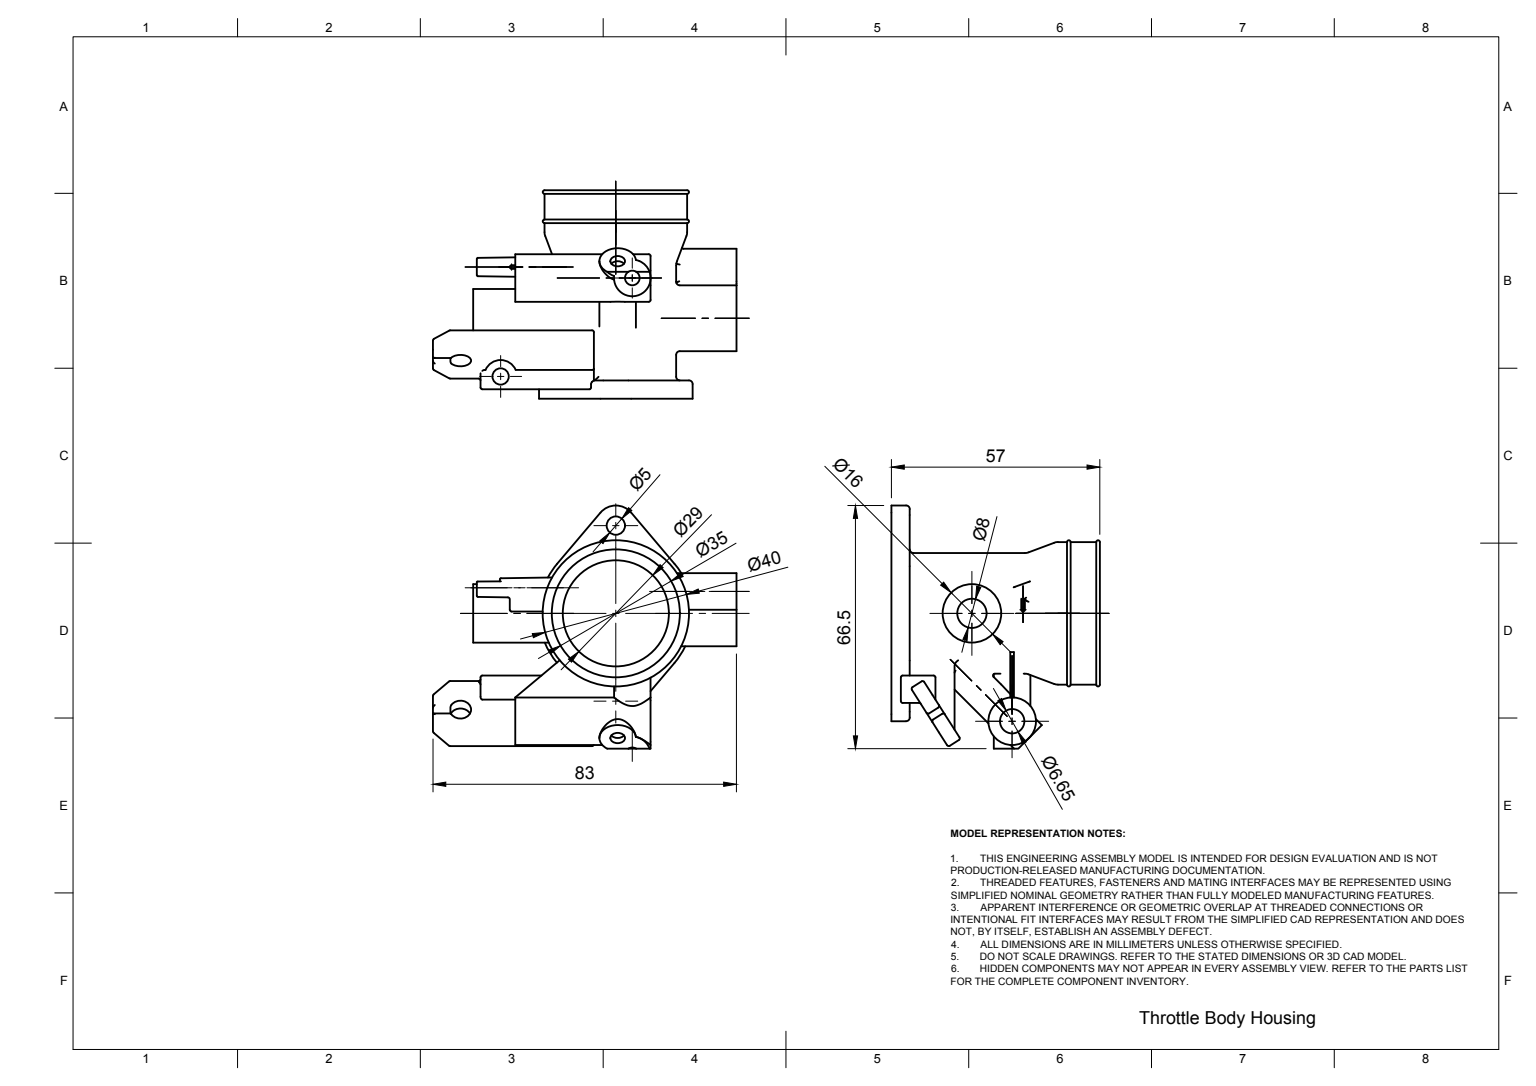
ISO-10303-21;
HEADER;
/* Generated by software containing ST-Developer
 * from STEP Tools, Inc. (www.steptools.com) 
 */

FILE_DESCRIPTION(
/* description */ ('STEP AP214'),
/* implementation_level */ '2;1');

FILE_NAME(
/* name */ 'Throttle Body Housing.step',
/* time_stamp */ '2026-10-07T12:18:07-07:00',
/* author */ (''),
/* organization */ (''),
/* preprocessor_version */ 'ST-DEVELOPER v20.2',
/* originating_system */ 'Autodesk Translation Framework v15.15.0.0',
/* authorisation */ '');

FILE_SCHEMA (('AUTOMOTIVE_DESIGN { 1 0 10303 214 3 1 1 }'));
ENDSEC;

DATA;
#10=MECHANICAL_DESIGN_GEOMETRIC_PRESENTATION_REPRESENTATION('',(#130),#62974);
#83=SPHERICAL_SURFACE('',#16593,0.5);
#84=SPHERICAL_SURFACE('',#16603,0.5);
#85=SPHERICAL_SURFACE('',#16608,0.5);
#86=SPHERICAL_SURFACE('',#16674,0.5);
#87=SPHERICAL_SURFACE('',#16680,0.5);
#88=SPHERICAL_SURFACE('',#16687,0.5);
#89=SPHERICAL_SURFACE('',#16695,0.5);
#90=SPHERICAL_SURFACE('',#16702,0.5);
#91=SPHERICAL_SURFACE('',#16709,0.5);
#92=SPHERICAL_SURFACE('',#16717,0.5);
#93=SPHERICAL_SURFACE('',#16725,0.5);
#94=SPHERICAL_SURFACE('',#16730,0.5);
#95=SPHERICAL_SURFACE('',#16733,0.5);
#96=SPHERICAL_SURFACE('',#16778,0.5);
#97=SPHERICAL_SURFACE('',#16816,1.);
#106=SHAPE_REPRESENTATION_RELATIONSHIP('SRR','None',#63029,#118);
#118=ADVANCED_BREP_SHAPE_REPRESENTATION('',(#142),#62970);
#130=STYLED_ITEM('',(#63090),#142);
#142=MANIFOLD_SOLID_BREP('Body1',#15200);
#168=(
BOUNDED_SURFACE()
B_SPLINE_SURFACE(3,2,((#50715,#50716,#50717),(#50718,#50719,#50720),(#50721,
#50722,#50723),(#50724,#50725,#50726),(#50727,#50728,#50729),(#50730,#50731,
#50732),(#50733,#50734,#50735),(#50736,#50737,#50738),(#50739,#50740,#50741),
(#50742,#50743,#50744),(#50745,#50746,#50747),(#50748,#50749,#50750),(#50751,
#50752,#50753),(#50754,#50755,#50756),(#50757,#50758,#50759),(#50760,#50761,
#50762),(#50763,#50764,#50765),(#50766,#50767,#50768),(#50769,#50770,#50771),
(#50772,#50773,#50774),(#50775,#50776,#50777),(#50778,#50779,#50780),(#50781,
#50782,#50783),(#50784,#50785,#50786),(#50787,#50788,#50789),(#50790,#50791,
#50792),(#50793,#50794,#50795),(#50796,#50797,#50798),(#50799,#50800,#50801),
(#50802,#50803,#50804),(#50805,#50806,#50807),(#50808,#50809,#50810),(#50811,
#50812,#50813),(#50814,#50815,#50816),(#50817,#50818,#50819),(#50820,#50821,
#50822),(#50823,#50824,#50825),(#50826,#50827,#50828),(#50829,#50830,#50831),
(#50832,#50833,#50834),(#50835,#50836,#50837),(#50838,#50839,#50840),(#50841,
#50842,#50843),(#50844,#50845,#50846),(#50847,#50848,#50849),(#50850,#50851,
#50852),(#50853,#50854,#50855),(#50856,#50857,#50858),(#50859,#50860,#50861),
(#50862,#50863,#50864),(#50865,#50866,#50867),(#50868,#50869,#50870),(#50871,
#50872,#50873),(#50874,#50875,#50876),(#50877,#50878,#50879),(#50880,#50881,
#50882),(#50883,#50884,#50885),(#50886,#50887,#50888),(#50889,#50890,#50891),
(#50892,#50893,#50894),(#50895,#50896,#50897),(#50898,#50899,#50900),(#50901,
#50902,#50903),(#50904,#50905,#50906),(#50907,#50908,#50909),(#50910,#50911,
#50912),(#50913,#50914,#50915),(#50916,#50917,#50918),(#50919,#50920,#50921),
(#50922,#50923,#50924),(#50925,#50926,#50927),(#50928,#50929,#50930),(#50931,
#50932,#50933),(#50934,#50935,#50936),(#50937,#50938,#50939),(#50940,#50941,
#50942),(#50943,#50944,#50945),(#50946,#50947,#50948),(#50949,#50950,#50951),
(#50952,#50953,#50954),(#50955,#50956,#50957),(#50958,#50959,#50960),(#50961,
#50962,#50963),(#50964,#50965,#50966),(#50967,#50968,#50969),(#50970,#50971,
#50972),(#50973,#50974,#50975),(#50976,#50977,#50978),(#50979,#50980,#50981),
(#50982,#50983,#50984),(#50985,#50986,#50987),(#50988,#50989,#50990),(#50991,
#50992,#50993),(#50994,#50995,#50996),(#50997,#50998,#50999),(#51000,#51001,
#51002),(#51003,#51004,#51005),(#51006,#51007,#51008),(#51009,#51010,#51011),
(#51012,#51013,#51014),(#51015,#51016,#51017),(#51018,#51019,#51020),(#51021,
#51022,#51023),(#51024,#51025,#51026),(#51027,#51028,#51029),(#51030,#51031,
#51032),(#51033,#51034,#51035),(#51036,#51037,#51038),(#51039,#51040,#51041),
(#51042,#51043,#51044),(#51045,#51046,#51047),(#51048,#51049,#51050),(#51051,
#51052,#51053),(#51054,#51055,#51056),(#51057,#51058,#51059),(#51060,#51061,
#51062),(#51063,#51064,#51065),(#51066,#51067,#51068),(#51069,#51070,#51071),
(#51072,#51073,#51074),(#51075,#51076,#51077),(#51078,#51079,#51080),(#51081,
#51082,#51083),(#51084,#51085,#51086),(#51087,#51088,#51089),(#51090,#51091,
#51092),(#51093,#51094,#51095),(#51096,#51097,#51098),(#51099,#51100,#51101),
(#51102,#51103,#51104),(#51105,#51106,#51107),(#51108,#51109,#51110),(#51111,
#51112,#51113),(#51114,#51115,#51116),(#51117,#51118,#51119),(#51120,#51121,
#51122),(#51123,#51124,#51125),(#51126,#51127,#51128),(#51129,#51130,#51131),
(#51132,#51133,#51134),(#51135,#51136,#51137),(#51138,#51139,#51140),(#51141,
#51142,#51143),(#51144,#51145,#51146),(#51147,#51148,#51149),(#51150,#51151,
#51152),(#51153,#51154,#51155),(#51156,#51157,#51158),(#51159,#51160,#51161),
(#51162,#51163,#51164),(#51165,#51166,#51167),(#51168,#51169,#51170),(#51171,
#51172,#51173),(#51174,#51175,#51176),(#51177,#51178,#51179),(#51180,#51181,
#51182),(#51183,#51184,#51185),(#51186,#51187,#51188),(#51189,#51190,#51191),
(#51192,#51193,#51194),(#51195,#51196,#51197),(#51198,#51199,#51200),(#51201,
#51202,#51203),(#51204,#51205,#51206),(#51207,#51208,#51209),(#51210,#51211,
#51212),(#51213,#51214,#51215),(#51216,#51217,#51218),(#51219,#51220,#51221),
(#51222,#51223,#51224),(#51225,#51226,#51227),(#51228,#51229,#51230),(#51231,
#51232,#51233),(#51234,#51235,#51236),(#51237,#51238,#51239),(#51240,#51241,
#51242),(#51243,#51244,#51245),(#51246,#51247,#51248),(#51249,#51250,#51251),
(#51252,#51253,#51254),(#51255,#51256,#51257),(#51258,#51259,#51260),(#51261,
#51262,#51263),(#51264,#51265,#51266),(#51267,#51268,#51269),(#51270,#51271,
#51272),(#51273,#51274,#51275),(#51276,#51277,#51278),(#51279,#51280,#51281),
(#51282,#51283,#51284),(#51285,#51286,#51287),(#51288,#51289,#51290),(#51291,
#51292,#51293),(#51294,#51295,#51296),(#51297,#51298,#51299),(#51300,#51301,
#51302),(#51303,#51304,#51305),(#51306,#51307,#51308),(#51309,#51310,#51311),
(#51312,#51313,#51314),(#51315,#51316,#51317),(#51318,#51319,#51320),(#51321,
#51322,#51323),(#51324,#51325,#51326),(#51327,#51328,#51329),(#51330,#51331,
#51332),(#51333,#51334,#51335),(#51336,#51337,#51338),(#51339,#51340,#51341),
(#51342,#51343,#51344),(#51345,#51346,#51347),(#51348,#51349,#51350),(#51351,
#51352,#51353),(#51354,#51355,#51356),(#51357,#51358,#51359),(#51360,#51361,
#51362),(#51363,#51364,#51365),(#51366,#51367,#51368),(#51369,#51370,#51371),
(#51372,#51373,#51374),(#51375,#51376,#51377),(#51378,#51379,#51380),(#51381,
#51382,#51383),(#51384,#51385,#51386),(#51387,#51388,#51389),(#51390,#51391,
#51392),(#51393,#51394,#51395),(#51396,#51397,#51398),(#51399,#51400,#51401),
(#51402,#51403,#51404),(#51405,#51406,#51407),(#51408,#51409,#51410),(#51411,
#51412,#51413),(#51414,#51415,#51416),(#51417,#51418,#51419),(#51420,#51421,
#51422),(#51423,#51424,#51425),(#51426,#51427,#51428),(#51429,#51430,#51431),
(#51432,#51433,#51434),(#51435,#51436,#51437),(#51438,#51439,#51440),(#51441,
#51442,#51443),(#51444,#51445,#51446),(#51447,#51448,#51449),(#51450,#51451,
#51452),(#51453,#51454,#51455),(#51456,#51457,#51458),(#51459,#51460,#51461),
(#51462,#51463,#51464),(#51465,#51466,#51467),(#51468,#51469,#51470),(#51471,
#51472,#51473),(#51474,#51475,#51476),(#51477,#51478,#51479),(#51480,#51481,
#51482),(#51483,#51484,#51485),(#51486,#51487,#51488),(#51489,#51490,#51491),
(#51492,#51493,#51494),(#51495,#51496,#51497),(#51498,#51499,#51500)),
 .UNSPECIFIED.,.T.,.F.,.F.)
B_SPLINE_SURFACE_WITH_KNOTS((4,2,2,2,2,2,2,2,2,2,2,2,2,2,2,2,2,2,2,2,2,
2,2,2,2,2,2,2,2,2,2,2,2,2,2,2,2,2,2,2,2,2,2,2,2,2,2,2,2,2,2,2,2,2,2,2,2,
2,2,2,2,2,2,2,2,2,2,2,2,2,2,2,2,2,2,2,2,2,2,2,2,2,2,2,2,2,2,2,2,2,2,2,2,
2,2,2,2,2,2,2,2,2,2,2,2,2,2,2,2,2,2,2,2,2,2,2,2,2,2,2,2,2,2,2,2,2,2,2,2,
2,4),(3,3),(0.,5.58974039156775E-5,0.000111794807831355,0.00022358961566271,
0.00044717923132542,0.000894358462650841,0.00178871692530168,0.00268307538795252,
0.00279487019578388,0.00290666500361523,0.00313025461927794,0.00357743385060336,
0.0044717923132542,0.00536615077590504,0.0054779455837364,0.00558974039156775,
0.00581333000723046,0.00626050923855589,0.00715486770120673,0.00804922616385757,
0.00827281577952028,0.00838461058735163,0.00849640539518299,0.00894358462650841,
0.00983794308915925,0.0107323015518101,0.0111794807831355,0.0114030703987982,
0.0115148652066296,0.0116266600144609,0.0125210184771118,0.0134153769397626,
0.013862556171088,0.0143097354024135,0.0145333250180762,0.0146451198259075,
0.0147569146337389,0.0152040938650643,0.0160984523277151,0.016992810790366,
0.0172164004060287,0.01732819521386,0.0174399900216914,0.0178871692530168,
0.0187815277156677,0.0196758861783185,0.0198994757939812,0.0201230654096439,
0.0205702446409693,0.0214646031036202,0.022358961566271,0.0228061407975964,
0.0230297304132591,0.0232533200289219,0.0241476784915727,0.0250420369542235,
0.0259363954168744,0.0261599850325371,0.0262717798403685,0.0263835746481998,
0.0268307538795252,0.0277251123421761,0.0286194708048269,0.0290666500361523,
0.029290239651815,0.0294020344596464,0.0295138292674777,0.0299610084988032,
0.0301845981144659,0.0302963929222972,0.0304081877301286,0.0313025461927794,
0.0321969046554303,0.0330912631180811,0.0332030579259125,0.0333148527337438,
0.0335384423494065,0.0339856215807319,0.0348799800433828,0.0357743385060336,
0.0359979281216963,0.0361097229295277,0.036221517737359,0.0366686969686845,
0.0375630554313353,0.0384574138939862,0.0389045931253116,0.0391281827409743,
0.0392399775488056,0.039351772356637,0.0402461308192878,0.0411404892819387,
0.0420348477445895,0.0424820269759149,0.0425938217837463,0.0427056165915777,
0.0429292062072404,0.0433763854385658,0.0438235646698912,0.044717923132542,
0.0451651023638675,0.0452768971716988,0.0453886919795302,0.0456122815951929,
0.0465066400578437,0.0474009985204946,0.04784817775182,0.0479599725596513,
0.0480717673674827,0.0482953569831454,0.0491897154457962,0.0500840739084471,
0.0505312531397725,0.0507548427554352,0.0508666375632666,0.0509784323710979,
0.0518727908337488,0.0527671492963996,0.0536615077590504,0.0538850973747132,
0.0539968921825445,0.0541086869903759,0.0545558662217013,0.0554502246843521,
0.056344583147003,0.0567917623783284,0.0570153519939911,0.0571271468018225,
0.0571830442057381,0.057210992907696,0.0572389416096538),(0.,1.),
 .UNSPECIFIED.)
GEOMETRIC_REPRESENTATION_ITEM()
RATIONAL_B_SPLINE_SURFACE(((1.,0.869037098890924,1.),(1.,0.869090662160833,
1.),(1.,0.869142132128297,1.),(1.,0.869241273997536,1.),(1.,0.869288882663707,
1.),(1.,0.869425835273797,1.),(1.,0.869509305917427,1.),(1.,0.869736328335375,
1.),(1.,0.869856492063896,1.),(1.,0.870124205131434,1.),(1.,0.870178998389397,
1.),(1.,0.869977707911342,1.),(1.,0.869356264735848,1.),(1.,0.867159523791841,
1.),(1.,0.865584183970151,1.),(1.,0.863281618119441,1.),(1.,0.86301835474559,
1.),(1.,0.862477312320675,1.),(1.,0.862200065545979,1.),(1.,0.861348450829986,
1.),(1.,0.860754210958995,1.),(1.,0.858894323573958,1.),(1.,0.857551540639133,
1.),(1.,0.853231873120265,1.),(1.,0.849963976579328,1.),(1.,0.8427337476379,
1.),(1.,0.838771159914112,1.),(1.,0.833964492549446,1.),(1.,0.83342564158097,
1.),(1.,0.832341102831786,1.),(1.,0.831795088875303,1.),(1.,0.83014615568217,
1.),(1.,0.829032346207458,1.),(1.,0.825650047625046,1.),(1.,0.823340697393356,
1.),(1.,0.816270214875414,1.),(1.,0.811366531889991,1.),(1.,0.801290493401484,
1.),(1.,0.796117786007922,1.),(1.,0.789558114002489,1.),(1.,0.788241524410975,
1.),(1.,0.786261176106014,1.),(1.,0.785600666410631,1.),(1.,0.784281253478811,
1.),(1.,0.783622032027989,1.),(1.,0.780329023537139,1.),(1.,0.777704514650253,
1.),(1.,0.76988692542286,1.),(1.,0.764749330047637,1.),(1.,0.75477051537079,
1.),(1.,0.749929030998746,1.),(1.,0.743012971461713,1.),(1.,0.740765474239869,
1.),(1.,0.73749827976927,1.),(1.,0.736426570328376,1.),(1.,0.734847329496033,
1.),(1.,0.734325595116705,1.),(1.,0.733292134556225,1.),(1.,0.732781563072735,
1.),(1.,0.728242967029025,1.),(1.,0.724610876621003,1.),(1.,0.718276943716503,
1.),(1.,0.715575135642169,1.),(1.,0.712312229125148,1.),(1.,0.711356200483893,
1.),(1.,0.709722323386846,1.),(1.,0.709044475655852,1.),(1.,0.708247344579823,
1.),(1.,0.708018238565296,1.),(1.,0.707730840005604,1.),(1.,0.707644376240716,
1.),(1.,0.707490608795043,1.),(1.,0.707423402545753,1.),(1.,0.707135559015692,
1.),(1.,0.707059523314824,1.),(1.,0.707285549205988,1.),(1.,0.708042221657254,
1.),(1.,0.710710092253751,1.),(1.,0.712621237041365,1.),(1.,0.715686665981657,
1.),(1.,0.716333543550958,1.),(1.,0.717353607349392,1.),(1.,0.717701919486094,
1.),(1.,0.718414964313171,1.),(1.,0.718779962361759,1.),(1.,0.720642167884513,
1.),(1.,0.722248110686464,1.),(1.,0.727379897082438,1.),(1.,0.731219242886661,
1.),(1.,0.739562059134817,1.),(1.,0.744065650037015,1.),(1.,0.750011006364496,
1.),(1.,0.751215898212902,1.),(1.,0.753654939425893,1.),(1.,0.754889413958793,
1.),(1.,0.758631191877784,1.),(1.,0.761160349547001,1.),(1.,0.768820010203822,
1.),(1.,0.774022074432147,1.),(1.,0.784467204631247,1.),(1.,0.789710609506525,
1.),(1.,0.797506397811445,1.),(1.,0.800093535602747,1.),(1.,0.803945021596591,
1.),(1.,0.805223982229172,1.),(1.,0.807770172561434,1.),(1.,0.80903292134295,
1.),(1.,0.815288089794111,1.),(1.,0.820107499923359,1.),(1.,0.829279685729609,
1.),(1.,0.833632779776828,1.),(1.,0.841777168809211,1.),(1.,0.845568802174027,
1.),(1.,0.849892563199079,1.),(1.,0.850736491533872,1.),(1.,0.851969804909359,
1.),(1.,0.852375793676684,1.),(1.,0.853174988795519,1.),(1.,0.853568068159912,
1.),(1.,0.855500704900974,1.),(1.,0.856941996550435,1.),(1.,0.860944601199298,
1.),(1.,0.863184927882986,1.),(1.,0.866767461005655,1.),(1.,0.868109793594765,
1.),(1.,0.869410481594525,1.),(1.,0.869725148569242,1.),(1.,0.870012890040282,
1.),(1.,0.870078086396283,1.),(1.,0.870128990964309,1.),(1.,0.870138141570321,
1.),(1.,0.870140676091054,1.),(1.,0.870134072965078,1.),(1.,0.870061808448095,
1.),(1.,0.869878426760649,1.),(1.,0.869416656440071,1.),(1.,0.869231611413219,
1.),(1.,0.868907522254946,1.),(1.,0.868791738615037,1.),(1.,0.868544686539316,
1.),(1.,0.868413337134317,1.),(1.,0.867163505604549,1.),(1.,0.865575442228637,
1.),(1.,0.861527724393334,1.),(1.,0.859067845844723,1.),(1.,0.853343564886148,
1.),(1.,0.850078971827717,1.),(1.,0.84598647975218,1.),(1.,0.845525923915504,
1.),(1.,0.844593252383724,1.),(1.,0.84412081177775,1.),(1.,0.842688930644052,
1.),(1.,0.841715504172781,1.),(1.,0.83874140215334,1.),(1.,0.836686926299113,
1.),(1.,0.830328826430023,1.),(1.,0.825830615536545,1.),(1.,0.816419106847222,
1.),(1.,0.81150547118942,1.),(1.,0.805169234170547,1.),(1.,0.803892294076685,
1.),(1.,0.801963643202623,1.),(1.,0.801318553163188,1.),(1.,0.800024181787751,
1.),(1.,0.799374551464301,1.),(1.,0.796123838581708,1.),(1.,0.793511112507122,
1.),(1.,0.785661232785625,1.),(1.,0.780412024366977,1.),(1.,0.770019050951368,
1.),(1.,0.76487497595969,1.),(1.,0.757351702086758,1.),(1.,0.754876228736365,
1.),(1.,0.751227350622943,1.),(1.,0.750021792912108,1.),(1.,0.748231675946372,
1.),(1.,0.747638007827609,1.),(1.,0.746457111568753,1.),(1.,0.745869506104255,
1.),(1.,0.740620037686994,1.),(1.,0.736256100649653,1.),(1.,0.728276221758877,
1.),(1.,0.724660242842317,1.),(1.,0.718324000111086,1.),(1.,0.715603718055959,
1.),(1.,0.712309706535428,1.),(1.,0.711342812014489,1.),(1.,0.710310353740139,
1.),(1.,0.710112755568336,1.),(1.,0.709736703375217,1.),(1.,0.709558069154282,
1.),(1.,0.709050371012769,1.),(1.,0.708749513760786,1.),(1.,0.70795992094024,
1.),(1.,0.707584199551303,1.),(1.,0.707134092959367,1.),(1.,0.70705970821773,
1.),(1.,0.707286843642986,1.),(1.,0.70803921126881,1.),(1.,0.710052147725902,
1.),(1.,0.710870383211632,1.),(1.,0.71207445357331,1.),(1.,0.712324328892365,
1.),(1.,0.712842122035176,1.),(1.,0.713110243316174,1.),(1.,0.713939993830723,
1.),(1.,0.714526359388936,1.),(1.,0.717617638747993,1.),(1.,0.720600584023788,
1.),(1.,0.727424242013839,1.),(1.,0.731264995819141,1.),(1.,0.737553652730096,
1.),(1.,0.739737848764794,1.),(1.,0.742566372039795,1.),(1.,0.74313699147918,
1.),(1.,0.744287770846871,1.),(1.,0.744868257643384,1.),(1.,0.746621209706891,
1.),(1.,0.747803690023989,1.),(1.,0.753778025133493,1.),(1.,0.758754654573864,
1.),(1.,0.768933369155768,1.),(1.,0.774135775395061,1.),(1.,0.781997810487323,
1.),(1.,0.784628358204622,1.),(1.,0.788575987637978,1.),(1.,0.789892170142193,
1.),(1.,0.791865311260895,1.),(1.,0.792522836387841,1.),(1.,0.793837245909085,
1.),(1.,0.794493861510745,1.),(1.,0.800385048001281,1.),(1.,0.80551453306944,
1.),(1.,0.815446188856963,1.),(1.,0.820248709446964,1.),(1.,0.829421742411055,
1.),(1.,0.833792601959078,1.),(1.,0.838919085477355,1.),(1.,0.839927506491091,
1.),(1.,0.841413476855047,1.),(1.,0.841904356336916,1.),(1.,0.842876996646255,
1.),(1.,0.843358860518912,1.),(1.,0.845737639832195,1.),(1.,0.847548776311049,
1.),(1.,0.852696372188048,1.),(1.,0.855747262756165,1.),(1.,0.861029201702321,
1.),(1.,0.863260436478246,1.),(1.,0.865941546711405,1.),(1.,0.86672419811369,
1.),(1.,0.867724144067475,1.),(1.,0.868028445735918,1.),(1.,0.868440362182281,
1.),(1.,0.868570244374482,1.),(1.,0.868753799883508,1.),(1.,0.868813107052922,
1.),(1.,0.868899233803952,1.),(1.,0.868927470387005,1.),(1.,0.868982996012711,
1.),(1.,0.86901031725597,1.),(1.,0.869037098890924,1.)))
REPRESENTATION_ITEM('')
SURFACE()
);
#169=(
BOUNDED_SURFACE()
B_SPLINE_SURFACE(3,2,((#52221,#52222,#52223),(#52224,#52225,#52226),(#52227,
#52228,#52229),(#52230,#52231,#52232),(#52233,#52234,#52235),(#52236,#52237,
#52238),(#52239,#52240,#52241),(#52242,#52243,#52244),(#52245,#52246,#52247),
(#52248,#52249,#52250),(#52251,#52252,#52253),(#52254,#52255,#52256),(#52257,
#52258,#52259),(#52260,#52261,#52262),(#52263,#52264,#52265),(#52266,#52267,
#52268),(#52269,#52270,#52271),(#52272,#52273,#52274),(#52275,#52276,#52277),
(#52278,#52279,#52280),(#52281,#52282,#52283),(#52284,#52285,#52286),(#52287,
#52288,#52289),(#52290,#52291,#52292),(#52293,#52294,#52295),(#52296,#52297,
#52298),(#52299,#52300,#52301),(#52302,#52303,#52304),(#52305,#52306,#52307),
(#52308,#52309,#52310),(#52311,#52312,#52313),(#52314,#52315,#52316),(#52317,
#52318,#52319),(#52320,#52321,#52322),(#52323,#52324,#52325),(#52326,#52327,
#52328),(#52329,#52330,#52331),(#52332,#52333,#52334),(#52335,#52336,#52337),
(#52338,#52339,#52340),(#52341,#52342,#52343),(#52344,#52345,#52346),(#52347,
#52348,#52349),(#52350,#52351,#52352),(#52353,#52354,#52355),(#52356,#52357,
#52358),(#52359,#52360,#52361),(#52362,#52363,#52364),(#52365,#52366,#52367),
(#52368,#52369,#52370),(#52371,#52372,#52373),(#52374,#52375,#52376),(#52377,
#52378,#52379),(#52380,#52381,#52382),(#52383,#52384,#52385),(#52386,#52387,
#52388),(#52389,#52390,#52391),(#52392,#52393,#52394),(#52395,#52396,#52397),
(#52398,#52399,#52400),(#52401,#52402,#52403),(#52404,#52405,#52406),(#52407,
#52408,#52409),(#52410,#52411,#52412),(#52413,#52414,#52415),(#52416,#52417,
#52418),(#52419,#52420,#52421),(#52422,#52423,#52424),(#52425,#52426,#52427),
(#52428,#52429,#52430),(#52431,#52432,#52433),(#52434,#52435,#52436),(#52437,
#52438,#52439),(#52440,#52441,#52442),(#52443,#52444,#52445),(#52446,#52447,
#52448),(#52449,#52450,#52451),(#52452,#52453,#52454),(#52455,#52456,#52457),
(#52458,#52459,#52460),(#52461,#52462,#52463),(#52464,#52465,#52466),(#52467,
#52468,#52469),(#52470,#52471,#52472),(#52473,#52474,#52475),(#52476,#52477,
#52478),(#52479,#52480,#52481),(#52482,#52483,#52484),(#52485,#52486,#52487),
(#52488,#52489,#52490),(#52491,#52492,#52493),(#52494,#52495,#52496),(#52497,
#52498,#52499),(#52500,#52501,#52502),(#52503,#52504,#52505),(#52506,#52507,
#52508),(#52509,#52510,#52511),(#52512,#52513,#52514),(#52515,#52516,#52517),
(#52518,#52519,#52520),(#52521,#52522,#52523),(#52524,#52525,#52526),(#52527,
#52528,#52529),(#52530,#52531,#52532),(#52533,#52534,#52535),(#52536,#52537,
#52538),(#52539,#52540,#52541),(#52542,#52543,#52544),(#52545,#52546,#52547),
(#52548,#52549,#52550),(#52551,#52552,#52553),(#52554,#52555,#52556),(#52557,
#52558,#52559),(#52560,#52561,#52562),(#52563,#52564,#52565),(#52566,#52567,
#52568),(#52569,#52570,#52571),(#52572,#52573,#52574),(#52575,#52576,#52577),
(#52578,#52579,#52580),(#52581,#52582,#52583),(#52584,#52585,#52586),(#52587,
#52588,#52589),(#52590,#52591,#52592),(#52593,#52594,#52595),(#52596,#52597,
#52598),(#52599,#52600,#52601),(#52602,#52603,#52604),(#52605,#52606,#52607),
(#52608,#52609,#52610),(#52611,#52612,#52613),(#52614,#52615,#52616),(#52617,
#52618,#52619),(#52620,#52621,#52622),(#52623,#52624,#52625),(#52626,#52627,
#52628),(#52629,#52630,#52631),(#52632,#52633,#52634),(#52635,#52636,#52637),
(#52638,#52639,#52640),(#52641,#52642,#52643),(#52644,#52645,#52646),(#52647,
#52648,#52649),(#52650,#52651,#52652),(#52653,#52654,#52655),(#52656,#52657,
#52658),(#52659,#52660,#52661),(#52662,#52663,#52664),(#52665,#52666,#52667),
(#52668,#52669,#52670),(#52671,#52672,#52673),(#52674,#52675,#52676),(#52677,
#52678,#52679),(#52680,#52681,#52682),(#52683,#52684,#52685),(#52686,#52687,
#52688),(#52689,#52690,#52691),(#52692,#52693,#52694),(#52695,#52696,#52697),
(#52698,#52699,#52700),(#52701,#52702,#52703),(#52704,#52705,#52706),(#52707,
#52708,#52709),(#52710,#52711,#52712),(#52713,#52714,#52715),(#52716,#52717,
#52718),(#52719,#52720,#52721),(#52722,#52723,#52724),(#52725,#52726,#52727),
(#52728,#52729,#52730),(#52731,#52732,#52733),(#52734,#52735,#52736),(#52737,
#52738,#52739),(#52740,#52741,#52742),(#52743,#52744,#52745),(#52746,#52747,
#52748),(#52749,#52750,#52751),(#52752,#52753,#52754),(#52755,#52756,#52757),
(#52758,#52759,#52760),(#52761,#52762,#52763),(#52764,#52765,#52766),(#52767,
#52768,#52769),(#52770,#52771,#52772),(#52773,#52774,#52775),(#52776,#52777,
#52778),(#52779,#52780,#52781),(#52782,#52783,#52784),(#52785,#52786,#52787),
(#52788,#52789,#52790),(#52791,#52792,#52793),(#52794,#52795,#52796),(#52797,
#52798,#52799),(#52800,#52801,#52802),(#52803,#52804,#52805),(#52806,#52807,
#52808),(#52809,#52810,#52811),(#52812,#52813,#52814),(#52815,#52816,#52817),
(#52818,#52819,#52820),(#52821,#52822,#52823),(#52824,#52825,#52826),(#52827,
#52828,#52829),(#52830,#52831,#52832),(#52833,#52834,#52835),(#52836,#52837,
#52838),(#52839,#52840,#52841),(#52842,#52843,#52844),(#52845,#52846,#52847),
(#52848,#52849,#52850),(#52851,#52852,#52853),(#52854,#52855,#52856),(#52857,
#52858,#52859),(#52860,#52861,#52862),(#52863,#52864,#52865),(#52866,#52867,
#52868),(#52869,#52870,#52871),(#52872,#52873,#52874),(#52875,#52876,#52877),
(#52878,#52879,#52880),(#52881,#52882,#52883),(#52884,#52885,#52886),(#52887,
#52888,#52889),(#52890,#52891,#52892),(#52893,#52894,#52895),(#52896,#52897,
#52898),(#52899,#52900,#52901),(#52902,#52903,#52904),(#52905,#52906,#52907),
(#52908,#52909,#52910),(#52911,#52912,#52913),(#52914,#52915,#52916),(#52917,
#52918,#52919),(#52920,#52921,#52922),(#52923,#52924,#52925),(#52926,#52927,
#52928),(#52929,#52930,#52931),(#52932,#52933,#52934),(#52935,#52936,#52937),
(#52938,#52939,#52940),(#52941,#52942,#52943),(#52944,#52945,#52946),(#52947,
#52948,#52949),(#52950,#52951,#52952),(#52953,#52954,#52955),(#52956,#52957,
#52958),(#52959,#52960,#52961),(#52962,#52963,#52964),(#52965,#52966,#52967),
(#52968,#52969,#52970),(#52971,#52972,#52973),(#52974,#52975,#52976),(#52977,
#52978,#52979),(#52980,#52981,#52982),(#52983,#52984,#52985),(#52986,#52987,
#52988),(#52989,#52990,#52991),(#52992,#52993,#52994),(#52995,#52996,#52997),
(#52998,#52999,#53000),(#53001,#53002,#53003),(#53004,#53005,#53006),(#53007,
#53008,#53009),(#53010,#53011,#53012),(#53013,#53014,#53015),(#53016,#53017,
#53018)),.UNSPECIFIED.,.T.,.F.,.F.)
B_SPLINE_SURFACE_WITH_KNOTS((4,2,2,2,2,2,2,2,2,2,2,2,2,2,2,2,2,2,2,2,2,
2,2,2,2,2,2,2,2,2,2,2,2,2,2,2,2,2,2,2,2,2,2,2,2,2,2,2,2,2,2,2,2,2,2,2,2,
2,2,2,2,2,2,2,2,2,2,2,2,2,2,2,2,2,2,2,2,2,2,2,2,2,2,2,2,2,2,2,2,2,2,2,2,
2,2,2,2,2,2,2,2,2,2,2,2,2,2,2,2,2,2,2,2,2,2,2,2,2,2,2,2,2,2,2,2,2,2,2,2,
2,2,2,4),(3,3),(0.,4.12881615541384E-5,8.25763231082768E-5,0.000165152646216554,
0.000330305292433107,0.000660610584866214,0.000990915877299321,0.00132122116973243,
0.00148637381594898,0.00156895013905726,0.00165152646216554,0.00198183175459864,
0.00264244233946486,0.00297274763189796,0.00313790027811452,0.00322047660122279,
0.00330305292433107,0.00396366350919728,0.0046242740940635,0.00495457938649661,
0.00503715570960488,0.00511973203271316,0.00528488467892971,0.00594549526379593,
0.00660610584866214,0.00693641114109525,0.00701898746420353,0.0071015637873118,
0.00726671643352836,0.00792732701839457,0.00858793760326078,0.009248548188127,
0.00990915877299321,0.0100743114192098,0.0102394640654263,0.0105697693578594,
0.0112303799427256,0.0118909905275919,0.0125516011124581,0.0132122116973243,
0.0138728222821905,0.0139553986052988,0.0140379749284071,0.0142031275746236,
0.0145334328670567,0.0151940434519229,0.0158546540367891,0.0165152646216554,
0.0166804172678719,0.0168455699140885,0.0171758752065216,0.0175061804989547,
0.0178364857913878,0.0181667910838209,0.0183319437300374,0.0184145200531457,
0.018497096376254,0.0188274016686871,0.0191577069611202,0.0194880122535533,
0.0196531648997699,0.0197357412228781,0.0198183175459864,0.0201486228384195,
0.0204789281308526,0.0208092334232857,0.020891809746394,0.0209743860695023,
0.0211395387157189,0.021469844008152,0.0215524203312602,0.0216349966543685,
0.0218001493005851,0.0221304545930182,0.0224607598854513,0.0227910651778844,
0.0231213704703175,0.0232039467934258,0.023286523116534,0.0234516757627506,
0.0237819810551837,0.0241122863476168,0.0244425916400499,0.0251032022249161,
0.0252683548711327,0.0254335075173492,0.0257638128097823,0.0264244233946486,
0.0270850339795148,0.027745644564381,0.0284062551492472,0.0285714077954638,
0.0287365604416803,0.0290668657341134,0.0297274763189796,0.0303880869038458,
0.0310486974887121,0.0317093080735783,0.0320396133660114,0.0322047660122279,
0.0323699186584445,0.0330305292433107,0.0336911398281769,0.0343517504130431,
0.0346820557054762,0.0348472083516928,0.0349297846748011,0.0350123609979093,
0.0356729715827756,0.0363335821676418,0.036994192752508,0.0370767690756163,
0.0371593453987245,0.0373244980449411,0.0376548033373742,0.0383154139222404,
0.0386457192146735,0.0388108718608901,0.0389760245071066,0.0396366350919728,
0.039966940384406,0.0402972456768391,0.0404623983230556,0.0405449746461639,
0.0406275509692722,0.0409578562617053,0.0412881615541384,0.0416184668465715,
0.0419487721390046,0.0421139247852211,0.0421965011083294,0.0422377892698836,
0.0422790774314377),(0.,1.),.UNSPECIFIED.)
GEOMETRIC_REPRESENTATION_ITEM()
RATIONAL_B_SPLINE_SURFACE(((1.,0.923590675042016,1.),(1.,0.923572320945391,
1.),(1.,0.923553587090577,1.),(1.,0.923515495478205,1.),(1.,0.923496115237016,
1.),(1.,0.923436971524286,1.),(1.,0.923396205307423,1.),(1.,0.923269889059141,
1.),(1.,0.923180325181551,1.),(1.,0.922895385428438,1.),(1.,0.922683818431749,
1.),(1.,0.922215055006499,1.),(1.,0.921957857869856,1.),(1.,0.921393597668949,
1.),(1.,0.921086537396165,1.),(1.,0.920583987620736,1.),(1.,0.920409463147971,
1.),(1.,0.920136456599823,1.),(1.,0.920043583473226,1.),(1.,0.919853965179493,
1.),(1.,0.919757130552995,1.),(1.,0.919264385051497,1.),(1.,0.918842556687909,
1.),(1.,0.917485342839882,1.),(1.,0.916458802712932,1.),(1.,0.914690614339645,
1.),(1.,0.914063012700798,1.),(1.,0.913057237216573,1.),(1.,0.912711240257362,
1.),(1.,0.912175163335873,1.),(1.,0.911993623483323,1.),(1.,0.911624678363091,
1.),(1.,0.911437120441042,1.),(1.,0.909726149783902,1.),(1.,0.908041888239718,
1.),(1.,0.904290424256204,1.),(1.,0.90222325436422,1.),(1.,0.898787650803265,
1.),(1.,0.897586580689637,1.),(1.,0.896009931734525,1.),(1.,0.895690686714278,
1.),(1.,0.895045201490737,1.),(1.,0.894719248531258,1.),(1.,0.893731649644609,
1.),(1.,0.893060263975502,1.),(1.,0.889636937842127,1.),(1.,0.886685904879282,
1.),(1.,0.880320125821774,1.),(1.,0.876905428959452,1.),(1.,0.871403913130991,
1.),(1.,0.869506798646649,1.),(1.,0.867052723787093,1.),(1.,0.866557553196408,
1.),(1.,0.865560870035344,1.),(1.,0.865059173595903,1.),(1.,0.863543964995002,
1.),(1.,0.862520333878055,1.),(1.,0.857333970909859,1.),(1.,0.852966736393177,
1.),(1.,0.843775067927313,1.),(1.,0.838950667880686,1.),(1.,0.828820205567495,
1.),(1.,0.823514183332928,1.),(1.,0.812391307349727,1.),(1.,0.806574504385483,
1.),(1.,0.798962220591142,1.),(1.,0.797421706068384,1.),(1.,0.794315888151595,
1.),(1.,0.792749600433445,1.),(1.,0.788010186024153,1.),(1.,0.784796515809518,
1.),(1.,0.77498973461648,1.),(1.,0.768230990620621,1.),(1.,0.754249477539376,
1.),(1.,0.7470267311596,1.),(1.,0.732090338555257,1.),(1.,0.724376719977163,
1.),(1.,0.708426290764442,1.),(1.,0.700189512530531,1.),(1.,0.683154153538125,
1.),(1.,0.674355607127678,1.),(1.,0.664115385685685,1.),(1.,0.66297302996927,
1.),(1.,0.660682162177284,1.),(1.,0.659533241882799,1.),(1.,0.65607598168352,
1.),(1.,0.653757142047767,1.),(1.,0.646758317475323,1.),(1.,0.642036016956393,
1.),(1.,0.627697700195677,1.),(1.,0.61790996153014,1.),(1.,0.597870566155991,
1.),(1.,0.58761854570598,1.),(1.,0.566657940545553,1.),(1.,0.555948596069607,
1.),(1.,0.542299741359184,1.),(1.,0.539556972501121,1.),(1.,0.53404656747395,
1.),(1.,0.531276245933983,1.),(1.,0.522962675372791,1.),(1.,0.517409973114278,
1.),(1.,0.506307878837006,1.),(1.,0.500758405674242,1.),(1.,0.489694670444622,
1.),(1.,0.484180295137749,1.),(1.,0.473229585826254,1.),(1.,0.467793092024575,
1.),(1.,0.459740217505025,1.),(1.,0.457073035061414,1.),(1.,0.453104759629238,
1.),(1.,0.451787428134069,1.),(1.,0.449164897866363,1.),(1.,0.447859036145478,
1.),(1.,0.441385443166445,1.),(1.,0.436368154024372,1.),(1.,0.426750681610345,
1.),(1.,0.422150388759125,1.),(1.,0.413481583263519,1.),(1.,0.409412966405537,
1.),(1.,0.403813005360145,1.),(1.,0.402030377100019,1.),(1.,0.399497383040528,
1.),(1.,0.398676556272897,1.),(1.,0.397084562446663,1.),(1.,0.396315545546773,
1.),(1.,0.392617462025358,1.),(1.,0.390121311666049,1.),(1.,0.386146893571918,
1.),(1.,0.384668848565874,1.),(1.,0.382812549250897,1.),(1.,0.382434470212711,
1.),(1.,0.38268919558194,1.),(1.,0.382776371338327,1.),(1.,0.383022089646797,
1.),(1.,0.383180660969252,1.),(1.,0.383762017423613,1.),(1.,0.384290482158863,
1.),(1.,0.386285206501931,1.),(1.,0.388161225874796,1.),(1.,0.391136736543832,
1.),(1.,0.391763914323658,1.),(1.,0.393077192923473,1.),(1.,0.393761818570545,
1.),(1.,0.395895524715283,1.),(1.,0.397424386821021,1.),(1.,0.402298884562898,
1.),(1.,0.405931683845182,1.),(1.,0.413815239487506,1.),(1.,0.418066059410145,
1.),(1.,0.42706069079461,1.),(1.,0.431804585246568,1.),(1.,0.441681473676376,
1.),(1.,0.446814558722576,1.),(1.,0.453420699181124,1.),(1.,0.454748719848507,
1.),(1.,0.457413317151073,1.),(1.,0.458750495400507,1.),(1.,0.462774945482169,
1.),(1.,0.465475093536882,1.),(1.,0.473614842385458,1.),(1.,0.479093267976819,
1.),(1.,0.490102288950609,1.),(1.,0.495633034030675,1.),(1.,0.506709011958283,
1.),(1.,0.512254349645873,1.),(1.,0.528870329213323,1.),(1.,0.539918495566728,
1.),(1.,0.553602176080216,1.),(1.,0.556334955909364,1.),(1.,0.561765821980307,
1.),(1.,0.564466028627623,1.),(1.,0.572520418051971,1.),(1.,0.577828317778608,
1.),(1.,0.593564847150334,1.),(1.,0.603805896926842,1.),(1.,0.623792543125198,
1.),(1.,0.633538444526384,1.),(1.,0.652550041804049,1.),(1.,0.661815883466955,
1.),(1.,0.679885915223711,1.),(1.,0.6886901762844,1.),(1.,0.699418770951675,
1.),(1.,0.701551513084995,1.),(1.,0.705785767125964,1.),(1.,0.707884945612412,
1.),(1.,0.714129661070711,1.),(1.,0.718222393457039,1.),(1.,0.730296979845767,
1.),(1.,0.738075438054285,1.),(1.,0.753124875298064,1.),(1.,0.760395819580576,
1.),(1.,0.774458730322372,1.),(1.,0.781250671280861,1.),(1.,0.794378512232147,
1.),(1.,0.800714394746321,1.),(1.,0.809889696081597,1.),(1.,0.81289333920085,
1.),(1.,0.817317988310256,1.),(1.,0.81877983910783,1.),(1.,0.821667696260936,
1.),(1.,0.823094832962587,1.),(1.,0.830147792104091,1.),(1.,0.835525690411864,
1.),(1.,0.845780003457637,1.),(1.,0.85065638391852,1.),(1.,0.859929290650844,
1.),(1.,0.864325793621342,1.),(1.,0.870573221979968,1.),(1.,0.872597774409058,
1.),(1.,0.875548982801159,1.),(1.,0.876518446809548,1.),(1.,0.877951374397237,
1.),(1.,0.878425435719338,1.),(1.,0.879364277600825,1.),(1.,0.87982934145049,
1.),(1.,0.883976089465827,1.),(1.,0.887386226523438,1.),(1.,0.893695391832222,
1.),(1.,0.896594377182112,1.),(1.,0.901916757914401,1.),(1.,0.904340130964184,
1.),(1.,0.906816643976781,1.),(1.,0.907088077234898,1.),(1.,0.907622483818774,
1.),(1.,0.907885627787149,1.),(1.,0.908663109051759,1.),(1.,0.909165497176662,
1.),(1.,0.910626625009093,1.),(1.,0.911539350769517,1.),(1.,0.91410668701056,
1.),(1.,0.915590785243887,1.),(1.,0.917522428376818,1.),(1.,0.918117142015421,
1.),(1.,0.918940550747601,1.),(1.,0.919203618073144,1.),(1.,0.919707451070459,
1.),(1.,0.919946845560599,1.),(1.,0.921084971631206,1.),(1.,0.921808216030194,
1.),(1.,0.922671204445732,1.),(1.,0.922921678056867,1.),(1.,0.923355716047376,
1.),(1.,0.923539280063381,1.),(1.,0.923768924823362,1.),(1.,0.923837844568734,
1.),(1.,0.923930235120147,1.),(1.,0.923959199701402,1.),(1.,0.924013530789645,
1.),(1.,0.924038911854136,1.),(1.,0.924156810216913,1.),(1.,0.924221785724258,
1.),(1.,0.924299796558392,1.),(1.,0.924312823752853,1.),(1.,0.924291460660933,
1.),(1.,0.924257066663858,1.),(1.,0.924143360666746,1.),(1.,0.924064049018983,
1.),(1.,0.923911786837651,1.),(1.,0.923855468182103,1.),(1.,0.923762549501941,
1.),(1.,0.923730168815134,1.),(1.,0.923679465051457,1.),(1.,0.923662208277328,
1.),(1.,0.923626979380171,1.),(1.,0.923609029138641,1.),(1.,0.923590675042016,
1.)))
REPRESENTATION_ITEM('')
SURFACE()
);
#170=(
BOUNDED_SURFACE()
B_SPLINE_SURFACE(3,2,((#55159,#55160,#55161),(#55162,#55163,#55164),(#55165,
#55166,#55167),(#55168,#55169,#55170),(#55171,#55172,#55173),(#55174,#55175,
#55176),(#55177,#55178,#55179),(#55180,#55181,#55182),(#55183,#55184,#55185),
(#55186,#55187,#55188),(#55189,#55190,#55191),(#55192,#55193,#55194),(#55195,
#55196,#55197),(#55198,#55199,#55200),(#55201,#55202,#55203),(#55204,#55205,
#55206),(#55207,#55208,#55209),(#55210,#55211,#55212),(#55213,#55214,#55215),
(#55216,#55217,#55218),(#55219,#55220,#55221),(#55222,#55223,#55224),(#55225,
#55226,#55227),(#55228,#55229,#55230),(#55231,#55232,#55233),(#55234,#55235,
#55236),(#55237,#55238,#55239),(#55240,#55241,#55242)),.UNSPECIFIED.,.F.,
 .F.,.F.)
B_SPLINE_SURFACE_WITH_KNOTS((4,2,2,2,2,2,2,2,2,2,2,2,2,4),(3,3),(0.00343304549842295,
0.00356923072896442,0.00370541595950589,0.00373946226714126,0.00377350857477663,
0.00384160119004736,0.00397778642058883,0.00404587903585957,0.00407992534349494,
0.00411397165113031,0.00425015688167178,0.00438634211221325,0.00445443472748398,
0.00452252734275472),(0.,1.),.UNSPECIFIED.)
GEOMETRIC_REPRESENTATION_ITEM()
RATIONAL_B_SPLINE_SURFACE(((1.,0.625459232033944,1.),(1.,0.624403554488493,
1.),(1.,0.624295083285682,1.),(1.,0.625831833978692,1.),(1.,0.627477973201858,
1.),(1.,0.630511098040852,1.),(1.,0.631166352850721,1.),(1.,0.632570492553873,
1.),(1.,0.633320984647136,1.),(1.,0.635690804695334,1.),(1.,0.637429575912633,
1.),(1.,0.643040864092948,1.),(1.,0.647308049492937,1.),(1.,0.654182879861181,
1.),(1.,0.656553630245541,1.),(1.,0.660189296321541,1.),(1.,0.661414443264157,
1.),(1.,0.663884637649682,1.),(1.,0.665127312746621,1.),(1.,0.671327551077645,
1.),(1.,0.676275464921448,1.),(1.,0.68573549857353,1.),(1.,0.69024936841657,
1.),(1.,0.696399354422299,1.),(1.,0.698350363530641,1.),(1.,0.70194011110859,
1.),(1.,0.703586217954793,1.),(1.,0.705067492006796,1.)))
REPRESENTATION_ITEM('')
SURFACE()
);
#171=(
BOUNDED_SURFACE()
B_SPLINE_SURFACE(3,2,((#55329,#55330,#55331),(#55332,#55333,#55334),(#55335,
#55336,#55337),(#55338,#55339,#55340)),.UNSPECIFIED.,.F.,.F.,.F.)
B_SPLINE_SURFACE_WITH_KNOTS((4,4),(3,3),(0.0261617207655415,0.0383020860576645),
(-4.27038486529046E-6,1.),.UNSPECIFIED.)
GEOMETRIC_REPRESENTATION_ITEM()
RATIONAL_B_SPLINE_SURFACE(((1.00000160860429,0.811655818092484,1.),(1.0000016253793,
0.809691707667514,1.),(1.00000164120802,0.80783839465713,1.),(1.00000165623531,
0.806078918112741,1.)))
REPRESENTATION_ITEM('')
SURFACE()
);
#172=(
BOUNDED_SURFACE()
B_SPLINE_SURFACE(3,2,((#55354,#55355,#55356),(#55357,#55358,#55359),(#55360,
#55361,#55362),(#55363,#55364,#55365),(#55366,#55367,#55368),(#55369,#55370,
#55371),(#55372,#55373,#55374),(#55375,#55376,#55377),(#55378,#55379,#55380),
(#55381,#55382,#55383),(#55384,#55385,#55386),(#55387,#55388,#55389),(#55390,
#55391,#55392),(#55393,#55394,#55395),(#55396,#55397,#55398),(#55399,#55400,
#55401),(#55402,#55403,#55404),(#55405,#55406,#55407),(#55408,#55409,#55410),
(#55411,#55412,#55413),(#55414,#55415,#55416),(#55417,#55418,#55419),(#55420,
#55421,#55422),(#55423,#55424,#55425),(#55426,#55427,#55428),(#55429,#55430,
#55431),(#55432,#55433,#55434),(#55435,#55436,#55437),(#55438,#55439,#55440),
(#55441,#55442,#55443),(#55444,#55445,#55446),(#55447,#55448,#55449),(#55450,
#55451,#55452),(#55453,#55454,#55455),(#55456,#55457,#55458),(#55459,#55460,
#55461),(#55462,#55463,#55464),(#55465,#55466,#55467),(#55468,#55469,#55470),
(#55471,#55472,#55473),(#55474,#55475,#55476),(#55477,#55478,#55479),(#55480,
#55481,#55482),(#55483,#55484,#55485),(#55486,#55487,#55488),(#55489,#55490,
#55491),(#55492,#55493,#55494),(#55495,#55496,#55497),(#55498,#55499,#55500),
(#55501,#55502,#55503),(#55504,#55505,#55506),(#55507,#55508,#55509),(#55510,
#55511,#55512),(#55513,#55514,#55515),(#55516,#55517,#55518),(#55519,#55520,
#55521),(#55522,#55523,#55524),(#55525,#55526,#55527),(#55528,#55529,#55530),
(#55531,#55532,#55533),(#55534,#55535,#55536),(#55537,#55538,#55539),(#55540,
#55541,#55542),(#55543,#55544,#55545),(#55546,#55547,#55548),(#55549,#55550,
#55551),(#55552,#55553,#55554),(#55555,#55556,#55557),(#55558,#55559,#55560),
(#55561,#55562,#55563),(#55564,#55565,#55566),(#55567,#55568,#55569),(#55570,
#55571,#55572),(#55573,#55574,#55575),(#55576,#55577,#55578),(#55579,#55580,
#55581),(#55582,#55583,#55584),(#55585,#55586,#55587),(#55588,#55589,#55590),
(#55591,#55592,#55593),(#55594,#55595,#55596),(#55597,#55598,#55599),(#55600,
#55601,#55602),(#55603,#55604,#55605),(#55606,#55607,#55608),(#55609,#55610,
#55611),(#55612,#55613,#55614),(#55615,#55616,#55617)),.UNSPECIFIED.,.F.,
 .F.,.F.)
B_SPLINE_SURFACE_WITH_KNOTS((4,2,2,2,2,2,2,2,2,2,2,2,2,2,2,2,2,2,2,2,2,
2,2,2,2,2,2,2,2,2,2,2,2,2,2,2,2,2,2,2,2,2,2,4),(3,3),(0.00330261648339416,
0.00340081661298013,0.0034990167425661,0.00359721687215207,0.00364631693694505,
0.00369541700173804,0.003793617131324,0.00389181726090997,0.00394091732570296,
0.00396546735809945,0.00399001739049594,0.00408821752008191,0.00418641764966788,
0.00428461777925385,0.00438281790883982,0.00448101803842579,0.00457921816801176,
0.00462831823280474,0.00467741829759773,0.0047756184271837,0.00487381855676967,
0.00492291862156265,0.00494746865395914,0.00497201868635564,0.00507021881594161,
0.00516841894552758,0.00526661907511355,0.00531571913990653,0.00536481920469952,
0.00546301933428548,0.00556121946387145,0.00561031952866444,0.00565941959345742,
0.00575761972304339,0.00585581985262936,0.00590491991742235,0.00595401998221533,
0.0060522201118013,0.00615042024138727,0.00624862037097324,0.00627317040336973,
0.00629772043576622,0.00634682050055921,0.00644502063014518),(0.,1.),
 .UNSPECIFIED.)
GEOMETRIC_REPRESENTATION_ITEM()
RATIONAL_B_SPLINE_SURFACE(((1.,0.811656622391199,1.),(1.,0.811832571892841,
1.),(1.,0.811683313300623,1.),(1.,0.810765075561372,1.),(1.,0.809996124532223,
1.),(1.,0.807864448627461,1.),(1.,0.806501656926263,1.),(1.,0.804028901809539,
1.),(1.,0.803130322510617,1.),(1.,0.801211698750432,1.),(1.,0.800191446782092,
1.),(1.,0.796961352096929,1.),(1.,0.794582241729763,1.),(1.,0.789440647694272,
1.),(1.,0.786677989170548,1.),(1.,0.782296748929349,1.),(1.,0.780796800906642,
1.),(1.,0.77849415738182,1.),(1.,0.777717216045269,1.),(1.,0.776155137355144,
1.),(1.,0.77536909367214,1.),(1.,0.771417467466651,1.),(1.,0.768187639991458,
1.),(1.,0.761682357768366,1.),(1.,0.758406710407249,1.),(1.,0.751903933721366,
1.),(1.,0.748676603631679,1.),(1.,0.742373233767419,1.),(1.,0.739347411643543,
1.),(1.,0.733646267736223,1.),(1.,0.730969295702006,1.),(1.,0.726052823770446,
1.),(1.,0.723813234691965,1.),(1.,0.720852062565936,1.),(1.,0.719931403475167,
1.),(1.,0.718235111366214,1.),(1.,0.717466660341387,1.),(1.,0.715409033219939,
1.),(1.,0.714366635072083,1.),(1.,0.712967965168178,1.),(1.,0.712611690057782,
1.),(1.,0.712607635738503,1.),(1.,0.712694626675192,1.),(1.,0.71295915503469,
1.),(1.,0.713069668154168,1.),(1.,0.713335587614801,1.),(1.,0.713491283850726,
1.),(1.,0.714377922232085,1.),(1.,0.715432840757552,1.),(1.,0.718169210541053,
1.),(1.,0.719850696145383,1.),(1.,0.723773857278612,1.),(1.,0.726015568252412,
1.),(1.,0.72974661827765,1.),(1.,0.731052887236837,1.),(1.,0.733748031839737,
1.),(1.,0.735140203148474,1.),(1.,0.739430403187765,1.),(1.,0.742441933617721,
1.),(1.,0.748666868677604,1.),(1.,0.751880423473639,1.),(1.,0.756780279406297,
1.),(1.,0.758426889889258,1.),(1.,0.761734578028716,1.),(1.,0.763382933672718,
1.),(1.,0.768291653115061,1.),(1.,0.7715165857284,1.),(1.,0.777785013497246,
1.),(1.,0.780828707268701,1.),(1.,0.785196484807998,1.),(1.,0.786619464822865,
1.),(1.,0.78938908710468,1.),(1.,0.790737454081499,1.),(1.,0.794640861183113,
1.),(1.,0.797024425496887,1.),(1.,0.801307056342078,1.),(1.,0.803206253057746,
1.),(1.,0.806472900192383,1.),(1.,0.807840481551189,1.),(1.,0.809185497223154,
1.),(1.,0.809436262730181,1.),(1.,0.809900438192552,1.),(1.,0.810114130417425,
1.),(1.,0.810695487125602,1.),(1.,0.811003336720787,1.),(1.,0.811689316099667,
1.),(1.,0.811829944488298,1.),(1.,0.811656622391197,1.)))
REPRESENTATION_ITEM('')
SURFACE()
);
#173=(
BOUNDED_SURFACE()
B_SPLINE_SURFACE(3,2,((#55619,#55620,#55621),(#55622,#55623,#55624),(#55625,
#55626,#55627),(#55628,#55629,#55630)),.UNSPECIFIED.,.F.,.F.,.F.)
B_SPLINE_SURFACE_WITH_KNOTS((4,4),(3,3),(-7.97972798949331E-17,0.0113332794371223),
(0.,1.),.UNSPECIFIED.)
GEOMETRIC_REPRESENTATION_ITEM()
RATIONAL_B_SPLINE_SURFACE(((1.,0.806431892643699,1.),(1.,0.808086137640199,
1.),(1.,0.809823081379547,1.),(1.,0.811656622391199,1.)))
REPRESENTATION_ITEM('')
SURFACE()
);
#174=(
BOUNDED_SURFACE()
B_SPLINE_SURFACE(3,2,((#55637,#55638,#55639),(#55640,#55641,#55642),(#55643,
#55644,#55645),(#55646,#55647,#55648),(#55649,#55650,#55651),(#55652,#55653,
#55654),(#55655,#55656,#55657),(#55658,#55659,#55660),(#55661,#55662,#55663),
(#55664,#55665,#55666),(#55667,#55668,#55669),(#55670,#55671,#55672),(#55673,
#55674,#55675),(#55676,#55677,#55678),(#55679,#55680,#55681),(#55682,#55683,
#55684),(#55685,#55686,#55687),(#55688,#55689,#55690),(#55691,#55692,#55693),
(#55694,#55695,#55696),(#55697,#55698,#55699),(#55700,#55701,#55702),(#55703,
#55704,#55705),(#55706,#55707,#55708),(#55709,#55710,#55711),(#55712,#55713,
#55714),(#55715,#55716,#55717),(#55718,#55719,#55720),(#55721,#55722,#55723),
(#55724,#55725,#55726),(#55727,#55728,#55729),(#55730,#55731,#55732),(#55733,
#55734,#55735),(#55736,#55737,#55738),(#55739,#55740,#55741),(#55742,#55743,
#55744),(#55745,#55746,#55747),(#55748,#55749,#55750),(#55751,#55752,#55753),
(#55754,#55755,#55756),(#55757,#55758,#55759),(#55760,#55761,#55762),(#55763,
#55764,#55765),(#55766,#55767,#55768),(#55769,#55770,#55771),(#55772,#55773,
#55774)),.UNSPECIFIED.,.F.,.F.,.F.)
B_SPLINE_SURFACE_WITH_KNOTS((4,2,2,2,2,2,2,2,2,2,2,2,2,2,2,2,2,2,2,2,2,
2,4),(3,3),(-4.82469966756049E-18,5.50518151362045E-5,0.000110103630272414,
0.000165155445408623,0.000192681352976728,0.000220207260544833,0.000275259075681042,
0.000330310890817251,0.000357836798385356,0.000371599752169408,0.000385362705953461,
0.00044041452108967,0.000495466336225879,0.000522992243793984,0.000550518151362089,
0.000605569966498298,0.000660621781634507,0.000688147689202612,0.000701910642986664,
0.000715673596770717,0.000770725411906926,0.000825777227043135,0.000880829042179345),
(0.,1.),.UNSPECIFIED.)
GEOMETRIC_REPRESENTATION_ITEM()
RATIONAL_B_SPLINE_SURFACE(((1.,0.707106781185485,1.),(1.,0.710477894989039,
1.),(1.,0.713841886492236,1.),(1.,0.720556846901308,1.),(1.,0.723907847252579,
1.),(1.,0.730596240721846,1.),(1.,0.733933644391114,1.),(1.,0.738927431407798,
1.),(1.,0.740594246210395,1.),(1.,0.743888192923081,1.),(1.,0.745518215666872,
1.),(1.,0.750357382687748,1.),(1.,0.753515818763767,1.),(1.,0.75969242534585,
1.),(1.,0.76271062408444,1.),(1.,0.76712420463012,1.),(1.,0.76857639446933,
1.),(1.,0.770724569363179,1.),(1.,0.771434643119713,1.),(1.,0.772836027726094,
1.),(1.,0.773528322117743,1.),(1.,0.776947799211149,1.),(1.,0.779549385320001,
1.),(1.,0.784478174057131,1.),(1.,0.78680540757744,1.),(1.,0.790078083140807,
1.),(1.,0.791132534016176,1.),(1.,0.793165396446497,1.),(1.,0.794146568495307,
1.),(1.,0.796938387532037,1.),(1.,0.79860524372839,1.),(1.,0.801549647651601,
1.),(1.,0.802827202148284,1.),(1.,0.804441694539674,1.),(1.,0.80492945694585,
1.),(1.,0.805583313651139,1.),(1.,0.805788296097707,1.),(1.,0.806171865231364,
1.),(1.,0.806350694157879,1.),(1.,0.807172777122824,1.),(1.,0.807603802187835,
1.),(1.,0.808025829002193,1.),(1.,0.808016790860372,1.),(1.,0.807558204302794,
1.),(1.,0.807108474283634,1.),(1.,0.806431892643561,1.)))
REPRESENTATION_ITEM('')
SURFACE()
);
#175=(
BOUNDED_SURFACE()
B_SPLINE_SURFACE(3,2,((#55886,#55887,#55888),(#55889,#55890,#55891),(#55892,
#55893,#55894),(#55895,#55896,#55897),(#55898,#55899,#55900),(#55901,#55902,
#55903),(#55904,#55905,#55906),(#55907,#55908,#55909),(#55910,#55911,#55912),
(#55913,#55914,#55915),(#55916,#55917,#55918),(#55919,#55920,#55921),(#55922,
#55923,#55924),(#55925,#55926,#55927),(#55928,#55929,#55930),(#55931,#55932,
#55933),(#55934,#55935,#55936),(#55937,#55938,#55939),(#55940,#55941,#55942),
(#55943,#55944,#55945),(#55946,#55947,#55948),(#55949,#55950,#55951),(#55952,
#55953,#55954),(#55955,#55956,#55957),(#55958,#55959,#55960),(#55961,#55962,
#55963),(#55964,#55965,#55966),(#55967,#55968,#55969),(#55970,#55971,#55972),
(#55973,#55974,#55975),(#55976,#55977,#55978),(#55979,#55980,#55981),(#55982,
#55983,#55984),(#55985,#55986,#55987),(#55988,#55989,#55990),(#55991,#55992,
#55993),(#55994,#55995,#55996),(#55997,#55998,#55999),(#56000,#56001,#56002),
(#56003,#56004,#56005),(#56006,#56007,#56008),(#56009,#56010,#56011),(#56012,
#56013,#56014),(#56015,#56016,#56017),(#56018,#56019,#56020),(#56021,#56022,
#56023),(#56024,#56025,#56026),(#56027,#56028,#56029),(#56030,#56031,#56032),
(#56033,#56034,#56035),(#56036,#56037,#56038),(#56039,#56040,#56041),(#56042,
#56043,#56044),(#56045,#56046,#56047),(#56048,#56049,#56050),(#56051,#56052,
#56053)),.UNSPECIFIED.,.F.,.F.,.F.)
B_SPLINE_SURFACE_WITH_KNOTS((4,2,2,2,2,2,2,2,2,2,2,2,2,2,2,2,2,2,2,2,2,
2,2,2,2,2,2,4),(3,3),(0.0032383527045278,0.00336554775906757,0.00349274281360733,
0.00355634034087722,0.00358813910451216,0.0036199378681471,0.00374713292268687,
0.00387432797722664,0.00390612674086158,0.00393792550449652,0.0040015230317664,
0.00412871808630617,0.00419231561357605,0.00422411437721099,0.00425591314084594,
0.0043831081953857,0.00451030324992547,0.00457390077719535,0.0046056995408303,
0.00463749830446524,0.004764693359005,0.00489188841354477,0.00492368717717971,
0.00495548594081465,0.00501908346808454,0.0051462785226243,0.00520987604989419,
0.00527347357716407),(0.,1.),.UNSPECIFIED.)
GEOMETRIC_REPRESENTATION_ITEM()
RATIONAL_B_SPLINE_SURFACE(((1.,0.70710678118655,1.),(1.,0.706213957993281,
1.),(1.,0.705443938786405,1.),(1.,0.704136988709561,1.),(1.,0.703600079667857,
1.),(1.,0.702960418588502,1.),(1.,0.70277481545753,1.),(1.,0.702536660935443,
1.),(1.,0.702463890650407,1.),(1.,0.702332362486225,1.),(1.,0.702273501931224,
1.),(1.,0.70201213439835,1.),(1.,0.701908295200086,1.),(1.,0.701873429093663,
1.),(1.,0.701942493739908,1.),(1.,0.702114701888608,1.),(1.,0.70215343927011,
1.),(1.,0.702238949474263,1.),(1.,0.702285595803191,1.),(1.,0.702435575186992,
1.),(1.,0.702549116540971,1.),(1.,0.702921418342714,1.),(1.,0.703211731033178,
1.),(1.,0.703677757909964,1.),(1.,0.703838232332125,1.),(1.,0.704082806712229,
1.),(1.,0.704164976900933,1.),(1.,0.704329977699004,1.),(1.,0.704412960144125,
1.),(1.,0.704825691362464,1.),(1.,0.705148590086159,1.),(1.,0.705745128898862,
1.),(1.,0.706018867880871,1.),(1.,0.706371078301196,1.),(1.,0.706478786100633,
1.),(1.,0.706623371663295,1.),(1.,0.706668657551497,1.),(1.,0.706752667613401,
1.),(1.,0.706791471875649,1.),(1.,0.706969088136416,1.),(1.,0.7070584672857,
1.),(1.,0.707125223844347,1.),(1.,0.707102609206611,1.),(1.,0.70700357459,
1.),(1.,0.706980197085667,1.),(1.,0.706926650254296,1.),(1.,0.706896532893769,
1.),(1.,0.706796567062846,1.),(1.,0.70671709597817,1.),(1.,0.706443815084179,
1.),(1.,0.706214968750598,1.),(1.,0.705818771778775,1.),(1.,0.705677922813091,
1.),(1.,0.70538206823473,1.),(1.,0.705226726837797,1.),(1.,0.705067492006796,
1.)))
REPRESENTATION_ITEM('')
SURFACE()
);
#176=(
BOUNDED_SURFACE()
B_SPLINE_SURFACE(3,2,((#56268,#56269,#56270),(#56271,#56272,#56273),(#56274,
#56275,#56276),(#56277,#56278,#56279),(#56280,#56281,#56282),(#56283,#56284,
#56285),(#56286,#56287,#56288),(#56289,#56290,#56291),(#56292,#56293,#56294),
(#56295,#56296,#56297),(#56298,#56299,#56300),(#56301,#56302,#56303),(#56304,
#56305,#56306),(#56307,#56308,#56309),(#56310,#56311,#56312),(#56313,#56314,
#56315),(#56316,#56317,#56318),(#56319,#56320,#56321),(#56322,#56323,#56324),
(#56325,#56326,#56327),(#56328,#56329,#56330),(#56331,#56332,#56333),(#56334,
#56335,#56336),(#56337,#56338,#56339),(#56340,#56341,#56342),(#56343,#56344,
#56345),(#56346,#56347,#56348),(#56349,#56350,#56351)),.UNSPECIFIED.,.F.,
 .F.,.F.)
B_SPLINE_SURFACE_WITH_KNOTS((4,2,2,2,2,2,2,2,2,2,2,2,2,4),(3,3),(0.0012120764411892,
0.0013497499377862,0.00148742343438319,0.00162509693098018,0.00176277042757717,
0.00203811742077116,0.00231346441396515,0.00258881140715913,0.00286415840035312,
0.0031395053935471,0.0032771788901441,0.00334601563844259,0.00338043401259184,
0.00341485238674109),(0.,1.),.UNSPECIFIED.)
GEOMETRIC_REPRESENTATION_ITEM()
RATIONAL_B_SPLINE_SURFACE(((1.,0.707106781186468,1.),(1.,0.72002470605839,
1.),(1.,0.732433086825891,1.),(1.,0.756294061054311,1.),(1.,0.767746781874307,
1.),(1.,0.789743409782971,1.),(1.,0.800289212024087,1.),(1.,0.820486268600631,
1.),(1.,0.830140018061829,1.),(1.,0.857814961348585,1.),(1.,0.874552353369404,
1.),(1.,0.904768093055729,1.),(1.,0.918244574153276,1.),(1.,0.942040431761282,
1.),(1.,0.952358767872154,1.),(1.,0.969924448818458,1.),(1.,0.977171377622921,
1.),(1.,0.988685707102147,1.),(1.,0.992953212410708,1.),(1.,0.997195607349612,
1.),(1.,0.998249987789548,1.),(1.,0.999301490798357,1.),(1.,0.999563645238205,
1.),(1.,0.999825517691477,1.),(1.,0.999890914840196,1.),(1.,0.999978110425983,
1.),(1.,0.999999927945283,1.),(1.,1.,1.)))
REPRESENTATION_ITEM('')
SURFACE()
);
#177=(
BOUNDED_SURFACE()
B_SPLINE_SURFACE(3,2,((#56602,#56603,#56604),(#56605,#56606,#56607),(#56608,
#56609,#56610),(#56611,#56612,#56613),(#56614,#56615,#56616),(#56617,#56618,
#56619),(#56620,#56621,#56622),(#56623,#56624,#56625),(#56626,#56627,#56628),
(#56629,#56630,#56631),(#56632,#56633,#56634),(#56635,#56636,#56637),(#56638,
#56639,#56640),(#56641,#56642,#56643),(#56644,#56645,#56646),(#56647,#56648,
#56649),(#56650,#56651,#56652),(#56653,#56654,#56655),(#56656,#56657,#56658),
(#56659,#56660,#56661),(#56662,#56663,#56664),(#56665,#56666,#56667),(#56668,
#56669,#56670),(#56671,#56672,#56673),(#56674,#56675,#56676),(#56677,#56678,
#56679),(#56680,#56681,#56682),(#56683,#56684,#56685)),.UNSPECIFIED.,.F.,
 .F.,.F.)
B_SPLINE_SURFACE_WITH_KNOTS((4,2,2,2,2,2,2,2,2,2,2,2,2,4),(3,3),(0.00121207644118946,
0.00134974993778644,0.00148742343438341,0.00162509693098039,0.00176277042757736,
0.00203811742077132,0.00231346441396527,0.00258881140715922,0.00286415840035317,
0.00313950539354712,0.0032771788901441,0.00334601563844259,0.00338043401259183,
0.00341485238674108),(0.,1.),.UNSPECIFIED.)
GEOMETRIC_REPRESENTATION_ITEM()
RATIONAL_B_SPLINE_SURFACE(((1.,0.707106781186544,1.),(1.,0.720024706058528,
1.),(1.,0.732433086825873,1.),(1.,0.756294061054466,1.),(1.,0.767746781874374,
1.),(1.,0.78974340978302,1.),(1.,0.800289212024211,1.),(1.,0.820486268600606,
1.),(1.,0.830140018061826,1.),(1.,0.857814961348716,1.),(1.,0.87455235336949,
1.),(1.,0.90476809305572,1.),(1.,0.918244574153158,1.),(1.,0.942040431761433,
1.),(1.,0.952358767872266,1.),(1.,0.969924448818365,1.),(1.,0.977171377622992,
1.),(1.,0.988685707102086,1.),(1.,0.99295321241071,1.),(1.,0.997195607349613,
1.),(1.,0.998249987789543,1.),(1.,0.99930149079836,1.),(1.,0.999563645238205,
1.),(1.,0.999825517691477,1.),(1.,0.999890914840191,1.),(1.,0.999978110425987,
1.),(1.,0.999999927945279,1.),(1.,1.,1.)))
REPRESENTATION_ITEM('')
SURFACE()
);
#178=(
BOUNDED_SURFACE()
B_SPLINE_SURFACE(3,2,((#56792,#56793,#56794),(#56795,#56796,#56797),(#56798,
#56799,#56800),(#56801,#56802,#56803),(#56804,#56805,#56806),(#56807,#56808,
#56809),(#56810,#56811,#56812),(#56813,#56814,#56815),(#56816,#56817,#56818),
(#56819,#56820,#56821),(#56822,#56823,#56824),(#56825,#56826,#56827),(#56828,
#56829,#56830),(#56831,#56832,#56833),(#56834,#56835,#56836),(#56837,#56838,
#56839),(#56840,#56841,#56842),(#56843,#56844,#56845),(#56846,#56847,#56848),
(#56849,#56850,#56851),(#56852,#56853,#56854),(#56855,#56856,#56857),(#56858,
#56859,#56860),(#56861,#56862,#56863),(#56864,#56865,#56866),(#56867,#56868,
#56869),(#56870,#56871,#56872),(#56873,#56874,#56875)),.UNSPECIFIED.,.F.,
 .F.,.F.)
B_SPLINE_SURFACE_WITH_KNOTS((4,2,2,2,2,2,2,2,2,2,2,2,2,4),(3,3),(-1.34164157599756E-5,
2.06868368462185E-5,5.47900894524126E-5,0.000122996594664801,0.000259409605089577,
0.00053223562593913,0.000805061646788683,0.00107788766763824,0.00135071368848779,
0.00162353970933734,0.00175995271976212,0.0018963657301869,0.00203277874061167,
0.00216919175103645),(0.,1.),.UNSPECIFIED.)
GEOMETRIC_REPRESENTATION_ITEM()
RATIONAL_B_SPLINE_SURFACE(((1.,1.,1.),(1.,1.00000001507238,1.),(1.,0.999978441292673,
1.),(1.,0.999891806781135,1.),(1.,0.9998267650581,1.),(1.,0.999566166629267,
1.),(1.,0.999305138400123,1.),(1.,0.99825771444247,1.),(1.,0.997206984918604,
1.),(1.,0.992977382403944,1.),(1.,0.988720812320532,1.),(1.,0.977229079290884,
1.),(1.,0.969993795445904,1.),(1.,0.952449695699923,1.),(1.,0.942140526220492,
1.),(1.,0.918365194495103,1.),(1.,0.90490049697849,1.),(1.,0.874707837529653,
1.),(1.,0.85798179866746,1.),(1.,0.830317205299946,1.),(1.,0.820664626400707,
1.),(1.,0.80047208844851,1.),(1.,0.789932732031198,1.),(1.,0.767926390428376,
1.),(1.,0.756459594779169,1.),(1.,0.732541332877355,1.),(1.,0.720089718170756,
1.),(1.,0.707106781186543,1.)))
REPRESENTATION_ITEM('')
SURFACE()
);
#179=(
BOUNDED_SURFACE()
B_SPLINE_SURFACE(3,2,((#56962,#56963,#56964),(#56965,#56966,#56967),(#56968,
#56969,#56970),(#56971,#56972,#56973),(#56974,#56975,#56976),(#56977,#56978,
#56979),(#56980,#56981,#56982),(#56983,#56984,#56985),(#56986,#56987,#56988),
(#56989,#56990,#56991),(#56992,#56993,#56994),(#56995,#56996,#56997),(#56998,
#56999,#57000),(#57001,#57002,#57003),(#57004,#57005,#57006),(#57007,#57008,
#57009),(#57010,#57011,#57012),(#57013,#57014,#57015),(#57016,#57017,#57018),
(#57019,#57020,#57021),(#57022,#57023,#57024),(#57025,#57026,#57027),(#57028,
#57029,#57030),(#57031,#57032,#57033),(#57034,#57035,#57036),(#57037,#57038,
#57039),(#57040,#57041,#57042),(#57043,#57044,#57045)),.UNSPECIFIED.,.F.,
 .F.,.F.)
B_SPLINE_SURFACE_WITH_KNOTS((4,2,2,2,2,2,2,2,2,2,2,2,2,4),(3,3),(-1.34164157599273E-5,
2.06868368462668E-5,5.47900894524609E-5,0.000122996594664849,0.000259409605089626,
0.000532235625939179,0.000805061646788732,0.00107788766763828,0.00135071368848784,
0.00162353970933739,0.00175995271976217,0.00189636573018694,0.00203277874061172,
0.0021691917510365),(0.,1.),.UNSPECIFIED.)
GEOMETRIC_REPRESENTATION_ITEM()
RATIONAL_B_SPLINE_SURFACE(((1.,1.,1.),(1.,1.00000001507238,1.),(1.,0.999978441292673,
1.),(1.,0.999891806781135,1.),(1.,0.9998267650581,1.),(1.,0.999566166629267,
1.),(1.,0.999305138400118,1.),(1.,0.998257714442481,1.),(1.,0.997206984918586,
1.),(1.,0.992977382403979,1.),(1.,0.988720812320531,1.),(1.,0.977229079290883,
1.),(1.,0.969993795445918,1.),(1.,0.952449695699907,1.),(1.,0.942140526220349,
1.),(1.,0.918365194495244,1.),(1.,0.904900496979517,1.),(1.,0.874707837530609,
1.),(1.,0.857981798667344,1.),(1.,0.830317205300004,1.),(1.,0.82066462640065,
1.),(1.,0.800472088448564,1.),(1.,0.789932732031166,1.),(1.,0.767926390428401,
1.),(1.,0.756459594779094,1.),(1.,0.732541332877426,1.),(1.,0.720089718170704,
1.),(1.,0.707106781186544,1.)))
REPRESENTATION_ITEM('')
SURFACE()
);
#180=(
BOUNDED_SURFACE()
B_SPLINE_SURFACE(3,2,((#57341,#57342,#57343),(#57344,#57345,#57346),(#57347,
#57348,#57349),(#57350,#57351,#57352),(#57353,#57354,#57355),(#57356,#57357,
#57358),(#57359,#57360,#57361),(#57362,#57363,#57364),(#57365,#57366,#57367),
(#57368,#57369,#57370),(#57371,#57372,#57373),(#57374,#57375,#57376),(#57377,
#57378,#57379),(#57380,#57381,#57382),(#57383,#57384,#57385),(#57386,#57387,
#57388),(#57389,#57390,#57391),(#57392,#57393,#57394),(#57395,#57396,#57397),
(#57398,#57399,#57400),(#57401,#57402,#57403),(#57404,#57405,#57406),(#57407,
#57408,#57409),(#57410,#57411,#57412),(#57413,#57414,#57415),(#57416,#57417,
#57418),(#57419,#57420,#57421),(#57422,#57423,#57424),(#57425,#57426,#57427),
(#57428,#57429,#57430),(#57431,#57432,#57433),(#57434,#57435,#57436),(#57437,
#57438,#57439),(#57440,#57441,#57442),(#57443,#57444,#57445),(#57446,#57447,
#57448),(#57449,#57450,#57451),(#57452,#57453,#57454),(#57455,#57456,#57457),
(#57458,#57459,#57460),(#57461,#57462,#57463),(#57464,#57465,#57466),(#57467,
#57468,#57469),(#57470,#57471,#57472),(#57473,#57474,#57475),(#57476,#57477,
#57478),(#57479,#57480,#57481),(#57482,#57483,#57484),(#57485,#57486,#57487),
(#57488,#57489,#57490),(#57491,#57492,#57493),(#57494,#57495,#57496),(#57497,
#57498,#57499),(#57500,#57501,#57502),(#57503,#57504,#57505),(#57506,#57507,
#57508),(#57509,#57510,#57511),(#57512,#57513,#57514),(#57515,#57516,#57517),
(#57518,#57519,#57520),(#57521,#57522,#57523),(#57524,#57525,#57526),(#57527,
#57528,#57529),(#57530,#57531,#57532),(#57533,#57534,#57535),(#57536,#57537,
#57538),(#57539,#57540,#57541),(#57542,#57543,#57544),(#57545,#57546,#57547),
(#57548,#57549,#57550),(#57551,#57552,#57553),(#57554,#57555,#57556),(#57557,
#57558,#57559),(#57560,#57561,#57562),(#57563,#57564,#57565),(#57566,#57567,
#57568),(#57569,#57570,#57571),(#57572,#57573,#57574),(#57575,#57576,#57577),
(#57578,#57579,#57580),(#57581,#57582,#57583),(#57584,#57585,#57586),(#57587,
#57588,#57589),(#57590,#57591,#57592),(#57593,#57594,#57595),(#57596,#57597,
#57598),(#57599,#57600,#57601),(#57602,#57603,#57604),(#57605,#57606,#57607),
(#57608,#57609,#57610),(#57611,#57612,#57613),(#57614,#57615,#57616),(#57617,
#57618,#57619),(#57620,#57621,#57622),(#57623,#57624,#57625),(#57626,#57627,
#57628),(#57629,#57630,#57631),(#57632,#57633,#57634),(#57635,#57636,#57637),
(#57638,#57639,#57640),(#57641,#57642,#57643),(#57644,#57645,#57646),(#57647,
#57648,#57649),(#57650,#57651,#57652),(#57653,#57654,#57655),(#57656,#57657,
#57658),(#57659,#57660,#57661),(#57662,#57663,#57664),(#57665,#57666,#57667),
(#57668,#57669,#57670),(#57671,#57672,#57673),(#57674,#57675,#57676),(#57677,
#57678,#57679),(#57680,#57681,#57682),(#57683,#57684,#57685),(#57686,#57687,
#57688),(#57689,#57690,#57691),(#57692,#57693,#57694),(#57695,#57696,#57697),
(#57698,#57699,#57700),(#57701,#57702,#57703),(#57704,#57705,#57706),(#57707,
#57708,#57709),(#57710,#57711,#57712),(#57713,#57714,#57715),(#57716,#57717,
#57718),(#57719,#57720,#57721),(#57722,#57723,#57724),(#57725,#57726,#57727),
(#57728,#57729,#57730),(#57731,#57732,#57733),(#57734,#57735,#57736),(#57737,
#57738,#57739),(#57740,#57741,#57742),(#57743,#57744,#57745),(#57746,#57747,
#57748),(#57749,#57750,#57751),(#57752,#57753,#57754),(#57755,#57756,#57757),
(#57758,#57759,#57760),(#57761,#57762,#57763),(#57764,#57765,#57766),(#57767,
#57768,#57769),(#57770,#57771,#57772),(#57773,#57774,#57775),(#57776,#57777,
#57778),(#57779,#57780,#57781),(#57782,#57783,#57784),(#57785,#57786,#57787),
(#57788,#57789,#57790),(#57791,#57792,#57793),(#57794,#57795,#57796),(#57797,
#57798,#57799),(#57800,#57801,#57802),(#57803,#57804,#57805),(#57806,#57807,
#57808),(#57809,#57810,#57811),(#57812,#57813,#57814),(#57815,#57816,#57817),
(#57818,#57819,#57820),(#57821,#57822,#57823),(#57824,#57825,#57826),(#57827,
#57828,#57829),(#57830,#57831,#57832),(#57833,#57834,#57835),(#57836,#57837,
#57838),(#57839,#57840,#57841),(#57842,#57843,#57844),(#57845,#57846,#57847),
(#57848,#57849,#57850),(#57851,#57852,#57853),(#57854,#57855,#57856),(#57857,
#57858,#57859),(#57860,#57861,#57862),(#57863,#57864,#57865),(#57866,#57867,
#57868),(#57869,#57870,#57871),(#57872,#57873,#57874),(#57875,#57876,#57877),
(#57878,#57879,#57880),(#57881,#57882,#57883),(#57884,#57885,#57886),(#57887,
#57888,#57889),(#57890,#57891,#57892),(#57893,#57894,#57895),(#57896,#57897,
#57898),(#57899,#57900,#57901),(#57902,#57903,#57904),(#57905,#57906,#57907),
(#57908,#57909,#57910),(#57911,#57912,#57913),(#57914,#57915,#57916),(#57917,
#57918,#57919),(#57920,#57921,#57922),(#57923,#57924,#57925),(#57926,#57927,
#57928),(#57929,#57930,#57931),(#57932,#57933,#57934),(#57935,#57936,#57937),
(#57938,#57939,#57940),(#57941,#57942,#57943),(#57944,#57945,#57946),(#57947,
#57948,#57949),(#57950,#57951,#57952),(#57953,#57954,#57955),(#57956,#57957,
#57958),(#57959,#57960,#57961),(#57962,#57963,#57964),(#57965,#57966,#57967),
(#57968,#57969,#57970),(#57971,#57972,#57973),(#57974,#57975,#57976),(#57977,
#57978,#57979),(#57980,#57981,#57982),(#57983,#57984,#57985),(#57986,#57987,
#57988),(#57989,#57990,#57991),(#57992,#57993,#57994),(#57995,#57996,#57997),
(#57998,#57999,#58000),(#58001,#58002,#58003),(#58004,#58005,#58006),(#58007,
#58008,#58009),(#58010,#58011,#58012),(#58013,#58014,#58015),(#58016,#58017,
#58018),(#58019,#58020,#58021),(#58022,#58023,#58024),(#58025,#58026,#58027),
(#58028,#58029,#58030),(#58031,#58032,#58033),(#58034,#58035,#58036),(#58037,
#58038,#58039),(#58040,#58041,#58042),(#58043,#58044,#58045),(#58046,#58047,
#58048),(#58049,#58050,#58051),(#58052,#58053,#58054),(#58055,#58056,#58057),
(#58058,#58059,#58060),(#58061,#58062,#58063),(#58064,#58065,#58066),(#58067,
#58068,#58069),(#58070,#58071,#58072),(#58073,#58074,#58075),(#58076,#58077,
#58078),(#58079,#58080,#58081),(#58082,#58083,#58084),(#58085,#58086,#58087),
(#58088,#58089,#58090),(#58091,#58092,#58093),(#58094,#58095,#58096),(#58097,
#58098,#58099),(#58100,#58101,#58102),(#58103,#58104,#58105),(#58106,#58107,
#58108),(#58109,#58110,#58111),(#58112,#58113,#58114),(#58115,#58116,#58117),
(#58118,#58119,#58120),(#58121,#58122,#58123),(#58124,#58125,#58126),(#58127,
#58128,#58129),(#58130,#58131,#58132),(#58133,#58134,#58135),(#58136,#58137,
#58138)),.UNSPECIFIED.,.T.,.F.,.F.)
B_SPLINE_SURFACE_WITH_KNOTS((4,2,2,2,2,2,2,2,2,2,2,2,2,2,2,2,2,2,2,2,2,
2,2,2,2,2,2,2,2,2,2,2,2,2,2,2,2,2,2,2,2,2,2,2,2,2,2,2,2,2,2,2,2,2,2,2,2,
2,2,2,2,2,2,2,2,2,2,2,2,2,2,2,2,2,2,2,2,2,2,2,2,2,2,2,2,2,2,2,2,2,2,2,2,
2,2,2,2,2,2,2,2,2,2,2,2,2,2,2,2,2,2,2,2,2,2,2,2,2,2,2,2,2,2,2,2,2,2,2,2,
2,2,2,4),(3,3),(0.,4.12881615541384E-5,8.25763231082768E-5,0.000165152646216554,
0.000330305292433107,0.000660610584866214,0.000990915877299321,0.00132122116973243,
0.00148637381594898,0.00156895013905726,0.00165152646216554,0.00198183175459864,
0.00264244233946486,0.00297274763189796,0.00313790027811452,0.00322047660122279,
0.00330305292433107,0.00396366350919728,0.0046242740940635,0.00495457938649661,
0.00503715570960488,0.00511973203271316,0.00528488467892971,0.00594549526379593,
0.00660610584866214,0.00693641114109525,0.00701898746420353,0.0071015637873118,
0.00726671643352836,0.00792732701839457,0.00858793760326078,0.009248548188127,
0.00990915877299321,0.0100743114192098,0.0102394640654263,0.0105697693578594,
0.0112303799427256,0.0118909905275919,0.0125516011124581,0.0132122116973243,
0.0138728222821905,0.0139553986052988,0.0140379749284071,0.0142031275746236,
0.0145334328670567,0.0151940434519229,0.0158546540367891,0.0165152646216554,
0.0166804172678719,0.0168455699140885,0.0171758752065216,0.0175061804989547,
0.0178364857913878,0.0181667910838209,0.0183319437300374,0.0184145200531457,
0.018497096376254,0.0188274016686871,0.0191577069611202,0.0194880122535533,
0.0196531648997699,0.0197357412228781,0.0198183175459864,0.0201486228384195,
0.0204789281308526,0.0208092334232857,0.020891809746394,0.0209743860695023,
0.0211395387157189,0.021469844008152,0.0215524203312602,0.0216349966543685,
0.0218001493005851,0.0221304545930182,0.0224607598854513,0.0227910651778844,
0.0231213704703175,0.0232039467934258,0.023286523116534,0.0234516757627506,
0.0237819810551837,0.0241122863476168,0.0244425916400499,0.0251032022249161,
0.0252683548711327,0.0254335075173492,0.0257638128097823,0.0264244233946486,
0.0270850339795148,0.027745644564381,0.0284062551492472,0.0285714077954638,
0.0287365604416803,0.0290668657341134,0.0297274763189796,0.0303880869038458,
0.0310486974887121,0.0317093080735783,0.0320396133660114,0.0322047660122279,
0.0323699186584445,0.0330305292433107,0.0336911398281769,0.0343517504130431,
0.0346820557054762,0.0348472083516928,0.0349297846748011,0.0350123609979093,
0.0356729715827756,0.0363335821676418,0.036994192752508,0.0370767690756163,
0.0371593453987245,0.0373244980449411,0.0376548033373742,0.0383154139222404,
0.0386457192146735,0.0388108718608901,0.0389760245071066,0.0396366350919728,
0.039966940384406,0.0402972456768391,0.0404623983230556,0.0405449746461639,
0.0406275509692722,0.0409578562617053,0.0412881615541384,0.0416184668465715,
0.0419487721390046,0.0421139247852211,0.0421965011083294,0.0422377892698836,
0.0422790774314377),(0.,1.),.UNSPECIFIED.)
GEOMETRIC_REPRESENTATION_ITEM()
RATIONAL_B_SPLINE_SURFACE(((1.,0.923590675042016,1.),(1.,0.923572320945391,
1.),(1.,0.923553587090577,1.),(1.,0.923515495478205,1.),(1.,0.923496115237016,
1.),(1.,0.923436971524286,1.),(1.,0.923396205307423,1.),(1.,0.923269889059141,
1.),(1.,0.923180325181551,1.),(1.,0.922895385428438,1.),(1.,0.922683818431749,
1.),(1.,0.922215055006499,1.),(1.,0.921957857869856,1.),(1.,0.921393597668949,
1.),(1.,0.921086537396165,1.),(1.,0.920583987620736,1.),(1.,0.920409463147971,
1.),(1.,0.920136456599823,1.),(1.,0.920043583473226,1.),(1.,0.919853965179493,
1.),(1.,0.919757130552995,1.),(1.,0.919264385051497,1.),(1.,0.918842556687909,
1.),(1.,0.917485342839882,1.),(1.,0.916458802712932,1.),(1.,0.914690614339645,
1.),(1.,0.914063012700798,1.),(1.,0.913057237216573,1.),(1.,0.912711240257362,
1.),(1.,0.912175163335873,1.),(1.,0.911993623483323,1.),(1.,0.911624678363091,
1.),(1.,0.911437120441042,1.),(1.,0.909726149783902,1.),(1.,0.908041888239718,
1.),(1.,0.904290424256204,1.),(1.,0.90222325436422,1.),(1.,0.898787650803265,
1.),(1.,0.897586580689637,1.),(1.,0.896009931734525,1.),(1.,0.895690686714278,
1.),(1.,0.895045201490737,1.),(1.,0.894719248531258,1.),(1.,0.893731649644609,
1.),(1.,0.893060263975502,1.),(1.,0.889636937842127,1.),(1.,0.886685904879282,
1.),(1.,0.880320125821774,1.),(1.,0.876905428959452,1.),(1.,0.871403913130991,
1.),(1.,0.869506798646649,1.),(1.,0.867052723787093,1.),(1.,0.866557553196408,
1.),(1.,0.865560870035344,1.),(1.,0.865059173595903,1.),(1.,0.863543964995002,
1.),(1.,0.862520333878055,1.),(1.,0.857333970909859,1.),(1.,0.852966736393177,
1.),(1.,0.843775067927313,1.),(1.,0.838950667880686,1.),(1.,0.828820205567495,
1.),(1.,0.823514183332928,1.),(1.,0.812391307349727,1.),(1.,0.806574504385483,
1.),(1.,0.798962220591142,1.),(1.,0.797421706068384,1.),(1.,0.794315888151595,
1.),(1.,0.792749600433445,1.),(1.,0.788010186024153,1.),(1.,0.784796515809518,
1.),(1.,0.77498973461648,1.),(1.,0.768230990620621,1.),(1.,0.754249477539376,
1.),(1.,0.7470267311596,1.),(1.,0.732090338555257,1.),(1.,0.724376719977163,
1.),(1.,0.708426290764442,1.),(1.,0.700189512530531,1.),(1.,0.683154153538125,
1.),(1.,0.674355607127678,1.),(1.,0.664115385685685,1.),(1.,0.66297302996927,
1.),(1.,0.660682162177284,1.),(1.,0.659533241882799,1.),(1.,0.65607598168352,
1.),(1.,0.653757142047767,1.),(1.,0.646758317475323,1.),(1.,0.642036016956393,
1.),(1.,0.627697700195677,1.),(1.,0.61790996153014,1.),(1.,0.597870566155991,
1.),(1.,0.58761854570598,1.),(1.,0.566657940545553,1.),(1.,0.555948596069607,
1.),(1.,0.542299741359184,1.),(1.,0.539556972501121,1.),(1.,0.53404656747395,
1.),(1.,0.531276245933983,1.),(1.,0.522962675372791,1.),(1.,0.517409973114278,
1.),(1.,0.506307878837006,1.),(1.,0.500758405674242,1.),(1.,0.489694670444622,
1.),(1.,0.484180295137749,1.),(1.,0.473229585826254,1.),(1.,0.467793092024575,
1.),(1.,0.459740217505025,1.),(1.,0.457073035061414,1.),(1.,0.453104759629238,
1.),(1.,0.451787428134069,1.),(1.,0.449164897866363,1.),(1.,0.447859036145478,
1.),(1.,0.441385443166445,1.),(1.,0.436368154024372,1.),(1.,0.426750681610345,
1.),(1.,0.422150388759125,1.),(1.,0.413481583263519,1.),(1.,0.409412966405537,
1.),(1.,0.403813005360145,1.),(1.,0.402030377100019,1.),(1.,0.399497383040528,
1.),(1.,0.398676556272897,1.),(1.,0.397084562446663,1.),(1.,0.396315545546773,
1.),(1.,0.392617462025358,1.),(1.,0.390121311666049,1.),(1.,0.386146893571918,
1.),(1.,0.384668848565874,1.),(1.,0.382812549250897,1.),(1.,0.382434470212711,
1.),(1.,0.38268919558194,1.),(1.,0.382776371338327,1.),(1.,0.383022089646797,
1.),(1.,0.383180660969252,1.),(1.,0.383762017423613,1.),(1.,0.384290482158863,
1.),(1.,0.386285206501931,1.),(1.,0.388161225874796,1.),(1.,0.391136736543832,
1.),(1.,0.391763914323658,1.),(1.,0.393077192923473,1.),(1.,0.393761818570545,
1.),(1.,0.395895524715283,1.),(1.,0.397424386821021,1.),(1.,0.402298884562898,
1.),(1.,0.405931683845182,1.),(1.,0.413815239487506,1.),(1.,0.418066059410145,
1.),(1.,0.42706069079461,1.),(1.,0.431804585246568,1.),(1.,0.441681473676376,
1.),(1.,0.446814558722576,1.),(1.,0.453420699181124,1.),(1.,0.454748719848507,
1.),(1.,0.457413317151073,1.),(1.,0.458750495400507,1.),(1.,0.462774945482169,
1.),(1.,0.465475093536882,1.),(1.,0.473614842385458,1.),(1.,0.479093267976819,
1.),(1.,0.490102288950609,1.),(1.,0.495633034030675,1.),(1.,0.506709011958283,
1.),(1.,0.512254349645873,1.),(1.,0.528870329213323,1.),(1.,0.539918495566728,
1.),(1.,0.553602176080216,1.),(1.,0.556334955909364,1.),(1.,0.561765821980307,
1.),(1.,0.564466028627623,1.),(1.,0.572520418051971,1.),(1.,0.577828317778608,
1.),(1.,0.593564847150334,1.),(1.,0.603805896926842,1.),(1.,0.623792543125198,
1.),(1.,0.633538444526384,1.),(1.,0.652550041804049,1.),(1.,0.661815883466955,
1.),(1.,0.679885915223711,1.),(1.,0.6886901762844,1.),(1.,0.699418770951675,
1.),(1.,0.701551513084995,1.),(1.,0.705785767125964,1.),(1.,0.707884945612412,
1.),(1.,0.714129661070711,1.),(1.,0.718222393457039,1.),(1.,0.730296979845767,
1.),(1.,0.738075438054285,1.),(1.,0.753124875298064,1.),(1.,0.760395819580576,
1.),(1.,0.774458730322372,1.),(1.,0.781250671280861,1.),(1.,0.794378512232147,
1.),(1.,0.800714394746321,1.),(1.,0.809889696081597,1.),(1.,0.81289333920085,
1.),(1.,0.817317988310256,1.),(1.,0.81877983910783,1.),(1.,0.821667696260936,
1.),(1.,0.823094832962587,1.),(1.,0.830147792104091,1.),(1.,0.835525690411864,
1.),(1.,0.845780003457637,1.),(1.,0.85065638391852,1.),(1.,0.859929290650844,
1.),(1.,0.864325793621342,1.),(1.,0.870573221979968,1.),(1.,0.872597774409058,
1.),(1.,0.875548982801159,1.),(1.,0.876518446809548,1.),(1.,0.877951374397237,
1.),(1.,0.878425435719338,1.),(1.,0.879364277600825,1.),(1.,0.87982934145049,
1.),(1.,0.883976089465827,1.),(1.,0.887386226523438,1.),(1.,0.893695391832222,
1.),(1.,0.896594377182112,1.),(1.,0.901916757914401,1.),(1.,0.904340130964184,
1.),(1.,0.906816643976781,1.),(1.,0.907088077234898,1.),(1.,0.907622483818774,
1.),(1.,0.907885627787149,1.),(1.,0.908663109051759,1.),(1.,0.909165497176662,
1.),(1.,0.910626625009093,1.),(1.,0.911539350769517,1.),(1.,0.91410668701056,
1.),(1.,0.915590785243887,1.),(1.,0.917522428376818,1.),(1.,0.918117142015421,
1.),(1.,0.918940550747601,1.),(1.,0.919203618073144,1.),(1.,0.919707451070459,
1.),(1.,0.919946845560599,1.),(1.,0.921084971631206,1.),(1.,0.921808216030194,
1.),(1.,0.922671204445732,1.),(1.,0.922921678056867,1.),(1.,0.923355716047376,
1.),(1.,0.923539280063381,1.),(1.,0.923768924823362,1.),(1.,0.923837844568734,
1.),(1.,0.923930235120147,1.),(1.,0.923959199701402,1.),(1.,0.924013530789645,
1.),(1.,0.924038911854136,1.),(1.,0.924156810216913,1.),(1.,0.924221785724258,
1.),(1.,0.924299796558392,1.),(1.,0.924312823752853,1.),(1.,0.924291460660933,
1.),(1.,0.924257066663858,1.),(1.,0.924143360666746,1.),(1.,0.924064049018983,
1.),(1.,0.923911786837651,1.),(1.,0.923855468182103,1.),(1.,0.923762549501941,
1.),(1.,0.923730168815134,1.),(1.,0.923679465051457,1.),(1.,0.923662208277328,
1.),(1.,0.923626979380171,1.),(1.,0.923609029138641,1.),(1.,0.923590675042016,
1.)))
REPRESENTATION_ITEM('')
SURFACE()
);
#181=(
BOUNDED_SURFACE()
B_SPLINE_SURFACE(3,2,((#58139,#58140,#58141),(#58142,#58143,#58144),(#58145,
#58146,#58147),(#58148,#58149,#58150),(#58151,#58152,#58153),(#58154,#58155,
#58156),(#58157,#58158,#58159),(#58160,#58161,#58162),(#58163,#58164,#58165),
(#58166,#58167,#58168),(#58169,#58170,#58171),(#58172,#58173,#58174),(#58175,
#58176,#58177),(#58178,#58179,#58180),(#58181,#58182,#58183),(#58184,#58185,
#58186),(#58187,#58188,#58189),(#58190,#58191,#58192),(#58193,#58194,#58195),
(#58196,#58197,#58198),(#58199,#58200,#58201),(#58202,#58203,#58204),(#58205,
#58206,#58207),(#58208,#58209,#58210),(#58211,#58212,#58213),(#58214,#58215,
#58216),(#58217,#58218,#58219),(#58220,#58221,#58222),(#58223,#58224,#58225),
(#58226,#58227,#58228),(#58229,#58230,#58231),(#58232,#58233,#58234),(#58235,
#58236,#58237),(#58238,#58239,#58240),(#58241,#58242,#58243),(#58244,#58245,
#58246),(#58247,#58248,#58249),(#58250,#58251,#58252),(#58253,#58254,#58255),
(#58256,#58257,#58258),(#58259,#58260,#58261),(#58262,#58263,#58264),(#58265,
#58266,#58267),(#58268,#58269,#58270),(#58271,#58272,#58273),(#58274,#58275,
#58276),(#58277,#58278,#58279),(#58280,#58281,#58282),(#58283,#58284,#58285),
(#58286,#58287,#58288),(#58289,#58290,#58291),(#58292,#58293,#58294),(#58295,
#58296,#58297),(#58298,#58299,#58300),(#58301,#58302,#58303),(#58304,#58305,
#58306),(#58307,#58308,#58309),(#58310,#58311,#58312),(#58313,#58314,#58315),
(#58316,#58317,#58318),(#58319,#58320,#58321),(#58322,#58323,#58324),(#58325,
#58326,#58327),(#58328,#58329,#58330),(#58331,#58332,#58333),(#58334,#58335,
#58336),(#58337,#58338,#58339),(#58340,#58341,#58342),(#58343,#58344,#58345),
(#58346,#58347,#58348),(#58349,#58350,#58351),(#58352,#58353,#58354),(#58355,
#58356,#58357),(#58358,#58359,#58360),(#58361,#58362,#58363),(#58364,#58365,
#58366),(#58367,#58368,#58369),(#58370,#58371,#58372),(#58373,#58374,#58375),
(#58376,#58377,#58378),(#58379,#58380,#58381),(#58382,#58383,#58384),(#58385,
#58386,#58387),(#58388,#58389,#58390),(#58391,#58392,#58393),(#58394,#58395,
#58396),(#58397,#58398,#58399),(#58400,#58401,#58402),(#58403,#58404,#58405),
(#58406,#58407,#58408),(#58409,#58410,#58411),(#58412,#58413,#58414),(#58415,
#58416,#58417),(#58418,#58419,#58420),(#58421,#58422,#58423),(#58424,#58425,
#58426),(#58427,#58428,#58429),(#58430,#58431,#58432),(#58433,#58434,#58435),
(#58436,#58437,#58438),(#58439,#58440,#58441),(#58442,#58443,#58444),(#58445,
#58446,#58447),(#58448,#58449,#58450),(#58451,#58452,#58453),(#58454,#58455,
#58456),(#58457,#58458,#58459),(#58460,#58461,#58462),(#58463,#58464,#58465),
(#58466,#58467,#58468),(#58469,#58470,#58471),(#58472,#58473,#58474),(#58475,
#58476,#58477),(#58478,#58479,#58480),(#58481,#58482,#58483),(#58484,#58485,
#58486),(#58487,#58488,#58489),(#58490,#58491,#58492),(#58493,#58494,#58495),
(#58496,#58497,#58498),(#58499,#58500,#58501),(#58502,#58503,#58504),(#58505,
#58506,#58507),(#58508,#58509,#58510),(#58511,#58512,#58513),(#58514,#58515,
#58516),(#58517,#58518,#58519),(#58520,#58521,#58522),(#58523,#58524,#58525),
(#58526,#58527,#58528),(#58529,#58530,#58531),(#58532,#58533,#58534),(#58535,
#58536,#58537),(#58538,#58539,#58540),(#58541,#58542,#58543),(#58544,#58545,
#58546),(#58547,#58548,#58549),(#58550,#58551,#58552),(#58553,#58554,#58555),
(#58556,#58557,#58558),(#58559,#58560,#58561),(#58562,#58563,#58564),(#58565,
#58566,#58567),(#58568,#58569,#58570),(#58571,#58572,#58573),(#58574,#58575,
#58576),(#58577,#58578,#58579),(#58580,#58581,#58582),(#58583,#58584,#58585),
(#58586,#58587,#58588),(#58589,#58590,#58591),(#58592,#58593,#58594),(#58595,
#58596,#58597),(#58598,#58599,#58600),(#58601,#58602,#58603),(#58604,#58605,
#58606),(#58607,#58608,#58609),(#58610,#58611,#58612),(#58613,#58614,#58615),
(#58616,#58617,#58618),(#58619,#58620,#58621),(#58622,#58623,#58624),(#58625,
#58626,#58627),(#58628,#58629,#58630),(#58631,#58632,#58633),(#58634,#58635,
#58636),(#58637,#58638,#58639),(#58640,#58641,#58642),(#58643,#58644,#58645),
(#58646,#58647,#58648),(#58649,#58650,#58651),(#58652,#58653,#58654),(#58655,
#58656,#58657),(#58658,#58659,#58660),(#58661,#58662,#58663),(#58664,#58665,
#58666),(#58667,#58668,#58669),(#58670,#58671,#58672),(#58673,#58674,#58675),
(#58676,#58677,#58678),(#58679,#58680,#58681),(#58682,#58683,#58684),(#58685,
#58686,#58687),(#58688,#58689,#58690),(#58691,#58692,#58693),(#58694,#58695,
#58696),(#58697,#58698,#58699),(#58700,#58701,#58702),(#58703,#58704,#58705),
(#58706,#58707,#58708),(#58709,#58710,#58711),(#58712,#58713,#58714),(#58715,
#58716,#58717),(#58718,#58719,#58720),(#58721,#58722,#58723),(#58724,#58725,
#58726),(#58727,#58728,#58729),(#58730,#58731,#58732),(#58733,#58734,#58735),
(#58736,#58737,#58738),(#58739,#58740,#58741),(#58742,#58743,#58744),(#58745,
#58746,#58747),(#58748,#58749,#58750),(#58751,#58752,#58753),(#58754,#58755,
#58756),(#58757,#58758,#58759),(#58760,#58761,#58762),(#58763,#58764,#58765),
(#58766,#58767,#58768),(#58769,#58770,#58771),(#58772,#58773,#58774),(#58775,
#58776,#58777),(#58778,#58779,#58780),(#58781,#58782,#58783),(#58784,#58785,
#58786),(#58787,#58788,#58789),(#58790,#58791,#58792),(#58793,#58794,#58795),
(#58796,#58797,#58798),(#58799,#58800,#58801),(#58802,#58803,#58804),(#58805,
#58806,#58807),(#58808,#58809,#58810),(#58811,#58812,#58813),(#58814,#58815,
#58816),(#58817,#58818,#58819),(#58820,#58821,#58822),(#58823,#58824,#58825),
(#58826,#58827,#58828),(#58829,#58830,#58831),(#58832,#58833,#58834),(#58835,
#58836,#58837),(#58838,#58839,#58840)),.UNSPECIFIED.,.F.,.F.,.F.)
B_SPLINE_SURFACE_WITH_KNOTS((4,2,2,2,2,2,2,2,2,2,2,2,2,2,2,2,2,2,2,2,2,
2,2,2,2,2,2,2,2,2,2,2,2,2,2,2,2,2,2,2,2,2,2,2,2,2,2,2,2,2,2,2,2,2,2,2,2,
2,2,2,2,2,2,2,2,2,2,2,2,2,2,2,2,2,2,2,2,2,2,2,2,2,2,2,2,2,2,2,2,2,2,2,2,
2,2,2,2,2,2,2,2,2,2,2,2,2,2,2,2,2,2,2,2,2,2,2,4),(3,3),(0.0290103847129019,
0.0295538338054091,0.0298255583516626,0.029893489488226,0.0299614206247894,
0.0300972828979162,0.0306407319904233,0.0311841810829305,0.031455905629184,
0.0315917679023108,0.0316596990388742,0.0317276301754376,0.0322710792679447,
0.0328145283604518,0.033357977452959,0.0334938397260857,0.0335617708626491,
0.0336297019992125,0.0339014265454661,0.0344448756379732,0.0349883247304803,
0.0352600492767339,0.0353279804132973,0.0353959115498607,0.0355317738229875,
0.0360752229154946,0.0366186720080017,0.0368903965542553,0.0370262588273821,
0.0371621211005088,0.037705570193016,0.0382490192855231,0.0387924683780302,
0.038928330651157,0.0389962617877204,0.0390641929242838,0.0393359174705374,
0.0398793665630445,0.0404228156555516,0.0406945402018052,0.0408304024749319,
0.0409662647480587,0.0415097138405659,0.042053162933073,0.0425966120255801,
0.0428683365718337,0.0430041988449605,0.0431400611180872,0.0436835102105944,
0.0442269593031015,0.0447704083956086,0.044838339532172,0.0449062706687354,
0.0450421329418622,0.0453138574881158,0.0458573065806229,0.04640075567313,
0.0465366179462568,0.0466045490828202,0.0466724802193836,0.0469442047656371,
0.0474876538581443,0.0480311029506514,0.0480990340872148,0.0481669652237782,
0.0483028274969049,0.0485745520431585,0.0491180011356656,0.0493897256819192,
0.049525587955046,0.0496614502281728,0.0502048993206799,0.050748348413187,
0.0512917975056942,0.0514276597788209,0.0515635220519477,0.0518352465982013,
0.0523786956907084,0.0529221447832155,0.0534655938757227,0.0536014561488494,
0.0537373184219762,0.0540090429682298,0.0541449052413566,0.0542807675144833,
0.0545524920607369,0.055095941153244,0.0556393902457512,0.0559111147920047,
0.0560469770651315,0.0561149082016949,0.0561828393382583,0.0567262884307654,
0.0572697375232725,0.0578131866157797,0.0579490488889065,0.0580849111620332,
0.0583566357082868,0.0589000848007939,0.0594435338933011,0.0597152584395546,
0.059783189576118,0.0598511207126814,0.0599869829858082,0.0605304320783153,
0.0610738811708224,0.061345605717076,0.0614814679902028,0.0615493991267662,
0.0616173302633296,0.0621607793558367,0.0627042284483438,0.0632476775408509,
0.0633156086774143,0.0633835398139777,0.0635194020871045,0.0637911266333581),
(-1.72788130968728E-6,1.),.UNSPECIFIED.)
GEOMETRIC_REPRESENTATION_ITEM()
RATIONAL_B_SPLINE_SURFACE(((1.00000094197663,0.727418595914212,1.),(1.00000094277455,
0.727187698108613,1.),(1.00000094430839,0.726743850528363,1.),(1.00000094768065,
0.725768013810579,1.),(1.00000094898323,0.725391083151896,1.),(1.0000009508298,
0.724856736725869,1.),(1.0000009512101,0.72474668983897,1.),(1.00000095199009,
0.724520983240094,1.),(1.00000095239004,0.724405249820312,1.),(1.00000095361912,
0.72404958662569,1.),(1.00000095447751,0.72380119340961,1.),(1.00000095895618,
0.72250519314825,1.),(1.00000096313739,0.721295268540489,1.),(1.00000097247495,
0.718593243085756,1.),(1.00000097763181,0.717100995140168,1.),(1.00000098591273,
0.714704729614825,1.),(1.00000098876372,0.713879733273474,1.),(1.00000099314999,
0.712610471336212,1.),(1.00000099463035,0.712182096269172,1.),(1.00000099687479,
0.711532620097953,1.),(1.00000099762691,0.711314976265769,1.),(1.00000099913852,
0.710877561277227,1.),(1.00000099989841,0.710657670723553,1.),(1.00000100674924,
0.708675232626428,1.),(1.00000101294924,0.706881126980666,1.),(1.00000102520803,
0.703333782029864,1.),(1.00000103126738,0.701580377140293,1.),(1.00000104286114,
0.698225469884114,1.),(1.00000104839618,0.696623786464909,1.),(1.00000105472174,
0.694793346516954,1.),(1.00000105595707,0.694435878132859,1.),(1.00000105775998,
0.693914167092214,1.),(1.00000105835303,0.693742555644265,1.),(1.00000105951902,
0.693405150014371,1.),(1.00000106009194,0.693239364605067,1.),(1.00000106290441,
0.692425515296011,1.),(1.00000106498762,0.69182269211634,1.),(1.0000010706726,
0.690177620996682,1.),(1.00000107370956,0.689298810815767,1.),(1.00000107793992,
0.688074663091584,1.),(1.00000107913354,0.687729261620368,1.),(1.00000107928995,
0.687684002572033,1.),(1.00000107906974,0.68774772463205,1.),(1.0000010784276,
0.687933540851868,1.),(1.00000107828083,0.687976012571821,1.),(1.00000107794993,
0.688071765808802,1.),(1.00000107776568,0.688125082395367,1.),(1.00000107715803,
0.688300919176998,1.),(1.0000010766791,0.688439508022508,1.),(1.00000107391216,
0.689240182223478,1.),(1.00000107050605,0.690225813636976,1.),(1.0000010612487,
0.692904628638751,1.),(1.00000105539763,0.694597763995586,1.),(1.00000104476396,
0.697674847330772,1.),(1.0000010409101,0.69879004455908,1.),(1.00000103466414,
0.700597449749866,1.),(1.00000103250463,0.70122234989242,1.),(1.0000010280305,
0.702517037582702,1.),(1.00000102571495,0.703187092703321,1.),(1.000001013759,
0.706646805799464,1.),(1.00000100311034,0.709728226570205,1.),(1.00000097986549,
0.716454630491264,1.),(1.00000096726932,0.720099604613224,1.),(1.0000009403451,
0.727890713049425,1.),(1.00000092601706,0.732036842434526,1.),(1.00000090715593,
0.73749472092308,1.),(1.00000090333614,0.738600061506044,1.),(1.00000089753751,
0.74027801909495,1.),(1.00000089559232,0.740840901529955,1.),(1.00000089168822,
0.741970640142475,1.),(1.00000088972839,0.742537758394899,1.),(1.00000087989184,
0.745384178455298,1.),(1.00000087190293,0.74769594190517,1.),(1.00000084763024,
0.754719772705337,1.),(1.00000083104128,0.75952014802879,1.),(1.00000079730879,
0.769281378915179,1.),(1.0000007801649,0.774242333982382,1.),(1.00000075421114,
0.781752620154195,1.),(1.00000074552009,0.784267564565214,1.),(1.00000073244522,
0.788051059686649,1.),(1.00000072808055,0.789314072476293,1.),(1.00000071934197,
0.791842771982262,1.),(1.00000071496481,0.793109396640888,1.),(1.00000069316053,
0.799418938941215,1.),(1.00000067591145,0.804410334492118,1.),(1.00000064200496,
0.81422191448303,1.),(1.00000062534704,0.819042245139272,1.),(1.00000059281998,
0.828454657464615,1.),(1.00000057695027,0.833046904849106,1.),(1.00000055389332,
0.839718934283668,1.),(1.00000054633241,0.841906847587564,1.),(1.00000053519969,
0.845128341016523,1.),(1.00000053152358,0.846192104502361,1.),(1.00000052424476,
0.848298387636058,1.),(1.00000052065556,0.849337000883416,1.),(1.00000050297139,
0.854454300511256,1.),(1.00000048965526,0.858307611902219,1.),(1.00000046484844,
0.865486003998872,1.),(1.00000045335714,0.868811260812436,1.),(1.00000043240277,
0.874874863226948,1.),(1.00000042293878,0.87761347324732,1.),(1.00000041358206,
0.880321043280489,1.),(1.00000041256186,0.880616260389349,1.),(1.000000410564,
0.881194384595568,1.),(1.00000040958579,0.88147745358052,1.),(1.00000040671335,
0.882308655927517,1.),(1.00000040488134,0.882838786291053,1.),(1.00000039963509,
0.884356904421394,1.),(1.0000003964705,0.885272645328228,1.),(1.00000038798589,
0.887727851822622,1.),(1.00000038367343,0.888975755802617,1.),(1.00000037782766,
0.890667356064376,1.),(1.00000037629401,0.891111152415122,1.),(1.00000037620463,
0.891137016136596,1.),(1.00000037627829,0.891115701568441,1.),(1.00000037652826,
0.891043367082923,1.),(1.00000037663496,0.891012491709624,1.),(1.00000037689415,
0.890937487212343,1.),(1.00000037704668,0.890893349204927,1.),(1.000000377923,
0.890639767831579,1.),(1.00000037898762,0.890331698329217,1.),(1.00000038323813,
0.889101720659685,1.),(1.00000038747899,0.887874535749084,1.),(1.00000039863949,
0.884645001760937,1.),(1.00000040555943,0.882642567397013,1.),(1.00000041480412,
0.879967413714825,1.),(1.00000041585162,0.879664298847342,1.),(1.0000004179871,
0.879046350923129,1.),(1.00000041907386,0.878731873543084,1.),(1.00000042238551,
0.877773573685649,1.),(1.00000042466376,0.877114313314577,1.),(1.00000043170345,
0.875077226776075,1.),(1.0000004366697,0.873640133605505,1.),(1.00000045234131,
0.869105213673524,1.),(1.00000046381801,0.865784181073996,1.),(1.00000048242379,
0.860400193058436,1.),(1.00000048885792,0.858538338109017,1.),(1.00000049884142,
0.855649395902143,1.),(1.00000050222466,0.854670383221197,1.),(1.00000050909947,
0.852681008046092,1.),(1.00000051259291,0.85167010350086,1.),(1.00000053030494,
0.846544742360046,1.),(1.00000054512528,0.842256156889833,1.),(1.00000057583858,
0.833368594516816,1.),(1.00000059173227,0.828769411125496,1.),(1.00000062439208,
0.81931858601259,1.),(1.00000064115875,0.814466783467411,1.),(1.00000066254231,
0.808278986583686,1.),(1.00000066684028,0.807035275537529,1.),(1.00000067547568,
0.804536435116907,1.),(1.00000067980235,0.803284419130001,1.),(1.00000069278865,
0.799526552678708,1.),(1.00000070146116,0.797016971575482,1.),(1.00000072748197,
0.789487284521765,1.),(1.00000074483388,0.784466133705224,1.),(1.00000077932073,
0.77448661498812,1.),(1.00000079645607,0.76952813210456,1.),(1.00000083026845,
0.759743783371996,1.),(1.00000084694591,0.754917798013528,1.),(1.00000086733813,
0.749016865533183,1.),(1.00000087139383,0.74784326137115,1.),(1.00000087942808,
0.745518375589863,1.),(1.00000088341008,0.744366098414126,1.),(1.00000089524472,
0.74094148805281,1.),(1.00000090298606,0.738701364424776,1.),(1.00000091435093,
0.735412692841522,1.),(1.00000091809802,0.734328390689723,1.),(1.0000009255056,
0.732184846770628,1.),(1.00000092916803,0.73112504109884,1.),(1.00000093998345,
0.727995364774212,1.),(1.00000094697548,0.725972070020501,1.),(1.00000096726284,
0.720101479727836,1.),(1.00000097986941,0.7164534949861,1.),(1.00000100306537,
0.709741240019853,1.),(1.00000101365467,0.706676997713043,1.),(1.00000102789253,
0.702556963714663,1.),(1.00000103236417,0.70126299759053,1.),(1.00000103864392,
0.69944581371337,1.),(1.00000104066589,0.698860712318966,1.),(1.00000104358993,
0.698014577829412,1.),(1.0000010445468,0.697737688580098,1.),(1.00000104641865,
0.697196027550747,1.),(1.0000010473343,0.696931065246606,1.),(1.00000105539338,
0.69459899336011,1.),(1.00000106126382,0.692900253988097,1.),(1.00000107051798,
0.690222363085288,1.),(1.00000107390152,0.689243262016709,1.),(1.00000107830538,
0.687968908792342,1.),(1.00000107932556,0.687673698960344,1.),(1.00000107921905,
0.687704517724663,1.),(1.00000107912874,0.687730650887494,1.),(1.00000107881281,
0.687822073848177,1.),(1.00000107858785,0.687887170866826,1.),(1.00000107772176,
0.688137791537803,1.),(1.00000107688939,0.688378656929289,1.),(1.00000107370219,
0.689300942103724,1.),(1.00000107065772,0.690181924746401,1.),(1.0000010631148,
0.692364632289744,1.),(1.00000105861603,0.693666449756497,1.),(1.00000105105817,
0.695853481128863,1.),(1.00000104840388,0.696621557639583,1.),(1.00000104494645,
0.697622039003881,1.),(1.00000104424769,0.69782424123167,1.),(1.00000104284087,
0.698231334628583,1.),(1.00000104213239,0.698436349669935,1.),(1.00000103999302,
0.699055423277568,1.),(1.00000103854822,0.699473508202277,1.),(1.00000103124828,
0.701585903182804,1.),(1.0000010251674,0.703345538833113,1.),(1.00000101291955,
0.706889718420206,1.),(1.00000100675193,0.708674454447466,1.),(1.00000099770163,
0.711293356482619,1.),(1.00000099471813,0.712156696596124,1.),(1.00000099032442,
0.713428111831309,1.),(1.00000098887343,0.713847987019327,1.),(1.00000098672121,
0.71447077836442,1.),(1.00000098600749,0.714677308358767,1.),(1.00000098459043,
0.715087365979716,1.),(1.00000098388775,0.715290702390871,1.),(1.00000097761853,
0.717104837900671,1.),(1.00000097243836,0.718603831103779,1.),(1.00000096309419,
0.721307768765821,1.),(1.00000095892963,0.722512874625052,1.),(1.00000095181024,
0.724573025448519,1.),(1.00000094885502,0.72542818325312,1.),(1.00000094630728,
0.72616542721051,1.),(1.00000094603498,0.726244223849717,1.),(1.00000094551225,
0.726395485734667,1.),(1.0000009452617,0.726467988945064,1.),(1.00000094454426,
0.726675594380443,1.),(1.00000094411234,0.726800580220694,1.),(1.00000094295592,
0.727135216917278,1.),(1.00000094237078,0.727304540475937,1.),(1.00000094197156,
0.72742006218996,1.)))
REPRESENTATION_ITEM('')
SURFACE()
);
#182=(
BOUNDED_SURFACE()
B_SPLINE_SURFACE(3,2,((#58863,#58864,#58865),(#58866,#58867,#58868),(#58869,
#58870,#58871),(#58872,#58873,#58874),(#58875,#58876,#58877),(#58878,#58879,
#58880),(#58881,#58882,#58883),(#58884,#58885,#58886),(#58887,#58888,#58889),
(#58890,#58891,#58892),(#58893,#58894,#58895),(#58896,#58897,#58898),(#58899,
#58900,#58901),(#58902,#58903,#58904),(#58905,#58906,#58907),(#58908,#58909,
#58910),(#58911,#58912,#58913),(#58914,#58915,#58916),(#58917,#58918,#58919),
(#58920,#58921,#58922),(#58923,#58924,#58925),(#58926,#58927,#58928),(#58929,
#58930,#58931),(#58932,#58933,#58934),(#58935,#58936,#58937),(#58938,#58939,
#58940),(#58941,#58942,#58943),(#58944,#58945,#58946),(#58947,#58948,#58949),
(#58950,#58951,#58952),(#58953,#58954,#58955),(#58956,#58957,#58958),(#58959,
#58960,#58961),(#58962,#58963,#58964)),.UNSPECIFIED.,.F.,.F.,.F.)
B_SPLINE_SURFACE_WITH_KNOTS((4,2,2,2,2,2,2,2,2,2,2,2,2,2,2,2,4),(3,3),(1.57074065524005,
1.71325309204606,1.85570985729722,1.99816662254838,2.14062338779954,2.28308015305071,
2.42553691830187,2.56799368355303,2.71045044880419,2.85290721405535,2.99536397930651,
3.13782074455768,3.28027750980884,3.42273427506,3.56519104031116,3.70764780556232,
3.85010457081348),(0.,1.00005567155485),.UNSPECIFIED.)
GEOMETRIC_REPRESENTATION_ITEM()
RATIONAL_B_SPLINE_SURFACE(((1.,0.707079920138348,1.00003261463259),(1.,
0.716086689006554,1.00003161179093),(1.,0.724920009118845,1.0000306282616),
(1.,0.742104597504674,1.00002871487609),(1.,0.75045582409158,1.00002778502455),
(1.,0.76656425844358,1.00002599146138),(1.,0.774321529260281,1.00002512774272),
(1.,0.789143223578738,1.00002347744919),(1.,0.796207699042566,1.00002269086852),
(1.,0.809559621853178,1.00002120422392),(1.,0.815847110870319,1.00002050415534),
(1.,0.827574222198235,1.00001919842229),(1.,0.833013877192258,1.00001859275419),
(1.,0.842986797390786,1.00001748233824),(1.,0.847520087651854,1.00001697758761),
(1.,0.855633281940707,1.00001607423933),(1.,0.859213204604135,1.0000156756396),
(1.,0.865383603626224,1.00001498860819),(1.,0.867974093167104,1.00001470017503),
(1.,0.872140077171102,1.00001423632141),(1.,0.873715580073823,1.00001406090002),
(1.,0.875836267380118,1.0000138247761),(1.,0.876381455942513,1.00001376407311),
(1.,0.876436251233421,1.00001375797203),(1.,0.875945858068014,1.00001381257393),
(1.,0.873934231083751,1.00001403655474),(1.,0.872412993324182,1.00001420593408),
(1.,0.868354473220934,1.00001465782233),(1.,0.865817182673778,1.00001494033215),
(1.,0.859751567664865,1.00001561569659),(1.,0.856223230287758,1.00001600855264),
(1.,0.848211026545572,1.00001690065632),(1.,0.843727317065168,1.00001739988648),
(1.,0.838788701080504,1.00001794976734)))
REPRESENTATION_ITEM('')
SURFACE()
);
#183=(
BOUNDED_SURFACE()
B_SPLINE_SURFACE(3,2,((#59053,#59054,#59055),(#59056,#59057,#59058),(#59059,
#59060,#59061),(#59062,#59063,#59064),(#59065,#59066,#59067),(#59068,#59069,
#59070),(#59071,#59072,#59073),(#59074,#59075,#59076),(#59077,#59078,#59079),
(#59080,#59081,#59082),(#59083,#59084,#59085),(#59086,#59087,#59088),(#59089,
#59090,#59091),(#59092,#59093,#59094),(#59095,#59096,#59097),(#59098,#59099,
#59100),(#59101,#59102,#59103),(#59104,#59105,#59106),(#59107,#59108,#59109),
(#59110,#59111,#59112),(#59113,#59114,#59115),(#59116,#59117,#59118),(#59119,
#59120,#59121),(#59122,#59123,#59124),(#59125,#59126,#59127),(#59128,#59129,
#59130),(#59131,#59132,#59133),(#59134,#59135,#59136),(#59137,#59138,#59139),
(#59140,#59141,#59142),(#59143,#59144,#59145),(#59146,#59147,#59148),(#59149,
#59150,#59151),(#59152,#59153,#59154),(#59155,#59156,#59157),(#59158,#59159,
#59160),(#59161,#59162,#59163),(#59164,#59165,#59166),(#59167,#59168,#59169),
(#59170,#59171,#59172),(#59173,#59174,#59175),(#59176,#59177,#59178),(#59179,
#59180,#59181),(#59182,#59183,#59184),(#59185,#59186,#59187),(#59188,#59189,
#59190),(#59191,#59192,#59193),(#59194,#59195,#59196),(#59197,#59198,#59199),
(#59200,#59201,#59202)),.UNSPECIFIED.,.F.,.F.,.F.)
B_SPLINE_SURFACE_WITH_KNOTS((4,2,2,2,2,2,2,2,2,2,2,2,2,2,2,2,2,2,2,2,2,
2,2,2,4),(3,3),(0.0168736397610245,0.0173205003855472,0.0177673610100698,
0.0178790761662005,0.0179907913223312,0.0182142216345925,0.0186610822591151,
0.0191079428836378,0.0195548035081605,0.0197782338204218,0.0198899489765524,
0.0200016641326831,0.0204485247572058,0.0205602399133364,0.0206719550694671,
0.0208953853817284,0.0213422460062511,0.0217891066307737,0.0222359672552964,
0.0224593975675577,0.0225711127236884,0.022682827879819,0.0231296885043417,
0.0235765491288643,0.024023409753387),(0.,1.),.UNSPECIFIED.)
GEOMETRIC_REPRESENTATION_ITEM()
RATIONAL_B_SPLINE_SURFACE(((1.,0.676185655324359,1.),(1.,0.67630322416838,
1.),(1.,0.676584997615303,1.),(1.,0.67743451044132,1.),(1.,0.678002280027087,
1.),(1.,0.678863512103858,1.),(1.,0.679043447440726,1.),(1.,0.679417253471516,
1.),(1.,0.679610743089326,1.),(1.,0.680209528048005,1.),(1.,0.680633128730709,
1.),(1.,0.681966035229257,1.),(1.,0.682937305222825,1.),(1.,0.684989680316945,
1.),(1.,0.686070826789687,1.),(1.,0.688291564262565,1.),(1.,0.689431193575673,
1.),(1.,0.691148055248714,1.),(1.,0.691721597513498,1.),(1.,0.692579366019322,
1.),(1.,0.692864861918766,1.),(1.,0.693432626773667,1.),(1.,0.693715104487649,
1.),(1.,0.695118751522096,1.),(1.,0.696213531941737,1.),(1.,0.697521120294898,
1.),(1.,0.697779622667988,1.),(1.,0.698289874383767,1.),(1.,0.698541099245874,
1.),(1.,0.699282339144899,1.),(1.,0.699759908934221,1.),(1.,0.701137406672921,
1.),(1.,0.701981987768826,1.),(1.,0.703498354563225,1.),(1.,0.704170174913113,
1.),(1.,0.705319738998922,1.),(1.,0.705797505956189,1.),(1.,0.706354933867263,
1.),(1.,0.706514227956655,1.),(1.,0.706711865981927,1.),(1.,0.706770862676804,
1.),(1.,0.70687484959442,1.),(1.,0.706919686161599,1.),(1.,0.707108074228766,
1.),(1.,0.707144248395913,1.),(1.,0.706992159157227,1.),(1.,0.706803894595462,
1.),(1.,0.706210527095295,1.),(1.,0.705805464605862,1.),(1.,0.705297251064667,
1.)))
REPRESENTATION_ITEM('')
SURFACE()
);
#184=(
BOUNDED_SURFACE()
B_SPLINE_SURFACE(3,2,((#59299,#59300,#59301),(#59302,#59303,#59304),(#59305,
#59306,#59307),(#59308,#59309,#59310),(#59311,#59312,#59313),(#59314,#59315,
#59316),(#59317,#59318,#59319),(#59320,#59321,#59322),(#59323,#59324,#59325),
(#59326,#59327,#59328),(#59329,#59330,#59331),(#59332,#59333,#59334),(#59335,
#59336,#59337),(#59338,#59339,#59340),(#59341,#59342,#59343),(#59344,#59345,
#59346),(#59347,#59348,#59349),(#59350,#59351,#59352),(#59353,#59354,#59355),
(#59356,#59357,#59358),(#59359,#59360,#59361),(#59362,#59363,#59364),(#59365,
#59366,#59367),(#59368,#59369,#59370),(#59371,#59372,#59373),(#59374,#59375,
#59376),(#59377,#59378,#59379),(#59380,#59381,#59382),(#59383,#59384,#59385),
(#59386,#59387,#59388),(#59389,#59390,#59391),(#59392,#59393,#59394),(#59395,
#59396,#59397),(#59398,#59399,#59400),(#59401,#59402,#59403),(#59404,#59405,
#59406),(#59407,#59408,#59409),(#59410,#59411,#59412),(#59413,#59414,#59415),
(#59416,#59417,#59418),(#59419,#59420,#59421),(#59422,#59423,#59424),(#59425,
#59426,#59427),(#59428,#59429,#59430),(#59431,#59432,#59433),(#59434,#59435,
#59436),(#59437,#59438,#59439),(#59440,#59441,#59442),(#59443,#59444,#59445),
(#59446,#59447,#59448),(#59449,#59450,#59451),(#59452,#59453,#59454),(#59455,
#59456,#59457),(#59458,#59459,#59460),(#59461,#59462,#59463),(#59464,#59465,
#59466),(#59467,#59468,#59469),(#59470,#59471,#59472),(#59473,#59474,#59475),
(#59476,#59477,#59478),(#59479,#59480,#59481),(#59482,#59483,#59484),(#59485,
#59486,#59487),(#59488,#59489,#59490),(#59491,#59492,#59493),(#59494,#59495,
#59496),(#59497,#59498,#59499),(#59500,#59501,#59502),(#59503,#59504,#59505),
(#59506,#59507,#59508),(#59509,#59510,#59511),(#59512,#59513,#59514),(#59515,
#59516,#59517),(#59518,#59519,#59520),(#59521,#59522,#59523),(#59524,#59525,
#59526),(#59527,#59528,#59529),(#59530,#59531,#59532),(#59533,#59534,#59535),
(#59536,#59537,#59538),(#59539,#59540,#59541),(#59542,#59543,#59544),(#59545,
#59546,#59547),(#59548,#59549,#59550),(#59551,#59552,#59553),(#59554,#59555,
#59556),(#59557,#59558,#59559),(#59560,#59561,#59562),(#59563,#59564,#59565),
(#59566,#59567,#59568),(#59569,#59570,#59571),(#59572,#59573,#59574),(#59575,
#59576,#59577),(#59578,#59579,#59580),(#59581,#59582,#59583),(#59584,#59585,
#59586)),.UNSPECIFIED.,.F.,.F.,.F.)
B_SPLINE_SURFACE_WITH_KNOTS((4,2,2,2,2,2,2,2,2,2,2,2,2,2,2,2,2,2,2,2,2,
2,2,2,2,2,2,2,2,2,2,2,2,2,2,2,2,2,2,2,2,2,2,2,2,2,2,4),(3,3),(0.0133656719252939,
0.0137531204885812,0.0139468447702248,0.0140437069110466,0.0140921379814575,
0.0141405690518684,0.0145280176151557,0.0149154661784429,0.0153029147417302,
0.0154966390233738,0.0155935011641956,0.0156419322346065,0.0156903633050174,
0.0160778118683047,0.0164652604315919,0.0168527089948792,0.0170464332765228,
0.0171432954173446,0.0172401575581664,0.0176276061214537,0.0180150546847409,
0.0184025032480282,0.0187899518113154,0.0191774003746027,0.0192742625154245,
0.0193711246562463,0.0195648489378899,0.0199522975011772,0.020049159641999,
0.0201460217828208,0.0203397460644644,0.0207271946277517,0.0211146431910389,
0.0215020917543262,0.0218895403176134,0.0222769888809007,0.0224707131625443,
0.0225675753033661,0.0226644374441879,0.0234393345707625,0.0238267831340497,
0.024214231697337,0.0246016802606242,0.0249891288239115,0.0250859909647333,
0.0251828531055551,0.0253765773871987,0.025764025950486),(0.,1.),
 .UNSPECIFIED.)
GEOMETRIC_REPRESENTATION_ITEM()
RATIONAL_B_SPLINE_SURFACE(((1.,0.9140223922261,1.),(1.,0.915030492709283,
1.),(1.,0.915858639583001,1.),(1.,0.916817715499207,1.),(1.,0.917090200413126,
1.),(1.,0.917426174788986,1.),(1.,0.917526038338742,1.),(1.,0.917657375959307,
1.),(1.,0.917698072660668,1.),(1.,0.917773091161791,1.),(1.,0.917807443115215,
1.),(1.,0.918088314388304,1.),(1.,0.918136915427419,1.),(1.,0.917843376479416,
1.),(1.,0.917501223822225,1.),(1.,0.916433977111706,1.),(1.,0.915708876551461,
1.),(1.,0.914337422509701,1.),(1.,0.913832945692125,1.),(1.,0.913005446344792,
1.),(1.,0.912717814337712,1.),(1.,0.912268679644456,1.),(1.,0.912115982606894,
1.),(1.,0.911805397365888,1.),(1.,0.911647430343649,1.),(1.,0.910201898284099,
1.),(1.,0.908747768522694,1.),(1.,0.905525061106013,1.),(1.,0.903756442170294,
1.),(1.,0.899923635221016,1.),(1.,0.897859417630057,1.),(1.,0.89455261711194,
1.),(1.,0.893415243056036,1.),(1.,0.891657695042151,1.),(1.,0.891062827486455,
1.),(1.,0.889859964219412,1.),(1.,0.889251636022491,1.),(1.,0.886176395534851,
1.),(1.,0.883608843556552,1.),(1.,0.878278885688577,1.),(1.,0.875516441111426,
1.),(1.,0.869813110038265,1.),(1.,0.86687219535343,1.),(1.,0.860825971449527,
1.),(1.,0.857720640581297,1.),(1.,0.851357997915466,1.),(1.,0.848100668446161,
1.),(1.,0.843941117270504,1.),(1.,0.843104810668739,1.),(1.,0.841423576195933,
1.),(1.,0.840578661667794,1.),(1.,0.838036046535061,1.),(1.,0.83632889783711,
1.),(1.,0.831173872679246,1.),(1.,0.827692420000005,1.),(1.,0.823293277529827,
1.),(1.,0.822411082406562,1.),(1.,0.820642174664206,1.),(1.,0.819755100414045,
1.),(1.,0.817090095259101,1.),(1.,0.815309850858671,1.),(1.,0.809961218322665,
1.),(1.,0.806384920527092,1.),(1.,0.799226404991901,1.),(1.,0.79564417490575,
1.),(1.,0.788489405141087,1.),(1.,0.784916853795515,1.),(1.,0.777797878098423,
1.),(1.,0.774251441980022,1.),(1.,0.767202304821984,1.),(1.,0.763699591208166,
1.),(1.,0.758492675884238,1.),(1.,0.756764909690213,1.),(1.,0.754186996432683,
1.),(1.,0.753329982306773,1.),(1.,0.75162086832093,1.),(1.,0.750768672063171,
1.),(1.,0.743147593559799,1.),(1.,0.736674219140203,1.),(1.,0.727518317868808,
1.),(1.,0.724558786513214,1.),(1.,0.718842636618393,1.),(1.,0.716086018731709,
1.),(1.,0.710794331727339,1.),(1.,0.708259263721099,1.),(1.,0.703429876147357,
1.),(1.,0.701135557954403,1.),(1.,0.698430453857348,1.),(1.,0.697897573909109,
1.),(1.,0.696848408664233,1.),(1.,0.696333170170124,1.),(1.,0.694818010360577,
1.),(1.,0.693847579638783,1.),(1.,0.691055128022452,1.),(1.,0.689351969841444,
1.),(1.,0.687806373745967,1.)))
REPRESENTATION_ITEM('')
SURFACE()
);
#185=(
BOUNDED_SURFACE()
B_SPLINE_SURFACE(3,2,((#59772,#59773,#59774),(#59775,#59776,#59777),(#59778,
#59779,#59780),(#59781,#59782,#59783),(#59784,#59785,#59786),(#59787,#59788,
#59789),(#59790,#59791,#59792),(#59793,#59794,#59795),(#59796,#59797,#59798),
(#59799,#59800,#59801),(#59802,#59803,#59804),(#59805,#59806,#59807),(#59808,
#59809,#59810),(#59811,#59812,#59813),(#59814,#59815,#59816),(#59817,#59818,
#59819),(#59820,#59821,#59822),(#59823,#59824,#59825),(#59826,#59827,#59828),
(#59829,#59830,#59831),(#59832,#59833,#59834),(#59835,#59836,#59837),(#59838,
#59839,#59840),(#59841,#59842,#59843),(#59844,#59845,#59846),(#59847,#59848,
#59849),(#59850,#59851,#59852),(#59853,#59854,#59855),(#59856,#59857,#59858),
(#59859,#59860,#59861),(#59862,#59863,#59864),(#59865,#59866,#59867),(#59868,
#59869,#59870),(#59871,#59872,#59873),(#59874,#59875,#59876),(#59877,#59878,
#59879),(#59880,#59881,#59882),(#59883,#59884,#59885),(#59886,#59887,#59888),
(#59889,#59890,#59891),(#59892,#59893,#59894),(#59895,#59896,#59897),(#59898,
#59899,#59900),(#59901,#59902,#59903),(#59904,#59905,#59906),(#59907,#59908,
#59909),(#59910,#59911,#59912),(#59913,#59914,#59915),(#59916,#59917,#59918),
(#59919,#59920,#59921),(#59922,#59923,#59924),(#59925,#59926,#59927),(#59928,
#59929,#59930),(#59931,#59932,#59933),(#59934,#59935,#59936),(#59937,#59938,
#59939),(#59940,#59941,#59942),(#59943,#59944,#59945),(#59946,#59947,#59948),
(#59949,#59950,#59951),(#59952,#59953,#59954),(#59955,#59956,#59957),(#59958,
#59959,#59960),(#59961,#59962,#59963),(#59964,#59965,#59966),(#59967,#59968,
#59969),(#59970,#59971,#59972),(#59973,#59974,#59975),(#59976,#59977,#59978),
(#59979,#59980,#59981),(#59982,#59983,#59984),(#59985,#59986,#59987),(#59988,
#59989,#59990),(#59991,#59992,#59993),(#59994,#59995,#59996),(#59997,#59998,
#59999),(#60000,#60001,#60002),(#60003,#60004,#60005),(#60006,#60007,#60008),
(#60009,#60010,#60011),(#60012,#60013,#60014),(#60015,#60016,#60017),(#60018,
#60019,#60020),(#60021,#60022,#60023),(#60024,#60025,#60026),(#60027,#60028,
#60029),(#60030,#60031,#60032),(#60033,#60034,#60035),(#60036,#60037,#60038),
(#60039,#60040,#60041),(#60042,#60043,#60044),(#60045,#60046,#60047),(#60048,
#60049,#60050),(#60051,#60052,#60053),(#60054,#60055,#60056),(#60057,#60058,
#60059),(#60060,#60061,#60062),(#60063,#60064,#60065),(#60066,#60067,#60068),
(#60069,#60070,#60071),(#60072,#60073,#60074),(#60075,#60076,#60077),(#60078,
#60079,#60080),(#60081,#60082,#60083),(#60084,#60085,#60086),(#60087,#60088,
#60089),(#60090,#60091,#60092),(#60093,#60094,#60095),(#60096,#60097,#60098),
(#60099,#60100,#60101),(#60102,#60103,#60104),(#60105,#60106,#60107),(#60108,
#60109,#60110),(#60111,#60112,#60113),(#60114,#60115,#60116),(#60117,#60118,
#60119),(#60120,#60121,#60122),(#60123,#60124,#60125),(#60126,#60127,#60128),
(#60129,#60130,#60131),(#60132,#60133,#60134),(#60135,#60136,#60137),(#60138,
#60139,#60140),(#60141,#60142,#60143),(#60144,#60145,#60146),(#60147,#60148,
#60149),(#60150,#60151,#60152),(#60153,#60154,#60155),(#60156,#60157,#60158),
(#60159,#60160,#60161),(#60162,#60163,#60164),(#60165,#60166,#60167),(#60168,
#60169,#60170),(#60171,#60172,#60173),(#60174,#60175,#60176),(#60177,#60178,
#60179),(#60180,#60181,#60182),(#60183,#60184,#60185),(#60186,#60187,#60188),
(#60189,#60190,#60191),(#60192,#60193,#60194),(#60195,#60196,#60197),(#60198,
#60199,#60200),(#60201,#60202,#60203),(#60204,#60205,#60206),(#60207,#60208,
#60209),(#60210,#60211,#60212),(#60213,#60214,#60215),(#60216,#60217,#60218),
(#60219,#60220,#60221),(#60222,#60223,#60224),(#60225,#60226,#60227),(#60228,
#60229,#60230),(#60231,#60232,#60233),(#60234,#60235,#60236),(#60237,#60238,
#60239),(#60240,#60241,#60242),(#60243,#60244,#60245),(#60246,#60247,#60248),
(#60249,#60250,#60251),(#60252,#60253,#60254),(#60255,#60256,#60257),(#60258,
#60259,#60260),(#60261,#60262,#60263),(#60264,#60265,#60266),(#60267,#60268,
#60269),(#60270,#60271,#60272),(#60273,#60274,#60275),(#60276,#60277,#60278),
(#60279,#60280,#60281),(#60282,#60283,#60284),(#60285,#60286,#60287),(#60288,
#60289,#60290),(#60291,#60292,#60293),(#60294,#60295,#60296),(#60297,#60298,
#60299),(#60300,#60301,#60302),(#60303,#60304,#60305),(#60306,#60307,#60308),
(#60309,#60310,#60311),(#60312,#60313,#60314),(#60315,#60316,#60317),(#60318,
#60319,#60320),(#60321,#60322,#60323),(#60324,#60325,#60326),(#60327,#60328,
#60329),(#60330,#60331,#60332),(#60333,#60334,#60335),(#60336,#60337,#60338),
(#60339,#60340,#60341),(#60342,#60343,#60344),(#60345,#60346,#60347),(#60348,
#60349,#60350),(#60351,#60352,#60353),(#60354,#60355,#60356),(#60357,#60358,
#60359),(#60360,#60361,#60362),(#60363,#60364,#60365),(#60366,#60367,#60368),
(#60369,#60370,#60371),(#60372,#60373,#60374),(#60375,#60376,#60377),(#60378,
#60379,#60380),(#60381,#60382,#60383),(#60384,#60385,#60386),(#60387,#60388,
#60389),(#60390,#60391,#60392),(#60393,#60394,#60395),(#60396,#60397,#60398),
(#60399,#60400,#60401),(#60402,#60403,#60404),(#60405,#60406,#60407),(#60408,
#60409,#60410),(#60411,#60412,#60413),(#60414,#60415,#60416),(#60417,#60418,
#60419),(#60420,#60421,#60422),(#60423,#60424,#60425),(#60426,#60427,#60428),
(#60429,#60430,#60431),(#60432,#60433,#60434),(#60435,#60436,#60437),(#60438,
#60439,#60440),(#60441,#60442,#60443),(#60444,#60445,#60446),(#60447,#60448,
#60449),(#60450,#60451,#60452),(#60453,#60454,#60455),(#60456,#60457,#60458),
(#60459,#60460,#60461),(#60462,#60463,#60464),(#60465,#60466,#60467),(#60468,
#60469,#60470),(#60471,#60472,#60473),(#60474,#60475,#60476),(#60477,#60478,
#60479),(#60480,#60481,#60482),(#60483,#60484,#60485),(#60486,#60487,#60488),
(#60489,#60490,#60491),(#60492,#60493,#60494),(#60495,#60496,#60497),(#60498,
#60499,#60500),(#60501,#60502,#60503),(#60504,#60505,#60506),(#60507,#60508,
#60509),(#60510,#60511,#60512),(#60513,#60514,#60515),(#60516,#60517,#60518),
(#60519,#60520,#60521),(#60522,#60523,#60524),(#60525,#60526,#60527),(#60528,
#60529,#60530),(#60531,#60532,#60533),(#60534,#60535,#60536),(#60537,#60538,
#60539),(#60540,#60541,#60542),(#60543,#60544,#60545),(#60546,#60547,#60548),
(#60549,#60550,#60551),(#60552,#60553,#60554),(#60555,#60556,#60557)),
 .UNSPECIFIED.,.T.,.F.,.F.)
B_SPLINE_SURFACE_WITH_KNOTS((4,2,2,2,2,2,2,2,2,2,2,2,2,2,2,2,2,2,2,2,2,
2,2,2,2,2,2,2,2,2,2,2,2,2,2,2,2,2,2,2,2,2,2,2,2,2,2,2,2,2,2,2,2,2,2,2,2,
2,2,2,2,2,2,2,2,2,2,2,2,2,2,2,2,2,2,2,2,2,2,2,2,2,2,2,2,2,2,2,2,2,2,2,2,
2,2,2,2,2,2,2,2,2,2,2,2,2,2,2,2,2,2,2,2,2,2,2,2,2,2,2,2,2,2,2,2,2,2,2,2,
2,4),(3,3),(0.,5.58974039156775E-5,0.000111794807831355,0.00022358961566271,
0.00044717923132542,0.000894358462650841,0.00178871692530168,0.00268307538795252,
0.00279487019578388,0.00290666500361523,0.00313025461927794,0.00357743385060336,
0.0044717923132542,0.00536615077590504,0.0054779455837364,0.00558974039156775,
0.00581333000723046,0.00626050923855589,0.00715486770120673,0.00804922616385757,
0.00827281577952028,0.00838461058735163,0.00849640539518299,0.00894358462650841,
0.00983794308915925,0.0107323015518101,0.0111794807831355,0.0114030703987982,
0.0115148652066296,0.0116266600144609,0.0125210184771118,0.0134153769397626,
0.013862556171088,0.0143097354024135,0.0145333250180762,0.0146451198259075,
0.0147569146337389,0.0152040938650643,0.0160984523277151,0.016992810790366,
0.0172164004060287,0.01732819521386,0.0174399900216914,0.0178871692530168,
0.0187815277156677,0.0196758861783185,0.0198994757939812,0.0201230654096439,
0.0205702446409693,0.0214646031036202,0.022358961566271,0.0228061407975964,
0.0230297304132591,0.0232533200289219,0.0241476784915727,0.0250420369542235,
0.0259363954168744,0.0261599850325371,0.0262717798403685,0.0263835746481998,
0.0268307538795252,0.0277251123421761,0.0286194708048269,0.0290666500361523,
0.029290239651815,0.0294020344596464,0.0295138292674777,0.0299610084988032,
0.0301845981144659,0.0302963929222972,0.0304081877301286,0.0313025461927794,
0.0321969046554303,0.0330912631180811,0.0332030579259125,0.0333148527337438,
0.0335384423494065,0.0339856215807319,0.0348799800433828,0.0357743385060336,
0.0359979281216963,0.0361097229295277,0.036221517737359,0.0366686969686845,
0.0375630554313353,0.0384574138939862,0.0389045931253116,0.0391281827409743,
0.0392399775488056,0.039351772356637,0.0402461308192878,0.0411404892819387,
0.0420348477445895,0.0424820269759149,0.0425938217837463,0.0427056165915777,
0.0429292062072404,0.0433763854385658,0.0438235646698912,0.044717923132542,
0.0451651023638675,0.0452768971716988,0.0453886919795302,0.0456122815951929,
0.0465066400578437,0.0474009985204946,0.04784817775182,0.0479599725596513,
0.0480717673674827,0.0482953569831454,0.0491897154457962,0.0500840739084471,
0.0505312531397725,0.0507548427554352,0.0508666375632666,0.0509784323710979,
0.0518727908337488,0.0527671492963996,0.0536615077590504,0.0538850973747132,
0.0539968921825445,0.0541086869903759,0.0545558662217013,0.0554502246843521,
0.056344583147003,0.0567917623783284,0.0570153519939911,0.0571271468018225,
0.0571830442057381,0.057210992907696,0.0572389416096538),(0.,1.),
 .UNSPECIFIED.)
GEOMETRIC_REPRESENTATION_ITEM()
RATIONAL_B_SPLINE_SURFACE(((1.,0.869037098890924,1.),(1.,0.869090662160833,
1.),(1.,0.869142132128297,1.),(1.,0.869241273997536,1.),(1.,0.869288882663707,
1.),(1.,0.869425835273797,1.),(1.,0.869509305917427,1.),(1.,0.869736328335375,
1.),(1.,0.869856492063896,1.),(1.,0.870124205131434,1.),(1.,0.870178998389397,
1.),(1.,0.869977707911342,1.),(1.,0.869356264735848,1.),(1.,0.867159523791841,
1.),(1.,0.865584183970151,1.),(1.,0.863281618119441,1.),(1.,0.86301835474559,
1.),(1.,0.862477312320675,1.),(1.,0.862200065545979,1.),(1.,0.861348450829986,
1.),(1.,0.860754210958995,1.),(1.,0.858894323573958,1.),(1.,0.857551540639133,
1.),(1.,0.853231873120265,1.),(1.,0.849963976579328,1.),(1.,0.8427337476379,
1.),(1.,0.838771159914112,1.),(1.,0.833964492549446,1.),(1.,0.83342564158097,
1.),(1.,0.832341102831786,1.),(1.,0.831795088875303,1.),(1.,0.83014615568217,
1.),(1.,0.829032346207458,1.),(1.,0.825650047625046,1.),(1.,0.823340697393356,
1.),(1.,0.816270214875414,1.),(1.,0.811366531889991,1.),(1.,0.801290493401484,
1.),(1.,0.796117786007922,1.),(1.,0.789558114002489,1.),(1.,0.788241524410975,
1.),(1.,0.786261176106014,1.),(1.,0.785600666410631,1.),(1.,0.784281253478811,
1.),(1.,0.783622032027989,1.),(1.,0.780329023537139,1.),(1.,0.777704514650253,
1.),(1.,0.76988692542286,1.),(1.,0.764749330047637,1.),(1.,0.75477051537079,
1.),(1.,0.749929030998746,1.),(1.,0.743012971461713,1.),(1.,0.740765474239869,
1.),(1.,0.73749827976927,1.),(1.,0.736426570328376,1.),(1.,0.734847329496033,
1.),(1.,0.734325595116705,1.),(1.,0.733292134556225,1.),(1.,0.732781563072735,
1.),(1.,0.728242967029025,1.),(1.,0.724610876621003,1.),(1.,0.718276943716503,
1.),(1.,0.715575135642169,1.),(1.,0.712312229125148,1.),(1.,0.711356200483893,
1.),(1.,0.709722323386846,1.),(1.,0.709044475655852,1.),(1.,0.708247344579823,
1.),(1.,0.708018238565296,1.),(1.,0.707730840005604,1.),(1.,0.707644376240716,
1.),(1.,0.707490608795043,1.),(1.,0.707423402545753,1.),(1.,0.707135559015692,
1.),(1.,0.707059523314824,1.),(1.,0.707285549205988,1.),(1.,0.708042221657254,
1.),(1.,0.710710092253751,1.),(1.,0.712621237041365,1.),(1.,0.715686665981657,
1.),(1.,0.716333543550958,1.),(1.,0.717353607349392,1.),(1.,0.717701919486094,
1.),(1.,0.718414964313171,1.),(1.,0.718779962361759,1.),(1.,0.720642167884513,
1.),(1.,0.722248110686464,1.),(1.,0.727379897082438,1.),(1.,0.731219242886661,
1.),(1.,0.739562059134817,1.),(1.,0.744065650037015,1.),(1.,0.750011006364496,
1.),(1.,0.751215898212902,1.),(1.,0.753654939425893,1.),(1.,0.754889413958793,
1.),(1.,0.758631191877784,1.),(1.,0.761160349547001,1.),(1.,0.768820010203822,
1.),(1.,0.774022074432147,1.),(1.,0.784467204631247,1.),(1.,0.789710609506525,
1.),(1.,0.797506397811445,1.),(1.,0.800093535602747,1.),(1.,0.803945021596591,
1.),(1.,0.805223982229172,1.),(1.,0.807770172561434,1.),(1.,0.80903292134295,
1.),(1.,0.815288089794111,1.),(1.,0.820107499923359,1.),(1.,0.829279685729609,
1.),(1.,0.833632779776828,1.),(1.,0.841777168809211,1.),(1.,0.845568802174027,
1.),(1.,0.849892563199079,1.),(1.,0.850736491533872,1.),(1.,0.851969804909359,
1.),(1.,0.852375793676684,1.),(1.,0.853174988795519,1.),(1.,0.853568068159912,
1.),(1.,0.855500704900974,1.),(1.,0.856941996550435,1.),(1.,0.860944601199298,
1.),(1.,0.863184927882986,1.),(1.,0.866767461005655,1.),(1.,0.868109793594765,
1.),(1.,0.869410481594525,1.),(1.,0.869725148569242,1.),(1.,0.870012890040282,
1.),(1.,0.870078086396283,1.),(1.,0.870128990964309,1.),(1.,0.870138141570321,
1.),(1.,0.870140676091054,1.),(1.,0.870134072965078,1.),(1.,0.870061808448095,
1.),(1.,0.869878426760649,1.),(1.,0.869416656440071,1.),(1.,0.869231611413219,
1.),(1.,0.868907522254946,1.),(1.,0.868791738615037,1.),(1.,0.868544686539316,
1.),(1.,0.868413337134317,1.),(1.,0.867163505604549,1.),(1.,0.865575442228637,
1.),(1.,0.861527724393334,1.),(1.,0.859067845844723,1.),(1.,0.853343564886148,
1.),(1.,0.850078971827717,1.),(1.,0.84598647975218,1.),(1.,0.845525923915504,
1.),(1.,0.844593252383724,1.),(1.,0.84412081177775,1.),(1.,0.842688930644052,
1.),(1.,0.841715504172781,1.),(1.,0.83874140215334,1.),(1.,0.836686926299113,
1.),(1.,0.830328826430023,1.),(1.,0.825830615536545,1.),(1.,0.816419106847222,
1.),(1.,0.81150547118942,1.),(1.,0.805169234170547,1.),(1.,0.803892294076685,
1.),(1.,0.801963643202623,1.),(1.,0.801318553163188,1.),(1.,0.800024181787751,
1.),(1.,0.799374551464301,1.),(1.,0.796123838581708,1.),(1.,0.793511112507122,
1.),(1.,0.785661232785625,1.),(1.,0.780412024366977,1.),(1.,0.770019050951368,
1.),(1.,0.76487497595969,1.),(1.,0.757351702086758,1.),(1.,0.754876228736365,
1.),(1.,0.751227350622943,1.),(1.,0.750021792912108,1.),(1.,0.748231675946372,
1.),(1.,0.747638007827609,1.),(1.,0.746457111568753,1.),(1.,0.745869506104255,
1.),(1.,0.740620037686994,1.),(1.,0.736256100649653,1.),(1.,0.728276221758877,
1.),(1.,0.724660242842317,1.),(1.,0.718324000111086,1.),(1.,0.715603718055959,
1.),(1.,0.712309706535428,1.),(1.,0.711342812014489,1.),(1.,0.710310353740139,
1.),(1.,0.710112755568336,1.),(1.,0.709736703375217,1.),(1.,0.709558069154282,
1.),(1.,0.709050371012769,1.),(1.,0.708749513760786,1.),(1.,0.70795992094024,
1.),(1.,0.707584199551303,1.),(1.,0.707134092959367,1.),(1.,0.70705970821773,
1.),(1.,0.707286843642986,1.),(1.,0.70803921126881,1.),(1.,0.710052147725902,
1.),(1.,0.710870383211632,1.),(1.,0.71207445357331,1.),(1.,0.712324328892365,
1.),(1.,0.712842122035176,1.),(1.,0.713110243316174,1.),(1.,0.713939993830723,
1.),(1.,0.714526359388936,1.),(1.,0.717617638747993,1.),(1.,0.720600584023788,
1.),(1.,0.727424242013839,1.),(1.,0.731264995819141,1.),(1.,0.737553652730096,
1.),(1.,0.739737848764794,1.),(1.,0.742566372039795,1.),(1.,0.74313699147918,
1.),(1.,0.744287770846871,1.),(1.,0.744868257643384,1.),(1.,0.746621209706891,
1.),(1.,0.747803690023989,1.),(1.,0.753778025133493,1.),(1.,0.758754654573864,
1.),(1.,0.768933369155768,1.),(1.,0.774135775395061,1.),(1.,0.781997810487323,
1.),(1.,0.784628358204622,1.),(1.,0.788575987637978,1.),(1.,0.789892170142193,
1.),(1.,0.791865311260895,1.),(1.,0.792522836387841,1.),(1.,0.793837245909085,
1.),(1.,0.794493861510745,1.),(1.,0.800385048001281,1.),(1.,0.80551453306944,
1.),(1.,0.815446188856963,1.),(1.,0.820248709446964,1.),(1.,0.829421742411055,
1.),(1.,0.833792601959078,1.),(1.,0.838919085477355,1.),(1.,0.839927506491091,
1.),(1.,0.841413476855047,1.),(1.,0.841904356336916,1.),(1.,0.842876996646255,
1.),(1.,0.843358860518912,1.),(1.,0.845737639832195,1.),(1.,0.847548776311049,
1.),(1.,0.852696372188048,1.),(1.,0.855747262756165,1.),(1.,0.861029201702321,
1.),(1.,0.863260436478246,1.),(1.,0.865941546711405,1.),(1.,0.86672419811369,
1.),(1.,0.867724144067475,1.),(1.,0.868028445735918,1.),(1.,0.868440362182281,
1.),(1.,0.868570244374482,1.),(1.,0.868753799883508,1.),(1.,0.868813107052922,
1.),(1.,0.868899233803952,1.),(1.,0.868927470387005,1.),(1.,0.868982996012711,
1.),(1.,0.86901031725597,1.),(1.,0.869037098890924,1.)))
REPRESENTATION_ITEM('')
SURFACE()
);
#186=(
BOUNDED_SURFACE()
B_SPLINE_SURFACE(3,2,((#60558,#60559,#60560),(#60561,#60562,#60563),(#60564,
#60565,#60566),(#60567,#60568,#60569),(#60570,#60571,#60572),(#60573,#60574,
#60575),(#60576,#60577,#60578),(#60579,#60580,#60581),(#60582,#60583,#60584),
(#60585,#60586,#60587),(#60588,#60589,#60590),(#60591,#60592,#60593),(#60594,
#60595,#60596),(#60597,#60598,#60599),(#60600,#60601,#60602),(#60603,#60604,
#60605),(#60606,#60607,#60608),(#60609,#60610,#60611),(#60612,#60613,#60614),
(#60615,#60616,#60617),(#60618,#60619,#60620),(#60621,#60622,#60623),(#60624,
#60625,#60626),(#60627,#60628,#60629),(#60630,#60631,#60632),(#60633,#60634,
#60635),(#60636,#60637,#60638),(#60639,#60640,#60641),(#60642,#60643,#60644),
(#60645,#60646,#60647),(#60648,#60649,#60650),(#60651,#60652,#60653),(#60654,
#60655,#60656),(#60657,#60658,#60659),(#60660,#60661,#60662),(#60663,#60664,
#60665),(#60666,#60667,#60668),(#60669,#60670,#60671),(#60672,#60673,#60674),
(#60675,#60676,#60677),(#60678,#60679,#60680),(#60681,#60682,#60683),(#60684,
#60685,#60686),(#60687,#60688,#60689),(#60690,#60691,#60692),(#60693,#60694,
#60695),(#60696,#60697,#60698),(#60699,#60700,#60701),(#60702,#60703,#60704),
(#60705,#60706,#60707)),.UNSPECIFIED.,.F.,.F.,.F.)
B_SPLINE_SURFACE_WITH_KNOTS((4,2,2,2,2,2,2,2,2,2,2,2,2,2,2,2,2,2,2,2,2,
2,2,2,4),(3,3),(-1.43114686768087E-17,0.000151016387548822,0.000302032775097659,
0.000453049162646496,0.000490803259533705,0.000528557356420914,0.000604065550195332,
0.000755081937744169,0.000906098325293005,0.000943852422180215,0.000981606519067424,
0.00105711471284184,0.00120813110039068,0.00135914748793952,0.00143465568171393,
0.00147240977860114,0.00151016387548835,0.00166118026303719,0.00181219665058603,
0.00196321303813486,0.00200096713502207,0.00203872123190928,0.0021142294256837,
0.00226524581323253,0.00241626220078137),(0.,1.),.UNSPECIFIED.)
GEOMETRIC_REPRESENTATION_ITEM()
RATIONAL_B_SPLINE_SURFACE(((1.,0.597614304667196,1.),(1.,0.597614548659316,
1.),(1.,0.597759141644792,1.),(1.,0.598330594325125,1.),(1.,0.598757253597273,
1.),(1.,0.599899281590871,1.),(1.,0.600614622994012,1.),(1.,0.601702544890616,
1.),(1.,0.601930044560374,1.),(1.,0.602404142171764,1.),(1.,0.602650079607565,
1.),(1.,0.603414616291635,1.),(1.,0.603959917797353,1.),(1.,0.605703947627896,
1.),(1.,0.607010476636725,1.),(1.,0.609926264739714,1.),(1.,0.611535514537476,
1.),(1.,0.613752265337911,1.),(1.,0.614205901208812,1.),(1.,0.615134253798264,
1.),(1.,0.61560958725321,1.),(1.,0.617063403759804,1.),(1.,0.618067502552084,
1.),(1.,0.621185868361561,1.),(1.,0.623406027602217,1.),(1.,0.628140854568891,
1.),(1.,0.63065552053793,1.),(1.,0.634661693683576,1.),(1.,0.636036157866121,
1.),(1.,0.638158552325295,1.),(1.,0.638876846031255,1.),(1.,0.640330763885221,
1.),(1.,0.641065138363023,1.),(1.,0.644774107930351,1.),(1.,0.647859895490701,
1.),(1.,0.654270816871591,1.),(1.,0.65759594902533,1.),(1.,0.664490189617747,
1.),(1.,0.668059281341528,1.),(1.,0.672677743668185,1.),(1.,0.673609777828573,
1.),(1.,0.675481455951091,1.),(1.,0.676422055868733,1.),(1.,0.679258012829202,
1.),(1.,0.681167525351118,1.),(1.,0.686951752951439,1.),(1.,0.690882126194853,
1.),(1.,0.698887084712717,1.),(1.,0.702961683112489,1.),(1.,0.707106781186548,
1.)))
REPRESENTATION_ITEM('')
SURFACE()
);
#187=(
BOUNDED_SURFACE()
B_SPLINE_SURFACE(3,2,((#60738,#60739,#60740),(#60741,#60742,#60743),(#60744,
#60745,#60746),(#60747,#60748,#60749),(#60750,#60751,#60752),(#60753,#60754,
#60755),(#60756,#60757,#60758),(#60759,#60760,#60761),(#60762,#60763,#60764),
(#60765,#60766,#60767),(#60768,#60769,#60770),(#60771,#60772,#60773),(#60774,
#60775,#60776),(#60777,#60778,#60779),(#60780,#60781,#60782),(#60783,#60784,
#60785),(#60786,#60787,#60788),(#60789,#60790,#60791),(#60792,#60793,#60794),
(#60795,#60796,#60797),(#60798,#60799,#60800),(#60801,#60802,#60803),(#60804,
#60805,#60806),(#60807,#60808,#60809),(#60810,#60811,#60812),(#60813,#60814,
#60815),(#60816,#60817,#60818),(#60819,#60820,#60821),(#60822,#60823,#60824),
(#60825,#60826,#60827),(#60828,#60829,#60830),(#60831,#60832,#60833),(#60834,
#60835,#60836),(#60837,#60838,#60839),(#60840,#60841,#60842),(#60843,#60844,
#60845),(#60846,#60847,#60848),(#60849,#60850,#60851),(#60852,#60853,#60854),
(#60855,#60856,#60857),(#60858,#60859,#60860),(#60861,#60862,#60863),(#60864,
#60865,#60866),(#60867,#60868,#60869),(#60870,#60871,#60872),(#60873,#60874,
#60875),(#60876,#60877,#60878),(#60879,#60880,#60881),(#60882,#60883,#60884),
(#60885,#60886,#60887),(#60888,#60889,#60890),(#60891,#60892,#60893),(#60894,
#60895,#60896),(#60897,#60898,#60899),(#60900,#60901,#60902),(#60903,#60904,
#60905),(#60906,#60907,#60908),(#60909,#60910,#60911),(#60912,#60913,#60914),
(#60915,#60916,#60917),(#60918,#60919,#60920),(#60921,#60922,#60923),(#60924,
#60925,#60926),(#60927,#60928,#60929),(#60930,#60931,#60932),(#60933,#60934,
#60935),(#60936,#60937,#60938),(#60939,#60940,#60941),(#60942,#60943,#60944),
(#60945,#60946,#60947),(#60948,#60949,#60950),(#60951,#60952,#60953),(#60954,
#60955,#60956),(#60957,#60958,#60959),(#60960,#60961,#60962),(#60963,#60964,
#60965),(#60966,#60967,#60968),(#60969,#60970,#60971),(#60972,#60973,#60974),
(#60975,#60976,#60977),(#60978,#60979,#60980),(#60981,#60982,#60983),(#60984,
#60985,#60986),(#60987,#60988,#60989),(#60990,#60991,#60992),(#60993,#60994,
#60995),(#60996,#60997,#60998),(#60999,#61000,#61001),(#61002,#61003,#61004),
(#61005,#61006,#61007),(#61008,#61009,#61010),(#61011,#61012,#61013),(#61014,
#61015,#61016),(#61017,#61018,#61019),(#61020,#61021,#61022),(#61023,#61024,
#61025),(#61026,#61027,#61028),(#61029,#61030,#61031),(#61032,#61033,#61034),
(#61035,#61036,#61037),(#61038,#61039,#61040),(#61041,#61042,#61043),(#61044,
#61045,#61046),(#61047,#61048,#61049),(#61050,#61051,#61052),(#61053,#61054,
#61055),(#61056,#61057,#61058),(#61059,#61060,#61061),(#61062,#61063,#61064),
(#61065,#61066,#61067),(#61068,#61069,#61070),(#61071,#61072,#61073),(#61074,
#61075,#61076),(#61077,#61078,#61079),(#61080,#61081,#61082),(#61083,#61084,
#61085),(#61086,#61087,#61088),(#61089,#61090,#61091),(#61092,#61093,#61094),
(#61095,#61096,#61097),(#61098,#61099,#61100),(#61101,#61102,#61103),(#61104,
#61105,#61106),(#61107,#61108,#61109),(#61110,#61111,#61112),(#61113,#61114,
#61115),(#61116,#61117,#61118),(#61119,#61120,#61121),(#61122,#61123,#61124),
(#61125,#61126,#61127),(#61128,#61129,#61130),(#61131,#61132,#61133),(#61134,
#61135,#61136),(#61137,#61138,#61139),(#61140,#61141,#61142),(#61143,#61144,
#61145),(#61146,#61147,#61148),(#61149,#61150,#61151),(#61152,#61153,#61154),
(#61155,#61156,#61157),(#61158,#61159,#61160),(#61161,#61162,#61163),(#61164,
#61165,#61166),(#61167,#61168,#61169),(#61170,#61171,#61172),(#61173,#61174,
#61175),(#61176,#61177,#61178),(#61179,#61180,#61181),(#61182,#61183,#61184),
(#61185,#61186,#61187),(#61188,#61189,#61190),(#61191,#61192,#61193),(#61194,
#61195,#61196),(#61197,#61198,#61199),(#61200,#61201,#61202),(#61203,#61204,
#61205),(#61206,#61207,#61208),(#61209,#61210,#61211),(#61212,#61213,#61214),
(#61215,#61216,#61217),(#61218,#61219,#61220),(#61221,#61222,#61223),(#61224,
#61225,#61226),(#61227,#61228,#61229),(#61230,#61231,#61232),(#61233,#61234,
#61235),(#61236,#61237,#61238),(#61239,#61240,#61241),(#61242,#61243,#61244),
(#61245,#61246,#61247),(#61248,#61249,#61250),(#61251,#61252,#61253),(#61254,
#61255,#61256),(#61257,#61258,#61259),(#61260,#61261,#61262),(#61263,#61264,
#61265),(#61266,#61267,#61268),(#61269,#61270,#61271),(#61272,#61273,#61274),
(#61275,#61276,#61277),(#61278,#61279,#61280),(#61281,#61282,#61283),(#61284,
#61285,#61286),(#61287,#61288,#61289),(#61290,#61291,#61292),(#61293,#61294,
#61295),(#61296,#61297,#61298),(#61299,#61300,#61301),(#61302,#61303,#61304),
(#61305,#61306,#61307),(#61308,#61309,#61310),(#61311,#61312,#61313),(#61314,
#61315,#61316),(#61317,#61318,#61319),(#61320,#61321,#61322),(#61323,#61324,
#61325),(#61326,#61327,#61328),(#61329,#61330,#61331),(#61332,#61333,#61334),
(#61335,#61336,#61337),(#61338,#61339,#61340),(#61341,#61342,#61343),(#61344,
#61345,#61346),(#61347,#61348,#61349),(#61350,#61351,#61352),(#61353,#61354,
#61355),(#61356,#61357,#61358),(#61359,#61360,#61361),(#61362,#61363,#61364),
(#61365,#61366,#61367),(#61368,#61369,#61370),(#61371,#61372,#61373),(#61374,
#61375,#61376),(#61377,#61378,#61379),(#61380,#61381,#61382),(#61383,#61384,
#61385),(#61386,#61387,#61388),(#61389,#61390,#61391),(#61392,#61393,#61394),
(#61395,#61396,#61397),(#61398,#61399,#61400),(#61401,#61402,#61403),(#61404,
#61405,#61406),(#61407,#61408,#61409),(#61410,#61411,#61412),(#61413,#61414,
#61415),(#61416,#61417,#61418),(#61419,#61420,#61421),(#61422,#61423,#61424),
(#61425,#61426,#61427),(#61428,#61429,#61430),(#61431,#61432,#61433),(#61434,
#61435,#61436),(#61437,#61438,#61439),(#61440,#61441,#61442),(#61443,#61444,
#61445),(#61446,#61447,#61448),(#61449,#61450,#61451),(#61452,#61453,#61454),
(#61455,#61456,#61457),(#61458,#61459,#61460),(#61461,#61462,#61463),(#61464,
#61465,#61466),(#61467,#61468,#61469),(#61470,#61471,#61472),(#61473,#61474,
#61475),(#61476,#61477,#61478),(#61479,#61480,#61481),(#61482,#61483,#61484),
(#61485,#61486,#61487),(#61488,#61489,#61490),(#61491,#61492,#61493),(#61494,
#61495,#61496),(#61497,#61498,#61499),(#61500,#61501,#61502),(#61503,#61504,
#61505),(#61506,#61507,#61508),(#61509,#61510,#61511),(#61512,#61513,#61514),
(#61515,#61516,#61517),(#61518,#61519,#61520),(#61521,#61522,#61523),(#61524,
#61525,#61526),(#61527,#61528,#61529)),.UNSPECIFIED.,.F.,.F.,.F.)
B_SPLINE_SURFACE_WITH_KNOTS((4,2,2,2,2,2,2,2,2,2,2,2,2,2,2,2,2,2,2,2,2,
2,2,2,2,2,2,2,2,2,2,2,2,2,2,2,2,2,2,2,2,2,2,2,2,2,2,2,2,2,2,2,2,2,2,2,2,
2,2,2,2,2,2,2,2,2,2,2,2,2,2,2,2,2,2,2,2,2,2,2,2,2,2,2,2,2,2,2,2,2,2,2,2,
2,2,2,2,2,2,2,2,2,2,2,2,2,2,2,2,2,2,2,2,2,2,2,2,2,2,2,2,2,2,2,2,2,2,2,2,
2,2,4),(3,3),(0.00550389531139888,0.00574810157344769,0.0058702047044721,
0.0059923078354965,0.00648072035959412,0.00745754540778936,0.0084343704559846,
0.00892278298008221,0.00916698924213102,0.00928909237315543,0.00941119550417983,
0.0103880205523751,0.0113648456005703,0.0118532581246679,0.0123416706487656,
0.0125858769108144,0.0127079800418388,0.0128300831728632,0.0133184956969608,
0.014295320745156,0.0152721457933513,0.0155163520554001,0.0156384551864245,
0.0157605583174489,0.0162489708415465,0.0172257958897417,0.018202620937937,
0.0184468271999858,0.0185689303310102,0.0186910334620346,0.0191794459861322,
0.0201562710343275,0.0211330960825227,0.0213773023445715,0.0214994054755959,
0.0216215086066203,0.0221099211307179,0.0230867461789132,0.0240635712271084,
0.024551983751206,0.0246740868822304,0.0247961900132548,0.0250403962753037,
0.0260172213234989,0.0269940463716941,0.0279708714198894,0.0282150776819382,
0.0283371808129626,0.028459283943987,0.0289476964680846,0.0299245215162798,
0.0309013465644751,0.0313897590885727,0.0316339653506215,0.0317560684816459,
0.0318781716126703,0.0323665841367679,0.0328549966608656,0.0333434091849632,
0.0338318217090608,0.0343202342331584,0.0345644404952072,0.0346865436262316,
0.034808646757256,0.0352970592813537,0.0357854718054513,0.0367622968536465,
0.0377391219018418,0.0379833281638906,0.038105431294915,0.0382275344259394,
0.038715946950037,0.0396927719982322,0.0406695970464275,0.0411580095705251,
0.0414022158325739,0.0415243189635983,0.0416464220946227,0.0426232471428179,
0.0436000721910132,0.0440884847151108,0.0445768972392084,0.045065309763306,
0.0453095160253549,0.0455537222874037,0.0465305473355989,0.0475073723837941,
0.047751578645843,0.0478736817768674,0.0479957849078918,0.0484841974319894,
0.0494610224801846,0.0504378475283799,0.0506820537904287,0.0508041569214531,
0.0509262600524775,0.0514146725765751,0.0523914976247703,0.0533683226729656,
0.0536125289350144,0.0537346320660388,0.0538567351970632,0.0543451477211608,
0.055321972769356,0.0562987978175513,0.0567872103416489,0.0569093134726733,
0.0570314166036977,0.0572756228657465,0.0582524479139418,0.059229272962137,
0.0602060980103322,0.0604503042723811,0.0605724074034055,0.0606945105344299,
0.0611829230585275,0.0621597481067227,0.063136573154918,0.0636249856790156,
0.0638691919410644,0.0639302435065766,0.0639912950720888,0.0641133982031132,
0.0646018107272108,0.0650902232513084,0.0655786357754061,0.0660670482995037,
0.0665554608236013,0.0667996670856501,0.0669217702166745,0.0670438733476989,
0.0680206983958942),(-4.72906511448186E-7,1.),.UNSPECIFIED.)
GEOMETRIC_REPRESENTATION_ITEM()
RATIONAL_B_SPLINE_SURFACE(((1.00000023498091,0.751556694153118,1.),(1.00000023378176,
0.752824548397775,1.),(1.00000023256666,0.754109265472953,1.),(1.00000023072186,
0.756059754072068,1.),(1.00000023010324,0.756713819297174,1.),(1.0000002288589,
0.758029444458224,1.),(1.000000228233,0.75869120103434,1.),(1.00000022508853,
0.76201582674644,1.),(1.00000022253726,0.76471326317563,1.),(1.00000021480751,
0.77288585853503,1.),(1.00000020955378,0.778440589326931,1.),(1.00000019899112,
0.789608400404832,1.),(1.00000019368186,0.795221829049161,1.),(1.00000018577219,
0.803584653975839,1.),(1.00000018314456,0.806362824271203,1.),(1.00000017922784,
0.810503941986009,1.),(1.00000017792638,0.811879961599245,1.),(1.00000017598177,
0.813935983448259,1.),(1.0000001753352,0.814619594228044,1.),(1.00000017404777,
0.815980786342396,1.),(1.00000017340658,0.816658712809378,1.),(1.00000016765943,
0.822735126197709,1.),(1.0000001627188,0.827958812159829,1.),(1.00000015326503,
0.837954194734113,1.),(1.00000014875159,0.842726222382481,1.),(1.00000014236885,
0.849474639737199,1.),(1.00000014030585,0.851655826992419,1.),(1.00000013632082,
0.855869168446521,1.),(1.00000013439877,0.857901334912284,1.),(1.00000013163084,
0.860827846311646,1.),(1.00000013072739,0.861783052685079,1.),(1.00000012940227,
0.863184085582916,1.),(1.00000012896558,0.863645799803543,1.),(1.00000012810242,
0.864558404613122,1.),(1.00000012767567,0.865009605497141,1.),(1.00000012557194,
0.867233865854088,1.),(1.00000012398733,0.868909259809825,1.),(1.00000011953754,
0.873613984612272,1.),(1.00000011697604,0.876322231319804,1.),(1.00000011271749,
0.880824759327638,1.),(1.00000011102027,0.882619221541114,1.),(1.00000010948111,
0.884246560006968,1.),(1.00000010920244,0.884541198563755,1.),(1.00000010882909,
0.884935937378963,1.),(1.00000010871208,0.885059646520894,1.),(1.00000010849312,
0.885291153381852,1.),(1.00000010839109,0.88539903398853,1.),(1.00000010792017,
0.885896934847654,1.),(1.00000010766867,0.886162837228243,1.),(1.00000010728335,
0.886570231636448,1.),(1.00000010751835,0.886321775490983,1.),(1.00000010894598,
0.884812349368159,1.),(1.00000011013867,0.883551331717548,1.),(1.00000011221839,
0.881352460936778,1.),(1.0000001126638,0.88088153148373,1.),(1.000000113376,
0.880128522727162,1.),(1.00000011362075,0.879869750411651,1.),(1.00000011412494,
0.879336683160622,1.),(1.00000011438458,0.879062164951402,1.),(1.00000011571638,
0.877654060682486,1.),(1.0000001168888,0.876414476784003,1.),(1.00000012070877,
0.872375657113504,1.),(1.00000012365859,0.869256837455263,1.),(1.0000001302817,
0.86225427633696,1.),(1.00000013395525,0.858370260865121,1.),(1.0000001389552,
0.853083860085661,1.),(1.00000013997561,0.852004991745369,1.),(1.00000014153605,
0.850355143413675,1.),(1.00000014206137,0.849799736088604,1.),(1.00000014311937,
0.848681114911057,1.),(1.00000014365233,0.848117621698517,1.),(1.00000014633638,
0.845279799797655,1.),(1.0000001485452,0.842944430835434,1.),(1.00000015533688,
0.835763650211785,1.),(1.00000016008491,0.830743595177666,1.),(1.0000001699216,
0.820343351831782,1.),(1.00000017501058,0.814962810757057,1.),(1.0000001828229,
0.806702912434936,1.),(1.00000018545676,0.803918154992135,1.),(1.00000018877756,
0.800407100997016,1.),(1.00000018944312,0.799703414672647,1.),(1.00000019077364,
0.798296664875502,1.),(1.00000019143901,0.797593180627382,1.),(1.00000019343504,
0.795482793926751,1.),(1.00000019476564,0.794075956555709,1.),(1.00000020141324,
0.78704750614951,1.),(1.00000020671441,0.781442625039865,1.),(1.00000021714846,
0.770410799011106,1.),(1.00000022228161,0.764983560872734,1.),(1.00000023222946,
0.754465779333137,1.),(1.00000023704448,0.749374905591535,1.),(1.00000024275479,
0.743337436815082,1.),(1.00000024388136,0.742146327927527,1.),(1.00000024554567,
0.740386673133335,1.),(1.00000024609518,0.739805676275109,1.),(1.00000024718247,
0.738656092994039,1.),(1.0000002477204,0.738087342446234,1.),(1.00000025038083,
0.735274497907314,1.),(1.00000025241562,0.73312312519276,1.),(1.00000025821379,
0.726992773429071,1.),(1.00000026167096,0.723337538949804,1.),(1.00000026763152,
0.717035483201795,1.),(1.00000027013488,0.714388705392069,1.),(1.00000027307154,
0.711283802444097,1.),(1.00000027391403,0.710393041672387,1.),(1.00000027496038,
0.70928675234185,1.),(1.00000027527292,0.708956297159223,1.),(1.0000002756858,
0.708519762422626,1.),(1.00000027581414,0.708384075000737,1.),(1.00000027605176,
0.708132837756234,1.),(1.0000002761608,0.708017549283914,1.),(1.00000027665727,
0.707492635552901,1.),(1.00000027689845,0.707237643899567,1.),(1.00000027707247,
0.707053652944908,1.),(1.00000027700532,0.707124653493474,1.),(1.00000027656751,
0.707587539289571,1.),(1.00000027619686,0.707979423441002,1.),(1.00000027515804,
0.709077765452766,1.),(1.00000027448986,0.709784221424154,1.),(1.00000027286305,
0.711504238909358,1.),(1.00000027190441,0.71251779792269,1.),(1.00000027025468,
0.714262047196191,1.),(1.00000026966948,0.714880773824933,1.),(1.00000026873957,
0.715863955555072,1.),(1.00000026842092,0.716200864287518,1.),(1.00000026776639,
0.716892893458133,1.),(1.00000026743032,0.717248218521567,1.),(1.00000026570947,
0.719067653552063,1.),(1.00000026420991,0.720653126054481,1.),(1.00000026098872,
0.724058862455822,1.),(1.00000025926709,0.725879130357689,1.),(1.00000025380292,
0.731656351861655,1.),(1.00000024976157,0.73592923685194,1.),(1.00000024105014,
0.745139754107446,1.),(1.00000023637996,0.750077498999356,1.),(1.00000023024597,
0.756562909310098,1.),(1.00000022900433,0.757875682834899,1.),(1.00000022712135,
0.759866544520447,1.),(1.00000022649027,0.760533782306009,1.),(1.00000022522155,
0.761875189848965,1.),(1.00000022458429,0.762548959437356,1.),(1.00000022139052,
0.765925697624077,1.),(1.00000021880595,0.768658341855167,1.),(1.00000021099365,
0.776918218582894,1.),(1.00000020570797,0.782506721948014,1.),(1.00000019512297,
0.793698161123683,1.),(1.0000001898233,0.799301448123694,1.),(1.00000018195664,
0.807618799497514,1.),(1.00000017934813,0.810376757675791,1.),(1.00000017546704,
0.81448020734433,1.),(1.00000017417861,0.815842445219629,1.),(1.00000017225527,
0.817875977839375,1.),(1.00000017161558,0.818552316235376,1.),(1.00000017034262,
0.819898209492926,1.),(1.00000016970896,0.82056816809445,1.),(1.00000016403231,
0.826570043806966,1.),(1.0000001591733,0.831707434235114,1.),(1.00000014991731,
0.841493708708982,1.),(1.00000014552003,0.846142917478774,1.),(1.00000013933591,
0.852681332968294,1.),(1.0000001373432,0.854788213702908,1.),(1.00000013350673,
0.858844481985634,1.),(1.00000013166296,0.860793881731502,1.),(1.00000012813688,
0.864521979247798,1.),(1.00000012645455,0.866300691342452,1.),(1.00000012406244,
0.868829842162124,1.),(1.00000012329029,0.869646238009235,1.),(1.00000012179807,
0.87122394532148,1.),(1.00000012107784,0.871985436590129,1.),(1.00000011760779,
0.875654291255009,1.),(1.00000011525083,0.87814628298712,1.),(1.00000011142444,
0.882191896881282,1.),(1.00000010995485,0.883745677395368,1.),(1.00000010871133,
0.885060444051895,1.),(1.00000010849234,0.885291984185686,1.),(1.00000010820926,
0.885591273045841,1.),(1.00000010812248,0.885683031852686,1.),(1.00000010796419,
0.885850383459224,1.),(1.00000010789265,0.885926031072474,1.),(1.00000010757428,
0.886262631448316,1.),(1.00000010744539,0.886398908559158,1.),(1.00000010742813,
0.886417163206912,1.),(1.0000001079088,0.885908946265843,1.),(1.00000010982151,
0.88388666077102,1.),(1.0000001112536,0.882372526971855,1.),(1.00000011362453,
0.879865758662412,1.),(1.00000011412778,0.879333674429881,1.),(1.00000011492607,
0.878489652629009,1.),(1.0000001151994,0.87820066249251,1.),(1.0000001157605,
0.877607413101931,1.),(1.00000011604836,0.877303065972634,1.),(1.00000011751912,
0.875748046563914,1.),(1.00000011879965,0.87439415067658,1.),(1.00000012293461,
0.870022288419149,1.),(1.00000012608197,0.866694610164977,1.),(1.00000013307372,
0.859302298416578,1.),(1.00000013691837,0.855237378460135,1.),(1.00000014211423,
0.849743845714332,1.),(1.00000014317292,0.848624503463328,1.),(1.0000001447894,
0.846915410070114,1.),(1.00000014533277,0.846340908054068,1.),(1.00000014642633,
0.845184698703843,1.),(1.0000001469768,0.844602685849943,1.),(1.00000014974713,
0.841673639940311,1.),(1.00000015202083,0.839269684772021,1.),(1.00000015899447,
0.831896507955678,1.),(1.00000016384702,0.826765951203782,1.),(1.00000017385695,
0.816182532882831,1.),(1.00000017901468,0.810729315211788,1.),(1.00000018690038,
0.80239183329862,1.),(1.00000018955373,0.799586467378934,1.),(1.00000019289228,
0.796056651380399,1.),(1.00000019356127,0.795349331223752,1.),(1.00000019489798,
0.793936034393844,1.),(1.00000019556608,0.793229659050175,1.),(1.00000019756922,
0.791111755587851,1.),(1.00000019890311,0.789701448963109,1.),(1.0000002055597,
0.782663492366119,1.),(1.00000021084436,0.777076066790433,1.),(1.00000022119435,
0.766133106017418,1.),(1.00000022625995,0.7607772915656,1.),(1.00000023601756,
0.750460654634383,1.),(1.00000024070987,0.745499520465223,1.),(1.00000024622976,
0.739663381402246,1.),(1.0000002473164,0.738514495390714,1.),(1.00000024891798,
0.736821157275602,1.),(1.00000024944697,0.736261859406495,1.),(1.00000025049176,
0.73515720721303,1.),(1.00000025100799,0.73461140273185,1.),(1.00000025355765,
0.731915666474236,1.),(1.00000025549664,0.729865595746991,1.),(1.00000026098678,
0.724060911408639,1.),(1.00000026421107,0.720651898486557,1.),(1.00000026965822,
0.714892677044352,1.),(1.00000027188102,0.712542530134079,1.),(1.00000027436892,
0.709912091354844,1.),(1.0000002750572,0.709184377859772,1.),(1.00000027586651,
0.708328704157888,1.),(1.0000002760991,0.708082793128139,1.),(1.00000027634216,
0.707825802489092,1.),(1.00000027638839,0.707776924211404,1.),(1.00000027647605,
0.707684238567988,1.),(1.00000027651752,0.707640402018307,1.),(1.00000027663423,
0.707517005252166,1.),(1.00000027670223,0.707445102385259,1.),(1.00000027699347,
0.707137182867287,1.),(1.00000027707025,0.707055995209309,1.),(1.00000027691727,
0.707217741884412,1.),(1.0000002766875,0.707460675529496,1.),(1.00000027592831,
0.708263359580143,1.),(1.0000002753989,0.708823108402302,1.),(1.00000027404836,
0.710251021221229,1.),(1.00000027322724,0.711119182945965,1.),(1.00000027130223,
0.713154483324201,1.),(1.00000027019833,0.71432161923774,1.),(1.00000026833779,
0.716288757540562,1.),(1.0000002676835,0.716980535502155,1.),(1.00000026665187,
0.718071263738537,1.),(1.00000026629963,0.71844368295856,1.),(1.00000026557859,
0.719206030037194,1.),(1.00000026520954,0.719596229989639,1.),(1.0000002618201,
0.723179856882723,1.),(1.000000258339,0.726860386021971,1.),(1.00000025448214,
0.730938217147024,1.)))
REPRESENTATION_ITEM('')
SURFACE()
);
#188=(
BOUNDED_SURFACE()
B_SPLINE_SURFACE(3,2,((#61530,#61531,#61532),(#61533,#61534,#61535),(#61536,
#61537,#61538),(#61539,#61540,#61541),(#61542,#61543,#61544),(#61545,#61546,
#61547),(#61548,#61549,#61550),(#61551,#61552,#61553),(#61554,#61555,#61556),
(#61557,#61558,#61559),(#61560,#61561,#61562),(#61563,#61564,#61565),(#61566,
#61567,#61568),(#61569,#61570,#61571),(#61572,#61573,#61574),(#61575,#61576,
#61577),(#61578,#61579,#61580),(#61581,#61582,#61583),(#61584,#61585,#61586),
(#61587,#61588,#61589),(#61590,#61591,#61592),(#61593,#61594,#61595),(#61596,
#61597,#61598),(#61599,#61600,#61601),(#61602,#61603,#61604),(#61605,#61606,
#61607),(#61608,#61609,#61610),(#61611,#61612,#61613),(#61614,#61615,#61616),
(#61617,#61618,#61619),(#61620,#61621,#61622),(#61623,#61624,#61625),(#61626,
#61627,#61628),(#61629,#61630,#61631),(#61632,#61633,#61634),(#61635,#61636,
#61637),(#61638,#61639,#61640),(#61641,#61642,#61643),(#61644,#61645,#61646),
(#61647,#61648,#61649),(#61650,#61651,#61652),(#61653,#61654,#61655),(#61656,
#61657,#61658),(#61659,#61660,#61661),(#61662,#61663,#61664),(#61665,#61666,
#61667),(#61668,#61669,#61670),(#61671,#61672,#61673),(#61674,#61675,#61676),
(#61677,#61678,#61679),(#61680,#61681,#61682),(#61683,#61684,#61685),(#61686,
#61687,#61688),(#61689,#61690,#61691),(#61692,#61693,#61694),(#61695,#61696,
#61697),(#61698,#61699,#61700),(#61701,#61702,#61703),(#61704,#61705,#61706),
(#61707,#61708,#61709),(#61710,#61711,#61712),(#61713,#61714,#61715),(#61716,
#61717,#61718),(#61719,#61720,#61721),(#61722,#61723,#61724),(#61725,#61726,
#61727),(#61728,#61729,#61730),(#61731,#61732,#61733),(#61734,#61735,#61736),
(#61737,#61738,#61739),(#61740,#61741,#61742),(#61743,#61744,#61745),(#61746,
#61747,#61748),(#61749,#61750,#61751),(#61752,#61753,#61754),(#61755,#61756,
#61757),(#61758,#61759,#61760),(#61761,#61762,#61763),(#61764,#61765,#61766),
(#61767,#61768,#61769),(#61770,#61771,#61772),(#61773,#61774,#61775),(#61776,
#61777,#61778),(#61779,#61780,#61781),(#61782,#61783,#61784),(#61785,#61786,
#61787),(#61788,#61789,#61790),(#61791,#61792,#61793),(#61794,#61795,#61796),
(#61797,#61798,#61799),(#61800,#61801,#61802),(#61803,#61804,#61805),(#61806,
#61807,#61808),(#61809,#61810,#61811),(#61812,#61813,#61814),(#61815,#61816,
#61817),(#61818,#61819,#61820),(#61821,#61822,#61823),(#61824,#61825,#61826),
(#61827,#61828,#61829),(#61830,#61831,#61832),(#61833,#61834,#61835),(#61836,
#61837,#61838),(#61839,#61840,#61841),(#61842,#61843,#61844),(#61845,#61846,
#61847),(#61848,#61849,#61850),(#61851,#61852,#61853),(#61854,#61855,#61856),
(#61857,#61858,#61859),(#61860,#61861,#61862),(#61863,#61864,#61865),(#61866,
#61867,#61868),(#61869,#61870,#61871),(#61872,#61873,#61874),(#61875,#61876,
#61877),(#61878,#61879,#61880),(#61881,#61882,#61883)),.UNSPECIFIED.,.F.,
 .F.,.F.)
B_SPLINE_SURFACE_WITH_KNOTS((4,2,2,2,2,2,2,2,2,2,2,2,2,2,2,2,2,2,2,2,2,
2,2,2,2,2,2,2,2,2,2,2,2,2,2,2,2,2,2,2,2,2,2,2,2,2,2,2,2,2,2,2,2,2,2,2,2,
2,4),(3,3),(0.00917852058677495,0.00979162970055923,0.0104047388143435,
0.0110178479281278,0.0113244024850199,0.011477679763466,0.0116309570419121,
0.0122440661556963,0.0128571752694806,0.0134702843832649,0.0136235616617109,
0.013700200300934,0.013776838940157,0.0140833934970491,0.0146965026108334,
0.0150030571677256,0.0153096117246177,0.0156161662815098,0.0157694435599559,
0.015922720838402,0.0162292753952941,0.0165358299521862,0.0168423845090784,
0.0171489390659705,0.0174554936228627,0.0175321322620857,0.0176087709013087,
0.0177620481797548,0.0180686027366469,0.0183751572935391,0.0189882664073233,
0.0191415436857694,0.0192181823249925,0.0192948209642155,0.0196013755211076,
0.0202144846348919,0.0208275937486762,0.0209808710271222,0.0211341483055683,
0.0214407028624604,0.0217472574193526,0.0218238960585756,0.0219005346977986,
0.0220538119762447,0.022666921090029,0.0232800302038133,0.0238931393175975,
0.0245062484313818,0.024812802988274,0.02496608026672,0.0251193575451661,
0.0257324666589504,0.0263455757727346,0.0269586848865189,0.0275717940003032,
0.0278783485571953,0.0280316258356414,0.0281849031140875,0.0287980122278717),
(0.,1.),.UNSPECIFIED.)
GEOMETRIC_REPRESENTATION_ITEM()
RATIONAL_B_SPLINE_SURFACE(((1.,0.695382524078308,1.),(1.,0.690973084826369,
1.),(1.,0.686397501074747,1.),(1.,0.676941961810577,1.),(1.,0.672061709768397,
1.),(1.,0.66203086632443,1.),(1.,0.656880116106326,1.),(1.,0.64898582257856,
1.),(1.,0.646326468817071,1.),(1.,0.642301097907339,1.),(1.,0.640953260446955,
1.),(1.,0.638246544124457,1.),(1.,0.636892439350123,1.),(1.,0.630130032747308,
1.),(1.,0.624736470834729,1.),(1.,0.614080890649201,1.),(1.,0.608818559901416,
1.),(1.,0.598549562946725,1.),(1.,0.593542431435649,1.),(1.,0.587544087100298,
1.),(1.,0.586357558941886,1.),(1.,0.58459974489545,1.),(1.,0.584017471589961,
1.),(1.,0.58286065407134,1.),(1.,0.582285714201984,1.),(1.,0.579441033435682,
1.),(1.,0.577255035039604,1.),(1.,0.57099407208922,1.),(1.,0.567215424254483,
1.),(1.,0.562263998546966,1.),(1.,0.56073312267832,1.),(1.,0.557933367235571,
1.),(1.,0.556664483779403,1.),(1.,0.554413089085532,1.),(1.,0.55343057236855,
1.),(1.,0.552191143920635,1.),(1.,0.551817026223423,1.),(1.,0.551150559711954,
1.),(1.,0.550860123121361,1.),(1.,0.550117918145604,1.),(1.,0.54979527502456,
1.),(1.,0.549497678024855,1.),(1.,0.54952272712658,1.),(1.,0.549923199329552,
1.),(1.,0.550298623229659,1.),(1.,0.551401777926261,1.),(1.,0.552129507376673,
1.),(1.,0.553938461937551,1.),(1.,0.555019683583193,1.),(1.,0.55659246824619,
1.),(1.,0.556918368573493,1.),(1.,0.557590793133884,1.),(1.,0.557937171309798,
1.),(1.,0.559006327612528,1.),(1.,0.559759125759416,1.),(1.,0.56213386569043,
1.),(1.,0.563872123771208,1.),(1.,0.567639632538003,1.),(1.,0.56966888369193,
1.),(1.,0.576165737003702,1.),(1.,0.581041953914996,1.),(1.,0.587734307209788,
1.),(1.,0.589102670011644,1.),(1.,0.591198589894367,1.),(1.,0.591904329882334,
1.),(1.,0.593326306107057,1.),(1.,0.59404298699,1.),(1.,0.597653969719517,
1.),(1.,0.600630906054337,1.),(1.,0.609794672912413,1.),(1.,0.616213457755282,
1.),(1.,0.629529817492585,1.),(1.,0.636427647260283,1.),(1.,0.64528002230528,
1.),(1.,0.647062576663052,1.),(1.,0.650647123113913,1.),(1.,0.652446504467237,
1.),(1.,0.657863706040612,1.),(1.,0.661500537891968,1.),(1.,0.668814039957785,
1.),(1.,0.672490718153945,1.),(1.,0.677105532455178,1.),(1.,0.678029446716273,
1.),(1.,0.679879041255836,1.),(1.,0.6808048791055,1.),(1.,0.683580788138606,
1.),(1.,0.685430538496766,1.),(1.,0.694672821737992,1.),(1.,0.702045375777937,
1.),(1.,0.716701955734308,1.),(1.,0.723986149925766,1.),(1.,0.738431955919895,
1.),(1.,0.745593682702893,1.),(1.,0.759767797075294,1.),(1.,0.766780270092341,
1.),(1.,0.777170190252166,1.),(1.,0.780612058728018,1.),(1.,0.785740760463396,
1.),(1.,0.787445924233964,1.),(1.,0.790834278540273,1.),(1.,0.792518300408504,
1.),(1.,0.800887468641132,1.),(1.,0.807419900116371,1.),(1.,0.820153190581628,
1.),(1.,0.826354102318175,1.),(1.,0.838415054767577,1.),(1.,0.844275167314104,
1.),(1.,0.855639785590181,1.),(1.,0.86114440303444,1.),(1.,0.869117500840641,
1.),(1.,0.871727822221485,1.),(1.,0.875569253717761,1.),(1.,0.876838215848048,
1.),(1.,0.879341120217273,1.),(1.,0.880576146721508,1.),(1.,0.886668389923952,
1.),(1.,0.891277339697025,1.),(1.,0.895607410402154,1.)))
REPRESENTATION_ITEM('')
SURFACE()
);
#189=(
BOUNDED_SURFACE()
B_SPLINE_SURFACE(3,2,((#61911,#61912,#61913),(#61914,#61915,#61916),(#61917,
#61918,#61919),(#61920,#61921,#61922),(#61923,#61924,#61925),(#61926,#61927,
#61928),(#61929,#61930,#61931),(#61932,#61933,#61934),(#61935,#61936,#61937),
(#61938,#61939,#61940),(#61941,#61942,#61943),(#61944,#61945,#61946),(#61947,
#61948,#61949),(#61950,#61951,#61952),(#61953,#61954,#61955),(#61956,#61957,
#61958),(#61959,#61960,#61961),(#61962,#61963,#61964),(#61965,#61966,#61967),
(#61968,#61969,#61970),(#61971,#61972,#61973),(#61974,#61975,#61976),(#61977,
#61978,#61979),(#61980,#61981,#61982),(#61983,#61984,#61985),(#61986,#61987,
#61988),(#61989,#61990,#61991),(#61992,#61993,#61994),(#61995,#61996,#61997),
(#61998,#61999,#62000),(#62001,#62002,#62003),(#62004,#62005,#62006),(#62007,
#62008,#62009),(#62010,#62011,#62012),(#62013,#62014,#62015),(#62016,#62017,
#62018),(#62019,#62020,#62021),(#62022,#62023,#62024),(#62025,#62026,#62027),
(#62028,#62029,#62030),(#62031,#62032,#62033),(#62034,#62035,#62036),(#62037,
#62038,#62039),(#62040,#62041,#62042),(#62043,#62044,#62045),(#62046,#62047,
#62048),(#62049,#62050,#62051),(#62052,#62053,#62054),(#62055,#62056,#62057),
(#62058,#62059,#62060),(#62061,#62062,#62063),(#62064,#62065,#62066),(#62067,
#62068,#62069),(#62070,#62071,#62072),(#62073,#62074,#62075),(#62076,#62077,
#62078),(#62079,#62080,#62081),(#62082,#62083,#62084),(#62085,#62086,#62087),
(#62088,#62089,#62090),(#62091,#62092,#62093),(#62094,#62095,#62096),(#62097,
#62098,#62099),(#62100,#62101,#62102),(#62103,#62104,#62105),(#62106,#62107,
#62108),(#62109,#62110,#62111),(#62112,#62113,#62114),(#62115,#62116,#62117),
(#62118,#62119,#62120),(#62121,#62122,#62123),(#62124,#62125,#62126),(#62127,
#62128,#62129),(#62130,#62131,#62132),(#62133,#62134,#62135),(#62136,#62137,
#62138),(#62139,#62140,#62141),(#62142,#62143,#62144),(#62145,#62146,#62147),
(#62148,#62149,#62150),(#62151,#62152,#62153),(#62154,#62155,#62156),(#62157,
#62158,#62159),(#62160,#62161,#62162),(#62163,#62164,#62165),(#62166,#62167,
#62168),(#62169,#62170,#62171),(#62172,#62173,#62174),(#62175,#62176,#62177),
(#62178,#62179,#62180),(#62181,#62182,#62183),(#62184,#62185,#62186),(#62187,
#62188,#62189),(#62190,#62191,#62192),(#62193,#62194,#62195),(#62196,#62197,
#62198),(#62199,#62200,#62201),(#62202,#62203,#62204),(#62205,#62206,#62207),
(#62208,#62209,#62210),(#62211,#62212,#62213),(#62214,#62215,#62216),(#62217,
#62218,#62219),(#62220,#62221,#62222),(#62223,#62224,#62225),(#62226,#62227,
#62228),(#62229,#62230,#62231),(#62232,#62233,#62234),(#62235,#62236,#62237),
(#62238,#62239,#62240),(#62241,#62242,#62243),(#62244,#62245,#62246),(#62247,
#62248,#62249),(#62250,#62251,#62252),(#62253,#62254,#62255),(#62256,#62257,
#62258)),.UNSPECIFIED.,.F.,.F.,.F.)
B_SPLINE_SURFACE_WITH_KNOTS((4,2,2,2,2,2,2,2,2,2,2,2,2,2,2,2,2,2,2,2,2,
2,2,2,2,2,2,2,2,2,2,2,2,2,2,2,2,2,2,2,2,2,2,2,2,2,2,2,2,2,2,2,2,2,2,2,2,
4),(3,3),(0.0134638639862926,0.0138444481692976,0.0142250323523026,0.0144153244438052,
0.0145104704895564,0.0145580435124321,0.0146056165353077,0.0149862007183127,
0.0153667849013178,0.0155570769928203,0.0156046500156959,0.0156522230385716,
0.0157473690843228,0.0161279532673279,0.0165085374503329,0.0166036834960842,
0.0166988295418354,0.0168891216333379,0.017269705816343,0.017650289999348,
0.0178405820908505,0.0179357281366018,0.0180308741823531,0.0184114583653581,
0.0187920425483631,0.0191726267313682,0.0195532109143732,0.0196007839372489,
0.0196483569601245,0.0197435030058757,0.0199337950973783,0.0203143792803833,
0.0206949634633883,0.0210755476463934,0.0211706936921447,0.0212182667150203,
0.0212658397378959,0.0214561318293984,0.0218367160124035,0.0222173001954085,
0.0225978843784136,0.0226930304241648,0.0227406034470404,0.0227881764699161,
0.0229784685614186,0.0233590527444236,0.0237396369274287,0.0239299290189312,
0.0240250750646825,0.0240726480875581,0.0241202211104337,0.0245008052934388,
0.0248813894764438,0.0252619736594488,0.0253095466823245,0.0253571197052001,
0.0254522657509514,0.0256425578424539),(0.,1.),.UNSPECIFIED.)
GEOMETRIC_REPRESENTATION_ITEM()
RATIONAL_B_SPLINE_SURFACE(((1.,0.902225890492542,1.),(1.,0.903132443490707,
1.),(1.,0.903653998020159,1.),(1.,0.903944517231158,1.),(1.,0.903713722905418,
1.),(1.,0.902804847362988,1.),(1.,0.902407978119384,1.),(1.,0.901670791643955,
1.),(1.,0.901401407340477,1.),(1.,0.900961642998138,1.),(1.,0.900809228648317,
1.),(1.,0.900493618235616,1.),(1.,0.900330315112404,1.),(1.,0.898811704236251,
1.),(1.,0.897115152223068,1.),(1.,0.8930832276658,1.),(1.,0.890747678105234,
1.),(1.,0.886791425592428,1.),(1.,0.885397053276724,1.),(1.,0.88356139649318,
1.),(1.,0.883189677780271,1.),(1.,0.882439027225991,1.),(1.,0.882059854491219,
1.),(1.,0.880910975326534,1.),(1.,0.880129910230349,1.),(1.,0.876151119296445,
1.),(1.,0.872733625123037,1.),(1.,0.865476631221263,1.),(1.,0.861636969494005,
1.),(1.,0.856594588614554,1.),(1.,0.855573946399914,1.),(1.,0.85350876220382,
1.),(1.,0.85246323174813,1.),(1.,0.849298841078223,1.),(1.,0.847155538255743,
1.),(1.,0.840632122902037,1.),(1.,0.836158689703462,1.),(1.,0.82699763309876,
1.),(1.,0.822309914051737,1.),(1.,0.815139949640102,1.),(1.,0.812726867725303,
1.),(1.,0.809075207829036,1.),(1.,0.807852647321983,1.),(1.,0.805397269639103,
1.),(1.,0.804163344999755,1.),(1.,0.797982958897003,1.),(1.,0.793019937597689,
1.),(1.,0.783088423023321,1.),(1.,0.778119879402164,1.),(1.,0.76820928668916,
1.),(1.,0.763267195819894,1.),(1.,0.75344296730385,1.),(1.,0.748560790284006,
1.),(1.,0.743122393008669,1.),(1.,0.742518700341634,1.),(1.,0.741315692842442,
1.),(1.,0.740716049307044,1.),(1.,0.738922777819631,1.),(1.,0.737734808757582,
1.),(1.,0.734194170605456,1.),(1.,0.731864767933108,1.),(1.,0.724974784496934,
1.),(1.,0.720512392415405,1.),(1.,0.711877877500243,1.),(1.,0.70770576200713,
1.),(1.,0.699681270084328,1.),(1.,0.69582890373149,1.),(1.,0.691232191837726,
1.),(1.,0.690323788182993,1.),(1.,0.688977948962119,1.),(1.,0.688531815215766,
1.),(1.,0.687646982863273,1.),(1.,0.687208339799286,1.),(1.,0.685033941452217,
1.),(1.,0.68335464007595,1.),(1.,0.678495463402553,1.),(1.,0.675494391175647,
1.),(1.,0.669957389536595,1.),(1.,0.667421498945256,1.),(1.,0.662800458311643,
1.),(1.,0.660715343376615,1.),(1.,0.658379180374724,1.),(1.,0.657925448212519,
1.),(1.,0.6572648494954,1.),(1.,0.657048060234475,1.),(1.,0.656622369647382,
1.),(1.,0.65641330403604,1.),(1.,0.655386526701698,1.),(1.,0.654624456485959,
1.),(1.,0.65250324404021,1.),(1.,0.65130900668008,1.),(1.,0.649293555942829,
1.),(1.,0.648472385523653,1.),(1.,0.647472276924539,1.),(1.,0.64717753120397,
1.),(1.,0.64678743528618,1.),(1.,0.646666074433016,1.),(1.,0.646496305039786,
1.),(1.,0.646441723439099,1.),(1.,0.646336727153311,1.),(1.,0.646286326879338,
1.),(1.,0.6458508188832,1.),(1.,0.645591760552018,1.),(1.,0.645249142331117,
1.),(1.,0.645165683168743,1.),(1.,0.645106841085182,1.),(1.,0.645131514983531,
1.),(1.,0.645188093182711,1.),(1.,0.645194786243544,1.),(1.,0.645208884878214,
1.),(1.,0.645216298795827,1.),(1.,0.64523934086315,1.),(1.,0.645255850813146,
1.),(1.,0.645307638180231,1.),(1.,0.645345156614371,1.),(1.,0.64538287972702,
1.)))
REPRESENTATION_ITEM('')
SURFACE()
);
#190=(
BOUNDED_SURFACE()
B_SPLINE_SURFACE(3,2,((#62260,#62261,#62262),(#62263,#62264,#62265),(#62266,
#62267,#62268),(#62269,#62270,#62271),(#62272,#62273,#62274),(#62275,#62276,
#62277),(#62278,#62279,#62280),(#62281,#62282,#62283),(#62284,#62285,#62286),
(#62287,#62288,#62289),(#62290,#62291,#62292),(#62293,#62294,#62295)),
 .UNSPECIFIED.,.F.,.F.,.F.)
B_SPLINE_SURFACE_WITH_KNOTS((4,2,2,2,2,4),(3,3),(-4.34222970080445E-17,
0.000193738907016803,0.000387477814033649,0.000484347267542072,0.000581216721050495,
0.000774955628067341),(0.,1.),.UNSPECIFIED.)
GEOMETRIC_REPRESENTATION_ITEM()
RATIONAL_B_SPLINE_SURFACE(((1.,0.902225890492542,1.),(1.,0.900702231639175,
1.),(1.,0.898361639865931,1.),(1.,0.892256701302875,1.),(1.,0.88849270261023,
1.),(1.,0.881893015251816,1.),(1.,0.87953374069531,1.),(1.,0.87451093966713,
1.),(1.,0.871866113555864,1.),(1.,0.863573635793879,1.),(1.,0.857564565511076,
1.),(1.,0.851143038957624,1.)))
REPRESENTATION_ITEM('')
SURFACE()
);
#191=(
BOUNDED_SURFACE()
B_SPLINE_SURFACE(3,2,((#62297,#62298,#62299),(#62300,#62301,#62302),(#62303,
#62304,#62305),(#62306,#62307,#62308),(#62309,#62310,#62311),(#62312,#62313,
#62314),(#62315,#62316,#62317),(#62318,#62319,#62320),(#62321,#62322,#62323),
(#62324,#62325,#62326),(#62327,#62328,#62329),(#62330,#62331,#62332),(#62333,
#62334,#62335),(#62336,#62337,#62338),(#62339,#62340,#62341),(#62342,#62343,
#62344),(#62345,#62346,#62347),(#62348,#62349,#62350),(#62351,#62352,#62353),
(#62354,#62355,#62356),(#62357,#62358,#62359),(#62360,#62361,#62362),(#62363,
#62364,#62365),(#62366,#62367,#62368),(#62369,#62370,#62371),(#62372,#62373,
#62374),(#62375,#62376,#62377),(#62378,#62379,#62380),(#62381,#62382,#62383),
(#62384,#62385,#62386),(#62387,#62388,#62389),(#62390,#62391,#62392),(#62393,
#62394,#62395),(#62396,#62397,#62398),(#62399,#62400,#62401),(#62402,#62403,
#62404),(#62405,#62406,#62407),(#62408,#62409,#62410),(#62411,#62412,#62413),
(#62414,#62415,#62416),(#62417,#62418,#62419),(#62420,#62421,#62422),(#62423,
#62424,#62425),(#62426,#62427,#62428),(#62429,#62430,#62431),(#62432,#62433,
#62434),(#62435,#62436,#62437),(#62438,#62439,#62440),(#62441,#62442,#62443),
(#62444,#62445,#62446),(#62447,#62448,#62449),(#62450,#62451,#62452),(#62453,
#62454,#62455),(#62456,#62457,#62458),(#62459,#62460,#62461),(#62462,#62463,
#62464),(#62465,#62466,#62467),(#62468,#62469,#62470),(#62471,#62472,#62473),
(#62474,#62475,#62476),(#62477,#62478,#62479),(#62480,#62481,#62482),(#62483,
#62484,#62485),(#62486,#62487,#62488),(#62489,#62490,#62491),(#62492,#62493,
#62494),(#62495,#62496,#62497),(#62498,#62499,#62500),(#62501,#62502,#62503),
(#62504,#62505,#62506),(#62507,#62508,#62509),(#62510,#62511,#62512),(#62513,
#62514,#62515),(#62516,#62517,#62518),(#62519,#62520,#62521),(#62522,#62523,
#62524),(#62525,#62526,#62527),(#62528,#62529,#62530),(#62531,#62532,#62533),
(#62534,#62535,#62536),(#62537,#62538,#62539),(#62540,#62541,#62542),(#62543,
#62544,#62545),(#62546,#62547,#62548),(#62549,#62550,#62551),(#62552,#62553,
#62554),(#62555,#62556,#62557),(#62558,#62559,#62560),(#62561,#62562,#62563),
(#62564,#62565,#62566),(#62567,#62568,#62569),(#62570,#62571,#62572),(#62573,
#62574,#62575),(#62576,#62577,#62578),(#62579,#62580,#62581),(#62582,#62583,
#62584),(#62585,#62586,#62587),(#62588,#62589,#62590),(#62591,#62592,#62593),
(#62594,#62595,#62596),(#62597,#62598,#62599),(#62600,#62601,#62602)),
 .UNSPECIFIED.,.F.,.F.,.F.)
B_SPLINE_SURFACE_WITH_KNOTS((4,2,2,2,2,2,2,2,2,2,2,2,2,2,2,2,2,2,2,2,2,
2,2,2,2,2,2,2,2,2,2,2,2,2,2,2,2,2,2,2,2,2,2,2,2,2,2,2,2,2,4),(3,3),(0.0137607578966189,
0.0141248143649128,0.0144888708332067,0.0148529273015007,0.0152169837697946,
0.0155810402380886,0.015672054355162,0.0157630684722355,0.0159450967063825,
0.0163091531746764,0.0166732096429704,0.0170372661112643,0.0174013225795583,
0.0175833508137052,0.0176743649307787,0.0177653790478522,0.0181294355161461,
0.0184934919844401,0.018857548452734,0.019039576686881,0.0191305908039545,
0.019221604921028,0.0195856613893219,0.0199497178576158,0.0203137743259098,
0.0203592813844465,0.0204047884429833,0.0204958025600567,0.0206778307942037,
0.0210418872624977,0.0214059437307916,0.0215879719649386,0.0216789860820121,
0.0217700001990855,0.0221340566673795,0.0224981131356734,0.0226801413698204,
0.0227256484283571,0.0227711554868939,0.0228621696039674,0.0232262260722613,
0.0235902825405552,0.0237723107747022,0.0238633248917757,0.0239543390088492,
0.0243183954771431,0.0246824519454371,0.025046508413731,0.0251375225308045,
0.025228536647878,0.0254105648820249),(0.,1.),.UNSPECIFIED.)
GEOMETRIC_REPRESENTATION_ITEM()
RATIONAL_B_SPLINE_SURFACE(((1.,0.851143038957625,1.),(1.,0.846479387833395,
1.),(1.,0.841684047649747,1.),(1.,0.831843628329292,1.),(1.,0.826798581401555,
1.),(1.,0.816468255419326,1.),(1.,0.811182939537333,1.),(1.,0.800378089079313,
1.),(1.,0.79485852833921,1.),(1.,0.783588798399719,1.),(1.,0.77783860835381,
1.),(1.,0.770507923158056,1.),(1.,0.769034635357085,1.),(1.,0.766073776121258,
1.),(1.,0.764586399638179,1.),(1.,0.760117744617778,1.),(1.,0.757125076740806,
1.),(1.,0.748108634667927,1.),(1.,0.742046356031758,1.),(1.,0.729832440045022,
1.),(1.,0.723680764192416,1.),(1.,0.711303823843107,1.),(1.,0.705078509161493,
1.),(1.,0.6925739237358,1.),(1.,0.686294583365353,1.),(1.,0.676854046105913,
1.),(1.,0.673703662794336,1.),(1.,0.668975704676001,1.),(1.,0.667399235894792,
1.),(1.,0.664246417134242,1.),(1.,0.662674576423675,1.),(1.,0.654839788640746,
1.),(1.,0.648649695295625,1.),(1.,0.636471040983231,1.),(1.,0.630482388018559,
1.),(1.,0.618763892218915,1.),(1.,0.613033921427266,1.),(1.,0.604686972618327,
1.),(1.,0.601946116421347,1.),(1.,0.597905078993139,1.),(1.,0.596569784084661,
1.),(1.,0.593924099614706,1.),(1.,0.592613436616545,1.),(1.,0.586158271598212,
1.),(1.,0.581281465080226,1.),(1.,0.572174439101757,1.),(1.,0.567944193517853,
1.),(1.,0.560213073119294,1.),(1.,0.55671214421852,1.),(1.,0.553237178148869,
1.),(1.,0.55285751778881,1.),(1.,0.55211129142054,1.),(1.,0.551744475791875,
1.),(1.,0.550665824157476,1.),(1.,0.549976737095303,1.),(1.,0.54799961392759,
1.),(1.,0.546801718122489,1.),(1.,0.543569310149808,1.),(1.,0.54189614782828,
1.),(1.,0.539515970413853,1.),(1.,0.53880894909132,1.),(1.,0.538473378107389,
1.),(1.,0.538482331182785,1.),(1.,0.538676931129144,1.),(1.,0.538772236119652,
1.),(1.,0.539021359113027,1.),(1.,0.539175170865797,1.),(1.,0.540085972132753,
1.),(1.,0.541267672929542,1.),(1.,0.544430358927514,1.),(1.,0.546411368970525,
1.),(1.,0.549911779882456,1.),(1.,0.551166829738738,1.),(1.,0.552839328341023,
1.),(1.,0.553179014364036,1.),(1.,0.553868601162557,1.),(1.,0.554218660677656,
1.),(1.,0.555280888150674,1.),(1.,0.55600596370185,1.),(1.,0.559710766897414,
1.),(1.,0.562927650586242,1.),(1.,0.569753621382414,1.),(1.,0.573362909796628,
1.),(1.,0.579004661887682,1.),(1.,0.580923392305157,1.),(1.,0.58385183530157,
1.),(1.,0.584836827643457,1.),(1.,0.586820704360992,1.),(1.,0.587816792889683,
1.),(1.,0.592815092417132,1.),(1.,0.596870022611588,1.),(1.,0.605033066578426,
1.),(1.,0.609141359017907,1.),(1.,0.617370572384848,1.),(1.,0.621491593376493,
1.),(1.,0.626634299394224,1.),(1.,0.627661241677736,1.),(1.,0.629705159449786,
1.),(1.,0.630723104403595,1.),(1.,0.633764717654218,1.),(1.,0.635776155601376,
1.),(1.,0.637771010909975,1.)))
REPRESENTATION_ITEM('')
SURFACE()
);
#258=FACE_BOUND('',#5265,.T.);
#259=FACE_BOUND('',#5266,.T.);
#260=FACE_BOUND('',#5277,.T.);
#261=FACE_BOUND('',#5278,.T.);
#262=FACE_BOUND('',#5319,.T.);
#263=FACE_BOUND('',#5320,.T.);
#264=FACE_BOUND('',#5321,.T.);
#265=FACE_BOUND('',#5370,.T.);
#266=FACE_BOUND('',#5374,.T.);
#267=FACE_BOUND('',#5378,.T.);
#268=FACE_BOUND('',#5384,.T.);
#269=FACE_BOUND('',#5386,.T.);
#270=FACE_BOUND('',#5387,.T.);
#271=FACE_BOUND('',#5412,.T.);
#272=FACE_BOUND('',#5413,.T.);
#273=FACE_BOUND('',#5448,.T.);
#274=FACE_BOUND('',#5461,.T.);
#669=PLANE('',#16645);
#670=PLANE('',#16646);
#671=PLANE('',#16647);
#672=PLANE('',#16652);
#673=PLANE('',#16656);
#674=PLANE('',#16659);
#675=PLANE('',#16662);
#676=PLANE('',#16665);
#677=PLANE('',#16675);
#678=PLANE('',#16742);
#679=PLANE('',#16743);
#680=PLANE('',#16745);
#681=PLANE('',#16746);
#682=PLANE('',#16749);
#683=PLANE('',#16754);
#684=PLANE('',#16755);
#685=PLANE('',#16759);
#686=PLANE('',#16765);
#687=PLANE('',#16768);
#688=PLANE('',#16769);
#689=PLANE('',#16779);
#690=PLANE('',#16780);
#691=PLANE('',#16784);
#692=PLANE('',#16790);
#693=PLANE('',#16791);
#694=PLANE('',#16797);
#695=PLANE('',#16798);
#696=PLANE('',#16802);
#697=PLANE('',#16803);
#698=PLANE('',#16804);
#699=PLANE('',#16806);
#700=PLANE('',#16807);
#701=PLANE('',#16808);
#702=PLANE('',#16809);
#703=PLANE('',#16810);
#704=PLANE('',#16812);
#705=PLANE('',#16813);
#706=PLANE('',#16814);
#707=PLANE('',#16841);
#708=PLANE('',#16847);
#709=PLANE('',#16848);
#710=PLANE('',#16849);
#711=PLANE('',#16850);
#712=PLANE('',#16851);
#713=PLANE('',#16855);
#770=ELLIPSE('',#16490,0.787132929614446,0.490404666125977);
#771=ELLIPSE('',#16525,11.474561377534,5.80198696989729);
#772=ELLIPSE('',#16570,0.707106781186205,0.500000000000487);
#773=ELLIPSE('',#16578,7.07106781186394,4.99999999999909);
#774=ELLIPSE('',#16581,7.07106781196844,5.00000000004573);
#775=ELLIPSE('',#16584,2.82842712474406,1.99999999999928);
#776=ELLIPSE('',#16607,0.707106781180475,0.49999999999776);
#777=ELLIPSE('',#16694,0.65489735345099,0.499999999998802);
#778=ELLIPSE('',#16701,0.654897353451537,0.499999999999167);
#779=ELLIPSE('',#16706,0.93246545981575,0.499999999999451);
#780=ELLIPSE('',#16708,0.570504795854994,0.499999999999747);
#781=ELLIPSE('',#16729,0.520708654805954,0.500000000000599);
#782=ELLIPSE('',#16741,0.707106781185331,0.499999999999033);
#783=ELLIPSE('',#16748,1.30979470690588,1.00000000000042);
#784=ELLIPSE('',#16751,1.06587697723058,0.998342579493648);
#785=ELLIPSE('',#16756,7.07106781178892,4.99999999996606);
#786=ELLIPSE('',#16758,7.07106781478535,5.00000000116881);
#787=ELLIPSE('',#16766,1.02590924137892,0.995770746428315);
#788=ELLIPSE('',#16782,0.707106781186607,0.499999999999867);
#789=ELLIPSE('',#16788,0.501870829776834,0.499498521952907);
#790=ELLIPSE('',#16789,0.501871930366977,0.4994982286229);
#791=ELLIPSE('',#16793,0.80842845737287,0.499999999999691);
#792=ELLIPSE('',#16796,1.18473126058658,1.00000495319552);
#793=ELLIPSE('',#16831,1.30979470690618,1.00000000000064);
#794=ELLIPSE('',#16852,8.39218913835177,4.49999999999994);
#917=B_SPLINE_CURVE_WITH_KNOTS('',3,(#45572,#45573,#45574,#45575,#45576,
#45577,#45578,#45579,#45580,#45581,#45582,#45583),.UNSPECIFIED.,.F.,.F.,
(4,2,2,2,2,4),(9.92264902769865E-7,0.0122814154766666,0.0227351808389828,
0.0425013028347888,0.0639899300112591,0.0846625935368686),.UNSPECIFIED.);
#918=B_SPLINE_CURVE_WITH_KNOTS('',3,(#45602,#45603,#45604,#45605,#45606,
#45607,#45608,#45609,#45610,#45611,#45612,#45613,#45614,#45615,#45616,#45617,
#45618,#45619,#45620,#45621,#45622,#45623,#45624,#45625,#45626,#45627,#45628,
#45629,#45630,#45631,#45632,#45633,#45634,#45635,#45636,#45637,#45638,#45639,
#45640,#45641,#45642,#45643,#45644,#45645,#45646,#45647,#45648,#45649,#45650,
#45651,#45652,#45653,#45654,#45655,#45656,#45657,#45658,#45659,#45660,#45661,
#45662,#45663,#45664,#45665,#45666,#45667,#45668,#45669,#45670,#45671,#45672,
#45673,#45674,#45675,#45676,#45677,#45678,#45679,#45680,#45681,#45682,#45683,
#45684,#45685,#45686,#45687,#45688,#45689,#45690,#45691,#45692,#45693,#45694,
#45695,#45696,#45697,#45698,#45699,#45700,#45701,#45702,#45703,#45704,#45705,
#45706,#45707,#45708,#45709,#45710,#45711,#45712,#45713,#45714,#45715,#45716,
#45717,#45718,#45719,#45720,#45721,#45722,#45723,#45724,#45725,#45726,#45727,
#45728,#45729,#45730,#45731,#45732,#45733,#45734,#45735,#45736,#45737,#45738,
#45739,#45740,#45741,#45742,#45743,#45744,#45745,#45746),.UNSPECIFIED.,
 .F.,.F.,(4,3,3,3,3,3,3,3,3,3,3,3,3,3,3,3,3,3,3,3,3,3,3,3,3,3,3,3,3,3,3,
3,3,3,3,3,3,3,3,3,3,3,3,3,3,3,3,3,4),(0.0054539128671712,0.00548380874985591,
0.00565888988694723,0.00577243026300616,0.00591674101958129,0.00595688595087576,
0.00598889639786886,0.00603110776681321,0.00606105177615643,0.00606817280695972,
0.00610520328963597,0.00625299641255915,0.00634967328930671,0.00654698557014318,
0.00663829480245699,0.00683895447912464,0.00692691631560727,0.00707122707218241,
0.00712902509780294,0.00714338245046997,0.00717946013961376,0.0072012572687105,
0.00721553782875754,0.00723732988878856,0.00727337941031582,0.0074173491882449,
0.00750415934190779,0.00770421253731256,0.00779278085505804,0.0079897749319241,
0.00808140236820829,0.00813211305141546,0.00820317794008171,0.00822571312478341,
0.00823868030383458,0.00827417239358472,0.00829786850307098,0.00837002388135854,
0.00855773776014578,0.00865864539450881,0.00884069465909997,0.00894726690765908,
0.00909157766423421,0.00912311752903997,0.00915838665328199,0.00916373304252177,
0.00919361503382806,0.00919981073166556,0.00923588842080934),
 .UNSPECIFIED.);
#919=B_SPLINE_CURVE_WITH_KNOTS('',3,(#45748,#45749,#45750,#45751),
 .UNSPECIFIED.,.F.,.F.,(4,4),(1.4574000303393E-16,0.0113332377793703),
 .UNSPECIFIED.);
#920=B_SPLINE_CURVE_WITH_KNOTS('',3,(#45753,#45754,#45755,#45756,#45757,
#45758,#45759,#45760,#45761,#45762,#45763,#45764,#45765,#45766,#45767,#45768,
#45769,#45770,#45771,#45772,#45773,#45774,#45775,#45776,#45777,#45778,#45779,
#45780,#45781,#45782,#45783,#45784,#45785,#45786,#45787,#45788,#45789,#45790,
#45791,#45792,#45793,#45794,#45795,#45796,#45797,#45798,#45799,#45800,#45801,
#45802,#45803,#45804,#45805,#45806,#45807,#45808,#45809,#45810,#45811,#45812,
#45813,#45814,#45815,#45816,#45817,#45818,#45819,#45820,#45821,#45822,#45823,
#45824,#45825,#45826,#45827,#45828,#45829,#45830,#45831,#45832,#45833,#45834,
#45835,#45836,#45837,#45838,#45839,#45840,#45841,#45842,#45843,#45844,#45845,
#45846,#45847,#45848,#45849,#45850,#45851,#45852,#45853,#45854,#45855,#45856,
#45857,#45858,#45859,#45860,#45861,#45862,#45863,#45864,#45865,#45866,#45867,
#45868,#45869,#45870,#45871,#45872,#45873,#45874,#45875,#45876,#45877,#45878,
#45879,#45880,#45881,#45882,#45883,#45884,#45885,#45886,#45887,#45888,#45889,
#45890,#45891,#45892,#45893,#45894,#45895,#45896,#45897,#45898,#45899,#45900,
#45901,#45902,#45903,#45904,#45905,#45906,#45907,#45908,#45909,#45910,#45911,
#45912,#45913,#45914,#45915,#45916,#45917,#45918,#45919,#45920,#45921,#45922,
#45923,#45924,#45925,#45926,#45927,#45928,#45929,#45930,#45931,#45932,#45933,
#45934,#45935,#45936,#45937,#45938,#45939,#45940,#45941,#45942,#45943,#45944,
#45945,#45946,#45947,#45948,#45949,#45950,#45951,#45952,#45953,#45954,#45955,
#45956,#45957,#45958,#45959,#45960,#45961,#45962,#45963,#45964,#45965,#45966,
#45967,#45968,#45969,#45970,#45971,#45972,#45973,#45974,#45975,#45976,#45977,
#45978,#45979,#45980,#45981,#45982,#45983,#45984,#45985,#45986,#45987,#45988,
#45989,#45990,#45991,#45992,#45993,#45994,#45995,#45996,#45997,#45998,#45999,
#46000,#46001,#46002,#46003,#46004,#46005,#46006,#46007,#46008,#46009,#46010,
#46011,#46012,#46013,#46014,#46015,#46016,#46017,#46018,#46019,#46020,#46021,
#46022,#46023,#46024,#46025,#46026,#46027,#46028,#46029,#46030,#46031,#46032),
 .UNSPECIFIED.,.F.,.F.,(4,3,3,3,3,3,3,3,3,3,3,3,3,3,3,3,3,3,3,3,3,3,3,3,
3,3,3,3,3,3,3,3,3,3,3,3,3,3,3,3,3,3,3,3,3,3,3,3,3,3,3,3,3,3,3,3,3,3,3,3,
3,3,3,3,3,3,3,3,3,3,3,3,3,3,3,3,3,3,3,3,3,3,3,3,3,3,3,3,3,3,3,3,3,4),(0.,
9.06394666082451E-5,9.84186019154758E-5,0.00018127893321649,0.000196344891157804,
0.000271918399824735,0.000293789584677031,0.000317238133128857,0.000339897999780917,
0.000342304633973775,0.000362557866432978,0.000390537263439263,0.000453197333041227,
0.000486049915227595,0.000543836799649477,0.000580320870217935,0.000626990715264167,
0.000634476266257726,0.00065020402445471,0.000657136132909784,0.000673323081798869,
0.000679795999561842,0.000725115732865958,0.000764841371010614,0.000815755199474182,
0.0008548576554711,0.000906394666082406,0.000929054532734454,0.000943371418524607,
0.000951714399386503,0.000997034132690586,0.00103051440248908,0.00108767359929875,
0.0011164662936885,0.00117831306590692,0.00120123217101674,0.001223632799211,
0.00124316188010154,0.00124629266586303,0.00126895253251506,0.00128486511176821,
0.00135959199912321,0.00136785720613342,0.00145023146573136,0.00145030648535944,
0.0014728913323834,0.00149133041292132,0.00149555119903544,0.00151188331859317,
0.00151821106568749,0.001532528558112,0.00154087093233953,0.00161565551529423,
0.00163151039894771,0.00169958627364771,0.00172214986555588,0.00176746959885996,
0.00178431737336985,0.00179012946551201,0.00181278933216405,0.00182701790521884,
0.00187007299327093,0.00190342879877218,0.00195723834581456,0.00199406826538032,
0.00204581493813314,0.00208470773198846,0.00209063844107407,0.00210736759864049,
0.00213002746529252,0.00213582758039994,0.00217534719859659,0.00222729219943231,
0.00226598666520473,0.00232019847227704,0.00235662613181287,0.0023672014340626,
0.00240194586511693,0.00241457759770203,0.00242460573176897,0.00244726559842101,
0.00251014587586458,0.00253790506502916,0.00260663317312218,0.00262854453163731,
0.00270404516267542,0.00271918399824546,0.00272854743294039,0.00274184386489749,
0.00275310480366504,0.00276450373154952,0.00280223551954616,0.00280982346485358,
0.00290046293146171),.UNSPECIFIED.);
#921=B_SPLINE_CURVE_WITH_KNOTS('',3,(#46034,#46035,#46036,#46037),
 .UNSPECIFIED.,.F.,.F.,(4,4),(0.,0.011206889852584),.UNSPECIFIED.);
#922=B_SPLINE_CURVE_WITH_KNOTS('',3,(#46039,#46040,#46041,#46042,#46043,
#46044,#46045,#46046,#46047,#46048,#46049,#46050,#46051,#46052,#46053,#46054,
#46055,#46056,#46057,#46058,#46059,#46060,#46061,#46062,#46063,#46064,#46065,
#46066,#46067,#46068,#46069,#46070,#46071,#46072,#46073,#46074,#46075,#46076,
#46077,#46078,#46079,#46080,#46081,#46082,#46083,#46084),.UNSPECIFIED.,
 .F.,.F.,(4,2,1,2,2,2,2,2,2,1,2,2,2,2,1,1,2,2,2,2,2,2,1,1,2,4),(0.000392395285594788,
0.000660337424393816,0.000794308909059438,0.00086129465139225,0.000928280393725061,
0.00119622336305629,0.00146416633238753,0.00173210930171876,0.00179909504405157,
0.00186608078638437,0.00200005227104998,0.0022679952403812,0.00253593820971242,
0.00256943108087883,0.00260292395204523,0.00266990969437803,0.00280388117904364,
0.00307182414837484,0.00333976711770605,0.00340675286003885,0.00347373860237165,
0.00350723147353805,0.00354072434470446,0.00360771008703726,0.00387565305636847,
0.0040894670158376),.UNSPECIFIED.);
#923=B_SPLINE_CURVE_WITH_KNOTS('',3,(#46090,#46091,#46092,#46093,#46094,
#46095,#46096,#46097),.UNSPECIFIED.,.F.,.F.,(4,3,1,4),(0.000295555998119065,
0.00492308001881893,0.00630130897220404,0.00659646431556111),
 .UNSPECIFIED.);
#924=B_SPLINE_CURVE_WITH_KNOTS('',3,(#46101,#46102,#46103,#46104,#46105,
#46106,#46107,#46108,#46109,#46110),.UNSPECIFIED.,.F.,.F.,(4,3,3,4),(-0.000295155343349986,
1.44198888940572E-17,0.0051169388442874,0.00600575297407752),
 .UNSPECIFIED.);
#925=B_SPLINE_CURVE_WITH_KNOTS('',3,(#46113,#46114,#46115,#46116,#46117,
#46118,#46119,#46120,#46121,#46122,#46123,#46124,#46125,#46126,#46127,#46128,
#46129,#46130,#46131,#46132,#46133,#46134,#46135,#46136,#46137,#46138,#46139,
#46140,#46141,#46142,#46143,#46144,#46145,#46146,#46147,#46148,#46149,#46150,
#46151,#46152,#46153),.UNSPECIFIED.,.F.,.F.,(4,2,2,2,1,2,2,2,2,2,2,1,1,
1,1,1,2,1,2,2,1,1,1,1,2,4),(0.0040894670158376,0.00414359602569968,0.00441153899503089,
0.0044785247373637,0.0045455104796965,0.00467948196436211,0.00494742493369333,
0.00521536790302455,0.00548331087235577,0.00561728235702139,0.00568426809935419,
0.005751253841687,0.00601919681101826,0.00628713978034951,0.00655508274968077,
0.00682302571901203,0.00709096868834328,0.00722494017300891,0.00729192591534172,
0.00735891165767452,0.00762685462700575,0.00789479759633698,0.0081627405656682,
0.00843068353499943,0.00869862650433066,0.00896656947366188),
 .UNSPECIFIED.);
#926=B_SPLINE_CURVE_WITH_KNOTS('',3,(#46155,#46156,#46157,#46158,#46159,
#46160,#46161,#46162,#46163,#46164,#46165,#46166,#46167,#46168,#46169,#46170,
#46171,#46172,#46173,#46174,#46175,#46176,#46177,#46178,#46179,#46180,#46181,
#46182,#46183,#46184,#46185,#46186,#46187,#46188,#46189,#46190,#46191,#46192,
#46193,#46194,#46195,#46196,#46197),.UNSPECIFIED.,.F.,.F.,(4,3,3,3,3,3,
3,3,3,3,3,3,3,3,4),(0.,0.000117052501055883,0.000153349582659865,0.000161023794644849,
0.0002300243739898,0.000239696739155573,0.000268361769654766,0.000317031808608993,
0.000383373956649677,0.000460048747979621,0.000467463358429797,0.000498386143644593,
0.000523040524368854,0.000536723539309575,0.000613398330639558),
 .UNSPECIFIED.);
#927=B_SPLINE_CURVE_WITH_KNOTS('',3,(#46198,#46199,#46200,#46201,#46202,
#46203,#46204,#46205,#46206,#46207,#46208,#46209,#46210,#46211,#46212,#46213,
#46214,#46215,#46216,#46217,#46218,#46219,#46220,#46221,#46222,#46223,#46224,
#46225,#46226,#46227,#46228,#46229,#46230,#46231,#46232,#46233,#46234,#46235,
#46236,#46237,#46238,#46239,#46240,#46241,#46242,#46243,#46244,#46245,#46246,
#46247,#46248,#46249,#46250,#46251,#46252,#46253,#46254,#46255,#46256,#46257,
#46258,#46259,#46260,#46261,#46262,#46263,#46264,#46265,#46266,#46267,#46268,
#46269,#46270,#46271,#46272,#46273,#46274,#46275,#46276,#46277,#46278,#46279,
#46280,#46281,#46282,#46283,#46284,#46285,#46286,#46287,#46288,#46289,#46290,
#46291,#46292,#46293,#46294,#46295,#46296,#46297,#46298,#46299,#46300,#46301,
#46302,#46303,#46304,#46305,#46306,#46307,#46308,#46309,#46310,#46311,#46312,
#46313,#46314,#46315,#46316,#46317,#46318,#46319,#46320,#46321,#46322,#46323,
#46324,#46325,#46326,#46327,#46328,#46329,#46330,#46331,#46332,#46333,#46334,
#46335,#46336,#46337,#46338,#46339),.UNSPECIFIED.,.F.,.F.,(4,3,3,3,3,3,
3,3,3,3,3,3,3,3,3,3,3,3,3,3,3,3,3,3,3,3,3,3,3,3,3,3,3,3,3,3,3,3,3,3,3,3,
3,3,3,3,3,4),(0.,0.000218348361755657,0.000288621513150416,0.000509762429138871,
0.000577243026300831,0.000649398404588435,0.000685476093732232,0.000721553782876029,
0.000757631472019826,0.000793709161163623,0.000865864539451206,0.00106157890238537,
0.00115448605260153,0.00136621152949033,0.00144310756575185,0.00151526294403943,
0.00158741832232702,0.00173172907890218,0.00193773404538904,0.00202035059205251,
0.00224290230807321,0.00230897210520284,0.00238112748349041,0.00245328286177799,
0.00259759361835315,0.00282626847197688,0.00288621513150347,0.00312835477281512,
0.00317483664465379,0.00342364710957266,0.00346345815780411,0.0034995358469479,
0.00353561353609168,0.00360776891437925,0.00375207967095438,0.00400768565379299,
0.00404070118410464,0.0042978895511761,0.00432932269725489,0.00458016139294931,
0.00461794421040514,0.00476225496698027,0.00479833265612405,0.00483441034526783,
0.00490656572355539,0.00516688963479163,0.00519518723670565,0.00545391286716091),
 .UNSPECIFIED.);
#928=B_SPLINE_CURVE_WITH_KNOTS('',3,(#46344,#46345,#46346,#46347,#46348,
#46349,#46350,#46351,#46352,#46353),.UNSPECIFIED.,.F.,.F.,(4,2,2,2,4),(-0.188504168620313,
-0.178198215106625,-0.166932202633752,-0.154946150113528,-0.14212773138048),
 .UNSPECIFIED.);
#929=B_SPLINE_CURVE_WITH_KNOTS('',3,(#46354,#46355,#46356,#46357,#46358,
#46359,#46360,#46361,#46362,#46363),.UNSPECIFIED.,.F.,.F.,(4,2,2,2,4),(-0.0468417359580142,
-0.0340233172249645,-0.0220372647047389,-0.0107712522318653,-0.000465298718183977),
 .UNSPECIFIED.);
#930=B_SPLINE_CURVE_WITH_KNOTS('',3,(#46372,#46373,#46374,#46375,#46376,
#46377,#46378,#46379,#46380,#46381,#46382,#46383,#46384,#46385,#46386,#46387,
#46388,#46389,#46390,#46391,#46392,#46393,#46394,#46395,#46396,#46397,#46398,
#46399,#46400,#46401,#46402,#46403,#46404,#46405,#46406,#46407,#46408,#46409,
#46410,#46411,#46412,#46413,#46414,#46415,#46416,#46417,#46418,#46419,#46420,
#46421,#46422,#46423,#46424,#46425,#46426,#46427,#46428,#46429,#46430,#46431,
#46432,#46433,#46434,#46435,#46436,#46437,#46438,#46439,#46440,#46441,#46442,
#46443,#46444,#46445,#46446,#46447,#46448,#46449,#46450,#46451,#46452,#46453,
#46454,#46455,#46456,#46457,#46458,#46459,#46460,#46461,#46462,#46463,#46464,
#46465,#46466,#46467,#46468,#46469,#46470,#46471,#46472,#46473,#46474,#46475,
#46476,#46477,#46478,#46479,#46480,#46481,#46482,#46483,#46484,#46485,#46486,
#46487,#46488,#46489,#46490,#46491,#46492,#46493,#46494,#46495,#46496,#46497,
#46498,#46499,#46500,#46501,#46502,#46503,#46504,#46505,#46506,#46507,#46508,
#46509,#46510,#46511,#46512,#46513,#46514,#46515,#46516,#46517,#46518,#46519,
#46520,#46521,#46522,#46523,#46524,#46525,#46526,#46527,#46528,#46529,#46530,
#46531,#46532,#46533,#46534,#46535,#46536,#46537,#46538,#46539,#46540,#46541,
#46542,#46543,#46544,#46545,#46546,#46547,#46548,#46549,#46550,#46551,#46552,
#46553,#46554,#46555,#46556,#46557,#46558,#46559,#46560,#46561,#46562,#46563,
#46564,#46565,#46566,#46567,#46568,#46569,#46570,#46571,#46572,#46573,#46574,
#46575,#46576,#46577,#46578,#46579,#46580,#46581,#46582,#46583,#46584,#46585,
#46586,#46587,#46588,#46589,#46590,#46591,#46592,#46593,#46594,#46595,#46596,
#46597,#46598,#46599,#46600,#46601,#46602,#46603,#46604,#46605,#46606,#46607,
#46608,#46609,#46610,#46611,#46612,#46613,#46614,#46615,#46616,#46617,#46618,
#46619,#46620,#46621,#46622,#46623,#46624,#46625,#46626,#46627,#46628,#46629,
#46630,#46631,#46632,#46633,#46634,#46635,#46636,#46637,#46638,#46639,#46640,
#46641,#46642,#46643,#46644,#46645,#46646,#46647,#46648,#46649,#46650,#46651,
#46652,#46653,#46654),.UNSPECIFIED.,.F.,.F.,(4,3,3,3,3,3,3,3,3,3,3,3,3,
3,3,3,3,3,3,3,3,3,3,3,3,3,3,3,3,3,3,3,3,3,3,3,3,3,3,3,3,3,3,3,3,3,3,3,3,
3,3,3,3,3,3,3,3,3,3,3,3,3,3,3,3,3,3,3,3,3,3,3,3,3,3,3,3,3,3,3,3,3,3,3,3,
3,3,3,3,3,3,3,3,3,4),(0.,0.0003242112872066,0.000357261792737838,0.000648422574413201,
0.000713397984116496,0.000972633861619801,0.00106849099687377,0.0012968451488264,
0.00142259046797538,0.001621056436033,0.00177571862495347,0.0017831620796363,
0.00186384905495805,0.00186421490143795,0.00190474131233878,0.0019452677232396,
0.00195192061876334,0.00212790648128734,0.00226947901044622,0.00247923627193231,
0.00259369029765284,0.00282972486348799,0.00291790158485946,0.00317934752697371,
0.00324211287206608,0.00352806077583578,0.0035663241592727,0.00370205576559277,
0.00372842980287601,0.00376895621377683,0.00378895854388717,0.00380948262467766,
0.00387581262257363,0.00389053544647929,0.00421474673368583,0.00422290205403573,
0.00453895802089236,0.00456943462611516,0.0048631693080989,0.00491535430262632,
0.00508806280169499,0.00517434618899021,0.00518738059530543,0.00522790700620624,
0.00526059483948565,0.00526843341710705,0.00534948623890867,0.00551159188251191,
0.00560569480955727,0.00583580316971839,0.00595096223417242,0.00616001445692487,
0.00629637362108293,0.00632212010052811,0.00633956008149765,0.00636264651142892,
0.00638274886077817,0.00640317292232973,0.00646917189092978,0.00648422574413136,
0.00664226599303563,0.00680843703133785,0.00698941739492064,0.00713264831854435,
0.0073378495654889,0.00745685960575085,0.00751255500574631,0.00753791242755247,
0.00757843883845328,0.00760003330101165,0.00761896524935409,0.00768763257202629,
0.00778107089295735,0.00803922882622409,0.00810528218016386,0.00839270938616917,
0.00842949346737037,0.00857015221794751,0.00859159911097363,0.00861458669111193,
0.00865905017453961,0.00867265193277526,0.00874805663922665,0.00875370475457689,
0.00907791604178338,0.00910510377824634,0.00940212732898988,0.00946374650435997,
0.00964367022755659,0.00972633861619637,0.00973375433433046,0.00982383413264779,
0.0100505499034029,0.0101833725565308,0.0103747611906094),.UNSPECIFIED.);
#931=B_SPLINE_CURVE_WITH_KNOTS('',3,(#46658,#46659,#46660,#46661,#46662,
#46663,#46664,#46665,#46666,#46667,#46668,#46669,#46670,#46671,#46672,#46673,
#46674,#46675,#46676,#46677,#46678,#46679),.UNSPECIFIED.,.F.,.F.,(4,2,2,
2,2,2,2,2,2,2,4),(-0.516489735213594,-0.403297365402408,-0.304637803925453,
-0.258291991281017,-0.235867650221037,-0.22650069343662,-0.22227817689503,
-0.203792144791807,-0.176538654710716,-0.119127477076588,-5.65372251348784E-7),
 .UNSPECIFIED.);
#932=B_SPLINE_CURVE_WITH_KNOTS('',3,(#46683,#46684,#46685,#46686,#46687,
#46688,#46689,#46690,#46691,#46692,#46693,#46694,#46695,#46696,#46697,#46698,
#46699,#46700,#46701,#46702,#46703,#46704,#46705,#46706,#46707,#46708,#46709,
#46710,#46711,#46712,#46713,#46714,#46715,#46716,#46717,#46718,#46719,#46720,
#46721,#46722,#46723,#46724,#46725,#46726,#46727,#46728,#46729,#46730,#46731,
#46732,#46733,#46734,#46735,#46736,#46737,#46738,#46739,#46740,#46741,#46742,
#46743,#46744,#46745,#46746,#46747,#46748,#46749,#46750,#46751,#46752,#46753,
#46754,#46755,#46756,#46757,#46758,#46759,#46760,#46761,#46762,#46763,#46764,
#46765,#46766,#46767,#46768,#46769,#46770,#46771,#46772,#46773,#46774,#46775,
#46776,#46777,#46778,#46779,#46780,#46781,#46782,#46783,#46784,#46785,#46786,
#46787,#46788,#46789,#46790,#46791,#46792,#46793,#46794,#46795,#46796,#46797,
#46798,#46799,#46800,#46801,#46802,#46803,#46804,#46805,#46806,#46807,#46808,
#46809,#46810,#46811,#46812,#46813,#46814,#46815,#46816,#46817,#46818,#46819,
#46820,#46821,#46822,#46823,#46824,#46825,#46826,#46827,#46828,#46829,#46830,
#46831,#46832,#46833,#46834,#46835,#46836,#46837,#46838,#46839,#46840,#46841,
#46842,#46843,#46844,#46845,#46846,#46847,#46848,#46849,#46850,#46851,#46852,
#46853,#46854,#46855,#46856,#46857,#46858,#46859,#46860,#46861,#46862,#46863,
#46864,#46865,#46866,#46867,#46868,#46869,#46870,#46871,#46872,#46873,#46874,
#46875,#46876,#46877,#46878,#46879,#46880,#46881,#46882,#46883,#46884,#46885,
#46886,#46887,#46888,#46889,#46890,#46891,#46892,#46893,#46894,#46895,#46896,
#46897,#46898,#46899,#46900,#46901,#46902,#46903,#46904,#46905,#46906,#46907,
#46908,#46909,#46910,#46911,#46912,#46913,#46914,#46915,#46916,#46917,#46918,
#46919,#46920,#46921,#46922,#46923,#46924,#46925,#46926,#46927,#46928,#46929,
#46930,#46931,#46932,#46933,#46934,#46935,#46936,#46937,#46938,#46939,#46940,
#46941,#46942,#46943,#46944,#46945,#46946,#46947,#46948,#46949,#46950,#46951,
#46952,#46953,#46954,#46955,#46956,#46957,#46958,#46959,#46960,#46961,#46962,
#46963,#46964,#46965,#46966,#46967,#46968,#46969,#46970,#46971,#46972,#46973,
#46974,#46975,#46976,#46977,#46978,#46979,#46980,#46981,#46982,#46983,#46984,
#46985,#46986,#46987,#46988,#46989,#46990,#46991,#46992,#46993,#46994,#46995,
#46996,#46997,#46998,#46999,#47000,#47001,#47002,#47003,#47004,#47005,#47006,
#47007,#47008,#47009,#47010,#47011,#47012,#47013,#47014,#47015,#47016,#47017,
#47018,#47019,#47020,#47021,#47022,#47023,#47024,#47025),.UNSPECIFIED.,
 .F.,.F.,(4,3,3,3,3,3,3,3,3,3,3,3,3,3,3,3,3,3,3,3,3,3,3,3,3,3,3,3,3,3,3,
3,3,3,3,3,3,3,3,3,3,3,3,3,3,3,3,3,3,3,3,3,3,3,3,3,3,3,3,3,3,3,3,3,3,3,3,
3,3,3,3,3,3,3,3,3,3,3,3,3,3,3,3,3,3,3,3,3,3,3,3,3,3,3,3,3,3,3,3,3,3,3,3,
3,3,3,3,3,3,3,3,3,3,3,4),(0.,0.000559340172070426,0.00056312127745191,0.00111868034414085,
0.00117480882670147,0.00139835043017606,0.00148111639279807,0.00153818547319366,
0.00160810299470246,0.0016343904416067,0.00167802051621126,0.00178762749494104,
0.00223736068828162,0.00239897267727689,0.00279670086035198,0.00300768662511807,
0.00335604103242234,0.00361373793821833,0.00363571111845751,0.00376481945685295,
0.0037755461614751,0.00384029321466327,0.00384546368298389,0.00391538120449268,
0.00391572188407732,0.00421697465550928,0.00447472137656305,0.00481726522761212,
0.00503406154863342,0.00511629473858952,0.00531373163466861,0.00541456290638466,
0.00559340172070379,0.00571204633238695,0.00573323676372139,0.00580315428523019,
0.00583811304598459,0.00586048502912534,0.00587307180673899,0.00600876663145698,
0.00615274189277417,0.00630500853253195,0.00660082053734943,0.00671208206484454,
0.00689619939885552,0.00719113780032637,0.00727142223691492,0.00741125727993251,
0.00748117480144131,0.00748562537787358,0.0075161335621957,0.0075510923229501,
0.0075591756922752,0.00763271703837717,0.0077798197594622,0.00783076240898527,
0.00807404583962471,0.00811043249502045,0.0083682956412184,0.00839010258105563,
0.00894944275312598,0.0089568174998829,0.00908927779614357,0.00910394297613539,
0.00915919531765236,0.00917751112674336,0.00922911283916116,0.00925109949730556,
0.00950878292519633,0.00954566299720578,0.0100681230972667,0.0101357118688264,
0.010627463269337,0.0107268460053846,0.0107672983123546,0.0108372158338634,
0.0108747847708707,0.0109071333553722,0.0110227987810239,0.0111868034414074,
0.0113191040911945,0.0114664735274426,0.0116063085704602,0.0116157576196813,
0.011676226091969,0.011689973073376,0.0117461436134777,0.0117642110435597,
0.0119127713350278,0.0123054837855481,0.0125080251066784,0.0128648239576184,
0.013104832388234,0.0134241641296888,0.0137030875195115,0.0139835043017591,
0.014302741201141,0.0145428444738295,0.0146030956561195,0.0146826795168471,
0.0147533972581463,0.0148225145598647,0.0149038256869558,0.0151021846458999,
0.0155067400228327,0.0156615248179702,0.0161116197724483,0.0162208649900406,
0.0167185606475561,0.016780205162111,0.0173277427187631,0.0173395453341813,
0.0176334296012555,0.0177861596802748,0.0178988855062517),.UNSPECIFIED.);
#933=B_SPLINE_CURVE_WITH_KNOTS('',3,(#47040,#47041,#47042,#47043,#47044,
#47045,#47046,#47047,#47048,#47049,#47050,#47051,#47052,#47053,#47054,#47055,
#47056,#47057,#47058,#47059,#47060,#47061,#47062,#47063,#47064,#47065,#47066,
#47067,#47068,#47069,#47070,#47071,#47072,#47073,#47074,#47075,#47076,#47077,
#47078,#47079,#47080,#47081,#47082,#47083,#47084,#47085,#47086,#47087,#47088,
#47089,#47090,#47091,#47092,#47093,#47094,#47095,#47096,#47097,#47098,#47099,
#47100,#47101,#47102,#47103,#47104,#47105,#47106,#47107,#47108,#47109,#47110,
#47111,#47112,#47113,#47114,#47115,#47116,#47117,#47118,#47119,#47120,#47121,
#47122,#47123,#47124,#47125,#47126,#47127,#47128,#47129,#47130,#47131,#47132,
#47133,#47134,#47135,#47136,#47137,#47138,#47139,#47140,#47141,#47142,#47143,
#47144,#47145,#47146,#47147,#47148,#47149,#47150,#47151,#47152,#47153,#47154,
#47155,#47156,#47157,#47158,#47159,#47160,#47161,#47162,#47163,#47164,#47165,
#47166,#47167,#47168,#47169,#47170,#47171,#47172,#47173,#47174,#47175,#47176,
#47177,#47178,#47179,#47180,#47181,#47182,#47183,#47184,#47185,#47186,#47187,
#47188,#47189,#47190,#47191,#47192,#47193,#47194,#47195,#47196,#47197,#47198,
#47199,#47200,#47201,#47202,#47203,#47204,#47205,#47206,#47207,#47208,#47209,
#47210,#47211,#47212,#47213,#47214,#47215,#47216,#47217,#47218,#47219,#47220,
#47221,#47222,#47223,#47224,#47225,#47226,#47227,#47228,#47229,#47230,#47231,
#47232,#47233,#47234,#47235,#47236,#47237,#47238,#47239,#47240,#47241,#47242,
#47243,#47244,#47245,#47246,#47247,#47248,#47249,#47250,#47251,#47252,#47253,
#47254,#47255,#47256,#47257,#47258,#47259,#47260,#47261,#47262,#47263,#47264,
#47265,#47266,#47267,#47268,#47269,#47270,#47271,#47272,#47273,#47274,#47275,
#47276,#47277,#47278,#47279,#47280,#47281,#47282,#47283,#47284,#47285,#47286,
#47287,#47288,#47289,#47290,#47291,#47292,#47293,#47294,#47295),
 .UNSPECIFIED.,.F.,.F.,(4,3,3,3,3,3,3,3,3,3,3,3,3,3,3,3,3,3,3,3,3,3,3,3,
3,3,3,3,3,3,3,3,3,3,3,3,3,3,3,3,3,3,3,3,3,3,3,3,3,3,3,3,3,3,3,3,3,3,3,3,
3,3,3,3,3,3,3,3,3,3,3,3,3,3,3,3,3,3,3,3,3,3,3,3,3,4),(0.,1.47382713762708E-5,
8.1640167161615E-5,0.000113040897811508,0.000162304556226174,0.00016328033432323,
0.000211569726454149,0.00032656066864646,0.000605462375354082,0.000653121337292909,
0.000979682005939359,0.000998956362101892,0.00130624267458581,0.00139206000816881,
0.00158846721825144,0.00163280334323226,0.00168663405119503,0.00171444351039387,
0.00173570554393496,0.00178475826250593,0.00179608367755548,0.0019593640118787,
0.0021764066902377,0.00228592468052514,0.00256676504196455,0.00261248534917158,
0.00293904601781802,0.00295591148826027,0.00310232635214124,0.00315005096599843,
0.00318396651930285,0.00322478660288365,0.00324700883855564,0.00326560668646445,
0.00334387779966514,0.00359216735511088,0.00373044383356633,0.00391872802375731,
0.00411563875046019,0.00424528869240374,0.00449954862961719,0.00457184936105017,
0.00488223509352117,0.0048984100296966,0.00522497069834303,0.00526373999263159,
0.0053589350810355,0.00538825103266625,0.00545405001538152,0.00555153136698946,
0.00564409445256484,0.00587809203563587,0.00602336155693145,0.00604137236995909,
0.0061180115657291,0.00612301253712069,0.0062046527042823,0.00621259546927448,
0.00640159142864471,0.00653121337292871,0.0067789487108179,0.00685777404157513,
0.00715546455766113,0.00718433471022155,0.00751089537886797,0.00753114977976008,
0.00783745604751438,0.00790600171572738,0.0081640167161608,0.00828000681041783,
0.00846668442947774,0.00849057738480722,0.00855994046092843,0.00857221755196882,
0.00861303763554962,0.00865314855613666,0.00865385771913043,0.00881713805345364,
0.00914369872210006,0.0093982633178075,0.00947025939074649,0.00977046583129307,
0.00979682005939291,0.0101233807280393,0.0101424271025616,0.0104499413966858),
 .UNSPECIFIED.);
#934=B_SPLINE_CURVE_WITH_KNOTS('',3,(#47297,#47298,#47299,#47300,#47301,
#47302,#47303,#47304,#47305,#47306,#47307,#47308,#47309,#47310,#47311,#47312,
#47313,#47314,#47315,#47316,#47317,#47318,#47319,#47320,#47321,#47322,#47323,
#47324,#47325,#47326,#47327,#47328,#47329,#47330,#47331,#47332,#47333,#47334,
#47335,#47336,#47337,#47338,#47339,#47340,#47341,#47342,#47343,#47344,#47345,
#47346,#47347,#47348,#47349,#47350,#47351,#47352,#47353,#47354,#47355,#47356,
#47357,#47358,#47359,#47360,#47361,#47362,#47363,#47364,#47365,#47366,#47367,
#47368,#47369,#47370,#47371,#47372,#47373,#47374,#47375,#47376,#47377,#47378,
#47379,#47380,#47381,#47382,#47383,#47384,#47385,#47386,#47387,#47388,#47389,
#47390,#47391,#47392,#47393,#47394,#47395,#47396,#47397,#47398,#47399,#47400,
#47401,#47402,#47403,#47404,#47405,#47406,#47407,#47408,#47409,#47410,#47411,
#47412,#47413,#47414,#47415,#47416,#47417,#47418,#47419,#47420,#47421,#47422,
#47423,#47424,#47425,#47426,#47427,#47428,#47429,#47430,#47431,#47432,#47433,
#47434,#47435,#47436,#47437,#47438,#47439,#47440,#47441,#47442,#47443,#47444,
#47445,#47446,#47447,#47448,#47449,#47450,#47451,#47452,#47453,#47454,#47455,
#47456,#47457,#47458,#47459,#47460,#47461,#47462,#47463,#47464,#47465,#47466,
#47467,#47468,#47469,#47470,#47471,#47472,#47473,#47474,#47475,#47476,#47477,
#47478,#47479,#47480,#47481,#47482,#47483,#47484,#47485,#47486,#47487,#47488,
#47489,#47490,#47491,#47492,#47493,#47494,#47495,#47496,#47497,#47498,#47499,
#47500,#47501,#47502,#47503,#47504,#47505,#47506,#47507,#47508,#47509,#47510,
#47511,#47512,#47513,#47514,#47515,#47516,#47517,#47518,#47519,#47520,#47521,
#47522,#47523,#47524,#47525,#47526,#47527,#47528,#47529,#47530,#47531,#47532,
#47533,#47534,#47535,#47536,#47537,#47538,#47539,#47540,#47541,#47542,#47543,
#47544,#47545,#47546,#47547,#47548,#47549,#47550,#47551,#47552,#47553,#47554,
#47555,#47556,#47557,#47558,#47559,#47560,#47561,#47562,#47563,#47564,#47565,
#47566,#47567,#47568,#47569,#47570,#47571,#47572,#47573,#47574,#47575,#47576,
#47577,#47578,#47579,#47580,#47581,#47582,#47583,#47584,#47585,#47586,#47587,
#47588,#47589,#47590,#47591,#47592,#47593,#47594,#47595,#47596,#47597,#47598,
#47599,#47600,#47601,#47602,#47603,#47604,#47605,#47606,#47607,#47608,#47609,
#47610,#47611,#47612,#47613,#47614,#47615,#47616,#47617,#47618,#47619,#47620,
#47621,#47622,#47623,#47624,#47625,#47626,#47627,#47628,#47629,#47630,#47631,
#47632,#47633,#47634,#47635,#47636,#47637,#47638,#47639,#47640,#47641,#47642,
#47643,#47644,#47645,#47646,#47647,#47648,#47649,#47650,#47651,#47652,#47653,
#47654,#47655,#47656,#47657,#47658,#47659,#47660,#47661,#47662,#47663,#47664,
#47665,#47666,#47667,#47668,#47669,#47670,#47671,#47672,#47673,#47674,#47675,
#47676,#47677,#47678,#47679,#47680,#47681,#47682,#47683,#47684,#47685,#47686,
#47687,#47688,#47689,#47690,#47691,#47692,#47693,#47694,#47695,#47696,#47697,
#47698,#47699,#47700,#47701,#47702,#47703,#47704,#47705,#47706,#47707,#47708,
#47709,#47710,#47711,#47712,#47713,#47714,#47715,#47716,#47717,#47718,#47719,
#47720,#47721,#47722,#47723,#47724,#47725,#47726,#47727,#47728,#47729,#47730,
#47731,#47732,#47733,#47734,#47735,#47736,#47737,#47738,#47739,#47740,#47741,
#47742,#47743,#47744,#47745,#47746,#47747,#47748,#47749,#47750,#47751,#47752,
#47753,#47754,#47755,#47756,#47757,#47758,#47759,#47760,#47761,#47762,#47763,
#47764,#47765,#47766,#47767,#47768,#47769,#47770,#47771,#47772,#47773,#47774,
#47775,#47776,#47777,#47778,#47779,#47780,#47781,#47782,#47783,#47784,#47785,
#47786,#47787,#47788,#47789,#47790,#47791,#47792,#47793,#47794,#47795,#47796,
#47797,#47798,#47799,#47800,#47801,#47802,#47803,#47804,#47805,#47806,#47807,
#47808,#47809,#47810,#47811,#47812,#47813,#47814,#47815,#47816,#47817,#47818,
#47819,#47820,#47821,#47822,#47823,#47824,#47825,#47826,#47827,#47828,#47829,
#47830,#47831,#47832,#47833,#47834,#47835,#47836,#47837,#47838,#47839,#47840,
#47841,#47842,#47843,#47844,#47845,#47846,#47847,#47848,#47849,#47850,#47851,
#47852,#47853,#47854,#47855,#47856,#47857,#47858,#47859,#47860,#47861,#47862,
#47863,#47864,#47865,#47866,#47867,#47868,#47869,#47870,#47871,#47872,#47873,
#47874,#47875,#47876,#47877,#47878,#47879,#47880,#47881,#47882,#47883,#47884,
#47885,#47886,#47887,#47888,#47889,#47890,#47891,#47892,#47893,#47894,#47895,
#47896,#47897,#47898,#47899,#47900,#47901,#47902,#47903,#47904,#47905,#47906,
#47907,#47908,#47909,#47910,#47911,#47912,#47913,#47914,#47915,#47916,#47917,
#47918,#47919,#47920,#47921,#47922,#47923,#47924,#47925,#47926,#47927,#47928,
#47929,#47930,#47931,#47932,#47933,#47934,#47935,#47936,#47937,#47938,#47939,
#47940,#47941,#47942,#47943,#47944,#47945,#47946,#47947,#47948,#47949,#47950,
#47951,#47952,#47953,#47954,#47955,#47956,#47957,#47958,#47959,#47960,#47961,
#47962,#47963,#47964,#47965,#47966,#47967,#47968,#47969,#47970,#47971,#47972,
#47973,#47974,#47975,#47976,#47977,#47978,#47979,#47980,#47981,#47982,#47983,
#47984,#47985,#47986,#47987,#47988,#47989,#47990,#47991,#47992,#47993,#47994,
#47995,#47996,#47997,#47998,#47999,#48000,#48001,#48002,#48003,#48004,#48005,
#48006,#48007,#48008,#48009,#48010,#48011,#48012,#48013,#48014,#48015,#48016,
#48017,#48018,#48019,#48020,#48021,#48022,#48023,#48024,#48025,#48026,#48027,
#48028,#48029,#48030,#48031,#48032,#48033,#48034,#48035,#48036,#48037,#48038,
#48039,#48040,#48041,#48042,#48043,#48044,#48045,#48046,#48047,#48048,#48049,
#48050,#48051,#48052,#48053,#48054,#48055,#48056,#48057,#48058,#48059,#48060,
#48061,#48062,#48063,#48064,#48065,#48066,#48067,#48068,#48069,#48070,#48071,
#48072,#48073,#48074,#48075,#48076,#48077,#48078,#48079,#48080,#48081,#48082,
#48083,#48084,#48085,#48086,#48087,#48088,#48089,#48090,#48091,#48092,#48093,
#48094,#48095,#48096,#48097,#48098,#48099,#48100,#48101,#48102,#48103,#48104,
#48105,#48106,#48107,#48108,#48109,#48110,#48111,#48112,#48113,#48114,#48115,
#48116,#48117,#48118,#48119,#48120,#48121,#48122,#48123,#48124,#48125,#48126,
#48127,#48128,#48129,#48130,#48131,#48132,#48133,#48134,#48135,#48136,#48137,
#48138,#48139,#48140,#48141,#48142,#48143,#48144,#48145,#48146,#48147,#48148,
#48149,#48150,#48151,#48152,#48153,#48154,#48155,#48156,#48157,#48158,#48159,
#48160,#48161,#48162,#48163,#48164,#48165,#48166,#48167,#48168,#48169,#48170,
#48171,#48172,#48173,#48174,#48175,#48176,#48177,#48178,#48179,#48180,#48181,
#48182,#48183,#48184,#48185,#48186,#48187,#48188,#48189,#48190,#48191,#48192,
#48193,#48194),.UNSPECIFIED.,.F.,.F.,(4,3,3,3,3,3,3,3,3,3,3,3,3,3,3,3,3,
3,3,3,3,3,3,3,3,3,3,3,3,3,3,3,3,3,3,3,3,3,3,3,3,3,3,3,3,3,3,3,3,3,3,3,3,
3,3,3,3,3,3,3,3,3,3,3,3,3,3,3,3,3,3,3,3,3,3,3,3,3,3,3,3,3,3,3,3,3,3,3,3,
3,3,3,3,3,3,3,3,3,3,3,3,3,3,3,3,3,3,3,3,3,3,3,3,3,3,3,3,3,3,3,3,3,3,3,3,
3,3,3,3,3,3,3,3,3,3,3,3,3,3,3,3,3,3,3,3,3,3,3,3,3,3,3,3,3,3,3,3,3,3,3,3,
3,3,3,3,3,3,3,3,3,3,3,3,3,3,3,3,3,3,3,3,3,3,3,3,3,3,3,3,3,3,3,3,3,3,3,3,
3,3,3,3,3,3,3,3,3,3,3,3,3,3,3,3,3,3,3,3,3,3,3,3,3,3,3,3,3,3,3,3,3,3,3,3,
3,3,3,3,3,3,3,3,3,3,3,3,3,3,3,3,3,3,3,3,3,3,3,3,3,3,3,3,3,3,3,3,3,3,3,3,
3,3,3,3,3,3,3,3,3,3,3,3,3,3,3,3,3,3,3,3,3,3,3,3,3,3,3,3,3,3,4),(1.35130087435845E-15,
0.000427333961361783,0.000452399919294745,0.000904799838588138,0.00135719975788153,
0.00137425621759972,0.00180959967717493,0.00185103340846359,0.00203579963682163,
0.00209026025768216,0.00214889961664498,0.00221006611721062,0.00226199959646833,
0.00232994525493375,0.00271439951576174,0.00316679943505514,0.00329151263938818,
0.00361919935434855,0.00407159927364195,0.00425769262375026,0.00452399919293536,
0.004742581270083,0.00497639911222876,0.00522872838875649,0.00542879903152217,
0.00547229268389153,0.00559420535263831,0.00565499899116887,0.00571154898108054,
0.00571619320255349,0.00576809897099221,0.00588119895081556,0.00620467062394714,
0.006333598870109,0.00678599878940244,0.00718388137198869,0.00723839870869588,
0.00769079862798932,0.00814319854728276,0.00816621717001466,0.00841231680488797,
0.0085354464035452,0.0085955984665762,0.00865214845648787,0.00865861451015506,
0.00870869844639954,0.00882179842622286,0.00904799838586948,0.00915120921437489,
0.00950039830516272,0.00995279822445595,0.0101355902621457,0.0104051981437492,
0.0108575980630424,0.0111189149255724,0.0113099979823357,0.0113645824124405,
0.0114873943974255,0.0115361979419823,0.0115927479318939,0.011610181923162,
0.0116492979218056,0.0117623979016288,0.0121006755023117,0.012214797820922,
0.0126671977402151,0.0130783720079958,0.0131195976595082,0.0135719975788014,
0.0140243974980945,0.0140519386107737,0.0142505974577411,0.0142947100135889,
0.0143636974375644,0.0144159988972164,0.0144767974173877,0.014537210921105,
0.0149291973366808,0.015021231024896,0.015381597255974,0.0158339971752671,
0.0159855037164582,0.0162863970945603,0.0167387970138534,0.0169449728021871,
0.0171911969331465,0.0174173968927931,0.0174229451715688,0.0175304968726164,
0.017542255502331,0.0176435968524397,0.017661493031398,0.0178997543853799,
0.0180959967717328,0.0185483966910259,0.0188499922611146,0.019000796610319,
0.0194531965296122,0.0197958007633236,0.0199055964489053,0.0203579963681984,
0.0207371351958851,0.0208103962874915,0.0209234962673148,0.0209717468832201,
0.0210365962471381,0.0210889332304238,0.0212060192761904,0.0212627962067846,
0.0216733657645927,0.0217151961260777,0.0221675960453708,0.0226033011190297,
0.0226199959646638,0.0230723958839569,0.02352479580325,0.0235268185559895,
0.0236378957830733,0.0236944457729849,0.0237509957628965,0.0239771957225431,
0.0239870003329634,0.0242033956821896,0.0242182941868268,0.0243164956620129,
0.0243343114281531,0.0244295956418361,0.0244504496828121,0.0248819955611292,
0.0249151395533867,0.0253343954804223,0.0253800487757404,0.0257867953997154,
0.0258451744241752,0.0262391953190085,0.0263105151891527,0.0266915952383015,
0.0267760697666888,0.0270089229795263,0.0271253799242098,0.0271439951575946,
0.0272005451475063,0.0272418465555986,0.0272570951374179,0.0273701951172412,
0.0275963950768877,0.0277082392254462,0.0280487949961807,0.0281755795546116,
0.0285011949154738,0.0289535948347668,0.0291130107793379,0.0294059947540599,
0.029858394673353,0.0300540403436757,0.0302898597551073,0.030310794592646,
0.0304078553652295,0.0304238945724693,0.0305259116030602,0.0305369945522925,
0.030763194511939,0.0309988867607011,0.031215594431232,0.031667994350525,
0.0319483580710528,0.032120394269818,0.0325727941891111,0.032902491485125,
0.0330251941084041,0.0333813343952388,0.0334775940276971,0.0335906940075203,
0.0336212117526858,0.033647243997432,0.0337037939873436,0.0337412639505102,
0.0338613888123318,0.0339299939469901,0.0343823938662831,0.0348248994526247,
0.0348347937855762,0.0352871937048692,0.0357395936241622,0.035792980893805,
0.0361919935434553,0.0362788063756478,0.0366443934627483,0.0367658817816997,
0.0370967933820413,0.0372098933618646,0.0372542658321182,0.0373229933416879,
0.03749888830684,0.0375491933013344,0.0377436804253305,0.0380015932206275,
0.0384539931399206,0.0387245633800817,0.0389063930592137,0.0393587929785068,
0.0397082869870636,0.0398111928977999,0.0399546805469956,0.0400373928574464,
0.0400779528497158,0.0401504928372697,0.040201261975522,0.0402070428271813,
0.040263592817093,0.0406943510040045,0.0407159927363861,0.0411683926556793,
0.0416207925749724,0.0416794507159706,0.0420731924942656,0.0425255924135587,
0.0426631474812632,0.0429088555037357,0.0429779923328519,0.0430316764271511,
0.0430910923126752,0.0431544637395062,0.0432041922924984,0.0434303922521449,
0.043644905175834,0.043882792171438,0.0443351920907311,0.0446223981991244,
0.0447875920100241,0.0452399919293172,0.0455956456638855,0.0456923918486102,
0.0458054918284335,0.0458383181596209,0.0459185918082567,0.0459595566553906,
0.0460807118303458,0.0461447917679033,0.046564511684252,0.0465971916871963,
0.0470495916064894,0.0475019915257824,0.0475283529694127,0.0479543914450755,
0.0484067913643685,0.0484873842239486,0.0488591912836615,0.0489651292319899,
0.0489722912634848,0.0490843814225022,0.0490853912433081,0.0492035625454086,
0.0493115912029546,0.0494417143659409,0.0497639911222476,0.0502163910415407,
0.0503915617699481,0.0506687909608337,0.0511211908801268,0.0513370475099055,
0.0515735907994198,0.0520259907187128,0.0522781180849262,0.0524783906380059,
0.052512674995964,0.0525349406279175,0.0525914906178291,0.0526298364378429,
0.0527045905976524,0.0527469056214694,0.0529307905572989,0.0532142274876769,
0.0533831904765919,0.053835590395885,0.0541443207096413,0.054287990315178,
0.054740390234471,0.0550682858845152,0.0551927901537641,0.0552493401436757,
0.0553058901335873,0.0554189901134106,0.055528729013877,0.0556451900730571,
0.0557582900528804,0.0557601597824457,0.0558181936376942,0.0558713900327036,
0.0558762162462772,0.055992094547227,0.0560975899923501,0.0564548298442276,
0.0565499899116432,0.0569164222442635,0.0570023898309362,0.0573768793379545,
0.0574547897502292,0.057836211703915,0.0579071896695223),.UNSPECIFIED.);
#935=B_SPLINE_CURVE_WITH_KNOTS('',3,(#48196,#48197,#48198,#48199,#48200,
#48201,#48202,#48203,#48204,#48205,#48206,#48207,#48208,#48209,#48210,#48211,
#48212,#48213,#48214,#48215,#48216,#48217,#48218,#48219,#48220,#48221,#48222,
#48223,#48224,#48225,#48226,#48227),.UNSPECIFIED.,.F.,.F.,(4,1,1,1,2,2,
2,1,2,2,2,1,1,1,1,1,2,2,1,1,1,4),(0.00150858273324743,0.00182098751393329,
0.00213339229461915,0.00244579707530502,0.00275820185599088,0.00283630305116235,
0.00291440424633382,0.00307060663667675,0.00338301141736263,0.00353921380770556,
0.0036954161980485,0.00400782097873437,0.00432022575942025,0.00463263054010612,
0.00494503532079199,0.00525744010147787,0.00556984488216374,0.00564794607733521,
0.00572604727250669,0.00588224966284963,0.00619465444353553,0.00650705856419875),
 .UNSPECIFIED.);
#936=B_SPLINE_CURVE_WITH_KNOTS('',3,(#48231,#48232,#48233,#48234,#48235,
#48236,#48237,#48238,#48239,#48240,#48241,#48242,#48243,#48244,#48245,#48246,
#48247,#48248,#48249,#48250,#48251,#48252,#48253,#48254,#48255,#48256,#48257,
#48258,#48259,#48260,#48261,#48262,#48263,#48264,#48265,#48266,#48267,#48268,
#48269,#48270,#48271,#48272,#48273,#48274,#48275,#48276,#48277,#48278,#48279,
#48280,#48281,#48282,#48283,#48284,#48285,#48286,#48287,#48288,#48289,#48290,
#48291,#48292,#48293,#48294,#48295,#48296,#48297,#48298,#48299,#48300,#48301,
#48302,#48303,#48304,#48305,#48306,#48307,#48308,#48309,#48310,#48311,#48312,
#48313,#48314,#48315,#48316,#48317,#48318,#48319,#48320,#48321,#48322,#48323,
#48324,#48325,#48326,#48327,#48328,#48329,#48330,#48331,#48332,#48333,#48334,
#48335,#48336,#48337,#48338,#48339,#48340,#48341),.UNSPECIFIED.,.F.,.F.,
(4,2,2,2,1,1,1,1,2,1,2,2,1,1,1,1,1,2,2,1,1,1,1,2,2,2,1,1,1,2,2,2,1,1,1,
1,1,2,2,1,1,1,1,1,1,2,2,2,1,2,2,2,1,1,1,1,1,2,2,1,1,1,1,1,2,1,2,2,1,1,1,
1,2,2,1,1,1,1,1,4),(0.,0.000327684171192303,0.000409605213990379,0.000491526256788455,
0.000655368342384606,0.000983052513576909,0.00131073668476921,0.00163842085596152,
0.00196610502715382,0.00212994711274997,0.002170907634149,0.00221186815554804,
0.0022937891983461,0.0026214733695384,0.00294915754073069,0.00327684171192298,
0.00360452588311527,0.00393221005430756,0.00401413109710564,0.00409605213990371,
0.00425989422549987,0.00458757839669218,0.0049152625678845,0.00524294673907681,
0.00540678882467297,0.00557063091026913,0.00589831508146146,0.00622599925265378,
0.00655368342384611,0.00688136759503843,0.0070452096806346,0.00712713072343267,
0.00720905176623075,0.00753673593742304,0.00786442010861533,0.00819210427980761,
0.0085197884509999,0.00884747262219219,0.00892939366499025,0.00901131470778832,
0.00917515679338446,0.00950284096457672,0.00983052513576899,0.0101582093069613,
0.0104858934781535,0.0108135776493458,0.0108954986921438,0.0109774197349419,
0.011141261820538,0.0114689459917303,0.0116327880773264,0.0117147091201244,
0.0117966301629225,0.0121243143341147,0.012451998505307,0.0127796826764992,
0.0131073668476915,0.0134350510188837,0.0135169720616818,0.0135988931044798,
0.0137627351900759,0.0140904193612682,0.0144181035324604,0.0147457877036527,
0.0150734718748449,0.015237313960441,0.0153192350032391,0.0154011560460371,
0.0157288402172293,0.0160565243884215,0.0163842085596138,0.016711892730806,
0.0170395769019982,0.0170805374233972,0.0171214979447962,0.0172034189875943,
0.0173672610731904,0.0176949452443827,0.018022629415575,0.0180959256708578),
 .UNSPECIFIED.);
#937=B_SPLINE_CURVE_WITH_KNOTS('',3,(#48343,#48344,#48345,#48346,#48347,
#48348,#48349,#48350,#48351,#48352,#48353,#48354,#48355,#48356,#48357,#48358,
#48359,#48360,#48361,#48362,#48363,#48364,#48365),.UNSPECIFIED.,.F.,.F.,
(4,1,2,1,2,2,1,1,1,1,1,2,2,2,4),(0.0180959256708578,0.0183503135867672,
0.0186779977579595,0.0188418398435556,0.0188828003649547,0.0189237608863537,
0.0190056819291518,0.019333366100344,0.0196610502715362,0.0199887344427285,
0.0203164186139207,0.020644102785113,0.020726023827911,0.0208079448707091,
0.0209717869563052),.UNSPECIFIED.);
#938=B_SPLINE_CURVE_WITH_KNOTS('',3,(#48373,#48374,#48375,#48376,#48377,
#48378,#48379,#48380,#48381,#48382,#48383,#48384,#48385,#48386,#48387,#48388,
#48389,#48390,#48391,#48392,#48393,#48394,#48395,#48396),.UNSPECIFIED.,
 .F.,.F.,(4,2,2,2,1,1,1,1,1,2,2,2,1,2,4),(0.,0.000404302057260319,0.000606453085890479,
0.000656990843048018,0.000707528600205558,0.000808604114520648,0.00121290617178103,
0.00161720822904141,0.00202151028630179,0.00242581234356217,0.00247635010071971,
0.00252688785787726,0.00262796337219236,0.00283011440082255,0.00287050024670353),
 .UNSPECIFIED.);
#939=B_SPLINE_CURVE_WITH_KNOTS('',3,(#48402,#48403,#48404,#48405,#48406,
#48407,#48408,#48409,#48410,#48411,#48412,#48413,#48414,#48415,#48416,#48417,
#48418,#48419,#48420,#48421,#48422,#48423,#48424,#48425,#48426,#48427,#48428,
#48429,#48430,#48431,#48432,#48433,#48434,#48435,#48436,#48437,#48438,#48439,
#48440,#48441,#48442,#48443,#48444,#48445,#48446,#48447,#48448,#48449,#48450,
#48451,#48452,#48453,#48454,#48455,#48456,#48457,#48458,#48459,#48460,#48461,
#48462,#48463,#48464,#48465,#48466,#48467,#48468,#48469,#48470,#48471,#48472,
#48473,#48474,#48475,#48476,#48477,#48478,#48479,#48480,#48481,#48482,#48483,
#48484,#48485,#48486,#48487,#48488,#48489,#48490,#48491,#48492,#48493,#48494,
#48495,#48496,#48497,#48498,#48499,#48500,#48501,#48502,#48503,#48504,#48505,
#48506,#48507,#48508,#48509,#48510,#48511,#48512,#48513,#48514,#48515,#48516,
#48517,#48518,#48519,#48520,#48521,#48522,#48523,#48524,#48525,#48526,#48527,
#48528,#48529,#48530,#48531,#48532,#48533,#48534,#48535,#48536,#48537,#48538,
#48539,#48540,#48541,#48542,#48543,#48544,#48545,#48546,#48547,#48548,#48549,
#48550,#48551,#48552,#48553,#48554,#48555,#48556,#48557,#48558,#48559,#48560,
#48561,#48562,#48563,#48564),.UNSPECIFIED.,.F.,.F.,(4,3,3,3,3,3,3,3,3,3,
3,3,3,3,3,3,3,3,3,3,3,3,3,3,3,3,3,3,3,3,3,3,3,3,3,3,3,3,3,3,3,3,3,3,3,3,
3,3,3,3,3,3,3,3,4),(0.,3.18639464890314E-5,6.37278929780629E-5,6.41210145326926E-5,
0.000127455785956126,0.000128345084208553,0.000254911571912252,0.000256986082187868,
0.00031863946489032,0.000321403032292237,0.000350503411379359,0.000353635933676641,
0.000382367357868398,0.000385879972497687,0.000509823143824565,0.00051482305046768,
0.000637278929780732,0.00064371589233994,0.000675940606633055,0.000701006822758811,
0.000708139232281018,0.000764734715736889,0.000772510059645793,0.000892190501693046,
0.000900992059381932,0.0010196462876492,0.00102913438127321,0.00105151023413824,
0.00106111543219135,0.00108337418062729,0.00109306546511644,0.00114710207360537,
0.00115687341539025,0.00127455785956153,0.00128412906516313,0.0013382857525396,
0.0013475774277107,0.00137014969902864,0.00137925494612773,0.00138608167227316,
0.00140201364551768,0.00141090288465876,0.00152946943147388,0.00153723730022466,
0.00165692521743007,0.00166315794950942,0.00168878916391913,0.00169457239304465,
0.00172065311040818,0.001725963985598,0.00178438100338628,0.00178871072439317,
0.0019118367893425,0.00191408283353941,0.00203929257529871),
 .UNSPECIFIED.);
#940=B_SPLINE_CURVE_WITH_KNOTS('',3,(#48568,#48569,#48570,#48571,#48572,
#48573,#48574,#48575,#48576,#48577,#48578,#48579,#48580,#48581,#48582,#48583,
#48584,#48585,#48586,#48587,#48588,#48589,#48590,#48591,#48592,#48593,#48594,
#48595,#48596,#48597,#48598,#48599,#48600,#48601,#48602,#48603,#48604,#48605,
#48606,#48607,#48608,#48609,#48610,#48611,#48612,#48613,#48614,#48615,#48616,
#48617,#48618,#48619,#48620,#48621,#48622,#48623,#48624,#48625,#48626,#48627,
#48628,#48629,#48630,#48631,#48632,#48633,#48634,#48635,#48636,#48637,#48638,
#48639,#48640,#48641,#48642,#48643,#48644,#48645,#48646,#48647,#48648,#48649,
#48650,#48651,#48652,#48653,#48654,#48655,#48656,#48657,#48658,#48659,#48660,
#48661,#48662,#48663,#48664,#48665,#48666,#48667,#48668,#48669,#48670,#48671,
#48672,#48673,#48674,#48675,#48676,#48677,#48678,#48679,#48680,#48681,#48682,
#48683,#48684,#48685,#48686,#48687,#48688,#48689,#48690,#48691,#48692,#48693,
#48694,#48695,#48696,#48697,#48698,#48699,#48700,#48701,#48702,#48703,#48704,
#48705,#48706,#48707,#48708,#48709,#48710,#48711,#48712,#48713,#48714,#48715,
#48716,#48717,#48718,#48719,#48720,#48721,#48722,#48723,#48724,#48725,#48726,
#48727,#48728,#48729,#48730,#48731,#48732,#48733,#48734,#48735,#48736,#48737,
#48738,#48739,#48740,#48741,#48742,#48743,#48744,#48745,#48746,#48747,#48748,
#48749,#48750,#48751,#48752,#48753,#48754,#48755,#48756,#48757,#48758,#48759,
#48760,#48761,#48762,#48763,#48764,#48765,#48766,#48767,#48768,#48769,#48770,
#48771,#48772,#48773,#48774,#48775,#48776,#48777,#48778,#48779,#48780,#48781,
#48782,#48783,#48784,#48785,#48786,#48787,#48788,#48789,#48790,#48791,#48792,
#48793,#48794,#48795,#48796,#48797,#48798,#48799,#48800,#48801,#48802,#48803,
#48804,#48805,#48806,#48807,#48808,#48809,#48810,#48811,#48812,#48813,#48814,
#48815,#48816,#48817,#48818,#48819,#48820,#48821,#48822,#48823,#48824,#48825,
#48826,#48827,#48828,#48829,#48830,#48831,#48832,#48833,#48834,#48835,#48836,
#48837,#48838,#48839,#48840,#48841,#48842,#48843,#48844,#48845,#48846,#48847,
#48848,#48849,#48850,#48851,#48852,#48853,#48854,#48855,#48856,#48857,#48858,
#48859,#48860,#48861,#48862,#48863,#48864,#48865,#48866,#48867,#48868,#48869,
#48870,#48871,#48872,#48873,#48874,#48875,#48876,#48877,#48878,#48879,#48880,
#48881,#48882,#48883,#48884,#48885,#48886,#48887,#48888,#48889,#48890,#48891,
#48892,#48893,#48894,#48895,#48896,#48897,#48898,#48899,#48900,#48901,#48902,
#48903,#48904),.UNSPECIFIED.,.F.,.F.,(4,3,3,3,3,3,3,3,3,3,3,3,3,3,3,3,3,
3,3,3,3,3,3,3,3,3,3,3,3,3,3,3,3,3,3,3,3,3,3,3,3,3,3,3,3,3,3,3,3,3,3,3,3,
3,3,3,3,3,3,3,3,3,3,3,3,3,3,3,3,3,3,3,3,3,3,3,3,3,3,3,3,3,3,3,3,3,3,3,3,
3,3,3,3,3,3,3,3,3,3,3,3,3,3,3,3,3,3,3,3,3,3,3,4),(0.000508896922368124,
0.00062679268456143,0.000694215802633637,0.000722273925456762,0.000770115844337078,
0.000786875242766394,0.000817979061112908,0.00087953468289915,0.00119981935441286,
0.00125017244343018,0.00157976306645661,0.0016208102039612,0.00195781302661255,
0.00199144796449223,0.00200493413523007,0.00203777768455861,0.00205203895394171,
0.00208410740462498,0.00214614867439737,0.00217676684475773,0.00233394447481585,
0.00236208572502323,0.00270788036409555,0.00273272348555424,0.00307964429810653,
0.00310336124608524,0.00326471182245848,0.00328868012635075,0.00331089450480051,
0.00333500984641712,0.00335704244288744,0.00338133956648349,0.00344925827006305,
0.00347399900661624,0.00381721458198522,0.00384463676714722,0.00418375979341684,
0.0042152745276782,0.00454893518005286,0.00458591228820918,0.00473101305800698,
0.00477123116847467,0.00477647916606545,0.00481756088854104,0.00482192941622211,
0.00486389060860741,0.0049128277143484,0.00495655004874015,0.00527642614332629,
0.00532718780927112,0.00564003173827683,0.00569782556980208,0.00600364422750113,
0.00606846333033304,0.00618545305026818,0.00625378221059853,0.0062763590005516,
0.00632181397973453,0.00634644165073127,0.00636726387109635,0.00643910109086401,
0.00673150520028908,0.00680973885139497,0.00709682934653332,0.00718037661192593,
0.00746321783764368,0.0075510143724569,0.00773633325272238,0.00782899269285512,
0.00783068046334138,0.00787532241292148,0.00792165213298785,0.00792272840334262,
0.00801488016841674,0.00819949185806941,0.00829228989351877,0.00856996656715454,
0.00866292765404969,0.00894215245343001,0.00903356541458061,0.00912622485471334,
0.00912891711519763,0.0091725545747797,0.00921888429484607,0.00922247490999389,
0.00931615226136386,0.00940420317511152,0.00969206179812406,0.00977484093564244,
0.0100699886879928,0.0101454786961734,0.0101648047219716,0.0102122670821918,
0.0102381381363061,0.0102597607703787,0.0102844678563724,0.0103307975764388,
0.0104499952267052,0.0105161164567042,0.0108316606729338,0.0108867542172351,
0.0112149921303994,0.011257391977766,0.0112630319454068,0.0113110990680315,
0.0113500514178987,0.0114072584462233,0.0114427108580314,0.0115996012232503,
0.0116280297382968,0.0119843864839696,0.0119986674988277,0.0123693052593585),
 .UNSPECIFIED.);
#941=B_SPLINE_CURVE_WITH_KNOTS('',3,(#48913,#48914,#48915,#48916,#48917,
#48918,#48919,#48920,#48921,#48922,#48923,#48924,#48925,#48926,#48927,#48928,
#48929,#48930,#48931,#48932,#48933,#48934,#48935,#48936,#48937,#48938,#48939,
#48940,#48941,#48942,#48943,#48944,#48945,#48946,#48947,#48948,#48949,#48950,
#48951,#48952,#48953,#48954,#48955,#48956,#48957,#48958,#48959,#48960,#48961,
#48962,#48963,#48964,#48965,#48966,#48967,#48968,#48969,#48970,#48971,#48972,
#48973,#48974,#48975,#48976,#48977,#48978,#48979,#48980,#48981,#48982,#48983,
#48984,#48985,#48986,#48987,#48988,#48989,#48990,#48991,#48992,#48993,#48994,
#48995,#48996,#48997,#48998,#48999,#49000,#49001,#49002,#49003,#49004,#49005,
#49006,#49007,#49008,#49009,#49010,#49011,#49012,#49013,#49014,#49015,#49016,
#49017,#49018,#49019,#49020,#49021,#49022,#49023,#49024,#49025,#49026,#49027,
#49028,#49029,#49030,#49031,#49032,#49033,#49034,#49035,#49036,#49037,#49038,
#49039,#49040,#49041,#49042),.UNSPECIFIED.,.F.,.F.,(4,3,3,3,3,3,3,3,3,3,
3,3,3,3,3,3,3,3,3,3,3,3,3,3,3,3,3,3,3,3,3,3,3,3,3,3,3,3,3,3,3,3,3,4),(0.,
0.000143006486471262,0.000286213476805868,0.000357892947021547,0.00036795089748439,
0.00039375248651578,0.00040474598723283,0.000429627568206775,0.00044154107698127,
0.000573487553939991,0.00058872143597501,0.000717955417591896,0.00073590179496875,
0.000863039500904423,0.000883082153962491,0.000899407029589682,0.000919877243710927,
0.000935823910690361,0.000956672333459362,0.00100881580072779,0.00103026251295622,
0.00115543610824654,0.00117744287194994,0.0013029129807526,0.00132462323094365,
0.00136141832069209,0.00137697769414036,0.00139821341044052,0.00141409436919456,
0.00145125851741666,0.00147180358993741,0.00160037565935921,0.00161898394893119,
0.00175023704203193,0.00176616430792498,0.00182545039553862,0.00183975448742187,
0.00186312708189405,0.0018765495771703,0.00190084390658505,0.00191334466691873,
0.00205189593230952,0.00220324218187337,0.00235488574389977),
 .UNSPECIFIED.);
#942=B_SPLINE_CURVE_WITH_KNOTS('',3,(#49048,#49049,#49050,#49051,#49052,
#49053,#49054,#49055,#49056,#49057,#49058,#49059,#49060,#49061,#49062,#49063,
#49064,#49065,#49066,#49067,#49068,#49069,#49070,#49071,#49072,#49073,#49074,
#49075,#49076,#49077,#49078,#49079,#49080,#49081,#49082,#49083,#49084,#49085,
#49086,#49087,#49088,#49089,#49090,#49091,#49092,#49093,#49094,#49095,#49096,
#49097,#49098,#49099,#49100,#49101,#49102,#49103,#49104,#49105,#49106,#49107,
#49108,#49109,#49110,#49111,#49112,#49113,#49114,#49115,#49116,#49117,#49118,
#49119,#49120,#49121,#49122,#49123,#49124,#49125,#49126,#49127,#49128,#49129,
#49130,#49131,#49132,#49133,#49134,#49135,#49136,#49137,#49138,#49139,#49140,
#49141,#49142,#49143,#49144,#49145,#49146,#49147,#49148,#49149,#49150,#49151,
#49152,#49153,#49154,#49155,#49156,#49157,#49158,#49159,#49160,#49161,#49162,
#49163,#49164,#49165,#49166,#49167,#49168,#49169,#49170,#49171,#49172,#49173,
#49174,#49175,#49176,#49177,#49178,#49179,#49180,#49181,#49182,#49183,#49184,
#49185,#49186,#49187,#49188,#49189,#49190,#49191,#49192,#49193,#49194,#49195,
#49196,#49197,#49198,#49199,#49200,#49201,#49202,#49203,#49204,#49205,#49206,
#49207,#49208,#49209,#49210,#49211,#49212,#49213,#49214,#49215,#49216,#49217,
#49218,#49219,#49220,#49221,#49222,#49223,#49224,#49225,#49226,#49227,#49228,
#49229,#49230,#49231,#49232,#49233,#49234,#49235,#49236,#49237,#49238,#49239,
#49240,#49241,#49242,#49243,#49244,#49245,#49246,#49247,#49248,#49249,#49250,
#49251,#49252,#49253,#49254,#49255,#49256,#49257,#49258,#49259,#49260,#49261,
#49262,#49263,#49264,#49265,#49266,#49267,#49268,#49269,#49270,#49271,#49272,
#49273,#49274,#49275,#49276,#49277,#49278,#49279,#49280,#49281,#49282,#49283,
#49284,#49285,#49286,#49287,#49288,#49289,#49290,#49291,#49292,#49293,#49294,
#49295,#49296,#49297,#49298,#49299,#49300,#49301,#49302,#49303,#49304,#49305,
#49306,#49307,#49308,#49309,#49310,#49311,#49312,#49313,#49314,#49315,#49316,
#49317,#49318,#49319,#49320,#49321,#49322,#49323,#49324,#49325,#49326,#49327,
#49328,#49329,#49330,#49331,#49332,#49333,#49334,#49335,#49336,#49337,#49338,
#49339,#49340,#49341,#49342,#49343,#49344,#49345,#49346,#49347,#49348,#49349,
#49350,#49351,#49352,#49353,#49354,#49355,#49356,#49357,#49358,#49359,#49360,
#49361,#49362,#49363,#49364,#49365,#49366,#49367,#49368,#49369,#49370,#49371,
#49372,#49373,#49374,#49375,#49376,#49377,#49378,#49379,#49380,#49381,#49382,
#49383,#49384,#49385,#49386,#49387,#49388,#49389,#49390,#49391,#49392,#49393,
#49394,#49395,#49396,#49397,#49398,#49399,#49400,#49401,#49402,#49403,#49404,
#49405,#49406,#49407,#49408,#49409,#49410,#49411,#49412,#49413,#49414,#49415,
#49416,#49417,#49418,#49419,#49420,#49421,#49422,#49423,#49424,#49425,#49426,
#49427,#49428,#49429,#49430,#49431,#49432,#49433,#49434,#49435,#49436,#49437,
#49438,#49439,#49440,#49441,#49442,#49443,#49444,#49445,#49446,#49447,#49448,
#49449,#49450,#49451,#49452,#49453,#49454,#49455,#49456,#49457,#49458,#49459,
#49460,#49461,#49462,#49463,#49464,#49465,#49466,#49467,#49468),
 .UNSPECIFIED.,.F.,.F.,(4,3,3,3,3,3,3,3,3,3,3,3,3,3,3,3,3,3,3,3,3,3,3,3,
3,3,3,3,3,3,3,3,3,3,3,3,3,3,3,3,3,3,3,3,3,3,3,3,3,3,3,3,3,3,3,3,3,3,3,3,
3,3,3,3,3,3,3,3,3,3,3,3,3,3,3,3,3,3,3,3,3,3,3,3,3,3,3,3,3,3,3,3,3,3,3,3,
3,3,3,3,3,3,3,3,3,3,3,3,3,3,3,3,3,3,3,3,3,3,3,3,3,3,3,3,3,3,3,3,3,3,3,3,
3,3,3,3,3,3,3,3,4),(0.0206553117127684,0.0206652454314341,0.020977754093757,
0.0209932652001871,0.0210342676712812,0.0210584056073977,0.0210752701423753,
0.0211390602079718,0.0211572750845636,0.0213003887218439,0.0213212849689401,
0.0216231006468298,0.021649304737693,0.0219458804428054,0.021977324506446,
0.0222687230927608,0.022305344275199,0.0223873492173872,0.0224693541595754,
0.0225513591017637,0.0225921303763807,0.0226333640439519,0.0226734259721932,
0.0227547651406014,0.0229175515000403,0.0229613838127049,0.0232435588607619,
0.0232894035814578,0.0235700957719074,0.0236174233502108,0.0238971166937416,
0.0239454431189638,0.0242734628877167,0.024552476688935,0.0246014826564697,
0.0246834875986579,0.0247165657485061,0.0247654925408462,0.0248807370535453,
0.0249295024252226,0.0252092956009399,0.0252575221939756,0.0255855419627286,
0.0258672170688867,0.0262415815002346,0.0265261212738976,0.0268976210377406,
0.0271859382610359,0.0275536605752466,0.0278466298598623,0.0278816803439996,
0.0279800382563648,0.0280119405217654,0.028045690228376,0.0281772804766694,
0.0282097001127526,0.0285080316106845,0.0288657396502586,0.0291697976252322,
0.0295217791877647,0.0298319150904524,0.0301778187252707,0.0304943913353953,
0.0308338582627768,0.0311572425264474,0.0314888172862714,0.0314898978002828,
0.0315719027424711,0.0316539076846594,0.031654635200809,0.0318179175690359,
0.031820437092583,0.032145937337789,0.0324834414874758,0.0328019768752952,
0.0331461052792798,0.0334580164128014,0.0337860361815545,0.0338084021110293,
0.0341140559503076,0.0341394015335586,0.0342780658346841,0.03430486008473,
0.0343600707768724,0.0343875772698666,0.0344420757190606,0.0344702734924882,
0.0347700954878137,0.0351310507499728,0.0354261350253198,0.0357541547940729,
0.0357903626390529,0.036082174562826,0.036410194331579,0.0364480861093856,
0.0364921992737673,0.0365301816915314,0.0365742042159556,0.0366122412866671,
0.0367382141003321,0.0367762502272079,0.0370662338690852,0.0371038366868402,
0.0373942536378383,0.0377222734065914,0.0377572542435978,0.0380502931753445,
0.0380830589309606,0.0382143030597211,0.0382457257725544,0.0382553055308152,
0.0382963080019093,0.0383783129440976,0.0384082492712995,0.0387063327128507,
0.0390343524816037,0.0390570819824594,0.0393623722503567,0.0393807475270067,
0.0396903920191098,0.0397039097155817,0.0398544019034863,0.0398652996031417,
0.0399459546746198,0.0400184117878628,0.0400265578380655,0.0403464315566159,
0.0403488907999544,0.0406710878644882,0.0406744513253689,0.0409931525516835,
0.041002471094122,0.0413150852190492,0.041330490862875,0.0414760016616697,
0.0414945007472516,0.0415564472644614,0.0415765056894398,0.0415966652495433,
0.041617508160534,0.0416368845266418),.UNSPECIFIED.);
#943=B_SPLINE_CURVE_WITH_KNOTS('',3,(#49471,#49472,#49473,#49474,#49475,
#49476,#49477,#49478,#49479,#49480,#49481,#49482,#49483,#49484,#49485,#49486,
#49487,#49488,#49489,#49490,#49491,#49492,#49493,#49494,#49495,#49496,#49497,
#49498,#49499,#49500,#49501,#49502,#49503,#49504,#49505,#49506,#49507,#49508,
#49509,#49510,#49511,#49512,#49513,#49514,#49515,#49516,#49517,#49518,#49519,
#49520,#49521,#49522,#49523,#49524,#49525,#49526,#49527,#49528,#49529,#49530,
#49531,#49532,#49533,#49534,#49535,#49536,#49537,#49538,#49539,#49540,#49541,
#49542,#49543,#49544,#49545,#49546,#49547,#49548,#49549,#49550,#49551,#49552,
#49553,#49554,#49555,#49556,#49557,#49558,#49559,#49560,#49561,#49562,#49563,
#49564,#49565,#49566,#49567,#49568,#49569,#49570,#49571,#49572,#49573,#49574,
#49575,#49576,#49577,#49578,#49579,#49580,#49581,#49582,#49583,#49584,#49585,
#49586,#49587,#49588,#49589,#49590,#49591,#49592,#49593,#49594,#49595,#49596,
#49597,#49598,#49599,#49600,#49601,#49602,#49603,#49604,#49605,#49606,#49607,
#49608,#49609,#49610,#49611,#49612,#49613,#49614,#49615,#49616,#49617,#49618,
#49619,#49620,#49621,#49622,#49623,#49624,#49625,#49626,#49627,#49628,#49629,
#49630,#49631,#49632,#49633,#49634,#49635,#49636,#49637,#49638,#49639,#49640,
#49641,#49642,#49643,#49644,#49645,#49646,#49647,#49648,#49649,#49650,#49651,
#49652,#49653,#49654,#49655,#49656,#49657,#49658,#49659,#49660,#49661,#49662,
#49663,#49664,#49665,#49666,#49667,#49668,#49669,#49670,#49671,#49672,#49673,
#49674,#49675,#49676,#49677,#49678,#49679,#49680,#49681,#49682,#49683,#49684,
#49685,#49686,#49687,#49688,#49689,#49690,#49691,#49692,#49693,#49694,#49695,
#49696,#49697,#49698,#49699,#49700,#49701,#49702,#49703,#49704,#49705,#49706,
#49707,#49708,#49709,#49710,#49711,#49712,#49713,#49714,#49715,#49716,#49717,
#49718,#49719,#49720,#49721,#49722,#49723,#49724,#49725,#49726,#49727,#49728,
#49729,#49730,#49731,#49732,#49733,#49734,#49735,#49736,#49737,#49738,#49739,
#49740,#49741,#49742,#49743,#49744,#49745,#49746,#49747,#49748,#49749,#49750,
#49751,#49752,#49753,#49754,#49755,#49756,#49757,#49758,#49759,#49760,#49761,
#49762,#49763,#49764,#49765,#49766,#49767,#49768,#49769,#49770,#49771,#49772,
#49773,#49774,#49775,#49776,#49777,#49778,#49779,#49780,#49781,#49782,#49783,
#49784,#49785,#49786,#49787,#49788,#49789,#49790,#49791,#49792,#49793,#49794,
#49795,#49796,#49797,#49798,#49799,#49800,#49801,#49802,#49803,#49804,#49805,
#49806,#49807,#49808,#49809,#49810,#49811,#49812,#49813,#49814,#49815,#49816,
#49817,#49818,#49819,#49820,#49821,#49822,#49823,#49824,#49825,#49826,#49827,
#49828,#49829,#49830,#49831,#49832,#49833,#49834,#49835,#49836,#49837,#49838,
#49839,#49840,#49841,#49842,#49843,#49844,#49845,#49846,#49847,#49848,#49849,
#49850,#49851,#49852,#49853,#49854,#49855,#49856,#49857,#49858,#49859,#49860,
#49861),.UNSPECIFIED.,.F.,.F.,(4,3,3,3,3,3,3,3,3,3,3,3,3,3,3,3,3,3,3,3,
3,3,3,3,3,3,3,3,3,3,3,3,3,3,3,3,3,3,3,3,3,3,3,3,3,3,3,3,3,3,3,3,3,3,3,3,
3,3,3,3,3,3,3,3,3,3,3,3,3,3,3,3,3,3,3,3,3,3,3,3,3,3,3,3,3,3,3,3,3,3,3,3,
3,3,3,3,3,3,3,3,3,3,3,3,3,3,3,3,3,3,3,3,3,3,3,3,3,3,3,3,3,3,3,3,3,3,3,3,
3,3,4),(0.041957164410437,0.0419580282593461,0.0419865304003811,0.0422778480319385,
0.0423145501691341,0.042598747472383,0.042642569937887,0.0429207530509651,
0.04297058970664,0.0430821721477515,0.0431345995910165,0.0431629890966594,
0.0432166045332047,0.0432438666760118,0.0432986094753929,0.0435677751170178,
0.0436266292441459,0.0439546490128989,0.0442172193461882,0.0442826687816519,
0.0445427409092368,0.0446106885504049,0.0447057005683472,0.0447746984347814,
0.0447872307357854,0.0448400446384891,0.0448567033769696,0.0448687931306013,
0.0449387083191578,0.0452667280879107,0.0455225904419517,0.0455947478566636,
0.0459227676254165,0.046178592821652,0.0462507873941694,0.0465074031590051,
0.0465788071629223,0.0465896703494642,0.0466719689207823,0.0468366677402474,
0.0469068269316752,0.0472348467004281,0.0474963684871569,0.0478908862379339,
0.0481574787691429,0.0482189060066868,0.0483829158910632,0.0484649208332514,
0.048488535463458,0.0485469257754396,0.0485713483333225,0.0486541709718429,
0.0488198358119608,0.0488749455441925,0.0492029653129454,0.0494827516683778,
0.0498590048504511,0.0501460513738034,0.0505150443879569,0.0508097071743785,
0.0511710839254627,0.0514736994554526,0.0514991036942155,0.0515811086364038,
0.0516397419533068,0.051663113578592,0.0518057633287904,0.0518271234629685,
0.0521377210298803,0.0524831630004743,0.0528013150691172,0.0531392025379801,
0.0534644977760899,0.053795242075486,0.0541272802645444,0.0544512816129918,
0.0547896633480624,0.0551073211504977,0.0554353409192506,0.0554516373676069,
0.0555173458614388,0.0555343525719785,0.0555993508036271,0.0556170522770077,
0.0557633606880035,0.0557824062888781,0.0561129301282526,0.0564194002255094,
0.0567732198580588,0.0570754397630152,0.0574034595317682,0.0574324401050507,
0.0577314793005211,0.058059499069274,0.0580904787336963,0.0582235089536505,
0.0582547858893481,0.0583055138958387,0.058375815716685,0.0584189997464737,
0.0587155386067799,0.0587471023565642,0.0590435583755328,0.0590747344055545,
0.0593715781442858,0.0594018599075076,0.0596995979130387,0.0597284330635356,
0.0598636077974152,0.0598914947728063,0.0599456127396034,0.059972965839742,
0.0599866152106975,0.0600276176817916,0.0600543950381653,0.0603556374505446,
0.0603797504464674,0.0606836572192975,0.0607044891413336,0.0610116769880505,
0.061028559959805,0.0611756868724269,0.0611903246948573,0.0612576918146152,
0.0612711334768389,0.0612986942857093,0.0613396967568034,0.0613519093639181,
0.0616677165255564,0.0616748080368333,0.0619121248264431),.UNSPECIFIED.);
#944=B_SPLINE_CURVE_WITH_KNOTS('',3,(#49864,#49865,#49866,#49867,#49868,
#49869,#49870,#49871,#49872,#49873,#49874,#49875,#49876,#49877,#49878,#49879,
#49880,#49881,#49882,#49883,#49884,#49885,#49886,#49887,#49888,#49889,#49890,
#49891,#49892,#49893,#49894,#49895,#49896,#49897,#49898,#49899,#49900,#49901,
#49902,#49903,#49904,#49905,#49906,#49907,#49908,#49909,#49910,#49911,#49912,
#49913,#49914,#49915,#49916,#49917,#49918,#49919,#49920,#49921,#49922,#49923,
#49924,#49925,#49926,#49927,#49928,#49929,#49930,#49931,#49932,#49933,#49934,
#49935,#49936,#49937,#49938,#49939,#49940,#49941,#49942,#49943,#49944,#49945,
#49946,#49947,#49948,#49949,#49950,#49951,#49952,#49953,#49954,#49955,#49956,
#49957,#49958,#49959,#49960,#49961,#49962,#49963,#49964,#49965,#49966,#49967,
#49968,#49969,#49970,#49971,#49972,#49973,#49974,#49975,#49976,#49977,#49978,
#49979,#49980,#49981),.UNSPECIFIED.,.F.,.F.,(4,2,1,1,1,1,1,2,2,1,1,1,2,
2,2,1,1,1,1,1,2,2,2,1,1,1,1,1,1,1,2,1,1,1,1,1,1,1,1,1,2,2,1,1,1,1,1,1,1,
1,2,2,1,1,1,1,1,1,2,2,1,1,1,1,1,1,2,2,2,1,1,1,1,1,2,2,1,1,1,1,1,1,2,1,2,
2,1,1,1,1,1,4),(0.0551992890963671,0.0552052082809216,0.0553145255250422,
0.0555331600132834,0.0557517945015246,0.0558611117456452,0.0559157703677055,
0.0559635966620083,0.0559704289897659,0.0564076979662487,0.0568449669427315,
0.0572822359192143,0.0577195048956971,0.0579381393839385,0.0580474566280592,
0.0581567738721799,0.0585940428486627,0.0590313118251455,0.0594685808016283,
0.0599058497781111,0.0603431187545939,0.0605617532428353,0.0606164118648956,
0.0606710704869559,0.0607803877310766,0.0612176567075593,0.061654925684042,
0.0620921946605247,0.0625294636370074,0.0629667326134901,0.0634040015899728,
0.0634586602120332,0.0635133188340935,0.0636226360782142,0.0638412705664556,
0.0642785395429383,0.0647158085194211,0.0651530774959038,0.0655903464723866,
0.0660276154488694,0.0664648844253521,0.0665195430474125,0.0665742016694728,
0.0666835189135935,0.0669021534018348,0.0673394223783175,0.0677766913548003,
0.068213960331283,0.0686512293077657,0.0690884982842484,0.0695257672607311,
0.0696350845048518,0.0697444017489724,0.0699630362372138,0.0704003052136965,
0.0708375741901792,0.0712748431666619,0.0717121121431446,0.0721493811196273,
0.0722040397416877,0.072258698363748,0.0723680156078687,0.07258665009611,
0.0730239190725927,0.0734611880490754,0.0738984570255581,0.0743357260020407,
0.0745543604902821,0.0747729949785234,0.0752102639550061,0.0756475329314888,
0.0760848019079715,0.0765220708844541,0.0769593398609368,0.0773966088374195,
0.0776152433256608,0.0778338778139022,0.0782711467903849,0.0787084157668675,
0.0791456847433502,0.0795829537198329,0.0800202226963156,0.0804574916727983,
0.0806761261610396,0.0807854434051603,0.0808947606492809,0.0813320296257635,
0.0817692986022461,0.0822065675787287,0.0826438365552113,0.0830811055316939,
0.0831743481010765),.UNSPECIFIED.);
#945=B_SPLINE_CURVE_WITH_KNOTS('',3,(#49982,#49983,#49984,#49985,#49986,
#49987,#49988,#49989,#49990,#49991,#49992,#49993,#49994,#49995,#49996,#49997,
#49998,#49999,#50000,#50001,#50002,#50003,#50004,#50005,#50006,#50007,#50008,
#50009,#50010,#50011,#50012,#50013,#50014,#50015,#50016,#50017,#50018,#50019,
#50020,#50021,#50022,#50023,#50024,#50025,#50026,#50027,#50028,#50029,#50030,
#50031,#50032,#50033,#50034,#50035,#50036,#50037,#50038,#50039,#50040,#50041,
#50042,#50043,#50044,#50045,#50046,#50047,#50048,#50049,#50050,#50051,#50052,
#50053,#50054,#50055,#50056,#50057,#50058,#50059,#50060,#50061,#50062,#50063,
#50064,#50065,#50066,#50067,#50068,#50069,#50070,#50071,#50072,#50073,#50074,
#50075,#50076,#50077,#50078,#50079,#50080,#50081,#50082,#50083,#50084,#50085,
#50086,#50087,#50088,#50089,#50090,#50091,#50092,#50093,#50094,#50095,#50096,
#50097,#50098,#50099,#50100,#50101,#50102,#50103,#50104,#50105,#50106),
 .UNSPECIFIED.,.F.,.F.,(4,2,1,1,2,2,1,2,2,2,1,1,1,1,1,2,1,1,2,2,1,1,1,1,
1,2,1,2,2,1,1,1,1,1,1,2,1,2,2,1,1,1,1,1,1,2,1,2,2,1,1,1,1,1,2,2,2,1,1,1,
1,1,2,2,2,1,1,1,1,2,1,2,2,1,1,1,1,1,1,2,1,1,2,2,1,1,1,1,1,1,2,4),(0.0272039191113106,
0.0275479455184106,0.0277665800066519,0.0278758972507726,0.0279305558728329,
0.0279852144948932,0.0284224834713757,0.0288597524478581,0.0289690696919787,
0.0290783869360993,0.0292970214243406,0.029734290400823,0.0301715593773054,
0.0306088283537878,0.0310460973302702,0.0314833663067526,0.0317020007949938,
0.0318113180391144,0.0318659766611747,0.031920635283235,0.0323579042597174,
0.0327951732361998,0.0332324422126821,0.0336697111891645,0.0341069801656468,
0.0345442491421292,0.0346535663862498,0.0347082250083101,0.0347628836303704,
0.0349815181186115,0.0354187870950939,0.0358560560715762,0.0362933250480586,
0.0367305940245409,0.0371678630010232,0.0376051319775056,0.0377144492216262,
0.0377691078436864,0.0378237664657467,0.0380424009539879,0.0384796699304703,
0.0389169389069527,0.039354207883435,0.0397914768599174,0.0402287458363998,
0.0406660148128821,0.0407753320570027,0.040829990679063,0.0408846493011233,
0.0411032837893645,0.0415405527658469,0.0419778217423292,0.0424150907188116,
0.042852359695294,0.0432896286717764,0.0435082631600175,0.0436175804041381,
0.0437268976482587,0.0441641666247411,0.0446014356012235,0.0450387045777058,
0.0454759735541882,0.0459132425306706,0.0461318770189118,0.0463505115071529,
0.0467877804836353,0.0472250494601177,0.0476623184366001,0.0480995874130824,
0.0485368563895648,0.048755490877806,0.0488648081219266,0.0489194667439869,
0.0489741253660472,0.0494113943425296,0.049848663319012,0.0502859322954944,
0.0507232012719768,0.0511604702484592,0.0515977392249416,0.0518163737131828,
0.0519256909573034,0.0519803495793637,0.0520350082014241,0.0524722771779065,
0.0529095461543889,0.0533468151308713,0.0537840841073537,0.0542213530838361,
0.0546586220603186,0.055095891036801,0.0551992890963671),.UNSPECIFIED.);
#946=B_SPLINE_CURVE_WITH_KNOTS('',3,(#50114,#50115,#50116,#50117,#50118,
#50119),.UNSPECIFIED.,.F.,.F.,(4,1,1,4),(0.00380072940365624,0.00412124310825456,
0.00444175681285289,0.00448635962221661),.UNSPECIFIED.);
#947=B_SPLINE_CURVE_WITH_KNOTS('',3,(#50121,#50122,#50123,#50124,#50125,
#50126,#50127,#50128,#50129,#50130,#50131,#50132,#50133,#50134,#50135,#50136,
#50137,#50138,#50139,#50140,#50141,#50142,#50143,#50144,#50145,#50146,#50147,
#50148,#50149,#50150,#50151,#50152,#50153,#50154,#50155,#50156,#50157,#50158,
#50159,#50160,#50161,#50162,#50163,#50164,#50165,#50166,#50167,#50168,#50169,
#50170,#50171,#50172,#50173,#50174,#50175,#50176,#50177,#50178,#50179,#50180,
#50181,#50182,#50183,#50184,#50185,#50186,#50187,#50188,#50189,#50190,#50191,
#50192,#50193,#50194,#50195,#50196,#50197,#50198,#50199,#50200,#50201,#50202,
#50203,#50204,#50205,#50206,#50207,#50208,#50209,#50210,#50211,#50212,#50213,
#50214,#50215,#50216,#50217,#50218,#50219,#50220,#50221,#50222,#50223,#50224,
#50225,#50226,#50227,#50228,#50229,#50230,#50231,#50232,#50233,#50234,#50235,
#50236,#50237,#50238),.UNSPECIFIED.,.F.,.F.,(4,3,3,3,3,3,3,3,3,3,3,3,3,
3,3,3,3,3,3,3,3,3,3,3,3,3,3,3,3,3,3,3,3,3,3,3,3,3,3,4),(0.00448635962221661,
0.00473358542950409,0.00476227051745122,0.00480233473052602,0.00482691085287281,
0.00484239894360081,0.00492023496407616,0.00508278422204955,0.00510688429789094,
0.00540329792664787,0.005480183189725,0.00572381163124619,0.00585348292348728,
0.00604432533584451,0.00622678424286061,0.00636483904044283,0.00641343584205939,
0.0064449674665924,0.00650676142924672,0.00652509589274198,0.00660008754740501,
0.00668535274504114,0.0069734073638536,0.00700586644963945,0.00706674043229878,
0.00708599487578904,0.00716007751974228,0.00732638015423778,0.00734684552356649,
0.00764689385883611,0.00772082703711819,0.00796740756343444,0.00809541822331551,
0.00828792126803276,0.0084706476028549,0.00860843497263109,0.00865852771923415,
0.00875251842491186,0.00884627452670677,0.00892894867722942),
 .UNSPECIFIED.);
#948=B_SPLINE_CURVE_WITH_KNOTS('',3,(#50246,#50247,#50248,#50249,#50250,
#50251,#50252,#50253,#50254,#50255,#50256,#50257,#50258,#50259,#50260,#50261,
#50262,#50263,#50264,#50265,#50266,#50267,#50268,#50269,#50270,#50271,#50272,
#50273,#50274,#50275,#50276,#50277,#50278,#50279,#50280,#50281,#50282,#50283,
#50284,#50285,#50286,#50287,#50288,#50289,#50290,#50291,#50292,#50293,#50294,
#50295,#50296,#50297,#50298,#50299,#50300,#50301,#50302,#50303,#50304,#50305,
#50306,#50307,#50308),.UNSPECIFIED.,.F.,.F.,(4,2,2,1,1,1,1,1,1,2,1,2,2,
1,1,1,1,1,1,2,2,2,1,2,2,2,1,1,1,1,1,2,2,2,1,1,1,2,2,1,1,1,1,1,4),(8.54252242016652E-18,
0.000160194806869816,0.000240292210304721,0.000320389613739627,0.000640779227479243,
0.000961168841218859,0.00128155845495848,0.00160194806869809,0.00192233768243771,
0.00224272729617732,0.00232282469961223,0.00236287340132968,0.00240292210304713,
0.00256311690991691,0.00288350652365649,0.00320389613739606,0.00352428575113563,
0.0038446753648752,0.00416506497861477,0.00448545459235434,0.00456555199578923,
0.00464564939922412,0.00480584420609392,0.00512623381983351,0.00528642862670331,
0.00536652603013821,0.00544662343357311,0.00576701304731269,0.00608740266105227,
0.00640779227479185,0.00672818188853143,0.00704857150227101,0.0072087663091408,
0.00728886371257569,0.00736896111601059,0.00768935072975016,0.00800974034348972,
0.00833012995722929,0.00849032476409908,0.00853037346581653,0.00857042216753398,
0.00865051957096888,0.00897090918470849,0.0092912987984481,0.00956209106146699),
 .UNSPECIFIED.);
#949=B_SPLINE_CURVE_WITH_KNOTS('',3,(#50310,#50311,#50312,#50313,#50314,
#50315,#50316,#50317,#50318,#50319,#50320,#50321,#50322,#50323,#50324,#50325,
#50326,#50327,#50328,#50329,#50330,#50331),.UNSPECIFIED.,.F.,.F.,(4,3,3,
3,3,3,3,4),(0.00956209106146699,0.00961168841218771,0.00976759725391833,
0.00980857291316444,0.00984954064048262,0.00993152890309068,0.0100957710509459,
0.0102524676396669),.UNSPECIFIED.);
#950=B_SPLINE_CURVE_WITH_KNOTS('',3,(#50332,#50333,#50334,#50335,#50336,
#50337,#50338,#50339,#50340,#50341,#50342,#50343,#50344,#50345,#50346,#50347,
#50348,#50349,#50350,#50351,#50352,#50353,#50354,#50355,#50356,#50357,#50358,
#50359,#50360,#50361,#50362,#50363,#50364,#50365,#50366,#50367,#50368,#50369,
#50370,#50371,#50372,#50373,#50374,#50375,#50376,#50377,#50378,#50379,#50380,
#50381,#50382,#50383,#50384,#50385,#50386,#50387,#50388,#50389,#50390,#50391,
#50392,#50393,#50394,#50395,#50396,#50397,#50398,#50399,#50400,#50401,#50402,
#50403,#50404,#50405,#50406,#50407,#50408,#50409,#50410,#50411,#50412,#50413,
#50414,#50415,#50416,#50417,#50418,#50419,#50420,#50421,#50422,#50423,#50424,
#50425,#50426,#50427,#50428,#50429,#50430,#50431,#50432,#50433,#50434,#50435,
#50436,#50437,#50438,#50439,#50440,#50441,#50442,#50443,#50444,#50445,#50446,
#50447,#50448,#50449,#50450,#50451,#50452,#50453,#50454,#50455,#50456,#50457,
#50458,#50459,#50460,#50461,#50462,#50463,#50464,#50465,#50466,#50467,#50468,
#50469,#50470,#50471,#50472,#50473,#50474,#50475,#50476,#50477,#50478,#50479,
#50480,#50481,#50482,#50483,#50484,#50485,#50486,#50487,#50488,#50489,#50490,
#50491,#50492,#50493,#50494,#50495,#50496,#50497,#50498,#50499,#50500,#50501,
#50502,#50503,#50504,#50505,#50506,#50507,#50508,#50509,#50510,#50511,#50512,
#50513,#50514,#50515,#50516,#50517,#50518,#50519,#50520,#50521,#50522,#50523,
#50524,#50525,#50526,#50527,#50528,#50529,#50530,#50531,#50532,#50533,#50534,
#50535,#50536,#50537,#50538,#50539,#50540,#50541,#50542,#50543,#50544,#50545,
#50546,#50547,#50548,#50549,#50550,#50551,#50552,#50553,#50554,#50555,#50556,
#50557,#50558,#50559,#50560,#50561,#50562,#50563,#50564,#50565,#50566,#50567,
#50568,#50569,#50570,#50571,#50572,#50573,#50574,#50575,#50576,#50577,#50578,
#50579,#50580,#50581,#50582,#50583,#50584,#50585,#50586,#50587,#50588,#50589,
#50590,#50591,#50592,#50593,#50594,#50595,#50596,#50597,#50598,#50599,#50600,
#50601,#50602,#50603,#50604,#50605,#50606,#50607,#50608,#50609,#50610,#50611,
#50612,#50613,#50614,#50615,#50616,#50617,#50618,#50619,#50620,#50621,#50622,
#50623,#50624,#50625,#50626,#50627,#50628,#50629,#50630,#50631,#50632,#50633,
#50634,#50635,#50636,#50637,#50638,#50639,#50640,#50641,#50642,#50643,#50644,
#50645,#50646,#50647,#50648,#50649,#50650,#50651,#50652,#50653,#50654,#50655,
#50656,#50657,#50658,#50659,#50660,#50661,#50662,#50663,#50664,#50665,#50666,
#50667,#50668,#50669,#50670,#50671,#50672,#50673,#50674,#50675,#50676,#50677,
#50678,#50679,#50680,#50681,#50682,#50683,#50684,#50685,#50686,#50687,#50688,
#50689,#50690,#50691,#50692,#50693,#50694,#50695,#50696,#50697,#50698,#50699,
#50700,#50701),.UNSPECIFIED.,.F.,.F.,(4,3,3,3,3,3,3,3,3,3,3,3,3,3,3,3,3,
3,3,3,3,3,3,3,3,3,3,3,3,3,3,3,3,3,3,3,3,3,3,3,3,3,3,3,3,3,3,3,3,3,3,3,3,
3,3,3,3,3,3,3,3,3,3,3,3,3,3,3,3,3,3,3,3,3,3,3,3,3,3,3,3,3,3,3,3,3,3,3,3,
3,3,3,3,3,3,3,3,3,3,3,3,3,3,3,3,3,3,3,3,3,3,3,3,3,3,3,3,3,3,3,3,3,3,4),
(2.59922340967641E-10,0.000262388289418012,0.000329189181563099,0.000467357547817636,
0.000524776578836023,0.000590373651190526,0.000605976118520986,0.00065597072354503,
0.000883792457061135,0.00104955315767209,0.00144104403044228,0.00157432973650817,
0.00200001764535897,0.00209910631534426,0.00256029609833201,0.00262388289418034,
0.00312154984340054,0.00314865947301643,0.00326198305548787,0.00327985361772545,
0.00334545069007997,0.00340244081200927,0.00341104776243449,0.00367343605185254,
0.00368317018991879,0.00419821263068866,0.00424371040228981,0.00472298920952478,
0.00480285009820333,0.0052477657883609,0.00536037435326884,0.00577254236719702,
0.00591605037941538,0.00603493065661509,0.00605465039573207,0.00612389765881176,
0.00616612480132412,0.00619309863725878,0.00629731894603315,0.00646939602860005,
0.0067448599582135,0.00682209552486926,0.0068822653254087,0.00695328966957829,
0.00701944169990729,0.00708448381428732,0.00734687210370539,0.00756558389005768,
0.00787164868254153,0.0081074466846592,0.0081340369719596,0.00837667669017726,
0.00839642526137767,0.00844379880569796,0.00846202233373219,0.00851084615263126,
0.0085276194060867,0.00864473211587614,0.00865881355079574,0.00892120184021382,
0.00917757482779576,0.0091835901296319,0.00944234903430452,0.00944597841904998,
0.00970599790514705,0.00970836670846806,0.00983739163427776,0.00983956085317709,
0.00990297905228762,0.00990515792553161,0.00993795646170887,0.00996850338831347,
0.00997075499788612,0.0102302598050392,0.0104914878165698,0.0104955315767223,
0.0107521972284278,0.0107579198661403,0.0110123944037893,0.0110203081555584,
0.0112720829688689,0.0112826964449765,0.011348293517331,0.0113810920535082,
0.0114017360867843,0.0114138905896855,0.0115313481146533,0.0115450847343945,
0.0117907037577083,0.0118074730238126,0.0120502249089893,0.0120698613132307,
0.0123098994004552,0.0123322496026488,0.0125946378920669,0.012829666102776,
0.012857026181485,0.0129882203261941,0.0130538173985486,0.013089795720895,
0.0131194144709031,0.0131550420289316,0.0132203550964659,0.0133511192354543,
0.0133818027603212,0.0136441910497393,0.0138755852809746,0.0139065793391574,
0.0141689676285755,0.0144021169982843,0.0146937442074117,0.0149304527077196,
0.0149561324968298,0.0150217295691844,0.0150627981915921,0.0150873266415389,
0.015195189240927,0.0152185207862479,0.0154599955937371,0.0157432973650841,
0.0159896040980766,0.0162680739439203,0.016519074845501,0.0167928505227559),
 .UNSPECIFIED.);
#951=B_SPLINE_CURVE_WITH_KNOTS('',3,(#51506,#51507,#51508,#51509,#51510,
#51511,#51512,#51513,#51514,#51515,#51516,#51517,#51518,#51519,#51520,#51521,
#51522,#51523,#51524,#51525,#51526,#51527,#51528,#51529,#51530,#51531,#51532,
#51533,#51534,#51535,#51536,#51537,#51538,#51539,#51540,#51541,#51542,#51543,
#51544,#51545,#51546,#51547,#51548,#51549,#51550,#51551,#51552,#51553,#51554,
#51555,#51556,#51557,#51558,#51559,#51560,#51561,#51562,#51563,#51564,#51565,
#51566,#51567,#51568,#51569,#51570,#51571,#51572,#51573,#51574,#51575,#51576,
#51577,#51578,#51579,#51580,#51581,#51582,#51583,#51584,#51585,#51586,#51587,
#51588,#51589,#51590,#51591,#51592,#51593,#51594,#51595,#51596,#51597,#51598,
#51599,#51600,#51601,#51602,#51603,#51604,#51605,#51606,#51607,#51608,#51609,
#51610,#51611,#51612,#51613,#51614,#51615,#51616,#51617,#51618,#51619,#51620,
#51621,#51622,#51623,#51624),.UNSPECIFIED.,.F.,.F.,(4,2,1,1,1,1,1,1,2,2,
2,1,2,1,1,1,1,1,2,1,2,2,1,1,1,1,1,2,2,2,1,1,1,1,1,1,2,2,2,1,1,1,1,1,1,2,
2,2,1,1,1,1,1,1,2,2,2,1,1,1,1,1,1,2,1,2,2,1,1,1,1,1,2,2,2,1,1,1,1,1,1,2,
1,2,2,1,1,4),(0.000691744478869641,0.000711184477407308,0.00081278225989404,
0.00121917338984095,0.00162556451978785,0.00203195564973476,0.00243834677968166,
0.00284473790962857,0.00325112903957547,0.00335272682206222,0.00345432460454896,
0.0035559223870357,0.00365752016952244,0.00406391129946942,0.00447030242941641,
0.00487669355936339,0.00528308468931038,0.00568947581925736,0.00609586694920435,
0.00629906251417784,0.00640066029666459,0.00650225807915134,0.00690864920909835,
0.00731504033904536,0.00772143146899237,0.00812782259893938,0.00853421372888639,
0.0089406048588334,0.00904220264132015,0.00909300153256353,0.00914380042380691,
0.00934699598878044,0.00975338711872751,0.0101597782486746,0.0105661693786217,
0.0109725605085687,0.0113789516385158,0.0114805494210026,0.0115313483122459,
0.0115821472034893,0.0117853427684629,0.0121917338984099,0.012598125028357,
0.0130045161583041,0.0134109072882511,0.0138172984181982,0.0140204939831718,
0.0141220917656585,0.0142236895481453,0.0146300806780924,0.0150364718080394,
0.0154428629379865,0.0158492540679336,0.0162556451978807,0.0166620363278277,
0.0168652318928013,0.016966829675288,0.0170684274577748,0.0174748185877219,
0.017881209717669,0.0182876008476161,0.0186939919775632,0.0191003831075103,
0.0195067742374574,0.0197099698024309,0.0198115675849177,0.0199131653674045,
0.0203195564973515,0.0207259476272986,0.0211323387572457,0.0215387298871928,
0.0219451210171399,0.022351512147087,0.0224531099295737,0.0225039088208171,
0.0225547077120605,0.0227579032770339,0.0231642944069809,0.0235706855369278,
0.0239770766668748,0.0243834677968217,0.0247898589267687,0.0249930544917421,
0.0250946522742289,0.0251454511654722,0.0251962500567156,0.0256026411866625,
0.0259925502271156),.UNSPECIFIED.);
#952=B_SPLINE_CURVE_WITH_KNOTS('',3,(#51628,#51629,#51630,#51631,#51632,
#51633,#51634,#51635,#51636,#51637,#51638,#51639),.UNSPECIFIED.,.F.,.F.,
(4,2,2,2,2,4),(0.193494937972427,0.221478557046408,0.257021340074901,0.304852388878296,
0.36775906785294,0.368268523654839),.UNSPECIFIED.);
#953=B_SPLINE_CURVE_WITH_KNOTS('',3,(#51648,#51649,#51650,#51651,#51652,
#51653,#51654,#51655,#51656,#51657,#51658,#51659,#51660,#51661,#51662,#51663,
#51664,#51665,#51666,#51667,#51668,#51669,#51670,#51671,#51672,#51673,#51674,
#51675,#51676,#51677,#51678,#51679,#51680,#51681,#51682,#51683,#51684,#51685,
#51686,#51687,#51688,#51689,#51690,#51691,#51692,#51693,#51694,#51695,#51696,
#51697,#51698,#51699,#51700,#51701,#51702,#51703,#51704,#51705,#51706,#51707,
#51708,#51709,#51710,#51711,#51712,#51713,#51714,#51715,#51716,#51717,#51718,
#51719,#51720,#51721,#51722,#51723,#51724,#51725,#51726,#51727,#51728,#51729,
#51730,#51731,#51732,#51733,#51734,#51735,#51736,#51737,#51738,#51739,#51740,
#51741,#51742,#51743,#51744,#51745,#51746,#51747,#51748,#51749,#51750,#51751,
#51752,#51753,#51754,#51755,#51756,#51757,#51758,#51759,#51760,#51761,#51762,
#51763,#51764,#51765,#51766,#51767,#51768,#51769,#51770,#51771,#51772,#51773),
 .UNSPECIFIED.,.F.,.F.,(4,1,1,1,1,2,2,2,2,2,1,1,1,1,1,1,1,2,2,2,1,1,1,1,
1,1,2,1,2,2,1,1,1,1,2,1,2,2,1,1,1,1,1,1,2,2,1,1,1,1,1,1,2,1,1,2,2,1,1,1,
1,1,1,2,2,2,1,1,1,1,1,1,2,1,2,2,1,1,1,1,1,2,2,2,1,1,1,1,2,1,1,1,2,4),(0.0267086453492391,
0.0268218145765036,0.0272282057064507,0.0276345968363977,0.0280409879663448,
0.0284473790962919,0.0286505746612654,0.0287521724437522,0.0288537702262389,
0.0289553680087257,0.0290569657912125,0.029260161356186,0.029666552486133,
0.0300729436160801,0.0304793347460271,0.0308857258759742,0.0312921170059213,
0.0316985081358683,0.0317493070271117,0.0318001059183551,0.0319017037008419,
0.0321048992658154,0.0325112903957626,0.0329176815257097,0.0333240726556568,
0.0337304637856039,0.0341368549155511,0.0343400504805246,0.0344416482630114,
0.0345432460454982,0.0349496371754453,0.0353560283053924,0.0357624194353395,
0.0361688105652867,0.0365752016952338,0.0367783972602073,0.0368799950426941,
0.0369307939339375,0.0369815928251809,0.0373879839551279,0.037794375085075,
0.0382007662150221,0.0386071573449691,0.0390135484749162,0.0394199396048632,
0.03952153738735,0.0396231351698367,0.0398263307348103,0.0402327218647573,
0.0406391129947044,0.0410455041246514,0.0414518952545985,0.0418582863845456,
0.0420614819495191,0.0421630797320059,0.0422138786232492,0.0422646775144926,
0.0426710686444397,0.0430774597743867,0.0434838509043337,0.0438902420342808,
0.0442966331642278,0.0447030242941749,0.0451094154241219,0.0451602143153653,
0.0452110132066086,0.0453126109890954,0.0455158065540689,0.0459221976840159,
0.0463285888139629,0.04673497994391,0.047141371073857,0.047547762203804,
0.0477509577687775,0.0478017566600209,0.0478525555512643,0.047954153333751,
0.0483605444636982,0.0487669355936454,0.0491733267235925,0.0495797178535397,
0.0499861089834869,0.0501893045484605,0.0502401034397039,0.0502909023309472,
0.050392500113434,0.0507988912433812,0.0512052823733283,0.0516116735032755,
0.051814869068249,0.0519164668507358,0.0519672657419792,0.0520053649104118,
0.0520180646332226),.UNSPECIFIED.);
#954=B_SPLINE_CURVE_WITH_KNOTS('',3,(#51778,#51779,#51780,#51781,#51782,
#51783,#51784,#51785,#51786,#51787,#51788,#51789,#51790,#51791,#51792,#51793,
#51794,#51795,#51796,#51797,#51798,#51799,#51800,#51801,#51802,#51803,#51804,
#51805,#51806,#51807,#51808,#51809,#51810,#51811,#51812,#51813,#51814,#51815,
#51816,#51817,#51818,#51819,#51820,#51821,#51822,#51823,#51824,#51825,#51826,
#51827,#51828,#51829,#51830,#51831,#51832,#51833,#51834,#51835,#51836,#51837,
#51838,#51839,#51840,#51841,#51842,#51843,#51844,#51845,#51846,#51847,#51848),
 .UNSPECIFIED.,.F.,.F.,(4,1,1,1,1,1,2,2,1,1,1,1,1,1,1,2,2,2,1,2,2,1,1,1,
1,1,1,2,2,2,1,1,1,1,1,1,2,1,2,2,1,1,1,1,2,1,2,2,1,1,1,1,4),(2.81851621706032E-10,
0.000430383770082051,0.000860767540164102,0.00129115131024615,0.0017215350803282,
0.00215191885041026,0.00258230262049231,0.00263610059175256,0.00268989856301282,
0.00279749450553333,0.00301268639057435,0.0034430701606564,0.00387345393073844,
0.00430383770082048,0.00473422147090253,0.00516460524098457,0.00537979712602559,
0.0054873930685461,0.00559498901106661,0.00581018089610763,0.00602537278114865,
0.00645575655123069,0.00688614032131272,0.00731652409139476,0.0077469078614768,
0.00817729163155883,0.00860767540164087,0.00903805917172291,0.00909185714298317,
0.00914565511424342,0.00925325105676395,0.00946844294180499,0.00989882671188708,
0.0103292104819692,0.0107595942520513,0.0111899780221333,0.0116203617922154,
0.0118355536772565,0.011943149619777,0.0120507455622975,0.0124811293323796,
0.0129115131024617,0.0133418968725438,0.013772280642626,0.0142026644127081,
0.0144178562977491,0.0145254522402697,0.0146330481827902,0.0150634319528723,
0.0154938157229543,0.0159241994930364,0.0163545832631185,0.0167022853636743),
 .UNSPECIFIED.);
#955=B_SPLINE_CURVE_WITH_KNOTS('',3,(#51850,#51851,#51852,#51853,#51854,
#51855,#51856,#51857,#51858,#51859,#51860,#51861,#51862,#51863,#51864,#51865,
#51866,#51867,#51868,#51869,#51870,#51871,#51872,#51873,#51874,#51875,#51876,
#51877,#51878,#51879,#51880,#51881,#51882,#51883,#51884,#51885,#51886,#51887,
#51888,#51889,#51890,#51891,#51892,#51893,#51894,#51895,#51896,#51897,#51898,
#51899,#51900,#51901,#51902,#51903,#51904,#51905,#51906,#51907,#51908,#51909,
#51910,#51911,#51912,#51913,#51914,#51915,#51916,#51917,#51918,#51919,#51920,
#51921,#51922,#51923,#51924,#51925,#51926,#51927,#51928,#51929,#51930,#51931,
#51932,#51933,#51934,#51935,#51936,#51937,#51938,#51939,#51940,#51941,#51942,
#51943,#51944,#51945,#51946,#51947,#51948,#51949,#51950,#51951,#51952,#51953,
#51954,#51955,#51956,#51957,#51958,#51959,#51960,#51961,#51962,#51963,#51964,
#51965,#51966,#51967,#51968,#51969,#51970,#51971),.UNSPECIFIED.,.F.,.F.,
(4,2,1,1,2,2,1,1,1,1,1,2,1,1,1,1,1,1,2,2,2,1,1,1,1,1,1,2,1,2,2,1,1,1,1,
1,1,2,1,2,2,1,1,1,1,1,1,2,2,1,1,1,1,1,1,1,1,2,2,2,1,1,1,1,1,1,2,2,2,1,1,
1,1,1,1,2,1,2,2,1,1,1,1,2,1,2,2,1,1,1,1,1,4),(0.0167022853636743,0.0167849670332005,
0.0170001589182416,0.0171077548607621,0.0171615528320224,0.0172153508032826,
0.0176457345733647,0.0180761183434467,0.0185065021135288,0.0189368858836108,
0.0193672696536929,0.0197976534237749,0.020228037193857,0.020658420963939,
0.0210888047340211,0.0215191885041031,0.0219495722741852,0.0223799560442672,
0.0228103398143493,0.0230255316993903,0.0231331276419108,0.0232407235844313,
0.0236711073545133,0.0241014911245954,0.0245318748946774,0.0249622586647594,
0.0253926424348414,0.0258230262049235,0.0260382180899645,0.0260920160612247,
0.026145814032485,0.0262534099750055,0.0266837937450876,0.0271141775151697,
0.0275445612852518,0.0279749450553339,0.028405328825416,0.0288357125954981,
0.0290509044805392,0.0291047024517994,0.0291585004230597,0.0292660963655802,
0.0296964801356624,0.0301268639057445,0.0305572476758266,0.0309876314459087,
0.0314180152159908,0.0318483989860729,0.0319021969573332,0.0319559949285935,
0.032063590871114,0.0322787827561551,0.0327091665262372,0.0331395502963193,
0.0335699340664014,0.0340003178364836,0.0344307016065657,0.0348610853766478,
0.0350762772616889,0.0352914691467299,0.0357218529168121,0.0361522366868942,
0.0365826204569763,0.0370130042270585,0.0374433879971406,0.0378737717672227,
0.0383041555373048,0.0383579535085651,0.0384117514798254,0.0385193474223459,
0.038734539307387,0.0391649230774692,0.0395953068475513,0.0400256906176335,
0.0404560743877157,0.0408864581577978,0.0411016500428389,0.0412092459853594,
0.0413168419278799,0.0417472256979621,0.0421776094680442,0.0426079932381263,
0.0430383770082085,0.0434687607782906,0.0436839526633316,0.0437377506345919,
0.0437915486058522,0.0438991445483727,0.0443295283184549,0.044759912088537,
0.0451902958586192,0.0456206796287013,0.0457216170362868),.UNSPECIFIED.);
#956=B_SPLINE_CURVE_WITH_KNOTS('',3,(#51973,#51974,#51975,#51976,#51977,
#51978,#51979,#51980,#51981,#51982,#51983,#51984,#51985,#51986,#51987,#51988,
#51989,#51990,#51991,#51992,#51993,#51994,#51995,#51996,#51997,#51998,#51999,
#52000,#52001,#52002,#52003,#52004,#52005,#52006,#52007,#52008,#52009,#52010,
#52011,#52012,#52013,#52014,#52015,#52016,#52017,#52018,#52019,#52020,#52021,
#52022,#52023,#52024,#52025,#52026,#52027,#52028,#52029,#52030,#52031,#52032,
#52033,#52034,#52035,#52036,#52037,#52038,#52039,#52040,#52041,#52042,#52043,
#52044,#52045,#52046,#52047,#52048,#52049,#52050,#52051,#52052,#52053,#52054,
#52055,#52056,#52057,#52058,#52059,#52060,#52061,#52062,#52063,#52064,#52065,
#52066,#52067,#52068,#52069,#52070,#52071,#52072,#52073,#52074,#52075,#52076,
#52077,#52078,#52079,#52080,#52081,#52082,#52083,#52084,#52085,#52086,#52087,
#52088,#52089,#52090,#52091,#52092,#52093,#52094,#52095,#52096,#52097,#52098,
#52099,#52100,#52101,#52102,#52103,#52104,#52105,#52106,#52107,#52108,#52109,
#52110,#52111,#52112,#52113,#52114,#52115,#52116,#52117),.UNSPECIFIED.,
 .F.,.F.,(4,3,3,3,3,3,3,3,3,3,3,3,3,3,3,3,3,3,3,3,3,3,3,3,3,3,3,3,3,3,3,
3,3,3,3,3,3,3,3,3,3,3,3,3,3,3,3,3,4),(0.0457216170362868,0.0459525676539145,
0.0460510633987835,0.0462662552838245,0.046373851226345,0.0463932769063991,
0.0464814471688656,0.0465034399505402,0.0466136393573502,0.046834101971899,
0.0469118309389477,0.0473422147090298,0.0477171542116892,0.047772598479112,
0.0482029822491941,0.0486019149928958,0.0486333660192762,0.0490448701065293,
0.0490637497893583,0.0491175477606186,0.0491556645204495,0.0491713457318789,
0.0492664939120745,0.0492789416743994,0.0494882446468033,0.0499245173295227,
0.0503549010996049,0.0503763267500335,0.0507852848696871,0.0512156686397693,
0.0512657528394623,0.0516460524098514,0.0520764361799336,0.0521560599808391,
0.0522673906331406,0.0522916280649747,0.0523787273298763,0.0523992240074953,
0.0525068199500158,0.0526013663393763,0.052937203720098,0.05304644767749,
0.0533675874901802,0.0537979712602624,0.0539356438209761,0.0542283550303446,
0.0546587388004268,0.0548232174784346,0.055089122570509),.UNSPECIFIED.);
#957=B_SPLINE_CURVE_WITH_KNOTS('',3,(#52126,#52127,#52128,#52129,#52130,
#52131),.UNSPECIFIED.,.F.,.F.,(4,2,4),(-0.349779142867042,-0.290997733300589,
-0.252766120019253),.UNSPECIFIED.);
#958=B_SPLINE_CURVE_WITH_KNOTS('',3,(#52145,#52146,#52147,#52148,#52149,
#52150,#52151,#52152,#52153,#52154,#52155,#52156,#52157,#52158,#52159,#52160,
#52161,#52162),.UNSPECIFIED.,.F.,.F.,(4,2,2,2,2,2,2,2,4),(-1.81830740171076,
-1.66679770229951,-1.51528800288825,-1.36374646868162,-1.21220493447498,
-1.06066340026809,-0.909121866061206,-0.757612166650203,-0.606102467239199),
 .UNSPECIFIED.);
#959=B_SPLINE_CURVE_WITH_KNOTS('',3,(#52163,#52164,#52165,#52166,#52167,
#52168,#52169,#52170,#52171,#52172,#52173,#52174,#52175,#52176,#52177,#52178,
#52179,#52180,#52181),.UNSPECIFIED.,.F.,.F.,(4,2,2,2,3,2,2,2,4),(-0.606102467239199,
-0.454592767826692,-0.303083068414184,-0.151541534207092,0.,0.151541534207344,
0.303083068414688,0.454592767826944,0.6061024672392),.UNSPECIFIED.);
#960=B_SPLINE_CURVE_WITH_KNOTS('',3,(#52184,#52185,#52186,#52187,#52188,
#52189,#52190,#52191,#52192,#52193,#52194,#52195,#52196,#52197,#52198,#52199,
#52200,#52201,#52202),.UNSPECIFIED.,.F.,.F.,(4,2,2,2,3,2,2,2,4),(1.81830740171076,
1.96981710112327,2.12132680053578,2.27286833474287,2.42440986894996,2.57595140315705,
2.72749293736415,2.87900263677665,3.03051233618916),.UNSPECIFIED.);
#961=B_SPLINE_CURVE_WITH_KNOTS('',3,(#52203,#52204,#52205,#52206,#52207,
#52208,#52209,#52210,#52211,#52212,#52213,#52214,#52215,#52216,#52217,#52218,
#52219,#52220),.UNSPECIFIED.,.F.,.F.,(4,2,2,2,2,2,2,2,4),(3.03051233618916,
3.18202203560017,3.33353173501117,3.48507326921806,3.63661480342494,3.78815633763183,
3.93969787183872,4.09120757124972,4.24271727066072),.UNSPECIFIED.);
#962=B_SPLINE_CURVE_WITH_KNOTS('',3,(#53022,#53023,#53024,#53025,#53026,
#53027,#53028,#53029,#53030,#53031,#53032,#53033,#53034,#53035,#53036,#53037,
#53038,#53039,#53040,#53041,#53042,#53043,#53044,#53045,#53046,#53047,#53048,
#53049,#53050,#53051,#53052,#53053,#53054,#53055,#53056,#53057,#53058,#53059,
#53060,#53061,#53062,#53063,#53064,#53065,#53066,#53067,#53068,#53069,#53070,
#53071,#53072,#53073,#53074,#53075,#53076,#53077,#53078,#53079,#53080,#53081,
#53082,#53083,#53084,#53085,#53086,#53087,#53088,#53089,#53090,#53091,#53092,
#53093,#53094,#53095,#53096,#53097,#53098,#53099,#53100,#53101,#53102,#53103,
#53104,#53105,#53106,#53107,#53108,#53109,#53110,#53111,#53112,#53113,#53114,
#53115,#53116,#53117,#53118,#53119,#53120,#53121,#53122,#53123,#53124,#53125,
#53126,#53127,#53128,#53129,#53130,#53131,#53132,#53133,#53134,#53135,#53136,
#53137,#53138,#53139,#53140,#53141,#53142,#53143,#53144,#53145,#53146,#53147,
#53148,#53149,#53150,#53151,#53152,#53153,#53154,#53155,#53156,#53157,#53158,
#53159,#53160,#53161,#53162,#53163,#53164,#53165,#53166,#53167,#53168,#53169,
#53170,#53171,#53172,#53173,#53174,#53175,#53176,#53177,#53178,#53179,#53180,
#53181,#53182,#53183,#53184,#53185,#53186,#53187,#53188,#53189,#53190,#53191,
#53192,#53193,#53194,#53195,#53196,#53197,#53198,#53199,#53200,#53201,#53202,
#53203,#53204,#53205,#53206,#53207,#53208,#53209,#53210,#53211,#53212,#53213,
#53214,#53215,#53216,#53217,#53218,#53219,#53220,#53221,#53222,#53223,#53224,
#53225,#53226,#53227,#53228,#53229,#53230,#53231,#53232,#53233,#53234,#53235,
#53236,#53237,#53238,#53239,#53240,#53241,#53242,#53243,#53244,#53245,#53246,
#53247,#53248,#53249,#53250,#53251,#53252,#53253,#53254,#53255,#53256,#53257,
#53258,#53259,#53260,#53261,#53262,#53263,#53264,#53265,#53266,#53267,#53268,
#53269,#53270,#53271,#53272,#53273,#53274,#53275,#53276,#53277,#53278,#53279,
#53280,#53281,#53282,#53283,#53284,#53285,#53286,#53287,#53288,#53289,#53290,
#53291,#53292,#53293,#53294,#53295,#53296,#53297,#53298,#53299,#53300,#53301,
#53302,#53303,#53304,#53305,#53306,#53307,#53308,#53309,#53310,#53311,#53312,
#53313,#53314,#53315,#53316,#53317,#53318,#53319,#53320,#53321,#53322,#53323,
#53324,#53325,#53326,#53327,#53328,#53329,#53330,#53331,#53332,#53333,#53334,
#53335,#53336,#53337,#53338,#53339,#53340,#53341,#53342,#53343,#53344,#53345,
#53346,#53347,#53348,#53349,#53350,#53351,#53352,#53353,#53354,#53355,#53356,
#53357,#53358,#53359,#53360,#53361,#53362,#53363,#53364,#53365,#53366,#53367,
#53368,#53369,#53370,#53371,#53372,#53373,#53374,#53375,#53376,#53377,#53378,
#53379,#53380,#53381,#53382,#53383,#53384,#53385,#53386,#53387,#53388,#53389,
#53390,#53391,#53392,#53393,#53394,#53395,#53396,#53397,#53398,#53399,#53400,
#53401,#53402,#53403,#53404,#53405,#53406,#53407,#53408,#53409,#53410,#53411,
#53412,#53413,#53414,#53415,#53416,#53417,#53418),.UNSPECIFIED.,.F.,.F.,
(4,3,3,3,3,3,3,3,3,3,3,3,3,3,3,3,3,3,3,3,3,3,3,3,3,3,3,3,3,3,3,3,3,3,3,
3,3,3,3,3,3,3,3,3,3,3,3,3,3,3,3,3,3,3,3,3,3,3,3,3,3,3,3,3,3,3,3,3,3,3,3,
3,3,3,3,3,3,3,3,3,3,3,3,3,3,3,3,3,3,3,3,3,3,3,3,3,3,3,3,3,3,3,3,3,3,3,3,
3,3,3,3,3,3,3,3,3,3,3,3,3,3,3,3,3,3,3,3,3,3,3,3,3,4),(0.000484419199971794,
0.000627975952031815,0.000633556641722834,0.000937055221123302,0.000941963928047723,
0.00124047713506422,0.00125595190406363,0.0015438228113822,0.00156993988007954,
0.00172693386808749,0.00180543086209147,0.00184712765684463,0.00188392785609545,
0.0019231050380993,0.00199911452758639,0.00215120575891999,0.00219791583211137,
0.00245570735767525,0.00251190380812729,0.00276063659439479,0.00282589178414321,
0.00313987976015913,0.00337182000724591,0.00345386773617505,0.00352490446840894,
0.00353236473017903,0.00361086172418301,0.00367813944513374,0.00376785571219098,
0.00398516274434557,0.0040818436882069,0.00439583166422282,0.00460142477316655,
0.00470981964023874,0.00491068197299154,0.00502380761625467,0.00506559805970609,
0.005143130947568,0.00518080160426262,0.00522005010126462,0.00522070868137605,
0.00525929859826661,0.00565178356828666,0.00584312899461437,0.00596577154430269,
0.00627975952031873,0.00646865865529118,0.00690773547235079,0.00709724487102262,
0.00717602996170373,0.00722172344836684,0.00725485607089141,0.00730022044237085,
0.00737871743637487,0.00741262727130941,0.00753571142438291,0.00772857997468013,
0.00816368737641506,0.00836205996678017,0.00879166332844721,0.00899754377132439,
0.00941963928047937,0.0096349306909179,0.00973362725649546,0.00979456994957919,
0.0098906212445035,0.00995430020341104,0.0100476152325115,0.010273940467961,
0.0106755911845437,0.0109137046578717,0.0113035671365759,0.0115540605555347,
0.0119315430886081,0.0121949278647927,0.0125595190406403,0.0128362231911716,
0.0131570039176619,0.0131874949926725,0.0133174226179354,0.0133444889806806,
0.0134778312741732,0.0135014829686886,0.0138154709447047,0.0141189436345339,
0.0144434468967369,0.0147591048294073,0.0150714228487691,0.0153981466426708,
0.0156993988008013,0.0160133867768174,0.0160358430959,0.0163273747528335,
0.0163540945915774,0.0164843687408416,0.0165130520803898,0.0165628657348456,
0.0166413627288497,0.0166718779414906,0.0169553507048658,0.0172693386808819,
0.0173052583666035,0.0175833266568981,0.0176206583646067,0.0178973146329142,
0.0179350856965279,0.0182113026089303,0.0182484317842081,0.0184046583785325,
0.0184826536878379,0.0185252905849465,0.0185605610228719,0.0185645390819485,
0.0186037875789505,0.0186822845729545,0.0188392785609626,0.0188708516293508,
0.0191532665369787,0.0191787177616934,0.0194672545129949,0.0194839639398301,
0.0196242485010029,0.019663496998005,0.019702745495007,0.019781242489011,
0.019786707220997,0.0199382364770191,0.0199386450109174,0.0200149458360611,
0.0200167334710231,0.0200913742141244,0.0200952304650272,0.0203967023487183),
 .UNSPECIFIED.);
#963=B_SPLINE_CURVE_WITH_KNOTS('',3,(#53436,#53437,#53438,#53439,#53440,
#53441,#53442,#53443,#53444,#53445),.UNSPECIFIED.,.F.,.F.,(4,2,2,2,4),(-0.0798726046250498,
-0.058584918995045,-0.0372972333650401,-0.0186486166825216,-3.09474668114262E-15),
 .UNSPECIFIED.);
#964=B_SPLINE_CURVE_WITH_KNOTS('',3,(#53449,#53450,#53451,#53452,#53453,
#53454,#53455,#53456,#53457,#53458),.UNSPECIFIED.,.F.,.F.,(4,2,2,2,4),(0.,
0.0191590048998788,0.0383180097997576,0.0590954157667988,0.07987282173384),
 .UNSPECIFIED.);
#965=B_SPLINE_CURVE_WITH_KNOTS('',3,(#53462,#53463,#53464,#53465,#53466,
#53467,#53468,#53469,#53470,#53471),.UNSPECIFIED.,.F.,.F.,(4,2,2,2,4),(-0.0798726046250503,
-0.0585849189950454,-0.0372972333650404,-0.0186486166825219,-3.33066907387547E-15),
 .UNSPECIFIED.);
#966=B_SPLINE_CURVE_WITH_KNOTS('',3,(#53474,#53475,#53476,#53477,#53478,
#53479,#53480,#53481,#53482,#53483),.UNSPECIFIED.,.F.,.F.,(4,2,2,2,4),(-0.329829240504479,
-0.311180623821963,-0.292532007139446,-0.271244321509442,-0.249956635879439),
 .UNSPECIFIED.);
#967=B_SPLINE_CURVE_WITH_KNOTS('',3,(#53493,#53494,#53495,#53496,#53497,
#53498,#53499,#53500,#53501,#53502,#53503,#53504,#53505,#53506),
 .UNSPECIFIED.,.F.,.F.,(4,2,2,2,2,1,1,4),(0.,0.000277353300508432,0.000554706601016864,
0.000693383251271085,0.000728052413834634,0.000762721576398184,0.000832059901525293,
0.00110941320203372),.UNSPECIFIED.);
#968=B_SPLINE_CURVE_WITH_KNOTS('',3,(#53508,#53509,#53510,#53511,#53512,
#53513,#53514,#53515,#53516,#53517,#53518,#53519,#53520,#53521,#53522,#53523,
#53524,#53525,#53526,#53527,#53528,#53529,#53530,#53531,#53532,#53533,#53534,
#53535),.UNSPECIFIED.,.F.,.F.,(4,3,3,3,3,3,3,3,3,4),(-0.000640854183641207,
-0.000630840837021816,-0.000620827490402424,-0.000600800797163639,-0.00059215928153463,
-0.000560747410686068,-0.000480640637730918,-0.000320427091820608,-0.000103815349030914,
0.),.UNSPECIFIED.);
#969=B_SPLINE_CURVE_WITH_KNOTS('',3,(#53536,#53537,#53538,#53539,#53540,
#53541,#53542,#53543,#53544,#53545,#53546,#53547,#53548,#53549,#53550,#53551,
#53552,#53553,#53554,#53555,#53556,#53557,#53558,#53559,#53560,#53561,#53562,
#53563,#53564,#53565,#53566),.UNSPECIFIED.,.F.,.F.,(4,3,3,3,3,3,3,3,3,3,
4),(0.000821733649844019,0.00095608668379176,0.00102326333982933,0.00109043999586689,
0.00115888309266042,0.00122479330794202,0.00129196996397958,0.00132555829199836,
0.00134235245600775,0.00135074953801244,0.00135914662001713),
 .UNSPECIFIED.);
#970=B_SPLINE_CURVE_WITH_KNOTS('',3,(#53570,#53571,#53572,#53573,#53574,
#53575,#53576,#53577,#53578,#53579,#53580,#53581),.UNSPECIFIED.,.F.,.F.,
(4,2,2,2,2,4),(-3.10489780410495,-3.10241912589423,-3.00106326608238,-2.79835154645867,
-2.60059139286912,-2.40283123927957),.UNSPECIFIED.);
#971=B_SPLINE_CURVE_WITH_KNOTS('',3,(#53583,#53584,#53585,#53586,#53587,
#53588,#53589,#53590,#53591,#53592,#53593,#53594,#53595,#53596,#53597,#53598,
#53599,#53600,#53601,#53602,#53603,#53604),.UNSPECIFIED.,.F.,.F.,(4,2,2,
2,2,2,2,2,2,2,4),(0.800943746426511,0.998703900016066,1.19646405360562,
1.39917577322933,1.50053163304119,1.60188749285304,1.70324335266489,1.80459921247675,
2.00731093210046,2.20507108569001,2.35815643982996),.UNSPECIFIED.);
#972=B_SPLINE_CURVE_WITH_KNOTS('',3,(#53606,#53607,#53608,#53609,#53610,
#53611,#53612,#53613,#53614,#53615,#53616,#53617,#53618,#53619,#53620,#53621,
#53622,#53623,#53624),.UNSPECIFIED.,.F.,.F.,(4,3,3,3,3,3,4),(0.00615127099246931,
0.00628627180839864,0.00635377221636331,0.00642127262432798,0.00669127425618666,
0.00696127588804534,0.00723127751990402),.UNSPECIFIED.);
#973=B_SPLINE_CURVE_WITH_KNOTS('',3,(#53626,#53627,#53628,#53629,#53630,
#53631,#53632,#53633,#53634,#53635,#53636,#53637,#53638,#53639,#53640,#53641,
#53642,#53643,#53644,#53645,#53646,#53647,#53648,#53649,#53650,#53651,#53652,
#53653,#53654,#53655,#53656,#53657,#53658,#53659,#53660,#53661,#53662,#53663,
#53664,#53665,#53666,#53667,#53668,#53669,#53670,#53671,#53672,#53673,#53674,
#53675,#53676,#53677,#53678,#53679,#53680,#53681,#53682,#53683),
 .UNSPECIFIED.,.F.,.F.,(4,3,3,3,3,3,3,3,3,3,3,3,3,3,3,3,3,3,3,4),(0.00228250782718276,
0.00261772248031453,0.00276610322284359,0.00288700207175879,0.003007900920674,
0.00324969861850441,0.00357540633747326,0.00373329401416523,0.00406460842083867,
0.00421688940982604,0.00445868710765645,0.00451913653211405,0.00457958595657165,
0.00470048480548686,0.00502296949144011,0.00518408020114767,0.00542587789897808,
0.00566767559680849,0.0059094732946389,0.00615127099246931),
 .UNSPECIFIED.);
#974=B_SPLINE_CURVE_WITH_KNOTS('',3,(#53687,#53688,#53689,#53690,#53691,
#53692,#53693,#53694,#53695,#53696,#53697,#53698,#53699,#53700,#53701,#53702,
#53703,#53704,#53705,#53706),.UNSPECIFIED.,.F.,.F.,(4,2,2,2,2,2,2,2,2,4),
(0.850611926930939,0.998703900016074,1.19646405360563,1.39917577322933,
1.50053163304119,1.60188749285304,1.7032433526649,1.80459921247675,2.00731093210046,
2.1806981097713),.UNSPECIFIED.);
#975=B_SPLINE_CURVE_WITH_KNOTS('',3,(#53714,#53715,#53716,#53717,#53718,
#53719,#53720,#53721,#53722,#53723,#53724,#53725,#53726,#53727,#53728,#53729,
#53730,#53731,#53732,#53733,#53734,#53735,#53736,#53737,#53738,#53739,#53740,
#53741,#53742),.UNSPECIFIED.,.F.,.F.,(4,2,2,2,2,2,2,2,3,2,2,2,2,4),(-1.31557498404543,
-1.19646405360563,-0.998703900016074,-0.80094374642652,-0.603183592836967,
-0.405423439247414,-0.202711719623707,-0.101355859811853,0.,0.101355859811854,
0.202711719623707,0.405423439247413,0.603183592836967,0.756268946977335),
 .UNSPECIFIED.);
#976=B_SPLINE_CURVE_WITH_KNOTS('',3,(#53743,#53744,#53745,#53746,#53747,
#53748,#53749,#53750,#53751,#53752,#53753,#53754,#53755,#53756,#53757,#53758,
#53759,#53760,#53761,#53762,#53763,#53764,#53765,#53766,#53767,#53768,#53769,
#53770,#53771,#53772,#53773,#53774,#53775,#53776,#53777,#53778,#53779,#53780,
#53781,#53782,#53783,#53784,#53785,#53786,#53787,#53788,#53789,#53790,#53791,
#53792,#53793,#53794,#53795,#53796,#53797,#53798,#53799,#53800,#53801,#53802,
#53803,#53804,#53805,#53806,#53807,#53808,#53809,#53810,#53811,#53812),
 .UNSPECIFIED.,.F.,.F.,(4,3,3,3,3,3,3,3,3,3,3,3,3,3,3,3,3,3,3,3,3,3,3,4),
(0.00228250782718277,0.00259180593297786,0.00274645498587541,0.00282377951232418,
0.00290110403877294,0.00321040214456803,0.00351970025036311,0.0038289983561582,
0.00413829646195329,0.00444759456774837,0.00452491909419713,0.0046022436206459,
0.00475689267354343,0.0050661907793385,0.00537548888513356,0.00568478699092863,
0.0059940850967237,0.0062772128484052,0.00630338320251876,0.00638070772896753,
0.00645803225541631,0.00661268130831385,0.00692197941410894,0.00723127751990404),
 .UNSPECIFIED.);
#977=B_SPLINE_CURVE_WITH_KNOTS('',3,(#53813,#53814,#53815,#53816,#53817,
#53818,#53819,#53820,#53821,#53822,#53823,#53824,#53825,#53826,#53827,#53828,
#53829,#53830,#53831,#53832,#53833),.UNSPECIFIED.,.F.,.F.,(4,2,2,2,2,3,
2,2,2,4),(2.44750603872918,2.60059139286912,2.79835154645867,3.00106326608238,
3.10241912589423,3.20377498570608,3.30513084551794,3.40648670532979,3.6091984249535,
3.78258560262431),.UNSPECIFIED.);
#978=B_SPLINE_CURVE_WITH_KNOTS('',3,(#53838,#53839,#53840,#53841,#53842,
#53843),.UNSPECIFIED.,.F.,.F.,(4,2,4),(-1.75663608064087,-1.67778100951734,
-1.61558523752689),.UNSPECIFIED.);
#979=B_SPLINE_CURVE_WITH_KNOTS('',3,(#53845,#53846,#53847,#53848,#53849,
#53850,#53851,#53852,#53853,#53854,#53855,#53856,#53857,#53858,#53859,#53860,
#53861,#53862,#53863,#53864,#53865,#53866,#53867,#53868,#53869,#53870,#53871,
#53872,#53873,#53874,#53875,#53876,#53877,#53878,#53879,#53880,#53881,#53882,
#53883,#53884,#53885,#53886,#53887,#53888,#53889,#53890,#53891,#53892,#53893,
#53894,#53895,#53896,#53897,#53898,#53899,#53900,#53901,#53902,#53903,#53904,
#53905,#53906,#53907,#53908,#53909,#53910,#53911,#53912,#53913,#53914,#53915,
#53916,#53917,#53918,#53919,#53920,#53921,#53922,#53923,#53924,#53925,#53926,
#53927,#53928,#53929,#53930,#53931,#53932,#53933,#53934,#53935,#53936,#53937,
#53938,#53939,#53940,#53941,#53942,#53943,#53944,#53945,#53946,#53947,#53948,
#53949,#53950),.UNSPECIFIED.,.F.,.F.,(4,3,3,3,3,3,3,3,3,3,3,3,3,3,3,3,3,
3,3,3,3,3,3,3,3,3,3,3,3,3,3,3,3,3,3,4),(0.0305709307873588,0.0306063950419885,
0.0306418592966182,0.0307023678095767,0.0307127878058775,0.0308370374836857,
0.0308546448243963,0.0309745186599934,0.0311143035117337,0.0311383588614337,
0.031350416372114,0.0313990237158669,0.0314220728984712,0.031639460489526,
0.0316879165996665,0.0317057869355086,0.0319209128177052,0.03197751646506,
0.0319895009725461,0.0320604294818055,0.0321313579910648,0.0322664035810511,
0.0322732150095836,0.0324971762357835,0.0325549976396122,0.0325569290466211,
0.0326983162209017,0.0326987860651398,0.0327695930842391,0.0327697145743992,
0.0328051206407264,0.0328051788290289,0.0328229109563437,0.0328317770200012,
0.0328362100518299,0.0328406430836586),.UNSPECIFIED.);
#980=B_SPLINE_CURVE_WITH_KNOTS('',3,(#53951,#53952,#53953,#53954,#53955,
#53956,#53957,#53958,#53959,#53960,#53961,#53962,#53963,#53964,#53965,#53966,
#53967,#53968,#53969,#53970,#53971,#53972,#53973,#53974,#53975,#53976,#53977,
#53978,#53979,#53980,#53981,#53982,#53983,#53984,#53985,#53986,#53987,#53988,
#53989,#53990,#53991,#53992,#53993,#53994,#53995,#53996,#53997,#53998,#53999,
#54000,#54001,#54002,#54003,#54004,#54005,#54006,#54007,#54008,#54009,#54010,
#54011,#54012,#54013,#54014,#54015,#54016,#54017,#54018,#54019,#54020,#54021,
#54022,#54023,#54024,#54025,#54026,#54027,#54028,#54029,#54030,#54031,#54032,
#54033,#54034,#54035),.UNSPECIFIED.,.F.,.F.,(4,3,3,3,3,3,3,3,3,3,3,3,3,
3,3,3,3,3,3,3,3,3,3,3,3,3,3,3,4),(2.5816516038653E-11,3.54600608128747E-5,
3.56641847997305E-5,7.10560249003594E-5,0.000142556163497147,0.000285313478397844,
0.000286667929283135,0.000508969327732133,0.000570626956795688,0.000578229350350693,
0.000800126093089386,0.000855940435193532,0.000871807784634396,0.0010892321962361,
0.00114125391359138,0.00116414093555289,0.00137785778404045,0.00142656739198922,
0.00145179194908138,0.00146223157678895,0.00149789576158867,0.00156922413118814,
0.00171188087038706,0.00173474788861624,0.00187461379195942,0.00199719434878491,
0.00201280376719228,0.00214889827835077,0.00228250782718276),
 .UNSPECIFIED.);
#981=B_SPLINE_CURVE_WITH_KNOTS('',3,(#54042,#54043,#54044,#54045,#54046,
#54047,#54048,#54049,#54050,#54051,#54052,#54053,#54054,#54055,#54056,#54057,
#54058,#54059,#54060,#54061,#54062,#54063),.UNSPECIFIED.,.F.,.F.,(4,2,2,
2,2,2,2,2,2,2,4),(0.427651316099875,0.508717953234535,0.577778895492431,
0.646839837750328,0.694519804488737,0.742199771227145,0.837559704703962,
0.981848513434963,1.12613732216597,1.41471493962797,1.47691071161843),
 .UNSPECIFIED.);
#982=B_SPLINE_CURVE_WITH_KNOTS('',3,(#54066,#54067,#54068,#54069,#54070,
#54071),.UNSPECIFIED.,.F.,.F.,(4,2,4),(0.0698399460344426,0.254358976617267,
0.427651316099875),.UNSPECIFIED.);
#983=B_SPLINE_CURVE_WITH_KNOTS('',3,(#54072,#54073,#54074,#54075,#54076,
#54077,#54078,#54079,#54080,#54081,#54082,#54083,#54084,#54085,#54086,#54087,
#54088,#54089,#54090,#54091,#54092,#54093,#54094,#54095,#54096,#54097,#54098,
#54099,#54100,#54101,#54102,#54103,#54104,#54105,#54106,#54107,#54108,#54109,
#54110,#54111,#54112,#54113,#54114,#54115,#54116,#54117,#54118,#54119,#54120,
#54121,#54122,#54123,#54124,#54125,#54126,#54127,#54128,#54129,#54130,#54131,
#54132,#54133,#54134,#54135,#54136,#54137,#54138,#54139,#54140,#54141,#54142,
#54143,#54144,#54145,#54146,#54147,#54148,#54149,#54150,#54151,#54152,#54153,
#54154,#54155,#54156,#54157,#54158,#54159,#54160,#54161,#54162,#54163,#54164,
#54165,#54166,#54167,#54168,#54169,#54170,#54171,#54172,#54173,#54174,#54175,
#54176,#54177,#54178,#54179,#54180,#54181,#54182,#54183,#54184,#54185,#54186,
#54187,#54188,#54189,#54190,#54191,#54192,#54193,#54194,#54195,#54196,#54197,
#54198,#54199,#54200,#54201,#54202,#54203,#54204,#54205,#54206,#54207,#54208,
#54209,#54210,#54211,#54212,#54213,#54214,#54215,#54216,#54217,#54218,#54219,
#54220,#54221,#54222,#54223,#54224,#54225,#54226,#54227,#54228,#54229,#54230,
#54231,#54232,#54233,#54234,#54235,#54236,#54237,#54238,#54239,#54240,#54241,
#54242,#54243,#54244,#54245,#54246,#54247,#54248,#54249,#54250,#54251,#54252,
#54253,#54254,#54255,#54256,#54257,#54258,#54259,#54260,#54261,#54262,#54263,
#54264,#54265,#54266,#54267,#54268,#54269,#54270,#54271,#54272,#54273,#54274,
#54275,#54276,#54277,#54278,#54279,#54280,#54281,#54282,#54283,#54284,#54285,
#54286,#54287,#54288,#54289,#54290,#54291,#54292,#54293,#54294,#54295,#54296,
#54297,#54298,#54299,#54300,#54301,#54302,#54303,#54304,#54305,#54306,#54307,
#54308,#54309,#54310,#54311,#54312,#54313,#54314,#54315,#54316,#54317,#54318,
#54319,#54320,#54321,#54322,#54323,#54324,#54325,#54326,#54327,#54328,#54329,
#54330,#54331,#54332,#54333,#54334,#54335,#54336,#54337,#54338,#54339,#54340,
#54341,#54342,#54343,#54344,#54345,#54346,#54347,#54348,#54349,#54350,#54351,
#54352,#54353,#54354,#54355,#54356,#54357,#54358,#54359,#54360,#54361,#54362,
#54363,#54364,#54365,#54366,#54367,#54368,#54369,#54370,#54371,#54372,#54373,
#54374,#54375,#54376,#54377,#54378,#54379,#54380,#54381,#54382,#54383,#54384,
#54385,#54386,#54387,#54388,#54389,#54390,#54391,#54392,#54393,#54394,#54395,
#54396,#54397,#54398,#54399,#54400,#54401,#54402,#54403,#54404,#54405,#54406,
#54407,#54408,#54409,#54410,#54411,#54412,#54413,#54414,#54415,#54416,#54417,
#54418,#54419,#54420,#54421,#54422,#54423,#54424,#54425,#54426,#54427,#54428,
#54429,#54430,#54431,#54432,#54433,#54434,#54435,#54436,#54437,#54438,#54439,
#54440,#54441,#54442,#54443,#54444,#54445,#54446,#54447,#54448,#54449,#54450,
#54451,#54452,#54453,#54454,#54455,#54456,#54457,#54458,#54459,#54460,#54461,
#54462,#54463,#54464,#54465,#54466,#54467,#54468,#54469,#54470,#54471,#54472,
#54473,#54474,#54475,#54476,#54477,#54478,#54479,#54480,#54481,#54482,#54483,
#54484,#54485,#54486,#54487,#54488,#54489,#54490,#54491,#54492,#54493,#54494,
#54495,#54496,#54497,#54498),.UNSPECIFIED.,.F.,.F.,(4,3,3,3,3,3,3,3,3,3,
3,3,3,3,3,3,3,3,3,3,3,3,3,3,3,3,3,3,3,3,3,3,3,3,3,3,3,3,3,3,3,3,3,3,3,3,
3,3,3,3,3,3,3,3,3,3,3,3,3,3,3,3,3,3,3,3,3,3,3,3,3,3,3,3,3,3,3,3,3,3,3,3,
3,3,3,3,3,3,3,3,3,3,3,3,3,3,3,3,3,3,3,3,3,3,3,3,3,3,3,3,3,3,3,3,3,3,3,3,
3,3,3,3,3,3,3,3,3,3,3,3,3,3,3,3,3,3,3,3,3,3,3,3,4),(0.0206286231325014,
0.0206447094230554,0.0206839579200574,0.0207013849168472,0.0207232064170594,
0.0210060975778275,0.0210371943930756,0.0213114656590281,0.0213511823690917,
0.0216174688377158,0.0216651703451078,0.0216940599097884,0.0217436673391119,
0.021770732718017,0.0218221643331159,0.0219243902561196,0.021979158321124,
0.0222328665245741,0.0222931462971402,0.0225427671520463,0.0226071342731563,
0.0227641282611644,0.0228426252551685,0.0228539704164397,0.0228818737521705,
0.0229211222491725,0.0229319636339267,0.0230100441327226,0.0231664468356769,
0.0232351102251887,0.0234801808337334,0.0235490982012049,0.0237950373987436,
0.0238630861772211,0.0241109051815931,0.0241770741532372,0.024427705018772,
0.0244910621292534,0.0245695591232575,0.0245864047557396,0.0246480561172615,
0.0247452759130522,0.0248050501052696,0.0251190380812858,0.0253821615172229,
0.025433026057302,0.0257470140333182,0.0260209637001603,0.0263749899853506,
0.0266613596160773,0.0269820800759253,0.027002965937383,0.0271425602282344,
0.0271599599253911,0.0272228290434084,0.0272384569193951,0.0273031166709421,
0.0273169539133992,0.0276309418894154,0.0279454744899221,0.0282589178414478,
0.0285877913758882,0.0288868937934803,0.0292299702284112,0.0295148697455127,
0.02987192891183,0.0301428456975452,0.0305135974218362,0.0307708216495776,
0.0308343041148486,0.0309278156375857,0.0309946223687894,0.0310063126315898,
0.0310848096255938,0.0311548982142129,0.03139879760161,0.0317950926599704,
0.0320267735536425,0.0324336477724454,0.032654749505675,0.0330705169098406,
0.0332827254577074,0.0337056378092121,0.0338641371581584,0.0339107014097399,
0.033943344025685,0.0339891984037439,0.034022518463526,0.0340676953977479,
0.034224689385756,0.0343388083882488,0.0345386773617722,0.0349693595359445,
0.0351666533138045,0.0354806412898207,0.0355972043577933,0.0357537404841202,
0.0357946292658369,0.0358319417780599,0.0358731262598409,0.0359101028303693,
0.035951623253845,0.0361086172418531,0.0362222760339768,0.0364226052178693,
0.0367365931938856,0.0368444295298401,0.0370505811699018,0.0373645691459181,
0.0374430661399221,0.0374637324729354,0.0375215631339262,0.0375409504156616,
0.0376181302752573,0.0376785571219343,0.0377723740804822,0.0379925450979505,
0.0380804310369398,0.0383065330739667,0.0386205210499829,0.0386948655346232,
0.0389345090259991,0.0390012628917026,0.0390130060200032,0.0390522545170052,
0.0390777695532355,0.0390915030140073,0.0391542118436117,0.0392484970020154,
0.0393068924677751,0.0395624849780316,0.0396114511725609,0.0398764729540479,
0.039914949116982,0.040033466942056,0.0401708366815631,0.0401904609300641,
0.0402173631023923,0.0403685816462537,0.0404444323885405,0.040482420371629,
0.04050444890608,0.040520443503722),.UNSPECIFIED.);
#984=B_SPLINE_CURVE_WITH_KNOTS('',3,(#54568,#54569,#54570,#54571,#54572,
#54573,#54574,#54575,#54576,#54577,#54578,#54579,#54580,#54581,#54582,#54583,
#54584,#54585,#54586,#54587,#54588,#54589,#54590,#54591,#54592,#54593,#54594,
#54595,#54596,#54597,#54598,#54599,#54600,#54601,#54602,#54603,#54604,#54605,
#54606,#54607,#54608,#54609,#54610,#54611,#54612,#54613,#54614,#54615,#54616,
#54617,#54618,#54619,#54620,#54621,#54622,#54623,#54624,#54625,#54626,#54627,
#54628,#54629,#54630,#54631),.UNSPECIFIED.,.F.,.F.,(4,3,3,3,3,3,3,3,3,3,
3,3,3,3,3,3,3,3,3,3,3,4),(0.,6.36402803474462E-5,0.000127280560694892,0.000159100700868616,
0.00017501077095548,0.000190920841042344,0.000254561121389809,0.000318201401737275,
0.000334111471824142,0.000350021541911008,0.000381841682084741,0.000445481962432199,
0.000477302102605929,0.000493212172692793,0.000509122242779658,0.000572762523127108,
0.000636402803474558,0.000668222943648282,0.00068413301373514,0.000700043083821997,
0.000763683364169407,0.000782835047457224),.UNSPECIFIED.);
#985=B_SPLINE_CURVE_WITH_KNOTS('',3,(#54633,#54634,#54635,#54636,#54637,
#54638,#54639,#54640,#54641,#54642,#54643,#54644,#54645,#54646,#54647),
 .UNSPECIFIED.,.F.,.F.,(4,2,2,1,2,2,1,1,4),(0.000782835047457224,0.000827323644516816,
0.000843233714603663,0.000859143784690511,0.000890963924864205,0.000954604205211594,
0.000986424345385289,0.00100233441547213,0.00101824448555897),
 .UNSPECIFIED.);
#986=B_SPLINE_CURVE_WITH_KNOTS('',3,(#54648,#54649,#54650,#54651,#54652,
#54653,#54654,#54655,#54656,#54657,#54658,#54659,#54660,#54661,#54662,#54663,
#54664,#54665,#54666,#54667,#54668,#54669,#54670,#54671,#54672,#54673,#54674,
#54675,#54676,#54677,#54678,#54679,#54680,#54681,#54682,#54683,#54684,#54685,
#54686,#54687),.UNSPECIFIED.,.F.,.F.,(4,3,3,3,3,3,3,3,3,3,3,3,3,4),(3.25260651745651E-19,
3.42965330670762E-5,6.88862345657144E-5,0.000138341881978896,0.000207969419140507,
0.000225387427278471,0.000242804328229345,0.000277624644722789,0.000347060433943642,
0.000381766477338011,0.000399119499035193,0.000416472520732376,0.000485836343494754,
0.000555296694309835),.UNSPECIFIED.);
#987=B_SPLINE_CURVE_WITH_KNOTS('',3,(#54698,#54699,#54700,#54701,#54702,
#54703,#54704,#54705,#54706,#54707,#54708,#54709,#54710,#54711,#54712,#54713,
#54714,#54715,#54716,#54717,#54718,#54719,#54720,#54721,#54722,#54723,#54724,
#54725,#54726,#54727,#54728,#54729,#54730,#54731,#54732,#54733,#54734,#54735,
#54736,#54737,#54738,#54739,#54740,#54741,#54742,#54743,#54744,#54745,#54746,
#54747,#54748,#54749,#54750,#54751,#54752,#54753,#54754,#54755,#54756,#54757,
#54758,#54759,#54760,#54761,#54762,#54763,#54764,#54765,#54766,#54767,#54768,
#54769,#54770,#54771,#54772,#54773,#54774,#54775,#54776,#54777,#54778,#54779,
#54780,#54781,#54782,#54783,#54784,#54785,#54786,#54787,#54788,#54789,#54790,
#54791,#54792,#54793,#54794,#54795,#54796,#54797,#54798,#54799,#54800,#54801,
#54802,#54803,#54804,#54805,#54806,#54807,#54808,#54809,#54810,#54811,#54812,
#54813,#54814,#54815,#54816,#54817,#54818,#54819,#54820,#54821,#54822,#54823,
#54824,#54825,#54826,#54827,#54828,#54829,#54830,#54831,#54832,#54833),
 .UNSPECIFIED.,.F.,.F.,(4,3,3,3,3,3,3,3,3,3,3,3,3,3,3,3,3,3,3,3,3,3,3,3,
3,3,3,3,3,3,3,3,3,3,3,3,3,3,3,3,3,3,3,3,3,4),(0.,4.91689726004813E-5,5.05531472505571E-5,
7.39482684633374E-5,7.58297208758408E-5,8.63848253908088E-5,9.88503858357188E-5,
0.000101106294501124,0.00014892407146761,0.00015165944175169,0.000199318832959595,
0.000202212589002255,0.000227489162627535,0.000249994600458649,0.000252765736252814,
0.000275444625287608,0.000300981075513535,0.000303318883503374,0.000352201416378833,
0.000353872030753934,0.000403559031113317,0.000404425178004494,0.000429260234366245,
0.000429701751629774,0.000454948636729993,0.000454978325255055,0.000505531472505623,
0.000506209072757505,0.000556084619756192,0.000557247649660384,0.000581361193381469,
0.000582659083595442,0.000593999480194102,0.000606637767006736,0.000607987133405275,
0.000657190914257281,0.000658445872483203,0.000707744061507826,0.00070863765270964,
0.00075829720875837,0.000758539102560875,0.000770935495570998,0.000770971495620867,
0.000783408714808202,0.000783573782383626,0.00080811238697951),
 .UNSPECIFIED.);
#988=B_SPLINE_CURVE_WITH_KNOTS('',3,(#54835,#54836,#54837,#54838,#54839,
#54840,#54841,#54842,#54843,#54844,#54845,#54846,#54847,#54848,#54849,#54850,
#54851,#54852,#54853,#54854,#54855,#54856,#54857,#54858,#54859,#54860,#54861,
#54862,#54863,#54864,#54865,#54866,#54867,#54868,#54869,#54870,#54871,#54872,
#54873,#54874,#54875,#54876,#54877,#54878,#54879,#54880,#54881,#54882,#54883,
#54884,#54885,#54886,#54887,#54888,#54889,#54890,#54891,#54892,#54893,#54894,
#54895,#54896,#54897,#54898,#54899,#54900,#54901,#54902,#54903,#54904,#54905,
#54906,#54907,#54908,#54909,#54910,#54911,#54912,#54913,#54914,#54915,#54916,
#54917,#54918,#54919,#54920,#54921,#54922,#54923,#54924,#54925,#54926,#54927,
#54928,#54929,#54930,#54931,#54932,#54933,#54934,#54935,#54936,#54937,#54938,
#54939,#54940,#54941,#54942,#54943,#54944,#54945,#54946,#54947,#54948,#54949,
#54950,#54951,#54952,#54953,#54954,#54955,#54956,#54957,#54958,#54959,#54960,
#54961,#54962,#54963,#54964),.UNSPECIFIED.,.F.,.F.,(4,3,3,3,3,3,3,3,3,3,
3,3,3,3,3,3,3,3,3,3,3,3,3,3,3,3,3,3,3,3,3,3,3,3,3,3,3,3,3,3,3,3,3,4),(0.00080811238697951,
0.000808302945491443,0.000808850356008893,0.000858169371998666,0.000859403503259436,
0.00090813769617751,0.000909956650509979,0.000922594937322613,0.00093315937462551,
0.000935233224135246,0.00095824545751998,0.00096050979776051,0.00100870006033539,
0.00101106294501103,0.00105948647079065,0.00106161609226155,0.00108689266588681,
0.00111055157423082,0.00111216923951207,0.00116181788716099,0.0011627223867626,
0.00121318172198154,0.00121327553401313,0.00126382868126365,0.00126454753268235,
0.00127646696807629,0.00127737780427383,0.00128910525488892,0.00129020045697118,
0.00131438182851419,0.00131580628731212,0.00136493497576474,0.00136682939005471,
0.00141548812301528,0.00141753931363807,0.00144076469664055,0.00144275336852841,
0.00146604127026582,0.00146787510376584,0.00151659441751637,0.00151798775480161,
0.00156714756476691,0.00156793293030094,0.00161770071201745),
 .UNSPECIFIED.);
#989=B_SPLINE_CURVE_WITH_KNOTS('',3,(#54988,#54989,#54990,#54991,#54992,
#54993,#54994,#54995,#54996,#54997),.UNSPECIFIED.,.F.,.F.,(4,2,2,2,4),(-0.00550601116947268,
0.,0.0481725175638029,0.0759608671644843,0.10231697822769),
 .UNSPECIFIED.);
#990=B_SPLINE_CURVE_WITH_KNOTS('',3,(#55034,#55035,#55036,#55037,#55038,
#55039,#55040,#55041,#55042,#55043,#55044,#55045,#55046,#55047,#55048,#55049,
#55050,#55051,#55052,#55053,#55054,#55055,#55056,#55057,#55058,#55059,#55060,
#55061,#55062,#55063,#55064,#55065,#55066,#55067,#55068,#55069,#55070,#55071,
#55072,#55073,#55074,#55075,#55076,#55077,#55078,#55079,#55080,#55081,#55082,
#55083,#55084,#55085,#55086,#55087,#55088,#55089,#55090,#55091,#55092,#55093,
#55094,#55095,#55096,#55097,#55098,#55099,#55100),.UNSPECIFIED.,.F.,.F.,
(4,3,3,3,3,3,3,3,3,3,3,3,3,3,3,3,3,3,3,3,3,3,4),(-0.0010038592303248,-0.000996016580088018,
-0.000988173929851109,-0.000972488629377284,-0.000941118028429635,-0.000909747427481985,
-0.000878376826534336,-0.0007756051487124,-0.000752894422743731,-0.000656768417933472,
-0.000627412018953126,-0.000596041418005469,-0.000564670817057813,-0.0005019296151625,
-0.000413395135354653,-0.000376447211371868,-0.000313706009476555,-0.000282335408528902,
-0.00025096480758125,-0.000169956252849148,-0.000125482403790632,-6.2741201895316E-5,
0.),.UNSPECIFIED.);
#991=B_SPLINE_CURVE_WITH_KNOTS('',3,(#55108,#55109,#55110,#55111,#55112,
#55113,#55114,#55115,#55116,#55117),.UNSPECIFIED.,.F.,.F.,(4,2,2,2,4),(2.3288001587927E-6,
0.0253758099388679,0.0507136033495846,0.103872134093849,0.104445029963715),
 .UNSPECIFIED.);
#992=B_SPLINE_CURVE_WITH_KNOTS('',3,(#55244,#55245,#55246,#55247,#55248,
#55249,#55250,#55251,#55252,#55253,#55254,#55255,#55256,#55257,#55258,#55259,
#55260,#55261,#55262,#55263,#55264,#55265,#55266,#55267,#55268,#55269,#55270,
#55271,#55272,#55273,#55274,#55275,#55276,#55277,#55278,#55279,#55280,#55281,
#55282,#55283,#55284,#55285,#55286,#55287,#55288,#55289,#55290,#55291,#55292,
#55293,#55294,#55295,#55296,#55297,#55298,#55299,#55300,#55301,#55302,#55303,
#55304,#55305,#55306,#55307,#55308,#55309,#55310,#55311,#55312,#55313,#55314,
#55315,#55316,#55317,#55318,#55319,#55320,#55321,#55322,#55323,#55324,#55325,
#55326,#55327,#55328),.UNSPECIFIED.,.F.,.F.,(4,3,3,3,3,3,3,3,3,3,3,3,3,
3,3,3,3,3,3,3,3,3,3,3,3,3,3,3,4),(0.,0.000132953866864794,0.000143131415743608,
0.000214697123615411,0.000250479977551313,0.00026681859857174,0.000286262831487215,
0.00030052042883516,0.000322045685423116,0.000334541694191434,0.000357828539359018,
0.000403373858123355,0.000429394247230825,0.000543906469566681,0.00057252566297444,
0.000615590207484267,0.00064409137084625,0.000651788086821203,0.000679874224782152,
0.000688237624566197,0.000715657078718053,0.00083666270204627,0.000858788494461667,
0.000989235649453088,0.00100191991020528,0.00103770276414118,0.00106699082305431,
0.00107348561807708,0.00114505132594889),.UNSPECIFIED.);
#993=B_SPLINE_CURVE_WITH_KNOTS('',3,(#55341,#55342,#55343,#55344),
 .UNSPECIFIED.,.F.,.F.,(4,4),(0.00036767516211002,0.0122424340459221),
 .UNSPECIFIED.);
#994=B_SPLINE_CURVE_WITH_KNOTS('',3,(#55345,#55346,#55347,#55348,#55349,
#55350,#55351,#55352),.UNSPECIFIED.,.F.,.F.,(4,2,2,4),(-0.0849227079013314,
-0.0799038204840182,-0.0443510460373534,-1.00047370417821E-6),
 .UNSPECIFIED.);
#995=B_SPLINE_CURVE_WITH_KNOTS('',3,(#55633,#55634,#55635,#55636),
 .UNSPECIFIED.,.F.,.F.,(4,4),(0.,0.0113332794370003),.UNSPECIFIED.);
#996=B_SPLINE_CURVE_WITH_KNOTS('',3,(#55777,#55778,#55779,#55780,#55781,
#55782,#55783,#55784,#55785,#55786,#55787,#55788,#55789,#55790,#55791,#55792,
#55793,#55794,#55795,#55796,#55797,#55798,#55799,#55800,#55801,#55802,#55803,
#55804,#55805,#55806,#55807,#55808,#55809,#55810,#55811,#55812,#55813,#55814,
#55815,#55816,#55817,#55818,#55819,#55820,#55821,#55822,#55823,#55824,#55825,
#55826,#55827,#55828,#55829,#55830,#55831,#55832,#55833,#55834,#55835,#55836,
#55837,#55838,#55839,#55840,#55841,#55842,#55843),.UNSPECIFIED.,.F.,.F.,
(4,3,3,3,3,3,3,3,3,3,3,3,3,3,3,3,3,3,3,3,3,3,4),(0.,5.50030531657853E-5,
0.000110006106331571,0.000165009159497356,0.000178759922788797,0.000192510686080239,
0.000220012212663132,0.000275015265828909,0.000330018318994686,0.00035751984557757,
0.000385021372160454,0.000440024425326228,0.000495027478492002,0.000508778241783447,
0.000522529005074892,0.000550030531657776,0.000605033584823541,0.000660036637989305,
0.000687538164572187,0.000715039691155069,0.000770042744320831,0.000825045797486593,
0.000880048850652355),.UNSPECIFIED.);
#997=B_SPLINE_CURVE_WITH_KNOTS('',3,(#55844,#55845,#55846,#55847,#55848,
#55849,#55850,#55851,#55852,#55853,#55854,#55855,#55856,#55857,#55858,#55859,
#55860,#55861,#55862,#55863,#55864,#55865,#55866,#55867,#55868,#55869,#55870,
#55871,#55872,#55873,#55874,#55875,#55876,#55877,#55878,#55879,#55880,#55881,
#55882),.UNSPECIFIED.,.F.,.F.,(4,1,1,2,2,1,2,1,2,2,2,1,1,2,2,2,1,1,2,1,
2,2,1,1,4),(5.96075724321896E-15,0.000108435279304831,0.000216870558603701,
0.00032530583790257,0.00035241465772729,0.000379523477552009,0.000433741117201448,
0.000542176396500325,0.000650611675799202,0.000677720495623919,0.000704829315448636,
0.000759046955098071,0.000867482234396948,0.000975917513695825,0.00103013515334526,
0.00105724397316998,0.0010843527929947,0.00119278807229356,0.00130122335159243,
0.00135544099124186,0.00138254981106657,0.00140965863089129,0.00151809391019014,
0.00162652918948899,0.00173496446878785),.UNSPECIFIED.);
#998=B_SPLINE_CURVE_WITH_KNOTS('',3,(#56242,#56243,#56244,#56245),
 .UNSPECIFIED.,.F.,.F.,(4,4),(1.78796901209599,1.79013675073573),
 .UNSPECIFIED.);
#999=B_SPLINE_CURVE_WITH_KNOTS('',3,(#56352,#56353,#56354,#56355,#56356,
#56357,#56358,#56359,#56360,#56361,#56362,#56363,#56364,#56365,#56366,#56367,
#56368,#56369,#56370,#56371,#56372,#56373,#56374,#56375,#56376,#56377,#56378,
#56379,#56380,#56381,#56382,#56383,#56384,#56385,#56386,#56387,#56388,#56389,
#56390,#56391,#56392,#56393,#56394),.UNSPECIFIED.,.F.,.F.,(4,3,3,3,3,3,
3,3,3,3,3,3,3,3,4),(-0.00218249118872392,-0.00216544047631201,-0.00214838976390011,
-0.0021142883390763,-0.00204608548942867,-0.00190967979013342,-0.00163686839154293,
-0.00136405699295245,-0.00109124559436196,-0.000818434195771467,-0.000545622797180978,
-0.000409217097885734,-0.000272811398590489,-0.000136405699295245,0.),
 .UNSPECIFIED.);
#1000=B_SPLINE_CURVE_WITH_KNOTS('',3,(#56398,#56399,#56400,#56401,#56402,
#56403),.UNSPECIFIED.,.F.,.F.,(4,2,4),(-0.0212734387247141,-0.0106371499207884,
-1.22408019587832E-6),.UNSPECIFIED.);
#1001=B_SPLINE_CURVE_WITH_KNOTS('',3,(#56406,#56407,#56408,#56409,#56410,
#56411,#56412,#56413,#56414,#56415,#56416,#56417,#56418,#56419,#56420,#56421,
#56422,#56423,#56424,#56425,#56426,#56427,#56428,#56429,#56430,#56431,#56432,
#56433),.UNSPECIFIED.,.F.,.F.,(4,3,3,3,3,3,3,3,3,4),(-0.00112201278880437,
-0.00110806877345402,-0.00109412475810366,-0.00106623672740295,-0.00101046066600152,
-0.000924145508874287,-0.000898908543198666,-0.00084313248179724,-0.000787356420395815,
-0.000675804297592954),.UNSPECIFIED.);
#1002=B_SPLINE_CURVE_WITH_KNOTS('',3,(#56434,#56435,#56436,#56437,#56438,
#56439,#56440,#56441),.UNSPECIFIED.,.F.,.F.,(4,2,2,4),(-0.0127135782228372,
0.,0.0940564686398219,0.200639665029003),.UNSPECIFIED.);
#1003=B_SPLINE_CURVE_WITH_KNOTS('',3,(#56473,#56474,#56475,#56476,#56477,
#56478,#56479,#56480,#56481,#56482,#56483,#56484,#56485,#56486,#56487,#56488,
#56489,#56490,#56491,#56492,#56493,#56494,#56495,#56496,#56497,#56498,#56499,
#56500,#56501,#56502,#56503,#56504,#56505,#56506,#56507,#56508,#56509,#56510,
#56511,#56512,#56513,#56514,#56515),.UNSPECIFIED.,.F.,.F.,(4,3,3,3,3,3,
3,3,3,3,3,3,3,3,4),(0.,0.00013646494075281,0.000272940213284047,0.000409423605142272,
0.000545889876308567,0.000818834814462857,0.00109177975261715,0.00136472469077144,
0.00163777665242055,0.00191061456708002,0.00204708703615716,0.00211531911473619,
0.00214944040496523,0.00216650044659966,0.0021835595052343),
 .UNSPECIFIED.);
#1004=B_SPLINE_CURVE_WITH_KNOTS('',3,(#56516,#56517,#56518,#56519,#56520,
#56521,#56522,#56523,#56524,#56525,#56526,#56527,#56528,#56529,#56530,#56531,
#56532,#56533,#56534,#56535,#56536,#56537,#56538,#56539,#56540,#56541,#56542,
#56543,#56544,#56545,#56546,#56547,#56548,#56549,#56550,#56551,#56552,#56553,
#56554,#56555,#56556,#56557,#56558),.UNSPECIFIED.,.F.,.F.,(4,3,3,3,3,3,
3,3,3,3,3,3,3,3,4),(-0.00218249118872365,-0.00216544047631174,-0.00214838976389984,
-0.00211428833907603,-0.00204608548942841,-0.00190967979013318,-0.00163686839154273,
-0.00136405699295227,-0.00109124559436182,-0.000818434195771367,-0.000545622797180915,
-0.000409217097885686,-0.000272811398590457,-0.000136405699295229,0.),
 .UNSPECIFIED.);
#1005=B_SPLINE_CURVE_WITH_KNOTS('',3,(#56559,#56560,#56561,#56562,#56563,
#56564,#56565,#56566,#56567,#56568,#56569,#56570,#56571,#56572,#56573,#56574,
#56575,#56576,#56577,#56578,#56579,#56580,#56581,#56582,#56583,#56584,#56585,
#56586,#56587,#56588,#56589,#56590,#56591,#56592,#56593,#56594,#56595,#56596,
#56597,#56598,#56599,#56600,#56601),.UNSPECIFIED.,.F.,.F.,(4,3,3,3,3,3,
3,3,3,3,3,3,3,3,4),(0.,0.000136464940752808,0.000272940213284044,0.000409423605142217,
0.000545889876308567,0.000818834814462855,0.00109177975261714,0.00136472469077143,
0.00163766962892572,0.00191061456708001,0.00204708703615715,0.00211531911473613,
0.00214944040496524,0.00216650044659965,0.0021835595052343),
 .UNSPECIFIED.);
#1006=B_SPLINE_CURVE_WITH_KNOTS('',3,(#56686,#56687,#56688,#56689,#56690,
#56691,#56692,#56693,#56694,#56695,#56696,#56697,#56698,#56699,#56700,#56701,
#56702,#56703,#56704,#56705,#56706,#56707,#56708,#56709,#56710,#56711,#56712,
#56713,#56714,#56715,#56716,#56717,#56718,#56719,#56720,#56721,#56722,#56723,
#56724,#56725,#56726,#56727,#56728,#56729,#56730,#56731,#56732,#56733,#56734,
#56735,#56736,#56737,#56738,#56739,#56740,#56741,#56742,#56743,#56744,#56745,
#56746,#56747,#56748,#56749,#56750,#56751,#56752,#56753,#56754,#56755,#56756,
#56757,#56758,#56759,#56760,#56761,#56762,#56763,#56764,#56765,#56766,#56767,
#56768,#56769,#56770,#56771,#56772,#56773,#56774,#56775,#56776,#56777,#56778,
#56779,#56780,#56781,#56782,#56783,#56784,#56785,#56786,#56787,#56788,#56789,
#56790,#56791),.UNSPECIFIED.,.F.,.F.,(4,3,3,3,3,3,3,3,3,3,3,3,3,3,3,3,3,
3,3,3,3,3,3,3,3,3,3,3,3,3,3,3,3,3,3,4),(0.0305709307873591,0.0306063950419888,
0.0306418592966185,0.030702367809577,0.0307127878058778,0.030837037483686,
0.0308546448243965,0.0309745186599938,0.0311143035117341,0.031138358861434,
0.0313504163721782,0.0313990237158671,0.0314220728984714,0.0316394604894248,
0.0316879165996668,0.0317057869355089,0.0319209128176095,0.0319775164650602,
0.0319895009725463,0.0320604294818057,0.032131357991065,0.0322664035810513,
0.0322732150095838,0.0324971762357433,0.0325549976396124,0.0325569290466212,
0.0326983162209018,0.03269878606514,0.0327695930842393,0.0327697145743993,
0.0328051206407265,0.032805178829029,0.0328229109563438,0.0328317770200012,
0.0328362100518299,0.0328406430836587),.UNSPECIFIED.);
#1007=B_SPLINE_CURVE_WITH_KNOTS('',3,(#56876,#56877,#56878,#56879,#56880,
#56881,#56882,#56883,#56884,#56885,#56886,#56887,#56888,#56889,#56890,#56891,
#56892,#56893,#56894,#56895,#56896,#56897,#56898,#56899,#56900,#56901,#56902,
#56903,#56904,#56905,#56906,#56907,#56908,#56909,#56910,#56911,#56912,#56913,
#56914,#56915,#56916,#56917,#56918,#56919,#56920,#56921,#56922,#56923,#56924,
#56925,#56926,#56927,#56928,#56929,#56930,#56931,#56932,#56933,#56934,#56935,
#56936,#56937,#56938,#56939,#56940,#56941,#56942,#56943,#56944,#56945,#56946,
#56947,#56948,#56949,#56950,#56951,#56952,#56953,#56954,#56955,#56956,#56957,
#56958,#56959,#56960),.UNSPECIFIED.,.F.,.F.,(4,3,3,3,3,3,3,3,3,3,3,3,3,
3,3,3,3,3,3,3,3,3,3,3,3,3,3,3,4),(3.95831162944544E-12,1.39313221873946E-7,
3.5460060852014E-5,7.10560249004281E-5,0.000142556163497197,0.000285313478397842,
0.000286667929283137,0.000508969327502391,0.000570626956795684,0.000578229350350691,
0.000800126092930885,0.000855940435193526,0.000871807784634421,0.00108923219617937,
0.00114125391359137,0.00116414093555289,0.00137785778304641,0.00142656739198921,
0.00145179194908681,0.00146223157678894,0.00149789576158867,0.00156922413118814,
0.00171188087038706,0.00173474788861616,0.00187461379195925,0.00199719434878491,
0.00201280376719234,0.00214889827835083,0.00228250782718277),
 .UNSPECIFIED.);
#1008=B_SPLINE_CURVE_WITH_KNOTS('',3,(#57050,#57051,#57052,#57053,#57054,
#57055,#57056,#57057,#57058,#57059,#57060,#57061,#57062,#57063,#57064,#57065,
#57066,#57067,#57068,#57069,#57070,#57071,#57072,#57073,#57074,#57075,#57076,
#57077,#57078,#57079,#57080,#57081,#57082,#57083,#57084,#57085,#57086,#57087,
#57088,#57089,#57090,#57091,#57092,#57093,#57094,#57095,#57096,#57097,#57098,
#57099,#57100,#57101,#57102,#57103,#57104,#57105,#57106,#57107,#57108,#57109,
#57110,#57111,#57112,#57113,#57114,#57115,#57116,#57117,#57118,#57119,#57120,
#57121,#57122,#57123,#57124,#57125,#57126,#57127,#57128,#57129,#57130,#57131,
#57132,#57133,#57134,#57135,#57136,#57137,#57138,#57139,#57140,#57141,#57142,
#57143,#57144,#57145,#57146,#57147,#57148,#57149,#57150,#57151,#57152,#57153,
#57154,#57155,#57156,#57157,#57158,#57159,#57160,#57161,#57162,#57163,#57164,
#57165,#57166,#57167,#57168,#57169,#57170,#57171,#57172,#57173,#57174,#57175,
#57176,#57177,#57178,#57179,#57180,#57181,#57182,#57183,#57184,#57185,#57186,
#57187,#57188,#57189,#57190,#57191,#57192,#57193,#57194,#57195,#57196,#57197,
#57198,#57199,#57200,#57201,#57202,#57203,#57204,#57205,#57206,#57207,#57208,
#57209,#57210,#57211,#57212,#57213,#57214,#57215,#57216,#57217,#57218,#57219,
#57220,#57221,#57222,#57223,#57224,#57225,#57226,#57227,#57228,#57229,#57230,
#57231,#57232,#57233,#57234,#57235,#57236,#57237,#57238,#57239,#57240,#57241,
#57242,#57243,#57244,#57245,#57246,#57247,#57248,#57249,#57250,#57251,#57252,
#57253,#57254,#57255,#57256,#57257,#57258,#57259,#57260,#57261,#57262,#57263,
#57264,#57265,#57266,#57267,#57268,#57269,#57270,#57271),.UNSPECIFIED.,
 .F.,.F.,(4,2,2,1,2,1,2,2,2,2,2,2,2,2,2,1,1,2,2,2,2,2,1,2,2,2,1,2,2,1,2,
1,2,2,2,1,2,2,2,2,2,2,2,2,2,1,1,2,2,2,1,2,2,2,2,2,2,2,1,2,2,2,2,2,2,2,2,
2,2,2,2,2,1,2,2,2,2,1,1,2,2,2,2,2,2,1,2,2,2,1,1,2,2,1,2,2,2,1,1,2,2,2,2,
1,2,2,2,2,2,2,1,1,2,2,2,2,2,2,2,2,1,2,2,4),(0.,0.000124188080077072,0.000186282120115608,
0.000248376160154143,0.000496752320308307,0.000993504640616636,0.00149025696092496,
0.00173863312107913,0.00180072716111768,0.00186282120115623,0.00198700928123333,
0.00248376160154172,0.0029805139218501,0.00347726624215848,0.00353936028219703,
0.00360145432223558,0.00372564240231269,0.0039740185624669,0.00447077088277532,
0.00496752320308375,0.00509171128316085,0.00515380532319941,0.00521589936323796,
0.00546427552339219,0.00596102784370064,0.00645778016400908,0.0067061563241633,
0.00683034440424042,0.00689243844427897,0.00695453248431752,0.00745128480462597,
0.00794803712493441,0.00844478944524286,0.00856897752531997,0.00869316560539708,
0.0089415417655513,0.00918991792570552,0.00925201196574408,0.00931410600578263,
0.00943829408585974,0.00993504640616816,0.0104317987264766,0.010928551046785,
0.0111769272069392,0.0112390212469778,0.0113011152870163,0.0114253033670935,
0.0119220556874019,0.0124188080077103,0.0126671841678646,0.0127913722479417,
0.0128534662879802,0.0129155603280188,0.0134123126483272,0.0139090649686356,
0.0141574411287899,0.014281629208867,0.0143437232489055,0.0144058172889441,
0.0149025696092525,0.015399321929561,0.0156476980897152,0.0157097921297537,
0.0157718861697923,0.0158960742498694,0.0163928265701779,0.0168895788904864,
0.0171379550506406,0.0172621431307177,0.0173242371707563,0.0173863312107948,
0.017510519290872,0.0176347073709491,0.0178830835311034,0.0183798358514119,
0.0188765881717205,0.0190007762517976,0.0190628702918362,0.0191249643318747,
0.019373340492029,0.0198700928123375,0.0203668451326459,0.0208635974529544,
0.0209877855330315,0.0210498795730701,0.0211119736131087,0.0213603497732629,
0.0218571020935714,0.0223538544138799,0.0226022305740341,0.0227264186541112,
0.0227885126941498,0.0228506067341884,0.0233473590544968,0.0238441113748053,
0.0243408636951138,0.0244650517751909,0.0245271458152295,0.0245892398552681,
0.0248376160154223,0.0253343683357308,0.0258311206560393,0.0260794968161935,
0.0261415908562321,0.0262036848962706,0.0263278729763477,0.0268246252966562,
0.0273213776169647,0.0278181299372732,0.0278802239773118,0.0279423180173503,
0.0280665060974275,0.0283148822575817,0.0288116345778902,0.0293083868981987,
0.029556763058353,0.0298051392185072,0.0303018915388157,0.0307986438591242,
0.0310470200192785,0.0311712080993556,0.0312333021393942,0.0312953961794328,
0.0317921484997413),.UNSPECIFIED.);
#1009=B_SPLINE_CURVE_WITH_KNOTS('',3,(#57274,#57275,#57276,#57277,#57278,
#57279,#57280,#57281,#57282,#57283,#57284,#57285,#57286,#57287,#57288,#57289,
#57290,#57291,#57292,#57293,#57294,#57295,#57296,#57297,#57298,#57299,#57300,
#57301,#57302,#57303,#57304,#57305,#57306,#57307,#57308,#57309,#57310,#57311,
#57312,#57313,#57314,#57315,#57316,#57317,#57318,#57319,#57320,#57321,#57322,
#57323,#57324,#57325,#57326,#57327,#57328,#57329,#57330,#57331,#57332,#57333,
#57334,#57335,#57336,#57337,#57338,#57339,#57340),.UNSPECIFIED.,.F.,.F.,
(4,3,3,3,3,3,3,3,3,3,3,3,3,3,3,3,3,3,3,3,3,3,4),(1.01984272302816E-10,7.14212642807727E-5,
0.00011606672308277,0.000198180758390202,0.00023213344616554,0.000261150126936228,
0.000290166807706916,0.000348200169248292,0.000436238575559047,0.000464266892331045,
0.000560937956114547,0.000580333615413797,0.000609350296184482,0.000638366976955167,
0.000696400338496545,0.000797480418061141,0.000812467061579307,0.000870500423120685,
0.000899517103891371,0.000914025444276714,0.000921279614469381,0.000924906699565713,
0.000928533784662045),.UNSPECIFIED.);
#1010=B_SPLINE_CURVE_WITH_KNOTS('',3,(#58842,#58843,#58844,#58845,#58846,
#58847,#58848,#58849),.UNSPECIFIED.,.F.,.F.,(4,2,2,4),(1.99674797794768E-6,
0.115795506675109,0.23027663807213,0.231396261216017),.UNSPECIFIED.);
#1011=B_SPLINE_CURVE_WITH_KNOTS('',3,(#58966,#58967,#58968,#58969,#58970,
#58971,#58972,#58973,#58974,#58975,#58976,#58977,#58978,#58979,#58980,#58981,
#58982,#58983,#58984,#58985,#58986,#58987,#58988,#58989,#58990,#58991),
 .UNSPECIFIED.,.F.,.F.,(4,1,2,1,1,2,2,2,2,2,1,1,1,1,1,2,4),(1.83170469685919E-10,
8.90982346471883E-5,0.000178196469294377,0.000222745586617969,0.000245020145279767,
0.000267294703941566,0.000356392938588793,0.000445491173236021,0.000534589407883249,
0.000556863966545041,0.000579138525206834,0.000623687642530402,0.000668236759853971,
0.000690511318515748,0.000701648597846644,0.000707217237512084,0.000712785877177525),
 .UNSPECIFIED.);
#1012=B_SPLINE_CURVE_WITH_KNOTS('',3,(#59043,#59044,#59045,#59046,#59047,
#59048),.UNSPECIFIED.,.F.,.F.,(4,2,4),(0.163612590061207,0.211914877806934,
0.237815857774527),.UNSPECIFIED.);
#1013=B_SPLINE_CURVE_WITH_KNOTS('',3,(#59204,#59205,#59206,#59207,#59208,
#59209,#59210,#59211,#59212,#59213,#59214,#59215,#59216,#59217,#59218,#59219,
#59220,#59221,#59222,#59223,#59224,#59225,#59226,#59227,#59228,#59229,#59230,
#59231,#59232,#59233,#59234,#59235,#59236,#59237,#59238,#59239,#59240,#59241,
#59242,#59243,#59244,#59245,#59246,#59247,#59248,#59249,#59250,#59251,#59252,
#59253,#59254,#59255,#59256,#59257,#59258,#59259,#59260,#59261,#59262,#59263,
#59264,#59265,#59266,#59267,#59268,#59269,#59270,#59271,#59272,#59273,#59274,
#59275,#59276,#59277,#59278,#59279,#59280,#59281,#59282),.UNSPECIFIED.,
 .F.,.F.,(4,3,3,3,3,3,3,3,3,3,3,3,3,3,3,3,3,3,3,3,3,3,3,3,3,3,4),(-0.00129891904736022,
-0.00129130819356754,-0.00128877124230316,-0.00127862343724565,-0.00125832782713064,
-0.00121773660690063,-0.00113655416644058,-0.00105537172598053,-0.00101478050575051,
-0.000994484895635494,-0.00097418928552048,-0.000893006845060438,-0.000811824404600395,
-0.000730641964140352,-0.000690050743910334,-0.000669755133795326,-0.000649459523680318,
-0.000568277083220278,-0.000487094642760238,-0.000405912202300198,-0.00036532098207018,
-0.000345025371955169,-0.000324729761840158,-0.000243547321380123,-0.000162364880920088,
-8.11824404600523E-5,-1.7130394325271E-17),.UNSPECIFIED.);
#1014=B_SPLINE_CURVE_WITH_KNOTS('',3,(#59283,#59284,#59285,#59286,#59287,
#59288,#59289,#59290),.UNSPECIFIED.,.F.,.F.,(4,2,2,4),(-0.00857562118451602,
4.87793563352587E-7,0.0211728314512976,0.051545416127519),.UNSPECIFIED.);
#1015=B_SPLINE_CURVE_WITH_KNOTS('',3,(#59291,#59292,#59293,#59294,#59295,
#59296,#59297,#59298),.UNSPECIFIED.,.F.,.F.,(4,2,2,4),(-0.147545167441897,
-0.135199000031876,-0.073467772649398,-1.78767173606405E-6),
 .UNSPECIFIED.);
#1016=B_SPLINE_CURVE_WITH_KNOTS('',3,(#59587,#59588,#59589,#59590,#59591,
#59592,#59593,#59594,#59595,#59596,#59597,#59598,#59599,#59600,#59601,#59602,
#59603,#59604,#59605,#59606,#59607,#59608,#59609,#59610,#59611,#59612,#59613,
#59614,#59615,#59616,#59617,#59618,#59619,#59620,#59621,#59622,#59623,#59624,
#59625,#59626,#59627,#59628,#59629),.UNSPECIFIED.,.F.,.F.,(4,3,3,3,3,3,
3,3,3,3,3,3,3,3,4),(0.,9.86527119726346E-5,0.000147453735011662,0.000250428443831339,
0.000294907470023324,0.000331770903776236,0.000368634337529148,0.000442361205034974,
0.0005160880725408,0.00055295150629371,0.000571383223170166,0.000575991152389278,
0.000578295116998834,0.000580599081608391,0.00058981494004661),
 .UNSPECIFIED.);
#1017=B_SPLINE_CURVE_WITH_KNOTS('',3,(#59630,#59631,#59632,#59633,#59634,
#59635,#59636,#59637,#59638,#59639,#59640,#59641,#59642,#59643,#59644,#59645,
#59646,#59647,#59648,#59649,#59650,#59651,#59652,#59653,#59654,#59655,#59656,
#59657,#59658,#59659,#59660),.UNSPECIFIED.,.F.,.F.,(4,3,3,3,3,3,3,3,3,3,
4),(0.,0.000277651260623857,0.000292700609901568,0.000476971360228736,0.000555302521247713,
0.000570297395023951,0.000664174349502761,0.00083295378187157,0.000971779412183499,
0.00104408940251943,0.00111060504249543),.UNSPECIFIED.);
#1018=B_SPLINE_CURVE_WITH_KNOTS('',3,(#59665,#59666,#59667,#59668,#59669,
#59670,#59671,#59672),.UNSPECIFIED.,.F.,.F.,(4,2,2,4),(-0.000622277040978629,
0.,0.0768376409886872,0.127182502679576),.UNSPECIFIED.);
#1019=B_SPLINE_CURVE_WITH_KNOTS('',3,(#59676,#59677,#59678,#59679,#59680,
#59681,#59682,#59683,#59684,#59685,#59686,#59687,#59688,#59689,#59690,#59691,
#59692,#59693,#59694,#59695,#59696,#59697,#59698,#59699,#59700,#59701,#59702,
#59703,#59704,#59705,#59706,#59707,#59708,#59709,#59710,#59711,#59712,#59713,
#59714,#59715,#59716,#59717,#59718,#59719,#59720,#59721,#59722,#59723,#59724,
#59725,#59726,#59727,#59728,#59729,#59730,#59731,#59732,#59733,#59734,#59735,
#59736,#59737,#59738,#59739,#59740,#59741,#59742,#59743,#59744,#59745,#59746,
#59747,#59748,#59749,#59750,#59751,#59752,#59753,#59754,#59755,#59756,#59757,
#59758,#59759,#59760,#59761,#59762,#59763,#59764,#59765,#59766,#59767,#59768,
#59769),.UNSPECIFIED.,.F.,.F.,(4,3,3,3,3,3,3,3,3,3,3,3,3,3,3,3,3,3,3,3,
3,3,3,3,3,3,3,3,3,3,3,4),(0.,5.04083481357633E-5,6.06628904997995E-5,0.00010114819054449,
0.000121325780999599,0.000151657226249498,0.000165282521792658,0.000178369354151246,
0.000204828211607868,0.000242651561999202,0.000258887470162885,0.000303314452499011,
0.000314495273876791,0.000328648098408335,0.0003429052739943,0.000363977342998827,
0.000424640233498611,0.000485303123998396,0.000515634569248287,0.000530800291873228,
0.00054596601449817,0.000606628904997954,0.000620350766208646,0.000687203566160806,
0.000727954685997538,0.000755915169194966,0.00077338354336116,0.000788617576497332,
0.000826258928547019,0.000849280466997126,0.00089781676624165,0.000970606247996704),
 .UNSPECIFIED.);
#1020=B_SPLINE_CURVE_WITH_KNOTS('',3,(#60714,#60715,#60716,#60717,#60718,
#60719,#60720,#60721,#60722,#60723,#60724,#60725),.UNSPECIFIED.,.F.,.F.,
(4,2,2,2,2,4),(-0.29661354335631,-0.278391574572434,-0.254432654164122,
-0.234687270338995,-0.214941886513867,-0.210821993248899),.UNSPECIFIED.);
#1021=B_SPLINE_CURVE_WITH_KNOTS('',3,(#61884,#61885,#61886,#61887,#61888,
#61889,#61890,#61891,#61892,#61893,#61894,#61895,#61896,#61897,#61898,#61899,
#61900,#61901,#61902,#61903,#61904,#61905,#61906,#61907,#61908),
 .UNSPECIFIED.,.F.,.F.,(4,3,3,3,3,3,3,3,4),(1.2869157614395E-10,0.00023065303768028,
0.000313885266238508,0.000470827899357743,0.000549299215917362,0.000588534874197172,
0.000608152703337074,0.000617961617907029,0.000627770532476985),
 .UNSPECIFIED.);
#1022=B_SPLINE_CURVE_WITH_KNOTS('',3,(#62605,#62606,#62607,#62608,#62609,
#62610,#62611,#62612,#62613,#62614),.UNSPECIFIED.,.F.,.F.,(4,2,2,2,4),(0.000465302741751488,
0.0107996201392302,0.0220542164513607,0.0339643336336735,0.0466183650451173),
 .UNSPECIFIED.);
#1023=B_SPLINE_CURVE_WITH_KNOTS('',3,(#62616,#62617,#62618,#62619,#62620,
#62621,#62622,#62623,#62624,#62625),.UNSPECIFIED.,.F.,.F.,(4,2,2,2,4),(0.141205929776987,
0.153859961188429,0.16577007837074,0.177024674682869,0.187358992080346),
 .UNSPECIFIED.);
#1045=CONICAL_SURFACE('',#16498,3.,0.0156237286204751);
#1046=CONICAL_SURFACE('',#16504,19.5,0.358770670270572);
#1047=CONICAL_SURFACE('',#16635,17.4363291775691,0.358770670270571);
#2044=LINE('',#45597,#3237);
#2045=LINE('',#46086,#3238);
#2046=LINE('',#46368,#3239);
#2047=LINE('',#47036,#3240);
#2048=LINE('',#48369,#3241);
#2049=LINE('',#48909,#3242);
#2050=LINE('',#49043,#3243);
#2051=LINE('',#50240,#3244);
#2052=LINE('',#50244,#3245);
#2053=LINE('',#51646,#3246);
#2054=LINE('',#52119,#3247);
#2055=LINE('',#52122,#3248);
#2056=LINE('',#52141,#3249);
#2057=LINE('',#53447,#3250);
#2058=LINE('',#53473,#3251);
#2059=LINE('',#53486,#3252);
#2060=LINE('',#53489,#3253);
#2061=LINE('',#53491,#3254);
#2062=LINE('',#53708,#3255);
#2063=LINE('',#53712,#3256);
#2064=LINE('',#54041,#3257);
#2065=LINE('',#54507,#3258);
#2066=LINE('',#54513,#3259);
#2067=LINE('',#54519,#3260);
#2068=LINE('',#54533,#3261);
#2069=LINE('',#54536,#3262);
#2070=LINE('',#54541,#3263);
#2071=LINE('',#54544,#3264);
#2072=LINE('',#54553,#3265);
#2073=LINE('',#54554,#3266);
#2074=LINE('',#54563,#3267);
#2075=LINE('',#54689,#3268);
#2076=LINE('',#54692,#3269);
#2077=LINE('',#54696,#3270);
#2078=LINE('',#54965,#3271);
#2079=LINE('',#54969,#3272);
#2080=LINE('',#54972,#3273);
#2081=LINE('',#54976,#3274);
#2082=LINE('',#54979,#3275);
#2083=LINE('',#54984,#3276);
#2084=LINE('',#54999,#3277);
#2085=LINE('',#55005,#3278);
#2086=LINE('',#55013,#3279);
#2087=LINE('',#55021,#3280);
#2088=LINE('',#55027,#3281);
#2089=LINE('',#55102,#3282);
#2090=LINE('',#55107,#3283);
#2091=LINE('',#55122,#3284);
#2092=LINE('',#55123,#3285);
#2093=LINE('',#55124,#3286);
#2094=LINE('',#55128,#3287);
#2095=LINE('',#55135,#3288);
#2096=LINE('',#55137,#3289);
#2097=LINE('',#55140,#3290);
#2098=LINE('',#55143,#3291);
#2099=LINE('',#55144,#3292);
#2100=LINE('',#55147,#3293);
#2101=LINE('',#55151,#3294);
#2102=LINE('',#55152,#3295);
#2103=LINE('',#55155,#3296);
#2104=LINE('',#55158,#3297);
#2105=LINE('',#56070,#3298);
#2106=LINE('',#56071,#3299);
#2107=LINE('',#56076,#3300);
#2108=LINE('',#56077,#3301);
#2109=LINE('',#56089,#3302);
#2110=LINE('',#56090,#3303);
#2111=LINE('',#56095,#3304);
#2112=LINE('',#56096,#3305);
#2113=LINE('',#56105,#3306);
#2114=LINE('',#56106,#3307);
#2115=LINE('',#56111,#3308);
#2116=LINE('',#56112,#3309);
#2117=LINE('',#56121,#3310);
#2118=LINE('',#56122,#3311);
#2119=LINE('',#56125,#3312);
#2120=LINE('',#56128,#3313);
#2121=LINE('',#56137,#3314);
#2122=LINE('',#56138,#3315);
#2123=LINE('',#56143,#3316);
#2124=LINE('',#56145,#3317);
#2125=LINE('',#56151,#3318);
#2126=LINE('',#56152,#3319);
#2127=LINE('',#56155,#3320);
#2128=LINE('',#56158,#3321);
#2129=LINE('',#56162,#3322);
#2130=LINE('',#56163,#3323);
#2131=LINE('',#56167,#3324);
#2132=LINE('',#56168,#3325);
#2133=LINE('',#56171,#3326);
#2134=LINE('',#56174,#3327);
#2135=LINE('',#56178,#3328);
#2136=LINE('',#56181,#3329);
#2137=LINE('',#56189,#3330);
#2138=LINE('',#56190,#3331);
#2139=LINE('',#56192,#3332);
#2140=LINE('',#56193,#3333);
#2141=LINE('',#56195,#3334);
#2142=LINE('',#56196,#3335);
#2143=LINE('',#56199,#3336);
#2144=LINE('',#56202,#3337);
#2145=LINE('',#56204,#3338);
#2146=LINE('',#56207,#3339);
#2147=LINE('',#56208,#3340);
#2148=LINE('',#56210,#3341);
#2149=LINE('',#56212,#3342);
#2150=LINE('',#56217,#3343);
#2151=LINE('',#56218,#3344);
#2152=LINE('',#56219,#3345);
#2153=LINE('',#56223,#3346);
#2154=LINE('',#56227,#3347);
#2155=LINE('',#56230,#3348);
#2156=LINE('',#56231,#3349);
#2157=LINE('',#56238,#3350);
#2158=LINE('',#56239,#3351);
#2159=LINE('',#56249,#3352);
#2160=LINE('',#56251,#3353);
#2161=LINE('',#56252,#3354);
#2162=LINE('',#56254,#3355);
#2163=LINE('',#56256,#3356);
#2164=LINE('',#56404,#3357);
#2165=LINE('',#56452,#3358);
#2166=LINE('',#56454,#3359);
#2167=LINE('',#56456,#3360);
#2168=LINE('',#56459,#3361);
#2169=LINE('',#56460,#3362);
#2170=LINE('',#56464,#3363);
#2171=LINE('',#56467,#3364);
#2172=LINE('',#56469,#3365);
#2173=LINE('',#56470,#3366);
#2174=LINE('',#57048,#3367);
#2175=LINE('',#57272,#3368);
#2176=LINE('',#58852,#3369);
#2177=LINE('',#58853,#3370);
#2178=LINE('',#58857,#3371);
#2179=LINE('',#58862,#3372);
#2180=LINE('',#58994,#3373);
#2181=LINE('',#58996,#3374);
#2182=LINE('',#58997,#3375);
#2183=LINE('',#59000,#3376);
#2184=LINE('',#59001,#3377);
#2185=LINE('',#59002,#3378);
#2186=LINE('',#59006,#3379);
#2187=LINE('',#59007,#3380);
#2188=LINE('',#59009,#3381);
#2189=LINE('',#59013,#3382);
#2190=LINE('',#59019,#3383);
#2191=LINE('',#59020,#3384);
#2192=LINE('',#59022,#3385);
#2193=LINE('',#59026,#3386);
#2194=LINE('',#59031,#3387);
#2195=LINE('',#59034,#3388);
#2196=LINE('',#59037,#3389);
#2197=LINE('',#59039,#3390);
#2198=LINE('',#59040,#3391);
#2199=LINE('',#59050,#3392);
#2200=LINE('',#59051,#3393);
#2201=LINE('',#60713,#3394);
#2202=LINE('',#62630,#3395);
#2203=LINE('',#62634,#3396);
#2204=LINE('',#62637,#3397);
#3237=VECTOR('',#20263,19.5);
#3238=VECTOR('',#20268,3.);
#3239=VECTOR('',#20283,19.5);
#3240=VECTOR('',#20302,16.5);
#3241=VECTOR('',#20309,1000.);
#3242=VECTOR('',#20322,1000.);
#3243=VECTOR('',#20325,1000.);
#3244=VECTOR('',#20338,1000.);
#3245=VECTOR('',#20341,1000.);
#3246=VECTOR('',#20374,8.);
#3247=VECTOR('',#20379,1000.);
#3248=VECTOR('',#20382,1000.);
#3249=VECTOR('',#20395,14.5);
#3250=VECTOR('',#20418,1000.);
#3251=VECTOR('',#20421,1000.);
#3252=VECTOR('',#20424,1000.);
#3253=VECTOR('',#20427,1000.);
#3254=VECTOR('',#20430,19.5);
#3255=VECTOR('',#20437,1000.);
#3256=VECTOR('',#20440,1000.);
#3257=VECTOR('',#20451,5.);
#3258=VECTOR('',#20462,2.);
#3259=VECTOR('',#20469,2.2295);
#3260=VECTOR('',#20476,17.5);
#3261=VECTOR('',#20491,1000.);
#3262=VECTOR('',#20494,1000.);
#3263=VECTOR('',#20499,1000.);
#3264=VECTOR('',#20502,1000.);
#3265=VECTOR('',#20513,1000.);
#3266=VECTOR('',#20514,1000.);
#3267=VECTOR('',#20525,3.3235);
#3268=VECTOR('',#20530,1000.);
#3269=VECTOR('',#20533,1000.);
#3270=VECTOR('',#20538,1000.);
#3271=VECTOR('',#20539,1000.);
#3272=VECTOR('',#20544,4.);
#3273=VECTOR('',#20547,4.);
#3274=VECTOR('',#20552,1000.);
#3275=VECTOR('',#20555,1000.);
#3276=VECTOR('',#20560,2.5);
#3277=VECTOR('',#20565,1000.);
#3278=VECTOR('',#20572,2.067);
#3279=VECTOR('',#20583,17.4363291775691);
#3280=VECTOR('',#20594,2.5);
#3281=VECTOR('',#20601,2.);
#3282=VECTOR('',#20612,1000.);
#3283=VECTOR('',#20617,1000.);
#3284=VECTOR('',#20622,1000.);
#3285=VECTOR('',#20623,1000.);
#3286=VECTOR('',#20624,1000.);
#3287=VECTOR('',#20627,1000.);
#3288=VECTOR('',#20636,1000.);
#3289=VECTOR('',#20637,1000.);
#3290=VECTOR('',#20640,1000.);
#3291=VECTOR('',#20643,1000.);
#3292=VECTOR('',#20644,1000.);
#3293=VECTOR('',#20647,1000.);
#3294=VECTOR('',#20652,1000.);
#3295=VECTOR('',#20653,1000.);
#3296=VECTOR('',#20656,1000.);
#3297=VECTOR('',#20661,1000.);
#3298=VECTOR('',#20700,1000.);
#3299=VECTOR('',#20701,1000.);
#3300=VECTOR('',#20706,1000.);
#3301=VECTOR('',#20707,1000.);
#3302=VECTOR('',#20720,1000.);
#3303=VECTOR('',#20721,1000.);
#3304=VECTOR('',#20726,1000.);
#3305=VECTOR('',#20727,1000.);
#3306=VECTOR('',#20738,1000.);
#3307=VECTOR('',#20739,1000.);
#3308=VECTOR('',#20744,1000.);
#3309=VECTOR('',#20745,1000.);
#3310=VECTOR('',#20756,1000.);
#3311=VECTOR('',#20757,1000.);
#3312=VECTOR('',#20760,1000.);
#3313=VECTOR('',#20763,1000.);
#3314=VECTOR('',#20774,1000.);
#3315=VECTOR('',#20775,1000.);
#3316=VECTOR('',#20780,1000.);
#3317=VECTOR('',#20783,1000.);
#3318=VECTOR('',#20792,1000.);
#3319=VECTOR('',#20793,1000.);
#3320=VECTOR('',#20796,1000.);
#3321=VECTOR('',#20799,1000.);
#3322=VECTOR('',#20804,1000.);
#3323=VECTOR('',#20805,1000.);
#3324=VECTOR('',#20812,1000.);
#3325=VECTOR('',#20813,1000.);
#3326=VECTOR('',#20816,1000.);
#3327=VECTOR('',#20819,1000.);
#3328=VECTOR('',#20824,1000.);
#3329=VECTOR('',#20827,1000.);
#3330=VECTOR('',#20838,1000.);
#3331=VECTOR('',#20839,1000.);
#3332=VECTOR('',#20842,1000.);
#3333=VECTOR('',#20843,1000.);
#3334=VECTOR('',#20846,1000.);
#3335=VECTOR('',#20847,1000.);
#3336=VECTOR('',#20850,1000.);
#3337=VECTOR('',#20853,1000.);
#3338=VECTOR('',#20856,1000.);
#3339=VECTOR('',#20859,1000.);
#3340=VECTOR('',#20860,1000.);
#3341=VECTOR('',#20861,1000.);
#3342=VECTOR('',#20862,1000.);
#3343=VECTOR('',#20867,1000.);
#3344=VECTOR('',#20868,1000.);
#3345=VECTOR('',#20869,1000.);
#3346=VECTOR('',#20872,1000.);
#3347=VECTOR('',#20875,1000.);
#3348=VECTOR('',#20878,1000.);
#3349=VECTOR('',#20879,1000.);
#3350=VECTOR('',#20886,1000.);
#3351=VECTOR('',#20887,1000.);
#3352=VECTOR('',#20894,1000.);
#3353=VECTOR('',#20895,1000.);
#3354=VECTOR('',#20896,1000.);
#3355=VECTOR('',#20899,1000.);
#3356=VECTOR('',#20900,1000.);
#3357=VECTOR('',#20923,1000.);
#3358=VECTOR('',#20942,1000.);
#3359=VECTOR('',#20945,1000.);
#3360=VECTOR('',#20948,1000.);
#3361=VECTOR('',#20953,1000.);
#3362=VECTOR('',#20954,1000.);
#3363=VECTOR('',#20959,1000.);
#3364=VECTOR('',#20962,1000.);
#3365=VECTOR('',#20965,1000.);
#3366=VECTOR('',#20966,1000.);
#3367=VECTOR('',#20973,1000.);
#3368=VECTOR('',#20974,1000.);
#3369=VECTOR('',#20983,1000.);
#3370=VECTOR('',#20984,1000.);
#3371=VECTOR('',#20989,1000.);
#3372=VECTOR('',#20996,1000.);
#3373=VECTOR('',#21001,1000.);
#3374=VECTOR('',#21002,1000.);
#3375=VECTOR('',#21003,1000.);
#3376=VECTOR('',#21006,1000.);
#3377=VECTOR('',#21007,1000.);
#3378=VECTOR('',#21008,1000.);
#3379=VECTOR('',#21011,1000.);
#3380=VECTOR('',#21012,1000.);
#3381=VECTOR('',#21013,1000.);
#3382=VECTOR('',#21016,1000.);
#3383=VECTOR('',#21025,1000.);
#3384=VECTOR('',#21026,1000.);
#3385=VECTOR('',#21027,1000.);
#3386=VECTOR('',#21034,1000.);
#3387=VECTOR('',#21041,1000.);
#3388=VECTOR('',#21044,1000.);
#3389=VECTOR('',#21049,1000.);
#3390=VECTOR('',#21050,1000.);
#3391=VECTOR('',#21051,1000.);
#3392=VECTOR('',#21054,1000.);
#3393=VECTOR('',#21055,1000.);
#3394=VECTOR('',#21084,1000.);
#3395=VECTOR('',#21127,1000.);
#3396=VECTOR('',#21132,1000.);
#3397=VECTOR('',#21135,1000.);
#3606=CYLINDRICAL_SURFACE('',#16495,19.5);
#3607=CYLINDRICAL_SURFACE('',#16513,16.5);
#3608=CYLINDRICAL_SURFACE('',#16530,5.);
#3609=CYLINDRICAL_SURFACE('',#16546,8.);
#3610=CYLINDRICAL_SURFACE('',#16549,9.);
#3611=CYLINDRICAL_SURFACE('',#16555,14.5);
#3612=CYLINDRICAL_SURFACE('',#16566,2.9);
#3613=CYLINDRICAL_SURFACE('',#16569,0.5);
#3614=CYLINDRICAL_SURFACE('',#16571,19.5);
#3615=CYLINDRICAL_SURFACE('',#16573,6.5);
#3616=CYLINDRICAL_SURFACE('',#16576,5.);
#3617=CYLINDRICAL_SURFACE('',#16579,5.);
#3618=CYLINDRICAL_SURFACE('',#16582,2.);
#3619=CYLINDRICAL_SURFACE('',#16587,2.2295);
#3620=CYLINDRICAL_SURFACE('',#16590,17.5);
#3621=CYLINDRICAL_SURFACE('',#16597,0.5);
#3622=CYLINDRICAL_SURFACE('',#16600,0.499999999999999);
#3623=CYLINDRICAL_SURFACE('',#16606,0.5);
#3624=CYLINDRICAL_SURFACE('',#16611,3.3235);
#3625=CYLINDRICAL_SURFACE('',#16614,0.5);
#3626=CYLINDRICAL_SURFACE('',#16616,0.5);
#3627=CYLINDRICAL_SURFACE('',#16618,4.);
#3628=CYLINDRICAL_SURFACE('',#16620,4.);
#3629=CYLINDRICAL_SURFACE('',#16622,5.5);
#3630=CYLINDRICAL_SURFACE('',#16624,2.5);
#3631=CYLINDRICAL_SURFACE('',#16627,0.5);
#3632=CYLINDRICAL_SURFACE('',#16629,2.067);
#3633=CYLINDRICAL_SURFACE('',#16639,2.5);
#3634=CYLINDRICAL_SURFACE('',#16642,2.);
#3635=CYLINDRICAL_SURFACE('',#16648,0.5);
#3636=CYLINDRICAL_SURFACE('',#16650,0.5);
#3637=CYLINDRICAL_SURFACE('',#16653,21.);
#3638=CYLINDRICAL_SURFACE('',#16660,5.5);
#3639=CYLINDRICAL_SURFACE('',#16663,21.);
#3640=CYLINDRICAL_SURFACE('',#16684,0.5);
#3641=CYLINDRICAL_SURFACE('',#16685,0.499999999999998);
#3642=CYLINDRICAL_SURFACE('',#16691,0.5);
#3643=CYLINDRICAL_SURFACE('',#16693,0.5);
#3644=CYLINDRICAL_SURFACE('',#16698,0.5);
#3645=CYLINDRICAL_SURFACE('',#16700,0.5);
#3646=CYLINDRICAL_SURFACE('',#16705,0.5);
#3647=CYLINDRICAL_SURFACE('',#16707,0.499999999999998);
#3648=CYLINDRICAL_SURFACE('',#16713,0.499999999999998);
#3649=CYLINDRICAL_SURFACE('',#16714,0.499999999999998);
#3650=CYLINDRICAL_SURFACE('',#16720,0.5);
#3651=CYLINDRICAL_SURFACE('',#16721,0.499999999999999);
#3652=CYLINDRICAL_SURFACE('',#16723,0.5);
#3653=CYLINDRICAL_SURFACE('',#16727,0.5);
#3654=CYLINDRICAL_SURFACE('',#16728,0.499999999999998);
#3655=CYLINDRICAL_SURFACE('',#16731,0.5);
#3656=CYLINDRICAL_SURFACE('',#16736,0.499999999999999);
#3657=CYLINDRICAL_SURFACE('',#16738,0.499999999999999);
#3658=CYLINDRICAL_SURFACE('',#16739,0.5);
#3659=CYLINDRICAL_SURFACE('',#16740,0.5);
#3660=CYLINDRICAL_SURFACE('',#16752,5.);
#3661=CYLINDRICAL_SURFACE('',#16757,5.);
#3662=CYLINDRICAL_SURFACE('',#16775,0.5);
#3663=CYLINDRICAL_SURFACE('',#16777,0.499999999999998);
#3664=CYLINDRICAL_SURFACE('',#16781,0.5);
#3665=CYLINDRICAL_SURFACE('',#16783,0.5);
#3666=CYLINDRICAL_SURFACE('',#16785,5.);
#3667=CYLINDRICAL_SURFACE('',#16786,5.);
#3668=CYLINDRICAL_SURFACE('',#16787,0.5);
#3669=CYLINDRICAL_SURFACE('',#16792,0.5);
#3670=CYLINDRICAL_SURFACE('',#16794,0.499999999999998);
#3671=CYLINDRICAL_SURFACE('',#16819,1.);
#3672=CYLINDRICAL_SURFACE('',#16822,0.5);
#3673=CYLINDRICAL_SURFACE('',#16823,1.);
#3674=CYLINDRICAL_SURFACE('',#16825,0.5);
#3675=CYLINDRICAL_SURFACE('',#16826,0.5);
#3676=CYLINDRICAL_SURFACE('',#16827,1.);
#3677=CYLINDRICAL_SURFACE('',#16828,0.5);
#3678=CYLINDRICAL_SURFACE('',#16829,1.);
#3679=CYLINDRICAL_SURFACE('',#16830,1.);
#3680=CYLINDRICAL_SURFACE('',#16832,1.);
#3681=CYLINDRICAL_SURFACE('',#16836,0.999999999999999);
#3682=CYLINDRICAL_SURFACE('',#16840,1.);
#3683=CYLINDRICAL_SURFACE('',#16853,4.5);
#4327=FACE_OUTER_BOUND('',#5258,.T.);
#4328=FACE_OUTER_BOUND('',#5259,.T.);
#4329=FACE_OUTER_BOUND('',#5260,.T.);
#4330=FACE_OUTER_BOUND('',#5261,.T.);
#4331=FACE_OUTER_BOUND('',#5262,.T.);
#4332=FACE_OUTER_BOUND('',#5263,.T.);
#4333=FACE_OUTER_BOUND('',#5264,.T.);
#4334=FACE_OUTER_BOUND('',#5267,.T.);
#4335=FACE_OUTER_BOUND('',#5268,.T.);
#4336=FACE_OUTER_BOUND('',#5269,.T.);
#4337=FACE_OUTER_BOUND('',#5270,.T.);
#4338=FACE_OUTER_BOUND('',#5271,.T.);
#4339=FACE_OUTER_BOUND('',#5272,.T.);
#4340=FACE_OUTER_BOUND('',#5273,.T.);
#4341=FACE_OUTER_BOUND('',#5274,.T.);
#4342=FACE_OUTER_BOUND('',#5275,.T.);
#4343=FACE_OUTER_BOUND('',#5276,.T.);
#4344=FACE_OUTER_BOUND('',#5279,.T.);
#4345=FACE_OUTER_BOUND('',#5280,.T.);
#4346=FACE_OUTER_BOUND('',#5281,.T.);
#4347=FACE_OUTER_BOUND('',#5282,.T.);
#4348=FACE_OUTER_BOUND('',#5283,.T.);
#4349=FACE_OUTER_BOUND('',#5284,.T.);
#4350=FACE_OUTER_BOUND('',#5285,.T.);
#4351=FACE_OUTER_BOUND('',#5286,.T.);
#4352=FACE_OUTER_BOUND('',#5287,.T.);
#4353=FACE_OUTER_BOUND('',#5288,.T.);
#4354=FACE_OUTER_BOUND('',#5289,.T.);
#4355=FACE_OUTER_BOUND('',#5290,.T.);
#4356=FACE_OUTER_BOUND('',#5291,.T.);
#4357=FACE_OUTER_BOUND('',#5292,.T.);
#4358=FACE_OUTER_BOUND('',#5293,.T.);
#4359=FACE_OUTER_BOUND('',#5294,.T.);
#4360=FACE_OUTER_BOUND('',#5295,.T.);
#4361=FACE_OUTER_BOUND('',#5296,.T.);
#4362=FACE_OUTER_BOUND('',#5297,.T.);
#4363=FACE_OUTER_BOUND('',#5298,.T.);
#4364=FACE_OUTER_BOUND('',#5299,.T.);
#4365=FACE_OUTER_BOUND('',#5300,.T.);
#4366=FACE_OUTER_BOUND('',#5301,.T.);
#4367=FACE_OUTER_BOUND('',#5302,.T.);
#4368=FACE_OUTER_BOUND('',#5303,.T.);
#4369=FACE_OUTER_BOUND('',#5304,.T.);
#4370=FACE_OUTER_BOUND('',#5305,.T.);
#4371=FACE_OUTER_BOUND('',#5306,.T.);
#4372=FACE_OUTER_BOUND('',#5307,.T.);
#4373=FACE_OUTER_BOUND('',#5308,.T.);
#4374=FACE_OUTER_BOUND('',#5309,.T.);
#4375=FACE_OUTER_BOUND('',#5310,.T.);
#4376=FACE_OUTER_BOUND('',#5311,.T.);
#4377=FACE_OUTER_BOUND('',#5312,.T.);
#4378=FACE_OUTER_BOUND('',#5313,.T.);
#4379=FACE_OUTER_BOUND('',#5314,.T.);
#4380=FACE_OUTER_BOUND('',#5315,.T.);
#4381=FACE_OUTER_BOUND('',#5316,.T.);
#4382=FACE_OUTER_BOUND('',#5317,.T.);
#4383=FACE_OUTER_BOUND('',#5318,.T.);
#4384=FACE_OUTER_BOUND('',#5322,.T.);
#4385=FACE_OUTER_BOUND('',#5323,.T.);
#4386=FACE_OUTER_BOUND('',#5324,.T.);
#4387=FACE_OUTER_BOUND('',#5325,.T.);
#4388=FACE_OUTER_BOUND('',#5326,.T.);
#4389=FACE_OUTER_BOUND('',#5327,.T.);
#4390=FACE_OUTER_BOUND('',#5328,.T.);
#4391=FACE_OUTER_BOUND('',#5329,.T.);
#4392=FACE_OUTER_BOUND('',#5330,.T.);
#4393=FACE_OUTER_BOUND('',#5331,.T.);
#4394=FACE_OUTER_BOUND('',#5332,.T.);
#4395=FACE_OUTER_BOUND('',#5333,.T.);
#4396=FACE_OUTER_BOUND('',#5334,.T.);
#4397=FACE_OUTER_BOUND('',#5335,.T.);
#4398=FACE_OUTER_BOUND('',#5336,.T.);
#4399=FACE_OUTER_BOUND('',#5337,.T.);
#4400=FACE_OUTER_BOUND('',#5338,.T.);
#4401=FACE_OUTER_BOUND('',#5339,.T.);
#4402=FACE_OUTER_BOUND('',#5340,.T.);
#4403=FACE_OUTER_BOUND('',#5341,.T.);
#4404=FACE_OUTER_BOUND('',#5342,.T.);
#4405=FACE_OUTER_BOUND('',#5343,.T.);
#4406=FACE_OUTER_BOUND('',#5344,.T.);
#4407=FACE_OUTER_BOUND('',#5345,.T.);
#4408=FACE_OUTER_BOUND('',#5346,.T.);
#4409=FACE_OUTER_BOUND('',#5347,.T.);
#4410=FACE_OUTER_BOUND('',#5348,.T.);
#4411=FACE_OUTER_BOUND('',#5349,.T.);
#4412=FACE_OUTER_BOUND('',#5350,.T.);
#4413=FACE_OUTER_BOUND('',#5351,.T.);
#4414=FACE_OUTER_BOUND('',#5352,.T.);
#4415=FACE_OUTER_BOUND('',#5353,.T.);
#4416=FACE_OUTER_BOUND('',#5354,.T.);
#4417=FACE_OUTER_BOUND('',#5355,.T.);
#4418=FACE_OUTER_BOUND('',#5356,.T.);
#4419=FACE_OUTER_BOUND('',#5357,.T.);
#4420=FACE_OUTER_BOUND('',#5358,.T.);
#4421=FACE_OUTER_BOUND('',#5359,.T.);
#4422=FACE_OUTER_BOUND('',#5360,.T.);
#4423=FACE_OUTER_BOUND('',#5361,.T.);
#4424=FACE_OUTER_BOUND('',#5362,.T.);
#4425=FACE_OUTER_BOUND('',#5363,.T.);
#4426=FACE_OUTER_BOUND('',#5364,.T.);
#4427=FACE_OUTER_BOUND('',#5365,.T.);
#4428=FACE_OUTER_BOUND('',#5366,.T.);
#4429=FACE_OUTER_BOUND('',#5367,.T.);
#4430=FACE_OUTER_BOUND('',#5368,.T.);
#4431=FACE_OUTER_BOUND('',#5369,.T.);
#4432=FACE_OUTER_BOUND('',#5371,.T.);
#4433=FACE_OUTER_BOUND('',#5372,.T.);
#4434=FACE_OUTER_BOUND('',#5373,.T.);
#4435=FACE_OUTER_BOUND('',#5375,.T.);
#4436=FACE_OUTER_BOUND('',#5376,.T.);
#4437=FACE_OUTER_BOUND('',#5377,.T.);
#4438=FACE_OUTER_BOUND('',#5379,.T.);
#4439=FACE_OUTER_BOUND('',#5380,.T.);
#4440=FACE_OUTER_BOUND('',#5381,.T.);
#4441=FACE_OUTER_BOUND('',#5382,.T.);
#4442=FACE_OUTER_BOUND('',#5383,.T.);
#4443=FACE_OUTER_BOUND('',#5385,.T.);
#4444=FACE_OUTER_BOUND('',#5388,.T.);
#4445=FACE_OUTER_BOUND('',#5389,.T.);
#4446=FACE_OUTER_BOUND('',#5390,.T.);
#4447=FACE_OUTER_BOUND('',#5391,.T.);
#4448=FACE_OUTER_BOUND('',#5392,.T.);
#4449=FACE_OUTER_BOUND('',#5393,.T.);
#4450=FACE_OUTER_BOUND('',#5394,.T.);
#4451=FACE_OUTER_BOUND('',#5395,.T.);
#4452=FACE_OUTER_BOUND('',#5396,.T.);
#4453=FACE_OUTER_BOUND('',#5397,.T.);
#4454=FACE_OUTER_BOUND('',#5398,.T.);
#4455=FACE_OUTER_BOUND('',#5399,.T.);
#4456=FACE_OUTER_BOUND('',#5400,.T.);
#4457=FACE_OUTER_BOUND('',#5401,.T.);
#4458=FACE_OUTER_BOUND('',#5402,.T.);
#4459=FACE_OUTER_BOUND('',#5403,.T.);
#4460=FACE_OUTER_BOUND('',#5404,.T.);
#4461=FACE_OUTER_BOUND('',#5405,.T.);
#4462=FACE_OUTER_BOUND('',#5406,.T.);
#4463=FACE_OUTER_BOUND('',#5407,.T.);
#4464=FACE_OUTER_BOUND('',#5408,.T.);
#4465=FACE_OUTER_BOUND('',#5409,.T.);
#4466=FACE_OUTER_BOUND('',#5410,.T.);
#4467=FACE_OUTER_BOUND('',#5411,.T.);
#4468=FACE_OUTER_BOUND('',#5414,.T.);
#4469=FACE_OUTER_BOUND('',#5415,.T.);
#4470=FACE_OUTER_BOUND('',#5416,.T.);
#4471=FACE_OUTER_BOUND('',#5417,.T.);
#4472=FACE_OUTER_BOUND('',#5418,.T.);
#4473=FACE_OUTER_BOUND('',#5419,.T.);
#4474=FACE_OUTER_BOUND('',#5420,.T.);
#4475=FACE_OUTER_BOUND('',#5421,.T.);
#4476=FACE_OUTER_BOUND('',#5422,.T.);
#4477=FACE_OUTER_BOUND('',#5423,.T.);
#4478=FACE_OUTER_BOUND('',#5424,.T.);
#4479=FACE_OUTER_BOUND('',#5425,.T.);
#4480=FACE_OUTER_BOUND('',#5426,.T.);
#4481=FACE_OUTER_BOUND('',#5427,.T.);
#4482=FACE_OUTER_BOUND('',#5428,.T.);
#4483=FACE_OUTER_BOUND('',#5429,.T.);
#4484=FACE_OUTER_BOUND('',#5430,.T.);
#4485=FACE_OUTER_BOUND('',#5431,.T.);
#4486=FACE_OUTER_BOUND('',#5432,.T.);
#4487=FACE_OUTER_BOUND('',#5433,.T.);
#4488=FACE_OUTER_BOUND('',#5434,.T.);
#4489=FACE_OUTER_BOUND('',#5435,.T.);
#4490=FACE_OUTER_BOUND('',#5436,.T.);
#4491=FACE_OUTER_BOUND('',#5437,.T.);
#4492=FACE_OUTER_BOUND('',#5438,.T.);
#4493=FACE_OUTER_BOUND('',#5439,.T.);
#4494=FACE_OUTER_BOUND('',#5440,.T.);
#4495=FACE_OUTER_BOUND('',#5441,.T.);
#4496=FACE_OUTER_BOUND('',#5442,.T.);
#4497=FACE_OUTER_BOUND('',#5443,.T.);
#4498=FACE_OUTER_BOUND('',#5444,.T.);
#4499=FACE_OUTER_BOUND('',#5445,.T.);
#4500=FACE_OUTER_BOUND('',#5446,.T.);
#4501=FACE_OUTER_BOUND('',#5447,.T.);
#4502=FACE_OUTER_BOUND('',#5449,.T.);
#4503=FACE_OUTER_BOUND('',#5450,.T.);
#4504=FACE_OUTER_BOUND('',#5451,.T.);
#4505=FACE_OUTER_BOUND('',#5452,.T.);
#4506=FACE_OUTER_BOUND('',#5453,.T.);
#4507=FACE_OUTER_BOUND('',#5454,.T.);
#4508=FACE_OUTER_BOUND('',#5455,.T.);
#4509=FACE_OUTER_BOUND('',#5456,.T.);
#4510=FACE_OUTER_BOUND('',#5457,.T.);
#4511=FACE_OUTER_BOUND('',#5458,.T.);
#4512=FACE_OUTER_BOUND('',#5459,.T.);
#4513=FACE_OUTER_BOUND('',#5460,.T.);
#5258=EDGE_LOOP('',(#13113,#13114,#13115,#13116,#13117,#13118));
#5259=EDGE_LOOP('',(#13119,#13120,#13121,#13122));
#5260=EDGE_LOOP('',(#13123,#13124,#13125,#13126,#13127,#13128,#13129,#13130,
#13131,#13132,#13133,#13134,#13135,#13136,#13137));
#5261=EDGE_LOOP('',(#13138,#13139,#13140,#13141,#13142));
#5262=EDGE_LOOP('',(#13143,#13144,#13145,#13146,#13147,#13148,#13149,#13150,
#13151,#13152));
#5263=EDGE_LOOP('',(#13153,#13154,#13155,#13156));
#5264=EDGE_LOOP('',(#13157,#13158,#13159,#13160,#13161,#13162,#13163,#13164,
#13165,#13166,#13167,#13168,#13169,#13170,#13171,#13172,#13173,#13174,#13175,
#13176,#13177,#13178,#13179,#13180,#13181));
#5265=EDGE_LOOP('',(#13182,#13183,#13184,#13185));
#5266=EDGE_LOOP('',(#13186,#13187));
#5267=EDGE_LOOP('',(#13188,#13189,#13190,#13191));
#5268=EDGE_LOOP('',(#13192,#13193,#13194,#13195,#13196,#13197,#13198,#13199));
#5269=EDGE_LOOP('',(#13200,#13201,#13202,#13203));
#5270=EDGE_LOOP('',(#13204,#13205,#13206,#13207));
#5271=EDGE_LOOP('',(#13208,#13209,#13210,#13211,#13212));
#5272=EDGE_LOOP('',(#13213,#13214,#13215,#13216,#13217));
#5273=EDGE_LOOP('',(#13218,#13219,#13220,#13221,#13222,#13223,#13224));
#5274=EDGE_LOOP('',(#13225,#13226,#13227,#13228,#13229,#13230));
#5275=EDGE_LOOP('',(#13231,#13232,#13233,#13234));
#5276=EDGE_LOOP('',(#13235,#13236,#13237,#13238));
#5277=EDGE_LOOP('',(#13239,#13240));
#5278=EDGE_LOOP('',(#13241,#13242));
#5279=EDGE_LOOP('',(#13243,#13244,#13245,#13246,#13247));
#5280=EDGE_LOOP('',(#13248,#13249,#13250,#13251));
#5281=EDGE_LOOP('',(#13252,#13253,#13254,#13255,#13256,#13257,#13258,#13259));
#5282=EDGE_LOOP('',(#13260,#13261,#13262,#13263));
#5283=EDGE_LOOP('',(#13264,#13265,#13266,#13267));
#5284=EDGE_LOOP('',(#13268,#13269,#13270,#13271,#13272,#13273,#13274));
#5285=EDGE_LOOP('',(#13275,#13276,#13277,#13278,#13279,#13280,#13281,#13282,
#13283,#13284,#13285,#13286,#13287));
#5286=EDGE_LOOP('',(#13288,#13289,#13290,#13291,#13292,#13293,#13294));
#5287=EDGE_LOOP('',(#13295,#13296,#13297,#13298,#13299,#13300,#13301,#13302,
#13303,#13304));
#5288=EDGE_LOOP('',(#13305,#13306,#13307,#13308,#13309,#13310));
#5289=EDGE_LOOP('',(#13311,#13312,#13313,#13314));
#5290=EDGE_LOOP('',(#13315,#13316,#13317,#13318));
#5291=EDGE_LOOP('',(#13319,#13320,#13321));
#5292=EDGE_LOOP('',(#13322,#13323,#13324,#13325));
#5293=EDGE_LOOP('',(#13326,#13327,#13328,#13329));
#5294=EDGE_LOOP('',(#13330,#13331,#13332));
#5295=EDGE_LOOP('',(#13333,#13334,#13335,#13336));
#5296=EDGE_LOOP('',(#13337,#13338,#13339));
#5297=EDGE_LOOP('',(#13340,#13341,#13342,#13343));
#5298=EDGE_LOOP('',(#13344,#13345,#13346,#13347,#13348,#13349));
#5299=EDGE_LOOP('',(#13350,#13351,#13352,#13353,#13354));
#5300=EDGE_LOOP('',(#13355,#13356,#13357,#13358,#13359));
#5301=EDGE_LOOP('',(#13360,#13361,#13362,#13363,#13364));
#5302=EDGE_LOOP('',(#13365,#13366,#13367,#13368));
#5303=EDGE_LOOP('',(#13369,#13370,#13371,#13372));
#5304=EDGE_LOOP('',(#13373,#13374,#13375,#13376));
#5305=EDGE_LOOP('',(#13377,#13378,#13379,#13380));
#5306=EDGE_LOOP('',(#13381,#13382,#13383,#13384));
#5307=EDGE_LOOP('',(#13385,#13386,#13387,#13388));
#5308=EDGE_LOOP('',(#13389,#13390,#13391,#13392));
#5309=EDGE_LOOP('',(#13393,#13394,#13395,#13396));
#5310=EDGE_LOOP('',(#13397,#13398,#13399,#13400));
#5311=EDGE_LOOP('',(#13401));
#5312=EDGE_LOOP('',(#13402));
#5313=EDGE_LOOP('',(#13403));
#5314=EDGE_LOOP('',(#13404,#13405,#13406,#13407));
#5315=EDGE_LOOP('',(#13408,#13409,#13410,#13411));
#5316=EDGE_LOOP('',(#13412,#13413,#13414,#13415));
#5317=EDGE_LOOP('',(#13416,#13417,#13418,#13419));
#5318=EDGE_LOOP('',(#13420,#13421,#13422,#13423,#13424,#13425,#13426,#13427));
#5319=EDGE_LOOP('',(#13428));
#5320=EDGE_LOOP('',(#13429));
#5321=EDGE_LOOP('',(#13430));
#5322=EDGE_LOOP('',(#13431,#13432,#13433,#13434));
#5323=EDGE_LOOP('',(#13435,#13436,#13437,#13438));
#5324=EDGE_LOOP('',(#13439,#13440,#13441,#13442));
#5325=EDGE_LOOP('',(#13443,#13444,#13445,#13446));
#5326=EDGE_LOOP('',(#13447,#13448));
#5327=EDGE_LOOP('',(#13449,#13450,#13451,#13452,#13453));
#5328=EDGE_LOOP('',(#13454,#13455,#13456,#13457,#13458));
#5329=EDGE_LOOP('',(#13459,#13460,#13461,#13462,#13463));
#5330=EDGE_LOOP('',(#13464,#13465,#13466,#13467));
#5331=EDGE_LOOP('',(#13468,#13469,#13470,#13471));
#5332=EDGE_LOOP('',(#13472,#13473,#13474,#13475));
#5333=EDGE_LOOP('',(#13476,#13477,#13478,#13479,#13480));
#5334=EDGE_LOOP('',(#13481,#13482));
#5335=EDGE_LOOP('',(#13483));
#5336=EDGE_LOOP('',(#13484,#13485,#13486,#13487));
#5337=EDGE_LOOP('',(#13488,#13489,#13490));
#5338=EDGE_LOOP('',(#13491,#13492,#13493,#13494));
#5339=EDGE_LOOP('',(#13495,#13496,#13497,#13498));
#5340=EDGE_LOOP('',(#13499,#13500,#13501));
#5341=EDGE_LOOP('',(#13502,#13503,#13504,#13505));
#5342=EDGE_LOOP('',(#13506,#13507,#13508,#13509));
#5343=EDGE_LOOP('',(#13510,#13511,#13512));
#5344=EDGE_LOOP('',(#13513,#13514,#13515,#13516));
#5345=EDGE_LOOP('',(#13517,#13518,#13519,#13520));
#5346=EDGE_LOOP('',(#13521,#13522,#13523));
#5347=EDGE_LOOP('',(#13524,#13525,#13526,#13527));
#5348=EDGE_LOOP('',(#13528,#13529,#13530,#13531));
#5349=EDGE_LOOP('',(#13532,#13533,#13534));
#5350=EDGE_LOOP('',(#13535,#13536,#13537,#13538));
#5351=EDGE_LOOP('',(#13539,#13540,#13541,#13542));
#5352=EDGE_LOOP('',(#13543,#13544,#13545));
#5353=EDGE_LOOP('',(#13546,#13547,#13548,#13549));
#5354=EDGE_LOOP('',(#13550,#13551,#13552,#13553));
#5355=EDGE_LOOP('',(#13554,#13555,#13556,#13557));
#5356=EDGE_LOOP('',(#13558,#13559,#13560));
#5357=EDGE_LOOP('',(#13561,#13562,#13563,#13564));
#5358=EDGE_LOOP('',(#13565,#13566,#13567,#13568));
#5359=EDGE_LOOP('',(#13569,#13570,#13571));
#5360=EDGE_LOOP('',(#13572,#13573,#13574,#13575));
#5361=EDGE_LOOP('',(#13576,#13577,#13578));
#5362=EDGE_LOOP('',(#13579,#13580,#13581,#13582));
#5363=EDGE_LOOP('',(#13583,#13584,#13585,#13586));
#5364=EDGE_LOOP('',(#13587,#13588,#13589,#13590));
#5365=EDGE_LOOP('',(#13591,#13592,#13593,#13594));
#5366=EDGE_LOOP('',(#13595,#13596,#13597,#13598));
#5367=EDGE_LOOP('',(#13599,#13600,#13601,#13602,#13603,#13604,#13605,#13606,
#13607));
#5368=EDGE_LOOP('',(#13608,#13609,#13610,#13611));
#5369=EDGE_LOOP('',(#13612,#13613,#13614,#13615,#13616,#13617,#13618,#13619));
#5370=EDGE_LOOP('',(#13620));
#5371=EDGE_LOOP('',(#13621,#13622,#13623,#13624,#13625));
#5372=EDGE_LOOP('',(#13626,#13627,#13628));
#5373=EDGE_LOOP('',(#13629,#13630,#13631,#13632));
#5374=EDGE_LOOP('',(#13633));
#5375=EDGE_LOOP('',(#13634,#13635,#13636,#13637,#13638,#13639));
#5376=EDGE_LOOP('',(#13640,#13641,#13642));
#5377=EDGE_LOOP('',(#13643,#13644,#13645,#13646,#13647,#13648,#13649));
#5378=EDGE_LOOP('',(#13650));
#5379=EDGE_LOOP('',(#13651,#13652,#13653,#13654));
#5380=EDGE_LOOP('',(#13655,#13656,#13657));
#5381=EDGE_LOOP('',(#13658,#13659,#13660,#13661,#13662));
#5382=EDGE_LOOP('',(#13663,#13664,#13665,#13666,#13667,#13668));
#5383=EDGE_LOOP('',(#13669));
#5384=EDGE_LOOP('',(#13670));
#5385=EDGE_LOOP('',(#13671,#13672,#13673,#13674,#13675,#13676,#13677,#13678));
#5386=EDGE_LOOP('',(#13679));
#5387=EDGE_LOOP('',(#13680));
#5388=EDGE_LOOP('',(#13681,#13682,#13683,#13684));
#5389=EDGE_LOOP('',(#13685,#13686,#13687,#13688));
#5390=EDGE_LOOP('',(#13689,#13690,#13691,#13692));
#5391=EDGE_LOOP('',(#13693,#13694,#13695));
#5392=EDGE_LOOP('',(#13696,#13697,#13698,#13699));
#5393=EDGE_LOOP('',(#13700,#13701,#13702,#13703));
#5394=EDGE_LOOP('',(#13704,#13705,#13706,#13707));
#5395=EDGE_LOOP('',(#13708,#13709,#13710,#13711));
#5396=EDGE_LOOP('',(#13712,#13713,#13714,#13715,#13716,#13717));
#5397=EDGE_LOOP('',(#13718,#13719,#13720));
#5398=EDGE_LOOP('',(#13721,#13722,#13723));
#5399=EDGE_LOOP('',(#13724,#13725,#13726,#13727));
#5400=EDGE_LOOP('',(#13728,#13729,#13730));
#5401=EDGE_LOOP('',(#13731,#13732,#13733,#13734,#13735,#13736,#13737,#13738,
#13739));
#5402=EDGE_LOOP('',(#13740,#13741,#13742,#13743));
#5403=EDGE_LOOP('',(#13744,#13745,#13746,#13747,#13748,#13749,#13750));
#5404=EDGE_LOOP('',(#13751,#13752,#13753,#13754,#13755,#13756,#13757,#13758,
#13759,#13760));
#5405=EDGE_LOOP('',(#13761,#13762,#13763,#13764));
#5406=EDGE_LOOP('',(#13765,#13766,#13767,#13768,#13769,#13770));
#5407=EDGE_LOOP('',(#13771,#13772,#13773,#13774));
#5408=EDGE_LOOP('',(#13775,#13776,#13777,#13778));
#5409=EDGE_LOOP('',(#13779,#13780,#13781,#13782));
#5410=EDGE_LOOP('',(#13783,#13784,#13785,#13786,#13787,#13788,#13789,#13790,
#13791,#13792,#13793,#13794,#13795,#13796,#13797,#13798));
#5411=EDGE_LOOP('',(#13799,#13800,#13801,#13802,#13803,#13804,#13805,#13806,
#13807,#13808,#13809,#13810,#13811,#13812));
#5412=EDGE_LOOP('',(#13813));
#5413=EDGE_LOOP('',(#13814));
#5414=EDGE_LOOP('',(#13815,#13816,#13817,#13818));
#5415=EDGE_LOOP('',(#13819,#13820,#13821,#13822));
#5416=EDGE_LOOP('',(#13823,#13824,#13825,#13826,#13827,#13828,#13829,#13830));
#5417=EDGE_LOOP('',(#13831,#13832,#13833,#13834));
#5418=EDGE_LOOP('',(#13835,#13836,#13837,#13838));
#5419=EDGE_LOOP('',(#13839,#13840,#13841,#13842,#13843,#13844,#13845));
#5420=EDGE_LOOP('',(#13846,#13847,#13848,#13849));
#5421=EDGE_LOOP('',(#13850,#13851,#13852,#13853));
#5422=EDGE_LOOP('',(#13854,#13855,#13856,#13857));
#5423=EDGE_LOOP('',(#13858,#13859,#13860,#13861,#13862,#13863,#13864,#13865,
#13866,#13867));
#5424=EDGE_LOOP('',(#13868,#13869,#13870,#13871,#13872,#13873,#13874,#13875));
#5425=EDGE_LOOP('',(#13876,#13877,#13878,#13879,#13880,#13881,#13882,#13883));
#5426=EDGE_LOOP('',(#13884,#13885,#13886,#13887,#13888,#13889,#13890,#13891));
#5427=EDGE_LOOP('',(#13892,#13893,#13894));
#5428=EDGE_LOOP('',(#13895,#13896,#13897,#13898));
#5429=EDGE_LOOP('',(#13899,#13900,#13901,#13902,#13903));
#5430=EDGE_LOOP('',(#13904,#13905,#13906,#13907));
#5431=EDGE_LOOP('',(#13908,#13909,#13910,#13911,#13912));
#5432=EDGE_LOOP('',(#13913,#13914,#13915,#13916,#13917));
#5433=EDGE_LOOP('',(#13918,#13919,#13920,#13921));
#5434=EDGE_LOOP('',(#13922,#13923,#13924,#13925));
#5435=EDGE_LOOP('',(#13926,#13927,#13928,#13929));
#5436=EDGE_LOOP('',(#13930,#13931,#13932,#13933));
#5437=EDGE_LOOP('',(#13934,#13935,#13936,#13937));
#5438=EDGE_LOOP('',(#13938,#13939,#13940,#13941));
#5439=EDGE_LOOP('',(#13942,#13943,#13944,#13945,#13946,#13947));
#5440=EDGE_LOOP('',(#13948,#13949,#13950,#13951));
#5441=EDGE_LOOP('',(#13952,#13953,#13954,#13955));
#5442=EDGE_LOOP('',(#13956,#13957,#13958,#13959));
#5443=EDGE_LOOP('',(#13960,#13961,#13962,#13963));
#5444=EDGE_LOOP('',(#13964,#13965,#13966,#13967));
#5445=EDGE_LOOP('',(#13968,#13969,#13970,#13971,#13972,#13973,#13974,#13975,
#13976,#13977));
#5446=EDGE_LOOP('',(#13978,#13979,#13980,#13981,#13982,#13983));
#5447=EDGE_LOOP('',(#13984));
#5448=EDGE_LOOP('',(#13985));
#5449=EDGE_LOOP('',(#13986,#13987,#13988,#13989,#13990));
#5450=EDGE_LOOP('',(#13991,#13992,#13993,#13994,#13995));
#5451=EDGE_LOOP('',(#13996,#13997,#13998,#13999));
#5452=EDGE_LOOP('',(#14000,#14001,#14002,#14003,#14004,#14005,#14006));
#5453=EDGE_LOOP('',(#14007,#14008,#14009,#14010));
#5454=EDGE_LOOP('',(#14011,#14012,#14013,#14014));
#5455=EDGE_LOOP('',(#14015,#14016,#14017,#14018,#14019));
#5456=EDGE_LOOP('',(#14020,#14021));
#5457=EDGE_LOOP('',(#14022,#14023,#14024,#14025,#14026,#14027,#14028,#14029));
#5458=EDGE_LOOP('',(#14030,#14031,#14032,#14033,#14034,#14035,#14036,#14037,
#14038,#14039,#14040,#14041,#14042,#14043,#14044));
#5459=EDGE_LOOP('',(#14045,#14046));
#5460=EDGE_LOOP('',(#14047,#14048,#14049,#14050,#14051,#14052,#14053,#14054,
#14055));
#5461=EDGE_LOOP('',(#14056));
#6003=CIRCLE('',#16491,17.0599057548774);
#6004=CIRCLE('',#16492,0.500000000000001);
#6005=CIRCLE('',#16493,0.500000000000001);
#6006=CIRCLE('',#16494,16.5718869058529);
#6007=CIRCLE('',#16496,19.5);
#6008=CIRCLE('',#16497,19.5);
#6009=CIRCLE('',#16499,2.50461426675156);
#6010=CIRCLE('',#16500,2.60305176675156);
#6011=CIRCLE('',#16501,2.50461426675156);
#6012=CIRCLE('',#16503,2.20465088114115);
#6013=CIRCLE('',#16505,19.3089875327072);
#6014=CIRCLE('',#16506,16.6910124672929);
#6015=CIRCLE('',#16507,16.6910124672929);
#6016=CIRCLE('',#16508,16.6910124672929);
#6017=CIRCLE('',#16509,16.6910124672929);
#6018=CIRCLE('',#16511,19.5);
#6019=CIRCLE('',#16512,3.);
#6020=CIRCLE('',#16514,16.5);
#6021=CIRCLE('',#16515,16.5);
#6022=CIRCLE('',#16516,16.5);
#6023=CIRCLE('',#16517,16.5);
#6024=CIRCLE('',#16518,16.5);
#6025=CIRCLE('',#16519,5.45169314906474);
#6026=CIRCLE('',#16520,16.5);
#6027=CIRCLE('',#16521,16.5);
#6028=CIRCLE('',#16522,16.5);
#6029=CIRCLE('',#16523,16.5);
#6030=CIRCLE('',#16524,16.5);
#6031=CIRCLE('',#16526,4.5992601276539);
#6032=CIRCLE('',#16528,19.5);
#6033=CIRCLE('',#16529,0.5);
#6034=CIRCLE('',#16531,5.);
#6035=CIRCLE('',#16533,5.5);
#6036=CIRCLE('',#16534,1.);
#6037=CIRCLE('',#16535,4.5);
#6038=CIRCLE('',#16536,1.);
#6039=CIRCLE('',#16538,0.5);
#6040=CIRCLE('',#16539,19.5);
#6041=CIRCLE('',#16540,1.00000000000008);
#6042=CIRCLE('',#16541,6.65199991070048);
#6043=CIRCLE('',#16542,1.00000000000005);
#6044=CIRCLE('',#16544,17.5);
#6045=CIRCLE('',#16545,1.);
#6046=CIRCLE('',#16547,8.);
#6047=CIRCLE('',#16548,6.65097177940297);
#6048=CIRCLE('',#16550,9.);
#6049=CIRCLE('',#16552,1.);
#6050=CIRCLE('',#16553,0.500000000000001);
#6051=CIRCLE('',#16554,0.5);
#6052=CIRCLE('',#16556,14.5);
#6053=CIRCLE('',#16557,14.5);
#6054=CIRCLE('',#16558,0.500000000000013);
#6055=CIRCLE('',#16559,4.31029789941839);
#6056=CIRCLE('',#16560,0.499999999999922);
#6057=CIRCLE('',#16562,6.5);
#6058=CIRCLE('',#16563,0.499999999999999);
#6059=CIRCLE('',#16564,6.);
#6060=CIRCLE('',#16565,0.5);
#6061=CIRCLE('',#16567,2.9);
#6062=CIRCLE('',#16568,2.9);
#6063=CIRCLE('',#16574,6.5);
#6064=CIRCLE('',#16575,6.5);
#6065=CIRCLE('',#16577,5.);
#6066=CIRCLE('',#16580,2.67271103248174);
#6067=CIRCLE('',#16583,2.);
#6068=CIRCLE('',#16585,2.);
#6069=CIRCLE('',#16586,2.);
#6070=CIRCLE('',#16588,2.2295);
#6071=CIRCLE('',#16589,2.2295);
#6072=CIRCLE('',#16591,17.5);
#6073=CIRCLE('',#16592,17.5);
#6074=CIRCLE('',#16594,0.500000000000001);
#6075=CIRCLE('',#16595,0.499999999999998);
#6076=CIRCLE('',#16596,0.500000000000003);
#6077=CIRCLE('',#16598,0.5);
#6078=CIRCLE('',#16599,0.5);
#6079=CIRCLE('',#16601,0.499999999999999);
#6080=CIRCLE('',#16602,0.5);
#6081=CIRCLE('',#16604,0.499999999999998);
#6082=CIRCLE('',#16605,0.5);
#6083=CIRCLE('',#16609,0.499999999999998);
#6084=CIRCLE('',#16610,0.499999999999998);
#6085=CIRCLE('',#16612,3.3235);
#6086=CIRCLE('',#16613,3.3235);
#6087=CIRCLE('',#16615,0.5);
#6088=CIRCLE('',#16617,0.5);
#6089=CIRCLE('',#16619,4.);
#6090=CIRCLE('',#16621,4.);
#6091=CIRCLE('',#16623,5.5);
#6092=CIRCLE('',#16625,2.5);
#6093=CIRCLE('',#16626,2.5);
#6094=CIRCLE('',#16628,0.5);
#6095=CIRCLE('',#16630,2.067);
#6096=CIRCLE('',#16631,2.067);
#6097=CIRCLE('',#16633,5.);
#6098=CIRCLE('',#16634,14.8183541121548);
#6099=CIRCLE('',#16636,17.4363291775691);
#6100=CIRCLE('',#16638,1.);
#6101=CIRCLE('',#16640,2.5);
#6102=CIRCLE('',#16641,2.5);
#6103=CIRCLE('',#16643,2.);
#6104=CIRCLE('',#16644,2.);
#6105=CIRCLE('',#16649,0.5);
#6106=CIRCLE('',#16651,0.5);
#6107=CIRCLE('',#16654,21.);
#6108=CIRCLE('',#16655,21.);
#6109=CIRCLE('',#16657,5.5);
#6110=CIRCLE('',#16658,21.);
#6111=CIRCLE('',#16661,5.5);
#6112=CIRCLE('',#16664,21.);
#6113=CIRCLE('',#16666,0.499999999999999);
#6114=CIRCLE('',#16667,0.5);
#6115=CIRCLE('',#16668,0.5);
#6116=CIRCLE('',#16669,0.5);
#6117=CIRCLE('',#16670,0.500000000000001);
#6118=CIRCLE('',#16672,0.500000000000001);
#6119=CIRCLE('',#16673,17.);
#6120=CIRCLE('',#16677,1.);
#6121=CIRCLE('',#16678,1.);
#6122=CIRCLE('',#16679,20.);
#6123=CIRCLE('',#16681,0.5);
#6124=CIRCLE('',#16682,0.500000000000001);
#6125=CIRCLE('',#16683,0.5);
#6126=CIRCLE('',#16686,0.500000000000002);
#6127=CIRCLE('',#16688,0.5);
#6128=CIRCLE('',#16689,0.5);
#6129=CIRCLE('',#16690,0.5);
#6130=CIRCLE('',#16692,0.5);
#6131=CIRCLE('',#16696,0.5);
#6132=CIRCLE('',#16697,0.5);
#6133=CIRCLE('',#16699,0.5);
#6134=CIRCLE('',#16703,0.5);
#6135=CIRCLE('',#16704,0.5);
#6136=CIRCLE('',#16710,0.499999999999998);
#6137=CIRCLE('',#16711,0.499999999999998);
#6138=CIRCLE('',#16712,0.5);
#6139=CIRCLE('',#16715,0.499999999999996);
#6140=CIRCLE('',#16716,0.499999999999998);
#6141=CIRCLE('',#16718,0.5);
#6142=CIRCLE('',#16719,0.5);
#6143=CIRCLE('',#16722,0.499999999999999);
#6144=CIRCLE('',#16724,0.499999999999998);
#6145=CIRCLE('',#16726,0.5);
#6146=CIRCLE('',#16732,0.5);
#6147=CIRCLE('',#16734,0.500000000000002);
#6148=CIRCLE('',#16735,0.500000000000001);
#6149=CIRCLE('',#16737,0.499999999999999);
#6150=CIRCLE('',#16744,1.);
#6151=CIRCLE('',#16747,1.);
#6152=CIRCLE('',#16750,0.959917621886371);
#6153=CIRCLE('',#16753,5.);
#6154=CIRCLE('',#16760,5.);
#6155=CIRCLE('',#16762,0.499999999999999);
#6156=CIRCLE('',#16763,6.);
#6157=CIRCLE('',#16764,0.499999999999999);
#6158=CIRCLE('',#16770,0.5);
#6159=CIRCLE('',#16772,0.499999999999998);
#6160=CIRCLE('',#16773,0.5);
#6161=CIRCLE('',#16774,0.500000000000001);
#6162=CIRCLE('',#16776,0.5);
#6163=CIRCLE('',#16795,0.499999999999998);
#6164=CIRCLE('',#16799,1.);
#6165=CIRCLE('',#16800,20.);
#6166=CIRCLE('',#16801,4.5);
#6167=CIRCLE('',#16805,2.39349905057784);
#6168=CIRCLE('',#16811,17.5);
#6169=CIRCLE('',#16815,0.5);
#6170=CIRCLE('',#16817,1.);
#6171=CIRCLE('',#16818,1.);
#6172=CIRCLE('',#16821,0.999999999999999);
#6173=CIRCLE('',#16824,1.);
#6174=CIRCLE('',#16833,1.);
#6175=CIRCLE('',#16835,1.);
#6176=CIRCLE('',#16837,1.);
#6177=CIRCLE('',#16839,1.);
#6178=CIRCLE('',#16843,1.);
#6179=CIRCLE('',#16844,0.999999999999999);
#6180=CIRCLE('',#16846,2.30308838114115);
#6181=CIRCLE('',#16854,4.5);
#7270=VERTEX_POINT('',#45570);
#7271=VERTEX_POINT('',#45571);
#7272=VERTEX_POINT('',#45584);
#7273=VERTEX_POINT('',#45586);
#7274=VERTEX_POINT('',#45588);
#7275=VERTEX_POINT('',#45590);
#7276=VERTEX_POINT('',#45594);
#7277=VERTEX_POINT('',#45596);
#7278=VERTEX_POINT('',#45600);
#7279=VERTEX_POINT('',#45601);
#7280=VERTEX_POINT('',#45747);
#7281=VERTEX_POINT('',#45752);
#7282=VERTEX_POINT('',#46033);
#7283=VERTEX_POINT('',#46038);
#7284=VERTEX_POINT('',#46085);
#7285=VERTEX_POINT('',#46087);
#7286=VERTEX_POINT('',#46089);
#7287=VERTEX_POINT('',#46098);
#7288=VERTEX_POINT('',#46100);
#7289=VERTEX_POINT('',#46112);
#7290=VERTEX_POINT('',#46154);
#7291=VERTEX_POINT('',#46341);
#7292=VERTEX_POINT('',#46342);
#7293=VERTEX_POINT('',#46365);
#7294=VERTEX_POINT('',#46367);
#7295=VERTEX_POINT('',#46369);
#7296=VERTEX_POINT('',#46371);
#7297=VERTEX_POINT('',#46655);
#7298=VERTEX_POINT('',#46657);
#7299=VERTEX_POINT('',#46680);
#7300=VERTEX_POINT('',#46682);
#7301=VERTEX_POINT('',#47028);
#7302=VERTEX_POINT('',#47032);
#7303=VERTEX_POINT('',#47033);
#7304=VERTEX_POINT('',#47035);
#7305=VERTEX_POINT('',#47037);
#7306=VERTEX_POINT('',#47039);
#7307=VERTEX_POINT('',#47296);
#7308=VERTEX_POINT('',#48195);
#7309=VERTEX_POINT('',#48228);
#7310=VERTEX_POINT('',#48230);
#7311=VERTEX_POINT('',#48342);
#7312=VERTEX_POINT('',#48366);
#7313=VERTEX_POINT('',#48368);
#7314=VERTEX_POINT('',#48370);
#7315=VERTEX_POINT('',#48372);
#7316=VERTEX_POINT('',#48397);
#7317=VERTEX_POINT('',#48399);
#7318=VERTEX_POINT('',#48401);
#7319=VERTEX_POINT('',#48565);
#7320=VERTEX_POINT('',#48567);
#7321=VERTEX_POINT('',#48906);
#7322=VERTEX_POINT('',#48908);
#7323=VERTEX_POINT('',#48910);
#7324=VERTEX_POINT('',#48912);
#7325=VERTEX_POINT('',#49044);
#7326=VERTEX_POINT('',#49045);
#7327=VERTEX_POINT('',#49047);
#7328=VERTEX_POINT('',#49469);
#7329=VERTEX_POINT('',#49862);
#7330=VERTEX_POINT('',#49863);
#7331=VERTEX_POINT('',#50108);
#7332=VERTEX_POINT('',#50112);
#7333=VERTEX_POINT('',#50113);
#7334=VERTEX_POINT('',#50120);
#7335=VERTEX_POINT('',#50239);
#7336=VERTEX_POINT('',#50241);
#7337=VERTEX_POINT('',#50243);
#7338=VERTEX_POINT('',#50245);
#7339=VERTEX_POINT('',#50309);
#7340=VERTEX_POINT('',#50703);
#7341=VERTEX_POINT('',#50704);
#7342=VERTEX_POINT('',#50706);
#7343=VERTEX_POINT('',#50708);
#7344=VERTEX_POINT('',#50712);
#7345=VERTEX_POINT('',#51501);
#7346=VERTEX_POINT('',#51503);
#7347=VERTEX_POINT('',#51505);
#7348=VERTEX_POINT('',#51627);
#7349=VERTEX_POINT('',#51640);
#7350=VERTEX_POINT('',#51644);
#7351=VERTEX_POINT('',#51647);
#7352=VERTEX_POINT('',#51776);
#7353=VERTEX_POINT('',#51777);
#7354=VERTEX_POINT('',#51849);
#7355=VERTEX_POINT('',#51972);
#7356=VERTEX_POINT('',#52118);
#7357=VERTEX_POINT('',#52120);
#7358=VERTEX_POINT('',#52124);
#7359=VERTEX_POINT('',#52125);
#7360=VERTEX_POINT('',#52132);
#7361=VERTEX_POINT('',#52134);
#7362=VERTEX_POINT('',#52138);
#7363=VERTEX_POINT('',#52140);
#7364=VERTEX_POINT('',#52143);
#7365=VERTEX_POINT('',#52144);
#7366=VERTEX_POINT('',#52182);
#7367=VERTEX_POINT('',#52183);
#7368=VERTEX_POINT('',#53019);
#7369=VERTEX_POINT('',#53021);
#7370=VERTEX_POINT('',#53419);
#7371=VERTEX_POINT('',#53423);
#7372=VERTEX_POINT('',#53424);
#7373=VERTEX_POINT('',#53426);
#7374=VERTEX_POINT('',#53428);
#7375=VERTEX_POINT('',#53432);
#7376=VERTEX_POINT('',#53433);
#7377=VERTEX_POINT('',#53435);
#7378=VERTEX_POINT('',#53446);
#7379=VERTEX_POINT('',#53448);
#7380=VERTEX_POINT('',#53459);
#7381=VERTEX_POINT('',#53461);
#7382=VERTEX_POINT('',#53472);
#7383=VERTEX_POINT('',#53485);
#7384=VERTEX_POINT('',#53487);
#7385=VERTEX_POINT('',#53507);
#7386=VERTEX_POINT('',#53568);
#7387=VERTEX_POINT('',#53569);
#7388=VERTEX_POINT('',#53582);
#7389=VERTEX_POINT('',#53605);
#7390=VERTEX_POINT('',#53625);
#7391=VERTEX_POINT('',#53684);
#7392=VERTEX_POINT('',#53686);
#7393=VERTEX_POINT('',#53707);
#7394=VERTEX_POINT('',#53709);
#7395=VERTEX_POINT('',#53711);
#7396=VERTEX_POINT('',#53713);
#7397=VERTEX_POINT('',#53835);
#7398=VERTEX_POINT('',#53836);
#7399=VERTEX_POINT('',#53844);
#7400=VERTEX_POINT('',#54038);
#7401=VERTEX_POINT('',#54040);
#7402=VERTEX_POINT('',#54064);
#7403=VERTEX_POINT('',#54500);
#7404=VERTEX_POINT('',#54501);
#7405=VERTEX_POINT('',#54503);
#7406=VERTEX_POINT('',#54506);
#7407=VERTEX_POINT('',#54510);
#7408=VERTEX_POINT('',#54512);
#7409=VERTEX_POINT('',#54516);
#7410=VERTEX_POINT('',#54518);
#7411=VERTEX_POINT('',#54522);
#7412=VERTEX_POINT('',#54523);
#7413=VERTEX_POINT('',#54525);
#7414=VERTEX_POINT('',#54529);
#7415=VERTEX_POINT('',#54530);
#7416=VERTEX_POINT('',#54532);
#7417=VERTEX_POINT('',#54534);
#7418=VERTEX_POINT('',#54538);
#7419=VERTEX_POINT('',#54540);
#7420=VERTEX_POINT('',#54542);
#7421=VERTEX_POINT('',#54546);
#7422=VERTEX_POINT('',#54550);
#7423=VERTEX_POINT('',#54551);
#7424=VERTEX_POINT('',#54556);
#7425=VERTEX_POINT('',#54560);
#7426=VERTEX_POINT('',#54562);
#7427=VERTEX_POINT('',#54566);
#7428=VERTEX_POINT('',#54567);
#7429=VERTEX_POINT('',#54632);
#7430=VERTEX_POINT('',#54688);
#7431=VERTEX_POINT('',#54690);
#7432=VERTEX_POINT('',#54695);
#7433=VERTEX_POINT('',#54697);
#7434=VERTEX_POINT('',#54834);
#7435=VERTEX_POINT('',#54967);
#7436=VERTEX_POINT('',#54971);
#7437=VERTEX_POINT('',#54975);
#7438=VERTEX_POINT('',#54977);
#7439=VERTEX_POINT('',#54981);
#7440=VERTEX_POINT('',#54983);
#7441=VERTEX_POINT('',#54987);
#7442=VERTEX_POINT('',#54998);
#7443=VERTEX_POINT('',#55002);
#7444=VERTEX_POINT('',#55004);
#7445=VERTEX_POINT('',#55008);
#7446=VERTEX_POINT('',#55012);
#7447=VERTEX_POINT('',#55018);
#7448=VERTEX_POINT('',#55020);
#7449=VERTEX_POINT('',#55024);
#7450=VERTEX_POINT('',#55026);
#7451=VERTEX_POINT('',#55033);
#7452=VERTEX_POINT('',#55101);
#7453=VERTEX_POINT('',#55105);
#7454=VERTEX_POINT('',#55106);
#7455=VERTEX_POINT('',#55120);
#7456=VERTEX_POINT('',#55121);
#7457=VERTEX_POINT('',#55126);
#7458=VERTEX_POINT('',#55127);
#7459=VERTEX_POINT('',#55132);
#7460=VERTEX_POINT('',#55133);
#7461=VERTEX_POINT('',#55136);
#7462=VERTEX_POINT('',#55138);
#7463=VERTEX_POINT('',#55142);
#7464=VERTEX_POINT('',#55146);
#7465=VERTEX_POINT('',#55150);
#7466=VERTEX_POINT('',#55154);
#7467=VERTEX_POINT('',#55631);
#7468=VERTEX_POINT('',#55775);
#7469=VERTEX_POINT('',#56057);
#7470=VERTEX_POINT('',#56059);
#7471=VERTEX_POINT('',#56063);
#7472=VERTEX_POINT('',#56064);
#7473=VERTEX_POINT('',#56066);
#7474=VERTEX_POINT('',#56073);
#7475=VERTEX_POINT('',#56074);
#7476=VERTEX_POINT('',#56079);
#7477=VERTEX_POINT('',#56080);
#7478=VERTEX_POINT('',#56082);
#7479=VERTEX_POINT('',#56086);
#7480=VERTEX_POINT('',#56087);
#7481=VERTEX_POINT('',#56092);
#7482=VERTEX_POINT('',#56093);
#7483=VERTEX_POINT('',#56098);
#7484=VERTEX_POINT('',#56102);
#7485=VERTEX_POINT('',#56103);
#7486=VERTEX_POINT('',#56108);
#7487=VERTEX_POINT('',#56109);
#7488=VERTEX_POINT('',#56114);
#7489=VERTEX_POINT('',#56118);
#7490=VERTEX_POINT('',#56119);
#7491=VERTEX_POINT('',#56124);
#7492=VERTEX_POINT('',#56126);
#7493=VERTEX_POINT('',#56130);
#7494=VERTEX_POINT('',#56131);
#7495=VERTEX_POINT('',#56133);
#7496=VERTEX_POINT('',#56140);
#7497=VERTEX_POINT('',#56141);
#7498=VERTEX_POINT('',#56147);
#7499=VERTEX_POINT('',#56154);
#7500=VERTEX_POINT('',#56156);
#7501=VERTEX_POINT('',#56160);
#7502=VERTEX_POINT('',#56170);
#7503=VERTEX_POINT('',#56172);
#7504=VERTEX_POINT('',#56177);
#7505=VERTEX_POINT('',#56179);
#7506=VERTEX_POINT('',#56183);
#7507=VERTEX_POINT('',#56187);
#7508=VERTEX_POINT('',#56198);
#7509=VERTEX_POINT('',#56200);
#7510=VERTEX_POINT('',#56206);
#7511=VERTEX_POINT('',#56209);
#7512=VERTEX_POINT('',#56211);
#7513=VERTEX_POINT('',#56215);
#7514=VERTEX_POINT('',#56216);
#7515=VERTEX_POINT('',#56221);
#7516=VERTEX_POINT('',#56222);
#7517=VERTEX_POINT('',#56224);
#7518=VERTEX_POINT('',#56226);
#7519=VERTEX_POINT('',#56228);
#7520=VERTEX_POINT('',#56233);
#7521=VERTEX_POINT('',#56235);
#7522=VERTEX_POINT('',#56237);
#7523=VERTEX_POINT('',#56241);
#7524=VERTEX_POINT('',#56248);
#7525=VERTEX_POINT('',#56250);
#7526=VERTEX_POINT('',#56255);
#7527=VERTEX_POINT('',#56263);
#7528=VERTEX_POINT('',#56265);
#7529=VERTEX_POINT('',#56396);
#7530=VERTEX_POINT('',#56446);
#7531=VERTEX_POINT('',#56448);
#7532=VERTEX_POINT('',#56463);
#7533=VERTEX_POINT('',#56465);
#7534=VERTEX_POINT('',#56472);
#7535=VERTEX_POINT('',#57047);
#7536=VERTEX_POINT('',#57049);
#7537=VERTEX_POINT('',#58856);
#7538=VERTEX_POINT('',#58860);
#7539=VERTEX_POINT('',#58965);
#7540=VERTEX_POINT('',#58995);
#7541=VERTEX_POINT('',#58999);
#7542=VERTEX_POINT('',#59003);
#7543=VERTEX_POINT('',#59005);
#7544=VERTEX_POINT('',#59008);
#7545=VERTEX_POINT('',#59010);
#7546=VERTEX_POINT('',#59012);
#7547=VERTEX_POINT('',#59018);
#7548=VERTEX_POINT('',#59021);
#7549=VERTEX_POINT('',#59030);
#7550=VERTEX_POINT('',#59032);
#7551=VERTEX_POINT('',#59038);
#7552=VERTEX_POINT('',#59042);
#7553=VERTEX_POINT('',#59049);
#7554=VERTEX_POINT('',#59203);
#7555=VERTEX_POINT('',#60712);
#7556=VERTEX_POINT('',#62604);
#7557=VERTEX_POINT('',#62615);
#7558=VERTEX_POINT('',#62633);
#7559=VERTEX_POINT('',#62635);
#9263=EDGE_CURVE('',#7270,#7271,#917,.F.);
#9264=EDGE_CURVE('',#7272,#7270,#770,.T.);
#9265=EDGE_CURVE('',#7273,#7272,#6003,.T.);
#9266=EDGE_CURVE('',#7274,#7273,#6004,.T.);
#9267=EDGE_CURVE('',#7275,#7274,#6005,.T.);
#9268=EDGE_CURVE('',#7271,#7275,#6006,.T.);
#9269=EDGE_CURVE('',#7276,#7276,#6007,.T.);
#9270=EDGE_CURVE('',#7276,#7277,#2044,.T.);
#9271=EDGE_CURVE('',#7277,#7277,#6008,.T.);
#9272=EDGE_CURVE('',#7278,#7279,#918,.T.);
#9273=EDGE_CURVE('',#7279,#7280,#919,.T.);
#9274=EDGE_CURVE('',#7280,#7281,#920,.T.);
#9275=EDGE_CURVE('',#7281,#7282,#921,.T.);
#9276=EDGE_CURVE('',#7282,#7283,#922,.T.);
#9277=EDGE_CURVE('',#7283,#7284,#2045,.T.);
#9278=EDGE_CURVE('',#7284,#7285,#6009,.T.);
#9279=EDGE_CURVE('',#7285,#7286,#923,.T.);
#9280=EDGE_CURVE('',#7286,#7287,#6010,.T.);
#9281=EDGE_CURVE('',#7287,#7288,#924,.T.);
#9282=EDGE_CURVE('',#7288,#7284,#6011,.T.);
#9283=EDGE_CURVE('',#7283,#7289,#925,.T.);
#9284=EDGE_CURVE('',#7289,#7290,#926,.T.);
#9285=EDGE_CURVE('',#7290,#7278,#927,.T.);
#9286=EDGE_CURVE('',#7291,#7292,#6012,.T.);
#9287=EDGE_CURVE('',#7285,#7291,#928,.T.);
#9288=EDGE_CURVE('',#7292,#7288,#929,.T.);
#9289=EDGE_CURVE('',#7293,#7293,#6013,.T.);
#9290=EDGE_CURVE('',#7293,#7294,#2046,.T.);
#9291=EDGE_CURVE('',#7294,#7295,#6014,.T.);
#9292=EDGE_CURVE('',#7295,#7296,#930,.T.);
#9293=EDGE_CURVE('',#7296,#7297,#6015,.T.);
#9294=EDGE_CURVE('',#7297,#7298,#931,.T.);
#9295=EDGE_CURVE('',#7298,#7299,#6016,.T.);
#9296=EDGE_CURVE('',#7299,#7300,#932,.T.);
#9297=EDGE_CURVE('',#7300,#7294,#6017,.T.);
#9298=EDGE_CURVE('',#7301,#7301,#6018,.T.);
#9299=EDGE_CURVE('',#7301,#7293,#6019,.T.);
#9300=EDGE_CURVE('',#7302,#7303,#6020,.T.);
#9301=EDGE_CURVE('',#7303,#7304,#2047,.T.);
#9302=EDGE_CURVE('',#7304,#7305,#6021,.T.);
#9303=EDGE_CURVE('',#7305,#7306,#933,.T.);
#9304=EDGE_CURVE('',#7306,#7307,#934,.T.);
#9305=EDGE_CURVE('',#7307,#7308,#935,.T.);
#9306=EDGE_CURVE('',#7308,#7309,#6022,.T.);
#9307=EDGE_CURVE('',#7309,#7310,#936,.T.);
#9308=EDGE_CURVE('',#7310,#7311,#937,.T.);
#9309=EDGE_CURVE('',#7311,#7312,#6023,.T.);
#9310=EDGE_CURVE('',#7313,#7312,#2048,.T.);
#9311=EDGE_CURVE('',#7314,#7313,#6024,.T.);
#9312=EDGE_CURVE('',#7314,#7315,#938,.T.);
#9313=EDGE_CURVE('',#7315,#7316,#6025,.T.);
#9314=EDGE_CURVE('',#7316,#7317,#6026,.T.);
#9315=EDGE_CURVE('',#7317,#7318,#939,.T.);
#9316=EDGE_CURVE('',#7318,#7319,#6027,.T.);
#9317=EDGE_CURVE('',#7319,#7320,#940,.T.);
#9318=EDGE_CURVE('',#7320,#7304,#6028,.T.);
#9319=EDGE_CURVE('',#7303,#7321,#6029,.T.);
#9320=EDGE_CURVE('',#7321,#7322,#2049,.T.);
#9321=EDGE_CURVE('',#7322,#7323,#6030,.T.);
#9322=EDGE_CURVE('',#7323,#7324,#941,.T.);
#9323=EDGE_CURVE('',#7324,#7302,#2050,.T.);
#9324=EDGE_CURVE('',#7325,#7326,#771,.T.);
#9325=EDGE_CURVE('',#7326,#7327,#942,.T.);
#9326=EDGE_CURVE('',#7327,#7328,#6031,.T.);
#9327=EDGE_CURVE('',#7328,#7325,#943,.T.);
#9328=EDGE_CURVE('',#7329,#7330,#944,.T.);
#9329=EDGE_CURVE('',#7330,#7329,#945,.T.);
#9330=EDGE_CURVE('',#7331,#7331,#6032,.T.);
#9331=EDGE_CURVE('',#7331,#7277,#6033,.T.);
#9332=EDGE_CURVE('',#7332,#7333,#946,.T.);
#9333=EDGE_CURVE('',#7333,#7334,#947,.T.);
#9334=EDGE_CURVE('',#7334,#7335,#2051,.T.);
#9335=EDGE_CURVE('',#7335,#7336,#6034,.T.);
#9336=EDGE_CURVE('',#7336,#7337,#2052,.T.);
#9337=EDGE_CURVE('',#7337,#7338,#948,.T.);
#9338=EDGE_CURVE('',#7338,#7339,#949,.T.);
#9339=EDGE_CURVE('',#7339,#7332,#950,.T.);
#9340=EDGE_CURVE('',#7340,#7341,#6035,.T.);
#9341=EDGE_CURVE('',#7342,#7340,#6036,.T.);
#9342=EDGE_CURVE('',#7343,#7342,#6037,.T.);
#9343=EDGE_CURVE('',#7341,#7343,#6038,.T.);
#9344=EDGE_CURVE('',#7276,#7344,#6039,.T.);
#9345=EDGE_CURVE('',#7344,#7344,#6040,.T.);
#9346=EDGE_CURVE('',#7330,#7345,#6041,.T.);
#9347=EDGE_CURVE('',#7346,#7345,#6042,.T.);
#9348=EDGE_CURVE('',#7347,#7346,#951,.T.);
#9349=EDGE_CURVE('',#7329,#7347,#6043,.T.);
#9350=EDGE_CURVE('',#7348,#7302,#952,.T.);
#9351=EDGE_CURVE('',#7349,#7348,#6044,.T.);
#9352=EDGE_CURVE('',#7349,#7321,#6045,.T.);
#9353=EDGE_CURVE('',#7350,#7350,#6046,.T.);
#9354=EDGE_CURVE('',#7350,#7346,#2053,.T.);
#9355=EDGE_CURVE('',#7345,#7351,#953,.T.);
#9356=EDGE_CURVE('',#7351,#7347,#6047,.T.);
#9357=EDGE_CURVE('',#7352,#7353,#954,.T.);
#9358=EDGE_CURVE('',#7353,#7354,#955,.T.);
#9359=EDGE_CURVE('',#7354,#7355,#956,.T.);
#9360=EDGE_CURVE('',#7355,#7356,#2054,.T.);
#9361=EDGE_CURVE('',#7356,#7357,#6048,.T.);
#9362=EDGE_CURVE('',#7357,#7352,#2055,.T.);
#9363=EDGE_CURVE('',#7358,#7359,#957,.F.);
#9364=EDGE_CURVE('',#7360,#7358,#6049,.T.);
#9365=EDGE_CURVE('',#7360,#7361,#6050,.T.);
#9366=EDGE_CURVE('',#7359,#7361,#6051,.T.);
#9367=EDGE_CURVE('',#7362,#7362,#6052,.T.);
#9368=EDGE_CURVE('',#7362,#7363,#2056,.T.);
#9369=EDGE_CURVE('',#7363,#7363,#6053,.T.);
#9370=EDGE_CURVE('',#7364,#7365,#958,.T.);
#9371=EDGE_CURVE('',#7365,#7364,#959,.T.);
#9372=EDGE_CURVE('',#7366,#7367,#960,.T.);
#9373=EDGE_CURVE('',#7367,#7366,#961,.T.);
#9374=EDGE_CURVE('',#7326,#7368,#6054,.T.);
#9375=EDGE_CURVE('',#7369,#7368,#962,.T.);
#9376=EDGE_CURVE('',#7370,#7369,#6055,.T.);
#9377=EDGE_CURVE('',#7327,#7370,#6056,.T.);
#9378=EDGE_CURVE('',#7371,#7372,#6057,.T.);
#9379=EDGE_CURVE('',#7371,#7373,#6058,.T.);
#9380=EDGE_CURVE('',#7374,#7373,#6059,.T.);
#9381=EDGE_CURVE('',#7372,#7374,#6060,.T.);
#9382=EDGE_CURVE('',#7375,#7376,#6061,.T.);
#9383=EDGE_CURVE('',#7375,#7377,#963,.T.);
#9384=EDGE_CURVE('',#7378,#7377,#2057,.T.);
#9385=EDGE_CURVE('',#7378,#7379,#964,.T.);
#9386=EDGE_CURVE('',#7379,#7380,#6062,.T.);
#9387=EDGE_CURVE('',#7380,#7381,#965,.T.);
#9388=EDGE_CURVE('',#7381,#7382,#2058,.T.);
#9389=EDGE_CURVE('',#7382,#7376,#966,.T.);
#9390=EDGE_CURVE('',#7383,#7382,#2059,.T.);
#9391=EDGE_CURVE('',#7384,#7383,#772,.T.);
#9392=EDGE_CURVE('',#7376,#7384,#2060,.T.);
#9393=EDGE_CURVE('',#7301,#7344,#2061,.T.);
#9394=EDGE_CURVE('',#7320,#7295,#967,.T.);
#9395=EDGE_CURVE('',#7300,#7385,#968,.T.);
#9396=EDGE_CURVE('',#7385,#7305,#969,.T.);
#9397=EDGE_CURVE('',#7386,#7387,#970,.T.);
#9398=EDGE_CURVE('',#7387,#7388,#971,.T.);
#9399=EDGE_CURVE('',#7389,#7388,#972,.T.);
#9400=EDGE_CURVE('',#7390,#7389,#973,.T.);
#9401=EDGE_CURVE('',#7390,#7391,#6063,.T.);
#9402=EDGE_CURVE('',#7392,#7391,#974,.T.);
#9403=EDGE_CURVE('',#7393,#7392,#2062,.T.);
#9404=EDGE_CURVE('',#7393,#7394,#6064,.T.);
#9405=EDGE_CURVE('',#7394,#7395,#2063,.T.);
#9406=EDGE_CURVE('',#7395,#7396,#975,.T.);
#9407=EDGE_CURVE('',#7371,#7396,#976,.T.);
#9408=EDGE_CURVE('',#7386,#7372,#977,.T.);
#9409=EDGE_CURVE('',#7397,#7398,#6065,.T.);
#9410=EDGE_CURVE('',#7397,#7386,#978,.T.);
#9411=EDGE_CURVE('',#7372,#7399,#979,.T.);
#9412=EDGE_CURVE('',#7399,#7390,#980,.T.);
#9413=EDGE_CURVE('',#7389,#7398,#773,.T.);
#9414=EDGE_CURVE('',#7368,#7400,#6066,.T.);
#9415=EDGE_CURVE('',#7400,#7401,#2064,.T.);
#9416=EDGE_CURVE('',#7396,#7401,#981,.F.);
#9417=EDGE_CURVE('',#7402,#7395,#774,.T.);
#9418=EDGE_CURVE('',#7401,#7402,#982,.F.);
#9419=EDGE_CURVE('',#7400,#7370,#983,.T.);
#9420=EDGE_CURVE('',#7403,#7404,#6067,.T.);
#9421=EDGE_CURVE('',#7403,#7405,#775,.T.);
#9422=EDGE_CURVE('',#7404,#7405,#6068,.T.);
#9423=EDGE_CURVE('',#7404,#7406,#2065,.T.);
#9424=EDGE_CURVE('',#7406,#7406,#6069,.T.);
#9425=EDGE_CURVE('',#7407,#7407,#6070,.T.);
#9426=EDGE_CURVE('',#7407,#7408,#2066,.T.);
#9427=EDGE_CURVE('',#7408,#7408,#6071,.T.);
#9428=EDGE_CURVE('',#7409,#7409,#6072,.T.);
#9429=EDGE_CURVE('',#7409,#7410,#2067,.T.);
#9430=EDGE_CURVE('',#7410,#7410,#6073,.T.);
#9431=EDGE_CURVE('',#7411,#7412,#6074,.T.);
#9432=EDGE_CURVE('',#7413,#7412,#6075,.T.);
#9433=EDGE_CURVE('',#7413,#7411,#6076,.T.);
#9434=EDGE_CURVE('',#7414,#7415,#6077,.T.);
#9435=EDGE_CURVE('',#7416,#7415,#2068,.T.);
#9436=EDGE_CURVE('',#7417,#7416,#6078,.T.);
#9437=EDGE_CURVE('',#7414,#7417,#2069,.T.);
#9438=EDGE_CURVE('',#7417,#7418,#6079,.T.);
#9439=EDGE_CURVE('',#7419,#7418,#2070,.T.);
#9440=EDGE_CURVE('',#7420,#7419,#6080,.T.);
#9441=EDGE_CURVE('',#7417,#7420,#2071,.T.);
#9442=EDGE_CURVE('',#7419,#7421,#6081,.T.);
#9443=EDGE_CURVE('',#7420,#7421,#6082,.T.);
#9444=EDGE_CURVE('',#7422,#7423,#776,.T.);
#9445=EDGE_CURVE('',#7379,#7422,#2072,.T.);
#9446=EDGE_CURVE('',#7423,#7378,#2073,.T.);
#9447=EDGE_CURVE('',#7414,#7424,#6083,.T.);
#9448=EDGE_CURVE('',#7424,#7415,#6084,.T.);
#9449=EDGE_CURVE('',#7425,#7425,#6085,.T.);
#9450=EDGE_CURVE('',#7425,#7426,#2074,.T.);
#9451=EDGE_CURVE('',#7426,#7426,#6086,.T.);
#9452=EDGE_CURVE('',#7427,#7428,#984,.T.);
#9453=EDGE_CURVE('',#7428,#7429,#985,.T.);
#9454=EDGE_CURVE('',#7429,#7273,#986,.T.);
#9455=EDGE_CURVE('',#7430,#7273,#2075,.T.);
#9456=EDGE_CURVE('',#7430,#7431,#6087,.T.);
#9457=EDGE_CURVE('',#7427,#7431,#2076,.T.);
#9458=EDGE_CURVE('',#7430,#7431,#6088,.T.);
#9459=EDGE_CURVE('',#7432,#7430,#2077,.T.);
#9460=EDGE_CURVE('',#7432,#7433,#987,.T.);
#9461=EDGE_CURVE('',#7433,#7434,#988,.T.);
#9462=EDGE_CURVE('',#7431,#7434,#2078,.T.);
#9463=EDGE_CURVE('',#7435,#7435,#6089,.T.);
#9464=EDGE_CURVE('',#7435,#7367,#2079,.T.);
#9465=EDGE_CURVE('',#7365,#7436,#2080,.T.);
#9466=EDGE_CURVE('',#7436,#7436,#6090,.T.);
#9467=EDGE_CURVE('',#7437,#7341,#2081,.T.);
#9468=EDGE_CURVE('',#7437,#7438,#6091,.T.);
#9469=EDGE_CURVE('',#7438,#7340,#2082,.T.);
#9470=EDGE_CURVE('',#7439,#7439,#6092,.T.);
#9471=EDGE_CURVE('',#7439,#7440,#2083,.T.);
#9472=EDGE_CURVE('',#7440,#7440,#6093,.T.);
#9473=EDGE_CURVE('',#7334,#7441,#989,.T.);
#9474=EDGE_CURVE('',#7442,#7441,#2084,.T.);
#9475=EDGE_CURVE('',#7335,#7442,#6094,.T.);
#9476=EDGE_CURVE('',#7443,#7443,#6095,.T.);
#9477=EDGE_CURVE('',#7443,#7444,#2085,.T.);
#9478=EDGE_CURVE('',#7444,#7444,#6096,.T.);
#9479=EDGE_CURVE('',#7362,#7445,#6097,.T.);
#9480=EDGE_CURVE('',#7445,#7445,#6098,.T.);
#9481=EDGE_CURVE('',#7445,#7446,#2086,.T.);
#9482=EDGE_CURVE('',#7446,#7446,#6099,.T.);
#9483=EDGE_CURVE('',#7446,#7410,#6100,.T.);
#9484=EDGE_CURVE('',#7447,#7447,#6101,.T.);
#9485=EDGE_CURVE('',#7447,#7448,#2087,.T.);
#9486=EDGE_CURVE('',#7448,#7448,#6102,.T.);
#9487=EDGE_CURVE('',#7449,#7449,#6103,.T.);
#9488=EDGE_CURVE('',#7449,#7450,#2088,.T.);
#9489=EDGE_CURVE('',#7450,#7450,#6104,.T.);
#9490=EDGE_CURVE('',#7355,#7451,#990,.T.);
#9491=EDGE_CURVE('',#7452,#7451,#2089,.T.);
#9492=EDGE_CURVE('',#7356,#7452,#6105,.T.);
#9493=EDGE_CURVE('',#7453,#7454,#2090,.T.);
#9494=EDGE_CURVE('',#7453,#7352,#991,.T.);
#9495=EDGE_CURVE('',#7454,#7357,#6106,.T.);
#9496=EDGE_CURVE('',#7455,#7456,#2091,.T.);
#9497=EDGE_CURVE('',#7456,#7340,#2092,.T.);
#9498=EDGE_CURVE('',#7438,#7455,#2093,.T.);
#9499=EDGE_CURVE('',#7457,#7458,#2094,.T.);
#9500=EDGE_CURVE('',#7458,#7456,#6107,.T.);
#9501=EDGE_CURVE('',#7455,#7457,#6108,.T.);
#9502=EDGE_CURVE('',#7459,#7460,#6109,.T.);
#9503=EDGE_CURVE('',#7457,#7459,#2095,.T.);
#9504=EDGE_CURVE('',#7461,#7437,#2096,.T.);
#9505=EDGE_CURVE('',#7462,#7461,#6110,.T.);
#9506=EDGE_CURVE('',#7460,#7462,#2097,.T.);
#9507=EDGE_CURVE('',#7459,#7463,#2098,.T.);
#9508=EDGE_CURVE('',#7463,#7458,#2099,.T.);
#9509=EDGE_CURVE('',#7460,#7464,#2100,.T.);
#9510=EDGE_CURVE('',#7464,#7463,#6111,.T.);
#9511=EDGE_CURVE('',#7462,#7465,#2101,.T.);
#9512=EDGE_CURVE('',#7465,#7464,#2102,.T.);
#9513=EDGE_CURVE('',#7461,#7466,#2103,.T.);
#9514=EDGE_CURVE('',#7466,#7465,#6112,.T.);
#9515=EDGE_CURVE('',#7292,#7291,#2104,.T.);
#9516=EDGE_CURVE('',#7317,#7429,#6113,.T.);
#9517=EDGE_CURVE('',#7275,#7317,#992,.T.);
#9518=EDGE_CURVE('',#7272,#7432,#993,.T.);
#9519=EDGE_CURVE('',#7282,#7270,#994,.T.);
#9520=EDGE_CURVE('',#7432,#7281,#6114,.T.);
#9521=EDGE_CURVE('',#7280,#7434,#6115,.T.);
#9522=EDGE_CURVE('',#7279,#7467,#6116,.T.);
#9523=EDGE_CURVE('',#7434,#7467,#995,.T.);
#9524=EDGE_CURVE('',#7319,#7468,#6117,.T.);
#9525=EDGE_CURVE('',#7467,#7468,#996,.T.);
#9526=EDGE_CURVE('',#7319,#7279,#997,.T.);
#9527=EDGE_CURVE('',#7318,#7427,#6118,.T.);
#9528=EDGE_CURVE('',#7468,#7427,#6119,.T.);
#9529=EDGE_CURVE('',#7465,#7469,#6120,.T.);
#9530=EDGE_CURVE('',#7470,#7466,#6121,.T.);
#9531=EDGE_CURVE('',#7469,#7470,#6122,.T.);
#9532=EDGE_CURVE('',#7471,#7472,#6123,.T.);
#9533=EDGE_CURVE('',#7472,#7473,#6124,.T.);
#9534=EDGE_CURVE('',#7471,#7473,#6125,.T.);
#9535=EDGE_CURVE('',#7472,#7361,#2105,.T.);
#9536=EDGE_CURVE('',#7359,#7471,#2106,.T.);
#9537=EDGE_CURVE('',#7474,#7475,#6126,.T.);
#9538=EDGE_CURVE('',#7473,#7475,#2107,.T.);
#9539=EDGE_CURVE('',#7474,#7472,#2108,.T.);
#9540=EDGE_CURVE('',#7476,#7477,#6127,.T.);
#9541=EDGE_CURVE('',#7477,#7478,#6128,.T.);
#9542=EDGE_CURVE('',#7476,#7478,#6129,.T.);
#9543=EDGE_CURVE('',#7479,#7480,#6130,.T.);
#9544=EDGE_CURVE('',#7477,#7480,#2109,.T.);
#9545=EDGE_CURVE('',#7479,#7476,#2110,.T.);
#9546=EDGE_CURVE('',#7481,#7482,#777,.T.);
#9547=EDGE_CURVE('',#7478,#7481,#2111,.T.);
#9548=EDGE_CURVE('',#7482,#7477,#2112,.T.);
#9549=EDGE_CURVE('',#7479,#7483,#6131,.T.);
#9550=EDGE_CURVE('',#7483,#7480,#6132,.T.);
#9551=EDGE_CURVE('',#7484,#7485,#6133,.T.);
#9552=EDGE_CURVE('',#7483,#7485,#2113,.T.);
#9553=EDGE_CURVE('',#7484,#7479,#2114,.T.);
#9554=EDGE_CURVE('',#7486,#7487,#778,.T.);
#9555=EDGE_CURVE('',#7480,#7486,#2115,.T.);
#9556=EDGE_CURVE('',#7487,#7483,#2116,.T.);
#9557=EDGE_CURVE('',#7484,#7488,#6134,.T.);
#9558=EDGE_CURVE('',#7488,#7485,#6135,.T.);
#9559=EDGE_CURVE('',#7489,#7490,#779,.T.);
#9560=EDGE_CURVE('',#7488,#7489,#2117,.T.);
#9561=EDGE_CURVE('',#7490,#7484,#2118,.T.);
#9562=EDGE_CURVE('',#7491,#7414,#2119,.T.);
#9563=EDGE_CURVE('',#7491,#7492,#780,.T.);
#9564=EDGE_CURVE('',#7424,#7492,#2120,.T.);
#9565=EDGE_CURVE('',#7493,#7494,#6136,.T.);
#9566=EDGE_CURVE('',#7493,#7495,#6137,.T.);
#9567=EDGE_CURVE('',#7494,#7495,#6138,.T.);
#9568=EDGE_CURVE('',#7415,#7494,#2121,.T.);
#9569=EDGE_CURVE('',#7493,#7424,#2122,.T.);
#9570=EDGE_CURVE('',#7496,#7497,#6139,.T.);
#9571=EDGE_CURVE('',#7418,#7497,#2123,.T.);
#9572=EDGE_CURVE('',#7416,#7418,#6140,.T.);
#9573=EDGE_CURVE('',#7496,#7416,#2124,.T.);
#9574=EDGE_CURVE('',#7496,#7498,#6141,.T.);
#9575=EDGE_CURVE('',#7497,#7498,#6142,.T.);
#9576=EDGE_CURVE('',#7498,#7495,#2125,.T.);
#9577=EDGE_CURVE('',#7494,#7496,#2126,.T.);
#9578=EDGE_CURVE('',#7499,#7498,#2127,.T.);
#9579=EDGE_CURVE('',#7500,#7499,#6143,.T.);
#9580=EDGE_CURVE('',#7497,#7500,#2128,.T.);
#9581=EDGE_CURVE('',#7500,#7501,#6144,.T.);
#9582=EDGE_CURVE('',#7421,#7501,#2129,.T.);
#9583=EDGE_CURVE('',#7500,#7419,#2130,.T.);
#9584=EDGE_CURVE('',#7499,#7501,#6145,.T.);
#9585=EDGE_CURVE('',#7501,#7423,#2131,.T.);
#9586=EDGE_CURVE('',#7422,#7499,#2132,.T.);
#9587=EDGE_CURVE('',#7502,#7493,#2133,.T.);
#9588=EDGE_CURVE('',#7502,#7503,#781,.T.);
#9589=EDGE_CURVE('',#7495,#7503,#2134,.T.);
#9590=EDGE_CURVE('',#7504,#7383,#2135,.T.);
#9591=EDGE_CURVE('',#7505,#7504,#6146,.T.);
#9592=EDGE_CURVE('',#7384,#7505,#2136,.T.);
#9593=EDGE_CURVE('',#7506,#7505,#6147,.T.);
#9594=EDGE_CURVE('',#7506,#7504,#6148,.T.);
#9595=EDGE_CURVE('',#7475,#7507,#6149,.T.);
#9596=EDGE_CURVE('',#7505,#7507,#2137,.T.);
#9597=EDGE_CURVE('',#7475,#7506,#2138,.T.);
#9598=EDGE_CURVE('',#7411,#7473,#2139,.T.);
#9599=EDGE_CURVE('',#7471,#7413,#2140,.T.);
#9600=EDGE_CURVE('',#7412,#7504,#2141,.T.);
#9601=EDGE_CURVE('',#7506,#7411,#2142,.T.);
#9602=EDGE_CURVE('',#7508,#7412,#2143,.T.);
#9603=EDGE_CURVE('',#7509,#7508,#782,.T.);
#9604=EDGE_CURVE('',#7413,#7509,#2144,.T.);
#9605=EDGE_CURVE('',#7482,#7486,#2145,.T.);
#9606=EDGE_CURVE('',#7510,#7360,#2146,.T.);
#9607=EDGE_CURVE('',#7490,#7358,#2147,.T.);
#9608=EDGE_CURVE('',#7476,#7511,#2148,.T.);
#9609=EDGE_CURVE('',#7511,#7512,#2149,.T.);
#9610=EDGE_CURVE('',#7510,#7512,#6150,.T.);
#9611=EDGE_CURVE('',#7513,#7514,#2150,.T.);
#9612=EDGE_CURVE('',#7514,#7488,#2151,.T.);
#9613=EDGE_CURVE('',#7489,#7513,#2152,.T.);
#9614=EDGE_CURVE('',#7515,#7516,#2153,.T.);
#9615=EDGE_CURVE('',#7516,#7517,#6151,.T.);
#9616=EDGE_CURVE('',#7518,#7517,#2154,.T.);
#9617=EDGE_CURVE('',#7518,#7519,#783,.T.);
#9618=EDGE_CURVE('',#7487,#7519,#2155,.T.);
#9619=EDGE_CURVE('',#7485,#7515,#2156,.T.);
#9620=EDGE_CURVE('',#7451,#7520,#6152,.T.);
#9621=EDGE_CURVE('',#7520,#7521,#784,.T.);
#9622=EDGE_CURVE('',#7521,#7522,#2157,.T.);
#9623=EDGE_CURVE('',#7522,#7452,#2158,.T.);
#9624=EDGE_CURVE('',#7388,#7523,#998,.T.);
#9625=EDGE_CURVE('',#7387,#7523,#6153,.T.);
#9626=EDGE_CURVE('',#7393,#7524,#2159,.T.);
#9627=EDGE_CURVE('',#7524,#7525,#2160,.T.);
#9628=EDGE_CURVE('',#7394,#7525,#2161,.T.);
#9629=EDGE_CURVE('',#7403,#7398,#2162,.T.);
#9630=EDGE_CURVE('',#7526,#7405,#2163,.T.);
#9631=EDGE_CURVE('',#7397,#7526,#785,.T.);
#9632=EDGE_CURVE('',#7523,#7389,#786,.T.);
#9633=EDGE_CURVE('',#7526,#7387,#6154,.T.);
#9634=EDGE_CURVE('',#7390,#7527,#6155,.T.);
#9635=EDGE_CURVE('',#7528,#7527,#6156,.T.);
#9636=EDGE_CURVE('',#7391,#7528,#6157,.T.);
#9637=EDGE_CURVE('',#7399,#7374,#999,.T.);
#9638=EDGE_CURVE('',#7441,#7529,#787,.T.);
#9639=EDGE_CURVE('',#7529,#7453,#1000,.T.);
#9640=EDGE_CURVE('',#7454,#7442,#2164,.T.);
#9641=EDGE_CURVE('',#7296,#7271,#1001,.T.);
#9642=EDGE_CURVE('',#7316,#7297,#1002,.T.);
#9643=EDGE_CURVE('',#7522,#7336,#6158,.T.);
#9644=EDGE_CURVE('',#7512,#7530,#6159,.T.);
#9645=EDGE_CURVE('',#7531,#7530,#6160,.T.);
#9646=EDGE_CURVE('',#7510,#7531,#6161,.T.);
#9647=EDGE_CURVE('',#7507,#7530,#2165,.T.);
#9648=EDGE_CURVE('',#7474,#7507,#6162,.T.);
#9649=EDGE_CURVE('',#7531,#7474,#2166,.T.);
#9650=EDGE_CURVE('',#7361,#7531,#2167,.T.);
#9651=EDGE_CURVE('',#7381,#7508,#2168,.T.);
#9652=EDGE_CURVE('',#7508,#7383,#2169,.T.);
#9653=EDGE_CURVE('',#7532,#7421,#2170,.T.);
#9654=EDGE_CURVE('',#7533,#7532,#788,.T.);
#9655=EDGE_CURVE('',#7420,#7533,#2171,.T.);
#9656=EDGE_CURVE('',#7377,#7532,#2172,.T.);
#9657=EDGE_CURVE('',#7533,#7375,#2173,.T.);
#9658=EDGE_CURVE('',#7373,#7534,#1003,.T.);
#9659=EDGE_CURVE('',#7534,#7528,#1004,.T.);
#9660=EDGE_CURVE('',#7527,#7399,#1005,.T.);
#9661=EDGE_CURVE('',#7391,#7534,#1006,.T.);
#9662=EDGE_CURVE('',#7534,#7371,#1007,.T.);
#9663=EDGE_CURVE('',#7402,#7535,#2174,.T.);
#9664=EDGE_CURVE('',#7535,#7536,#1008,.T.);
#9665=EDGE_CURVE('',#7392,#7536,#2175,.T.);
#9666=EDGE_CURVE('',#7521,#7337,#1009,.T.);
#9667=EDGE_CURVE('',#7311,#7535,#789,.T.);
#9668=EDGE_CURVE('',#7298,#7309,#1010,.T.);
#9669=EDGE_CURVE('',#7536,#7314,#790,.T.);
#9670=EDGE_CURVE('',#7524,#7313,#2176,.T.);
#9671=EDGE_CURVE('',#7525,#7312,#2177,.T.);
#9672=EDGE_CURVE('',#7537,#7478,#2178,.T.);
#9673=EDGE_CURVE('',#7511,#7537,#791,.T.);
#9674=EDGE_CURVE('',#7511,#7538,#6163,.T.);
#9675=EDGE_CURVE('',#7530,#7538,#2179,.T.);
#9676=EDGE_CURVE('',#7539,#7537,#1011,.T.);
#9677=EDGE_CURVE('',#7538,#7539,#792,.T.);
#9678=EDGE_CURVE('',#7509,#7380,#2180,.T.);
#9679=EDGE_CURVE('',#7540,#7503,#2181,.T.);
#9680=EDGE_CURVE('',#7513,#7540,#2182,.T.);
#9681=EDGE_CURVE('',#7541,#7469,#2183,.T.);
#9682=EDGE_CURVE('',#7470,#7518,#2184,.T.);
#9683=EDGE_CURVE('',#7517,#7349,#2185,.T.);
#9684=EDGE_CURVE('',#7348,#7542,#6164,.T.);
#9685=EDGE_CURVE('',#7542,#7543,#2186,.T.);
#9686=EDGE_CURVE('',#7543,#7343,#2187,.T.);
#9687=EDGE_CURVE('',#7342,#7544,#2188,.T.);
#9688=EDGE_CURVE('',#7544,#7545,#6165,.T.);
#9689=EDGE_CURVE('',#7545,#7546,#2189,.T.);
#9690=EDGE_CURVE('',#7546,#7541,#6166,.T.);
#9691=EDGE_CURVE('',#7542,#7547,#2190,.T.);
#9692=EDGE_CURVE('',#7547,#7502,#2191,.T.);
#9693=EDGE_CURVE('',#7492,#7548,#2192,.T.);
#9694=EDGE_CURVE('',#7548,#7543,#6167,.T.);
#9695=EDGE_CURVE('',#7423,#7532,#2193,.T.);
#9696=EDGE_CURVE('',#7503,#7549,#2194,.T.);
#9697=EDGE_CURVE('',#7549,#7550,#6168,.T.);
#9698=EDGE_CURVE('',#7540,#7550,#2195,.T.);
#9699=EDGE_CURVE('',#7519,#7466,#2196,.T.);
#9700=EDGE_CURVE('',#7341,#7551,#2197,.T.);
#9701=EDGE_CURVE('',#7551,#7481,#2198,.T.);
#9702=EDGE_CURVE('',#7550,#7552,#1012,.T.);
#9703=EDGE_CURVE('',#7552,#7553,#2199,.T.);
#9704=EDGE_CURVE('',#7553,#7516,#2200,.T.);
#9705=EDGE_CURVE('',#7515,#7514,#6169,.T.);
#9706=EDGE_CURVE('',#7332,#7554,#1013,.T.);
#9707=EDGE_CURVE('',#7308,#7554,#1014,.T.);
#9708=EDGE_CURVE('',#7307,#7529,#1015,.T.);
#9709=EDGE_CURVE('',#7385,#7339,#1016,.T.);
#9710=EDGE_CURVE('',#7520,#7306,#1017,.T.);
#9711=EDGE_CURVE('',#7349,#7553,#6170,.T.);
#9712=EDGE_CURVE('',#7321,#7553,#6171,.T.);
#9713=EDGE_CURVE('',#7322,#7552,#1018,.T.);
#9714=EDGE_CURVE('',#7323,#7549,#6172,.T.);
#9715=EDGE_CURVE('',#7547,#7549,#1019,.T.);
#9716=EDGE_CURVE('',#7547,#7324,#6173,.T.);
#9717=EDGE_CURVE('',#7555,#7491,#2201,.T.);
#9718=EDGE_CURVE('',#7555,#7548,#1020,.T.);
#9719=EDGE_CURVE('',#7551,#7555,#793,.T.);
#9720=EDGE_CURVE('',#7464,#7541,#6174,.T.);
#9721=EDGE_CURVE('',#7463,#7546,#6175,.T.);
#9722=EDGE_CURVE('',#7458,#7545,#6176,.T.);
#9723=EDGE_CURVE('',#7456,#7544,#6177,.T.);
#9724=EDGE_CURVE('',#7554,#7299,#1021,.T.);
#9725=EDGE_CURVE('',#7290,#7320,#6178,.T.);
#9726=EDGE_CURVE('',#7289,#7295,#6179,.T.);
#9727=EDGE_CURVE('',#7287,#7556,#1022,.T.);
#9728=EDGE_CURVE('',#7557,#7286,#1023,.T.);
#9729=EDGE_CURVE('',#7556,#7557,#6180,.T.);
#9730=EDGE_CURVE('',#7556,#7557,#2202,.T.);
#9731=EDGE_CURVE('',#7558,#7539,#2203,.T.);
#9732=EDGE_CURVE('',#7558,#7559,#794,.T.);
#9733=EDGE_CURVE('',#7491,#7559,#2204,.T.);
#9734=EDGE_CURVE('',#7558,#7559,#6181,.T.);
#13113=ORIENTED_EDGE('',*,*,#9263,.F.);
#13114=ORIENTED_EDGE('',*,*,#9264,.F.);
#13115=ORIENTED_EDGE('',*,*,#9265,.F.);
#13116=ORIENTED_EDGE('',*,*,#9266,.F.);
#13117=ORIENTED_EDGE('',*,*,#9267,.F.);
#13118=ORIENTED_EDGE('',*,*,#9268,.F.);
#13119=ORIENTED_EDGE('',*,*,#9269,.T.);
#13120=ORIENTED_EDGE('',*,*,#9270,.T.);
#13121=ORIENTED_EDGE('',*,*,#9271,.T.);
#13122=ORIENTED_EDGE('',*,*,#9270,.F.);
#13123=ORIENTED_EDGE('',*,*,#9272,.T.);
#13124=ORIENTED_EDGE('',*,*,#9273,.T.);
#13125=ORIENTED_EDGE('',*,*,#9274,.T.);
#13126=ORIENTED_EDGE('',*,*,#9275,.T.);
#13127=ORIENTED_EDGE('',*,*,#9276,.T.);
#13128=ORIENTED_EDGE('',*,*,#9277,.T.);
#13129=ORIENTED_EDGE('',*,*,#9278,.T.);
#13130=ORIENTED_EDGE('',*,*,#9279,.T.);
#13131=ORIENTED_EDGE('',*,*,#9280,.T.);
#13132=ORIENTED_EDGE('',*,*,#9281,.T.);
#13133=ORIENTED_EDGE('',*,*,#9282,.T.);
#13134=ORIENTED_EDGE('',*,*,#9277,.F.);
#13135=ORIENTED_EDGE('',*,*,#9283,.T.);
#13136=ORIENTED_EDGE('',*,*,#9284,.T.);
#13137=ORIENTED_EDGE('',*,*,#9285,.T.);
#13138=ORIENTED_EDGE('',*,*,#9286,.F.);
#13139=ORIENTED_EDGE('',*,*,#9287,.F.);
#13140=ORIENTED_EDGE('',*,*,#9278,.F.);
#13141=ORIENTED_EDGE('',*,*,#9282,.F.);
#13142=ORIENTED_EDGE('',*,*,#9288,.F.);
#13143=ORIENTED_EDGE('',*,*,#9289,.T.);
#13144=ORIENTED_EDGE('',*,*,#9290,.T.);
#13145=ORIENTED_EDGE('',*,*,#9291,.T.);
#13146=ORIENTED_EDGE('',*,*,#9292,.T.);
#13147=ORIENTED_EDGE('',*,*,#9293,.T.);
#13148=ORIENTED_EDGE('',*,*,#9294,.T.);
#13149=ORIENTED_EDGE('',*,*,#9295,.T.);
#13150=ORIENTED_EDGE('',*,*,#9296,.T.);
#13151=ORIENTED_EDGE('',*,*,#9297,.T.);
#13152=ORIENTED_EDGE('',*,*,#9290,.F.);
#13153=ORIENTED_EDGE('',*,*,#9298,.F.);
#13154=ORIENTED_EDGE('',*,*,#9299,.T.);
#13155=ORIENTED_EDGE('',*,*,#9289,.F.);
#13156=ORIENTED_EDGE('',*,*,#9299,.F.);
#13157=ORIENTED_EDGE('',*,*,#9300,.T.);
#13158=ORIENTED_EDGE('',*,*,#9301,.T.);
#13159=ORIENTED_EDGE('',*,*,#9302,.T.);
#13160=ORIENTED_EDGE('',*,*,#9303,.T.);
#13161=ORIENTED_EDGE('',*,*,#9304,.T.);
#13162=ORIENTED_EDGE('',*,*,#9305,.T.);
#13163=ORIENTED_EDGE('',*,*,#9306,.T.);
#13164=ORIENTED_EDGE('',*,*,#9307,.T.);
#13165=ORIENTED_EDGE('',*,*,#9308,.T.);
#13166=ORIENTED_EDGE('',*,*,#9309,.T.);
#13167=ORIENTED_EDGE('',*,*,#9310,.F.);
#13168=ORIENTED_EDGE('',*,*,#9311,.F.);
#13169=ORIENTED_EDGE('',*,*,#9312,.T.);
#13170=ORIENTED_EDGE('',*,*,#9313,.T.);
#13171=ORIENTED_EDGE('',*,*,#9314,.T.);
#13172=ORIENTED_EDGE('',*,*,#9315,.T.);
#13173=ORIENTED_EDGE('',*,*,#9316,.T.);
#13174=ORIENTED_EDGE('',*,*,#9317,.T.);
#13175=ORIENTED_EDGE('',*,*,#9318,.T.);
#13176=ORIENTED_EDGE('',*,*,#9301,.F.);
#13177=ORIENTED_EDGE('',*,*,#9319,.T.);
#13178=ORIENTED_EDGE('',*,*,#9320,.T.);
#13179=ORIENTED_EDGE('',*,*,#9321,.T.);
#13180=ORIENTED_EDGE('',*,*,#9322,.T.);
#13181=ORIENTED_EDGE('',*,*,#9323,.T.);
#13182=ORIENTED_EDGE('',*,*,#9324,.T.);
#13183=ORIENTED_EDGE('',*,*,#9325,.T.);
#13184=ORIENTED_EDGE('',*,*,#9326,.T.);
#13185=ORIENTED_EDGE('',*,*,#9327,.T.);
#13186=ORIENTED_EDGE('',*,*,#9328,.T.);
#13187=ORIENTED_EDGE('',*,*,#9329,.T.);
#13188=ORIENTED_EDGE('',*,*,#9330,.T.);
#13189=ORIENTED_EDGE('',*,*,#9331,.T.);
#13190=ORIENTED_EDGE('',*,*,#9271,.F.);
#13191=ORIENTED_EDGE('',*,*,#9331,.F.);
#13192=ORIENTED_EDGE('',*,*,#9332,.T.);
#13193=ORIENTED_EDGE('',*,*,#9333,.T.);
#13194=ORIENTED_EDGE('',*,*,#9334,.T.);
#13195=ORIENTED_EDGE('',*,*,#9335,.T.);
#13196=ORIENTED_EDGE('',*,*,#9336,.T.);
#13197=ORIENTED_EDGE('',*,*,#9337,.T.);
#13198=ORIENTED_EDGE('',*,*,#9338,.T.);
#13199=ORIENTED_EDGE('',*,*,#9339,.T.);
#13200=ORIENTED_EDGE('',*,*,#9340,.F.);
#13201=ORIENTED_EDGE('',*,*,#9341,.F.);
#13202=ORIENTED_EDGE('',*,*,#9342,.F.);
#13203=ORIENTED_EDGE('',*,*,#9343,.F.);
#13204=ORIENTED_EDGE('',*,*,#9269,.F.);
#13205=ORIENTED_EDGE('',*,*,#9344,.T.);
#13206=ORIENTED_EDGE('',*,*,#9345,.F.);
#13207=ORIENTED_EDGE('',*,*,#9344,.F.);
#13208=ORIENTED_EDGE('',*,*,#9329,.F.);
#13209=ORIENTED_EDGE('',*,*,#9346,.T.);
#13210=ORIENTED_EDGE('',*,*,#9347,.F.);
#13211=ORIENTED_EDGE('',*,*,#9348,.F.);
#13212=ORIENTED_EDGE('',*,*,#9349,.F.);
#13213=ORIENTED_EDGE('',*,*,#9300,.F.);
#13214=ORIENTED_EDGE('',*,*,#9350,.F.);
#13215=ORIENTED_EDGE('',*,*,#9351,.F.);
#13216=ORIENTED_EDGE('',*,*,#9352,.T.);
#13217=ORIENTED_EDGE('',*,*,#9319,.F.);
#13218=ORIENTED_EDGE('',*,*,#9353,.F.);
#13219=ORIENTED_EDGE('',*,*,#9354,.T.);
#13220=ORIENTED_EDGE('',*,*,#9347,.T.);
#13221=ORIENTED_EDGE('',*,*,#9355,.T.);
#13222=ORIENTED_EDGE('',*,*,#9356,.T.);
#13223=ORIENTED_EDGE('',*,*,#9348,.T.);
#13224=ORIENTED_EDGE('',*,*,#9354,.F.);
#13225=ORIENTED_EDGE('',*,*,#9357,.T.);
#13226=ORIENTED_EDGE('',*,*,#9358,.T.);
#13227=ORIENTED_EDGE('',*,*,#9359,.T.);
#13228=ORIENTED_EDGE('',*,*,#9360,.T.);
#13229=ORIENTED_EDGE('',*,*,#9361,.T.);
#13230=ORIENTED_EDGE('',*,*,#9362,.T.);
#13231=ORIENTED_EDGE('',*,*,#9363,.F.);
#13232=ORIENTED_EDGE('',*,*,#9364,.F.);
#13233=ORIENTED_EDGE('',*,*,#9365,.T.);
#13234=ORIENTED_EDGE('',*,*,#9366,.F.);
#13235=ORIENTED_EDGE('',*,*,#9367,.T.);
#13236=ORIENTED_EDGE('',*,*,#9368,.T.);
#13237=ORIENTED_EDGE('',*,*,#9369,.F.);
#13238=ORIENTED_EDGE('',*,*,#9368,.F.);
#13239=ORIENTED_EDGE('',*,*,#9370,.T.);
#13240=ORIENTED_EDGE('',*,*,#9371,.T.);
#13241=ORIENTED_EDGE('',*,*,#9372,.T.);
#13242=ORIENTED_EDGE('',*,*,#9373,.T.);
#13243=ORIENTED_EDGE('',*,*,#9325,.F.);
#13244=ORIENTED_EDGE('',*,*,#9374,.T.);
#13245=ORIENTED_EDGE('',*,*,#9375,.F.);
#13246=ORIENTED_EDGE('',*,*,#9376,.F.);
#13247=ORIENTED_EDGE('',*,*,#9377,.F.);
#13248=ORIENTED_EDGE('',*,*,#9378,.F.);
#13249=ORIENTED_EDGE('',*,*,#9379,.T.);
#13250=ORIENTED_EDGE('',*,*,#9380,.F.);
#13251=ORIENTED_EDGE('',*,*,#9381,.F.);
#13252=ORIENTED_EDGE('',*,*,#9382,.F.);
#13253=ORIENTED_EDGE('',*,*,#9383,.T.);
#13254=ORIENTED_EDGE('',*,*,#9384,.F.);
#13255=ORIENTED_EDGE('',*,*,#9385,.T.);
#13256=ORIENTED_EDGE('',*,*,#9386,.T.);
#13257=ORIENTED_EDGE('',*,*,#9387,.T.);
#13258=ORIENTED_EDGE('',*,*,#9388,.T.);
#13259=ORIENTED_EDGE('',*,*,#9389,.T.);
#13260=ORIENTED_EDGE('',*,*,#9389,.F.);
#13261=ORIENTED_EDGE('',*,*,#9390,.F.);
#13262=ORIENTED_EDGE('',*,*,#9391,.F.);
#13263=ORIENTED_EDGE('',*,*,#9392,.F.);
#13264=ORIENTED_EDGE('',*,*,#9298,.T.);
#13265=ORIENTED_EDGE('',*,*,#9393,.T.);
#13266=ORIENTED_EDGE('',*,*,#9345,.T.);
#13267=ORIENTED_EDGE('',*,*,#9393,.F.);
#13268=ORIENTED_EDGE('',*,*,#9318,.F.);
#13269=ORIENTED_EDGE('',*,*,#9394,.T.);
#13270=ORIENTED_EDGE('',*,*,#9291,.F.);
#13271=ORIENTED_EDGE('',*,*,#9297,.F.);
#13272=ORIENTED_EDGE('',*,*,#9395,.T.);
#13273=ORIENTED_EDGE('',*,*,#9396,.T.);
#13274=ORIENTED_EDGE('',*,*,#9302,.F.);
#13275=ORIENTED_EDGE('',*,*,#9397,.T.);
#13276=ORIENTED_EDGE('',*,*,#9398,.T.);
#13277=ORIENTED_EDGE('',*,*,#9399,.F.);
#13278=ORIENTED_EDGE('',*,*,#9400,.F.);
#13279=ORIENTED_EDGE('',*,*,#9401,.T.);
#13280=ORIENTED_EDGE('',*,*,#9402,.F.);
#13281=ORIENTED_EDGE('',*,*,#9403,.F.);
#13282=ORIENTED_EDGE('',*,*,#9404,.T.);
#13283=ORIENTED_EDGE('',*,*,#9405,.T.);
#13284=ORIENTED_EDGE('',*,*,#9406,.T.);
#13285=ORIENTED_EDGE('',*,*,#9407,.F.);
#13286=ORIENTED_EDGE('',*,*,#9378,.T.);
#13287=ORIENTED_EDGE('',*,*,#9408,.F.);
#13288=ORIENTED_EDGE('',*,*,#9409,.F.);
#13289=ORIENTED_EDGE('',*,*,#9410,.T.);
#13290=ORIENTED_EDGE('',*,*,#9408,.T.);
#13291=ORIENTED_EDGE('',*,*,#9411,.T.);
#13292=ORIENTED_EDGE('',*,*,#9412,.T.);
#13293=ORIENTED_EDGE('',*,*,#9400,.T.);
#13294=ORIENTED_EDGE('',*,*,#9413,.T.);
#13295=ORIENTED_EDGE('',*,*,#9375,.T.);
#13296=ORIENTED_EDGE('',*,*,#9414,.T.);
#13297=ORIENTED_EDGE('',*,*,#9415,.T.);
#13298=ORIENTED_EDGE('',*,*,#9416,.F.);
#13299=ORIENTED_EDGE('',*,*,#9406,.F.);
#13300=ORIENTED_EDGE('',*,*,#9417,.F.);
#13301=ORIENTED_EDGE('',*,*,#9418,.F.);
#13302=ORIENTED_EDGE('',*,*,#9415,.F.);
#13303=ORIENTED_EDGE('',*,*,#9419,.T.);
#13304=ORIENTED_EDGE('',*,*,#9376,.T.);
#13305=ORIENTED_EDGE('',*,*,#9420,.F.);
#13306=ORIENTED_EDGE('',*,*,#9421,.T.);
#13307=ORIENTED_EDGE('',*,*,#9422,.F.);
#13308=ORIENTED_EDGE('',*,*,#9423,.T.);
#13309=ORIENTED_EDGE('',*,*,#9424,.T.);
#13310=ORIENTED_EDGE('',*,*,#9423,.F.);
#13311=ORIENTED_EDGE('',*,*,#9425,.T.);
#13312=ORIENTED_EDGE('',*,*,#9426,.T.);
#13313=ORIENTED_EDGE('',*,*,#9427,.F.);
#13314=ORIENTED_EDGE('',*,*,#9426,.F.);
#13315=ORIENTED_EDGE('',*,*,#9428,.T.);
#13316=ORIENTED_EDGE('',*,*,#9429,.T.);
#13317=ORIENTED_EDGE('',*,*,#9430,.F.);
#13318=ORIENTED_EDGE('',*,*,#9429,.F.);
#13319=ORIENTED_EDGE('',*,*,#9431,.T.);
#13320=ORIENTED_EDGE('',*,*,#9432,.F.);
#13321=ORIENTED_EDGE('',*,*,#9433,.T.);
#13322=ORIENTED_EDGE('',*,*,#9434,.T.);
#13323=ORIENTED_EDGE('',*,*,#9435,.F.);
#13324=ORIENTED_EDGE('',*,*,#9436,.F.);
#13325=ORIENTED_EDGE('',*,*,#9437,.F.);
#13326=ORIENTED_EDGE('',*,*,#9438,.T.);
#13327=ORIENTED_EDGE('',*,*,#9439,.F.);
#13328=ORIENTED_EDGE('',*,*,#9440,.F.);
#13329=ORIENTED_EDGE('',*,*,#9441,.F.);
#13330=ORIENTED_EDGE('',*,*,#9440,.T.);
#13331=ORIENTED_EDGE('',*,*,#9442,.T.);
#13332=ORIENTED_EDGE('',*,*,#9443,.F.);
#13333=ORIENTED_EDGE('',*,*,#9444,.F.);
#13334=ORIENTED_EDGE('',*,*,#9445,.F.);
#13335=ORIENTED_EDGE('',*,*,#9385,.F.);
#13336=ORIENTED_EDGE('',*,*,#9446,.F.);
#13337=ORIENTED_EDGE('',*,*,#9434,.F.);
#13338=ORIENTED_EDGE('',*,*,#9447,.T.);
#13339=ORIENTED_EDGE('',*,*,#9448,.T.);
#13340=ORIENTED_EDGE('',*,*,#9449,.F.);
#13341=ORIENTED_EDGE('',*,*,#9450,.T.);
#13342=ORIENTED_EDGE('',*,*,#9451,.F.);
#13343=ORIENTED_EDGE('',*,*,#9450,.F.);
#13344=ORIENTED_EDGE('',*,*,#9452,.T.);
#13345=ORIENTED_EDGE('',*,*,#9453,.T.);
#13346=ORIENTED_EDGE('',*,*,#9454,.T.);
#13347=ORIENTED_EDGE('',*,*,#9455,.F.);
#13348=ORIENTED_EDGE('',*,*,#9456,.T.);
#13349=ORIENTED_EDGE('',*,*,#9457,.F.);
#13350=ORIENTED_EDGE('',*,*,#9458,.F.);
#13351=ORIENTED_EDGE('',*,*,#9459,.F.);
#13352=ORIENTED_EDGE('',*,*,#9460,.T.);
#13353=ORIENTED_EDGE('',*,*,#9461,.T.);
#13354=ORIENTED_EDGE('',*,*,#9462,.F.);
#13355=ORIENTED_EDGE('',*,*,#9463,.F.);
#13356=ORIENTED_EDGE('',*,*,#9464,.T.);
#13357=ORIENTED_EDGE('',*,*,#9372,.F.);
#13358=ORIENTED_EDGE('',*,*,#9373,.F.);
#13359=ORIENTED_EDGE('',*,*,#9464,.F.);
#13360=ORIENTED_EDGE('',*,*,#9370,.F.);
#13361=ORIENTED_EDGE('',*,*,#9371,.F.);
#13362=ORIENTED_EDGE('',*,*,#9465,.T.);
#13363=ORIENTED_EDGE('',*,*,#9466,.T.);
#13364=ORIENTED_EDGE('',*,*,#9465,.F.);
#13365=ORIENTED_EDGE('',*,*,#9340,.T.);
#13366=ORIENTED_EDGE('',*,*,#9467,.F.);
#13367=ORIENTED_EDGE('',*,*,#9468,.T.);
#13368=ORIENTED_EDGE('',*,*,#9469,.T.);
#13369=ORIENTED_EDGE('',*,*,#9470,.T.);
#13370=ORIENTED_EDGE('',*,*,#9471,.T.);
#13371=ORIENTED_EDGE('',*,*,#9472,.F.);
#13372=ORIENTED_EDGE('',*,*,#9471,.F.);
#13373=ORIENTED_EDGE('',*,*,#9473,.T.);
#13374=ORIENTED_EDGE('',*,*,#9474,.F.);
#13375=ORIENTED_EDGE('',*,*,#9475,.F.);
#13376=ORIENTED_EDGE('',*,*,#9334,.F.);
#13377=ORIENTED_EDGE('',*,*,#9476,.F.);
#13378=ORIENTED_EDGE('',*,*,#9477,.T.);
#13379=ORIENTED_EDGE('',*,*,#9478,.F.);
#13380=ORIENTED_EDGE('',*,*,#9477,.F.);
#13381=ORIENTED_EDGE('',*,*,#9367,.F.);
#13382=ORIENTED_EDGE('',*,*,#9479,.T.);
#13383=ORIENTED_EDGE('',*,*,#9480,.T.);
#13384=ORIENTED_EDGE('',*,*,#9479,.F.);
#13385=ORIENTED_EDGE('',*,*,#9480,.F.);
#13386=ORIENTED_EDGE('',*,*,#9481,.T.);
#13387=ORIENTED_EDGE('',*,*,#9482,.T.);
#13388=ORIENTED_EDGE('',*,*,#9481,.F.);
#13389=ORIENTED_EDGE('',*,*,#9482,.F.);
#13390=ORIENTED_EDGE('',*,*,#9483,.T.);
#13391=ORIENTED_EDGE('',*,*,#9430,.T.);
#13392=ORIENTED_EDGE('',*,*,#9483,.F.);
#13393=ORIENTED_EDGE('',*,*,#9484,.T.);
#13394=ORIENTED_EDGE('',*,*,#9485,.T.);
#13395=ORIENTED_EDGE('',*,*,#9486,.F.);
#13396=ORIENTED_EDGE('',*,*,#9485,.F.);
#13397=ORIENTED_EDGE('',*,*,#9487,.F.);
#13398=ORIENTED_EDGE('',*,*,#9488,.T.);
#13399=ORIENTED_EDGE('',*,*,#9489,.T.);
#13400=ORIENTED_EDGE('',*,*,#9488,.F.);
#13401=ORIENTED_EDGE('',*,*,#9424,.F.);
#13402=ORIENTED_EDGE('',*,*,#9489,.F.);
#13403=ORIENTED_EDGE('',*,*,#9476,.T.);
#13404=ORIENTED_EDGE('',*,*,#9360,.F.);
#13405=ORIENTED_EDGE('',*,*,#9490,.T.);
#13406=ORIENTED_EDGE('',*,*,#9491,.F.);
#13407=ORIENTED_EDGE('',*,*,#9492,.F.);
#13408=ORIENTED_EDGE('',*,*,#9493,.F.);
#13409=ORIENTED_EDGE('',*,*,#9494,.T.);
#13410=ORIENTED_EDGE('',*,*,#9362,.F.);
#13411=ORIENTED_EDGE('',*,*,#9495,.F.);
#13412=ORIENTED_EDGE('',*,*,#9496,.T.);
#13413=ORIENTED_EDGE('',*,*,#9497,.T.);
#13414=ORIENTED_EDGE('',*,*,#9469,.F.);
#13415=ORIENTED_EDGE('',*,*,#9498,.T.);
#13416=ORIENTED_EDGE('',*,*,#9499,.T.);
#13417=ORIENTED_EDGE('',*,*,#9500,.T.);
#13418=ORIENTED_EDGE('',*,*,#9496,.F.);
#13419=ORIENTED_EDGE('',*,*,#9501,.T.);
#13420=ORIENTED_EDGE('',*,*,#9502,.F.);
#13421=ORIENTED_EDGE('',*,*,#9503,.F.);
#13422=ORIENTED_EDGE('',*,*,#9501,.F.);
#13423=ORIENTED_EDGE('',*,*,#9498,.F.);
#13424=ORIENTED_EDGE('',*,*,#9468,.F.);
#13425=ORIENTED_EDGE('',*,*,#9504,.F.);
#13426=ORIENTED_EDGE('',*,*,#9505,.F.);
#13427=ORIENTED_EDGE('',*,*,#9506,.F.);
#13428=ORIENTED_EDGE('',*,*,#9486,.T.);
#13429=ORIENTED_EDGE('',*,*,#9472,.T.);
#13430=ORIENTED_EDGE('',*,*,#9369,.T.);
#13431=ORIENTED_EDGE('',*,*,#9507,.T.);
#13432=ORIENTED_EDGE('',*,*,#9508,.T.);
#13433=ORIENTED_EDGE('',*,*,#9499,.F.);
#13434=ORIENTED_EDGE('',*,*,#9503,.T.);
#13435=ORIENTED_EDGE('',*,*,#9509,.T.);
#13436=ORIENTED_EDGE('',*,*,#9510,.T.);
#13437=ORIENTED_EDGE('',*,*,#9507,.F.);
#13438=ORIENTED_EDGE('',*,*,#9502,.T.);
#13439=ORIENTED_EDGE('',*,*,#9511,.T.);
#13440=ORIENTED_EDGE('',*,*,#9512,.T.);
#13441=ORIENTED_EDGE('',*,*,#9509,.F.);
#13442=ORIENTED_EDGE('',*,*,#9506,.T.);
#13443=ORIENTED_EDGE('',*,*,#9513,.T.);
#13444=ORIENTED_EDGE('',*,*,#9514,.T.);
#13445=ORIENTED_EDGE('',*,*,#9511,.F.);
#13446=ORIENTED_EDGE('',*,*,#9505,.T.);
#13447=ORIENTED_EDGE('',*,*,#9515,.T.);
#13448=ORIENTED_EDGE('',*,*,#9286,.T.);
#13449=ORIENTED_EDGE('',*,*,#9516,.F.);
#13450=ORIENTED_EDGE('',*,*,#9517,.F.);
#13451=ORIENTED_EDGE('',*,*,#9267,.T.);
#13452=ORIENTED_EDGE('',*,*,#9266,.T.);
#13453=ORIENTED_EDGE('',*,*,#9454,.F.);
#13454=ORIENTED_EDGE('',*,*,#9518,.F.);
#13455=ORIENTED_EDGE('',*,*,#9264,.T.);
#13456=ORIENTED_EDGE('',*,*,#9519,.F.);
#13457=ORIENTED_EDGE('',*,*,#9275,.F.);
#13458=ORIENTED_EDGE('',*,*,#9520,.F.);
#13459=ORIENTED_EDGE('',*,*,#9460,.F.);
#13460=ORIENTED_EDGE('',*,*,#9520,.T.);
#13461=ORIENTED_EDGE('',*,*,#9274,.F.);
#13462=ORIENTED_EDGE('',*,*,#9521,.T.);
#13463=ORIENTED_EDGE('',*,*,#9461,.F.);
#13464=ORIENTED_EDGE('',*,*,#9522,.T.);
#13465=ORIENTED_EDGE('',*,*,#9523,.F.);
#13466=ORIENTED_EDGE('',*,*,#9521,.F.);
#13467=ORIENTED_EDGE('',*,*,#9273,.F.);
#13468=ORIENTED_EDGE('',*,*,#9524,.T.);
#13469=ORIENTED_EDGE('',*,*,#9525,.F.);
#13470=ORIENTED_EDGE('',*,*,#9522,.F.);
#13471=ORIENTED_EDGE('',*,*,#9526,.F.);
#13472=ORIENTED_EDGE('',*,*,#9527,.T.);
#13473=ORIENTED_EDGE('',*,*,#9528,.F.);
#13474=ORIENTED_EDGE('',*,*,#9524,.F.);
#13475=ORIENTED_EDGE('',*,*,#9316,.F.);
#13476=ORIENTED_EDGE('',*,*,#9315,.F.);
#13477=ORIENTED_EDGE('',*,*,#9516,.T.);
#13478=ORIENTED_EDGE('',*,*,#9453,.F.);
#13479=ORIENTED_EDGE('',*,*,#9452,.F.);
#13480=ORIENTED_EDGE('',*,*,#9527,.F.);
#13481=ORIENTED_EDGE('',*,*,#9456,.F.);
#13482=ORIENTED_EDGE('',*,*,#9458,.T.);
#13483=ORIENTED_EDGE('',*,*,#9449,.T.);
#13484=ORIENTED_EDGE('',*,*,#9529,.F.);
#13485=ORIENTED_EDGE('',*,*,#9514,.F.);
#13486=ORIENTED_EDGE('',*,*,#9530,.F.);
#13487=ORIENTED_EDGE('',*,*,#9531,.F.);
#13488=ORIENTED_EDGE('',*,*,#9532,.T.);
#13489=ORIENTED_EDGE('',*,*,#9533,.T.);
#13490=ORIENTED_EDGE('',*,*,#9534,.F.);
#13491=ORIENTED_EDGE('',*,*,#9366,.T.);
#13492=ORIENTED_EDGE('',*,*,#9535,.F.);
#13493=ORIENTED_EDGE('',*,*,#9532,.F.);
#13494=ORIENTED_EDGE('',*,*,#9536,.F.);
#13495=ORIENTED_EDGE('',*,*,#9537,.T.);
#13496=ORIENTED_EDGE('',*,*,#9538,.F.);
#13497=ORIENTED_EDGE('',*,*,#9533,.F.);
#13498=ORIENTED_EDGE('',*,*,#9539,.F.);
#13499=ORIENTED_EDGE('',*,*,#9540,.T.);
#13500=ORIENTED_EDGE('',*,*,#9541,.T.);
#13501=ORIENTED_EDGE('',*,*,#9542,.F.);
#13502=ORIENTED_EDGE('',*,*,#9543,.T.);
#13503=ORIENTED_EDGE('',*,*,#9544,.F.);
#13504=ORIENTED_EDGE('',*,*,#9540,.F.);
#13505=ORIENTED_EDGE('',*,*,#9545,.F.);
#13506=ORIENTED_EDGE('',*,*,#9546,.F.);
#13507=ORIENTED_EDGE('',*,*,#9547,.F.);
#13508=ORIENTED_EDGE('',*,*,#9541,.F.);
#13509=ORIENTED_EDGE('',*,*,#9548,.F.);
#13510=ORIENTED_EDGE('',*,*,#9549,.T.);
#13511=ORIENTED_EDGE('',*,*,#9550,.T.);
#13512=ORIENTED_EDGE('',*,*,#9543,.F.);
#13513=ORIENTED_EDGE('',*,*,#9551,.T.);
#13514=ORIENTED_EDGE('',*,*,#9552,.F.);
#13515=ORIENTED_EDGE('',*,*,#9549,.F.);
#13516=ORIENTED_EDGE('',*,*,#9553,.F.);
#13517=ORIENTED_EDGE('',*,*,#9554,.F.);
#13518=ORIENTED_EDGE('',*,*,#9555,.F.);
#13519=ORIENTED_EDGE('',*,*,#9550,.F.);
#13520=ORIENTED_EDGE('',*,*,#9556,.F.);
#13521=ORIENTED_EDGE('',*,*,#9557,.T.);
#13522=ORIENTED_EDGE('',*,*,#9558,.T.);
#13523=ORIENTED_EDGE('',*,*,#9551,.F.);
#13524=ORIENTED_EDGE('',*,*,#9559,.F.);
#13525=ORIENTED_EDGE('',*,*,#9560,.F.);
#13526=ORIENTED_EDGE('',*,*,#9557,.F.);
#13527=ORIENTED_EDGE('',*,*,#9561,.F.);
#13528=ORIENTED_EDGE('',*,*,#9562,.F.);
#13529=ORIENTED_EDGE('',*,*,#9563,.T.);
#13530=ORIENTED_EDGE('',*,*,#9564,.F.);
#13531=ORIENTED_EDGE('',*,*,#9447,.F.);
#13532=ORIENTED_EDGE('',*,*,#9565,.F.);
#13533=ORIENTED_EDGE('',*,*,#9566,.T.);
#13534=ORIENTED_EDGE('',*,*,#9567,.F.);
#13535=ORIENTED_EDGE('',*,*,#9565,.T.);
#13536=ORIENTED_EDGE('',*,*,#9568,.F.);
#13537=ORIENTED_EDGE('',*,*,#9448,.F.);
#13538=ORIENTED_EDGE('',*,*,#9569,.F.);
#13539=ORIENTED_EDGE('',*,*,#9570,.T.);
#13540=ORIENTED_EDGE('',*,*,#9571,.F.);
#13541=ORIENTED_EDGE('',*,*,#9572,.F.);
#13542=ORIENTED_EDGE('',*,*,#9573,.F.);
#13543=ORIENTED_EDGE('',*,*,#9570,.F.);
#13544=ORIENTED_EDGE('',*,*,#9574,.T.);
#13545=ORIENTED_EDGE('',*,*,#9575,.F.);
#13546=ORIENTED_EDGE('',*,*,#9567,.T.);
#13547=ORIENTED_EDGE('',*,*,#9576,.F.);
#13548=ORIENTED_EDGE('',*,*,#9574,.F.);
#13549=ORIENTED_EDGE('',*,*,#9577,.F.);
#13550=ORIENTED_EDGE('',*,*,#9575,.T.);
#13551=ORIENTED_EDGE('',*,*,#9578,.F.);
#13552=ORIENTED_EDGE('',*,*,#9579,.F.);
#13553=ORIENTED_EDGE('',*,*,#9580,.F.);
#13554=ORIENTED_EDGE('',*,*,#9581,.T.);
#13555=ORIENTED_EDGE('',*,*,#9582,.F.);
#13556=ORIENTED_EDGE('',*,*,#9442,.F.);
#13557=ORIENTED_EDGE('',*,*,#9583,.F.);
#13558=ORIENTED_EDGE('',*,*,#9579,.T.);
#13559=ORIENTED_EDGE('',*,*,#9584,.T.);
#13560=ORIENTED_EDGE('',*,*,#9581,.F.);
#13561=ORIENTED_EDGE('',*,*,#9444,.T.);
#13562=ORIENTED_EDGE('',*,*,#9585,.F.);
#13563=ORIENTED_EDGE('',*,*,#9584,.F.);
#13564=ORIENTED_EDGE('',*,*,#9586,.F.);
#13565=ORIENTED_EDGE('',*,*,#9566,.F.);
#13566=ORIENTED_EDGE('',*,*,#9587,.F.);
#13567=ORIENTED_EDGE('',*,*,#9588,.T.);
#13568=ORIENTED_EDGE('',*,*,#9589,.F.);
#13569=ORIENTED_EDGE('',*,*,#9436,.T.);
#13570=ORIENTED_EDGE('',*,*,#9572,.T.);
#13571=ORIENTED_EDGE('',*,*,#9438,.F.);
#13572=ORIENTED_EDGE('',*,*,#9391,.T.);
#13573=ORIENTED_EDGE('',*,*,#9590,.F.);
#13574=ORIENTED_EDGE('',*,*,#9591,.F.);
#13575=ORIENTED_EDGE('',*,*,#9592,.F.);
#13576=ORIENTED_EDGE('',*,*,#9593,.T.);
#13577=ORIENTED_EDGE('',*,*,#9591,.T.);
#13578=ORIENTED_EDGE('',*,*,#9594,.F.);
#13579=ORIENTED_EDGE('',*,*,#9595,.T.);
#13580=ORIENTED_EDGE('',*,*,#9596,.F.);
#13581=ORIENTED_EDGE('',*,*,#9593,.F.);
#13582=ORIENTED_EDGE('',*,*,#9597,.F.);
#13583=ORIENTED_EDGE('',*,*,#9534,.T.);
#13584=ORIENTED_EDGE('',*,*,#9598,.F.);
#13585=ORIENTED_EDGE('',*,*,#9433,.F.);
#13586=ORIENTED_EDGE('',*,*,#9599,.F.);
#13587=ORIENTED_EDGE('',*,*,#9594,.T.);
#13588=ORIENTED_EDGE('',*,*,#9600,.F.);
#13589=ORIENTED_EDGE('',*,*,#9431,.F.);
#13590=ORIENTED_EDGE('',*,*,#9601,.F.);
#13591=ORIENTED_EDGE('',*,*,#9432,.T.);
#13592=ORIENTED_EDGE('',*,*,#9602,.F.);
#13593=ORIENTED_EDGE('',*,*,#9603,.F.);
#13594=ORIENTED_EDGE('',*,*,#9604,.F.);
#13595=ORIENTED_EDGE('',*,*,#9544,.T.);
#13596=ORIENTED_EDGE('',*,*,#9555,.T.);
#13597=ORIENTED_EDGE('',*,*,#9605,.F.);
#13598=ORIENTED_EDGE('',*,*,#9548,.T.);
#13599=ORIENTED_EDGE('',*,*,#9606,.T.);
#13600=ORIENTED_EDGE('',*,*,#9364,.T.);
#13601=ORIENTED_EDGE('',*,*,#9607,.F.);
#13602=ORIENTED_EDGE('',*,*,#9561,.T.);
#13603=ORIENTED_EDGE('',*,*,#9553,.T.);
#13604=ORIENTED_EDGE('',*,*,#9545,.T.);
#13605=ORIENTED_EDGE('',*,*,#9608,.T.);
#13606=ORIENTED_EDGE('',*,*,#9609,.T.);
#13607=ORIENTED_EDGE('',*,*,#9610,.F.);
#13608=ORIENTED_EDGE('',*,*,#9611,.T.);
#13609=ORIENTED_EDGE('',*,*,#9612,.T.);
#13610=ORIENTED_EDGE('',*,*,#9560,.T.);
#13611=ORIENTED_EDGE('',*,*,#9613,.T.);
#13612=ORIENTED_EDGE('',*,*,#9614,.T.);
#13613=ORIENTED_EDGE('',*,*,#9615,.T.);
#13614=ORIENTED_EDGE('',*,*,#9616,.F.);
#13615=ORIENTED_EDGE('',*,*,#9617,.T.);
#13616=ORIENTED_EDGE('',*,*,#9618,.F.);
#13617=ORIENTED_EDGE('',*,*,#9556,.T.);
#13618=ORIENTED_EDGE('',*,*,#9552,.T.);
#13619=ORIENTED_EDGE('',*,*,#9619,.T.);
#13620=ORIENTED_EDGE('',*,*,#9427,.T.);
#13621=ORIENTED_EDGE('',*,*,#9491,.T.);
#13622=ORIENTED_EDGE('',*,*,#9620,.T.);
#13623=ORIENTED_EDGE('',*,*,#9621,.T.);
#13624=ORIENTED_EDGE('',*,*,#9622,.T.);
#13625=ORIENTED_EDGE('',*,*,#9623,.T.);
#13626=ORIENTED_EDGE('',*,*,#9624,.F.);
#13627=ORIENTED_EDGE('',*,*,#9398,.F.);
#13628=ORIENTED_EDGE('',*,*,#9625,.T.);
#13629=ORIENTED_EDGE('',*,*,#9404,.F.);
#13630=ORIENTED_EDGE('',*,*,#9626,.T.);
#13631=ORIENTED_EDGE('',*,*,#9627,.T.);
#13632=ORIENTED_EDGE('',*,*,#9628,.F.);
#13633=ORIENTED_EDGE('',*,*,#9451,.T.);
#13634=ORIENTED_EDGE('',*,*,#9629,.F.);
#13635=ORIENTED_EDGE('',*,*,#9420,.T.);
#13636=ORIENTED_EDGE('',*,*,#9422,.T.);
#13637=ORIENTED_EDGE('',*,*,#9630,.F.);
#13638=ORIENTED_EDGE('',*,*,#9631,.F.);
#13639=ORIENTED_EDGE('',*,*,#9409,.T.);
#13640=ORIENTED_EDGE('',*,*,#9624,.T.);
#13641=ORIENTED_EDGE('',*,*,#9632,.T.);
#13642=ORIENTED_EDGE('',*,*,#9399,.T.);
#13643=ORIENTED_EDGE('',*,*,#9421,.F.);
#13644=ORIENTED_EDGE('',*,*,#9629,.T.);
#13645=ORIENTED_EDGE('',*,*,#9413,.F.);
#13646=ORIENTED_EDGE('',*,*,#9632,.F.);
#13647=ORIENTED_EDGE('',*,*,#9625,.F.);
#13648=ORIENTED_EDGE('',*,*,#9633,.F.);
#13649=ORIENTED_EDGE('',*,*,#9630,.T.);
#13650=ORIENTED_EDGE('',*,*,#9487,.T.);
#13651=ORIENTED_EDGE('',*,*,#9634,.T.);
#13652=ORIENTED_EDGE('',*,*,#9635,.F.);
#13653=ORIENTED_EDGE('',*,*,#9636,.F.);
#13654=ORIENTED_EDGE('',*,*,#9401,.F.);
#13655=ORIENTED_EDGE('',*,*,#9637,.F.);
#13656=ORIENTED_EDGE('',*,*,#9411,.F.);
#13657=ORIENTED_EDGE('',*,*,#9381,.T.);
#13658=ORIENTED_EDGE('',*,*,#9638,.T.);
#13659=ORIENTED_EDGE('',*,*,#9639,.T.);
#13660=ORIENTED_EDGE('',*,*,#9493,.T.);
#13661=ORIENTED_EDGE('',*,*,#9640,.T.);
#13662=ORIENTED_EDGE('',*,*,#9474,.T.);
#13663=ORIENTED_EDGE('',*,*,#9641,.T.);
#13664=ORIENTED_EDGE('',*,*,#9268,.T.);
#13665=ORIENTED_EDGE('',*,*,#9517,.T.);
#13666=ORIENTED_EDGE('',*,*,#9314,.F.);
#13667=ORIENTED_EDGE('',*,*,#9642,.T.);
#13668=ORIENTED_EDGE('',*,*,#9293,.F.);
#13669=ORIENTED_EDGE('',*,*,#9353,.T.);
#13670=ORIENTED_EDGE('',*,*,#9466,.F.);
#13671=ORIENTED_EDGE('',*,*,#9361,.F.);
#13672=ORIENTED_EDGE('',*,*,#9492,.T.);
#13673=ORIENTED_EDGE('',*,*,#9623,.F.);
#13674=ORIENTED_EDGE('',*,*,#9643,.T.);
#13675=ORIENTED_EDGE('',*,*,#9335,.F.);
#13676=ORIENTED_EDGE('',*,*,#9475,.T.);
#13677=ORIENTED_EDGE('',*,*,#9640,.F.);
#13678=ORIENTED_EDGE('',*,*,#9495,.T.);
#13679=ORIENTED_EDGE('',*,*,#9478,.T.);
#13680=ORIENTED_EDGE('',*,*,#9463,.T.);
#13681=ORIENTED_EDGE('',*,*,#9610,.T.);
#13682=ORIENTED_EDGE('',*,*,#9644,.T.);
#13683=ORIENTED_EDGE('',*,*,#9645,.F.);
#13684=ORIENTED_EDGE('',*,*,#9646,.F.);
#13685=ORIENTED_EDGE('',*,*,#9645,.T.);
#13686=ORIENTED_EDGE('',*,*,#9647,.F.);
#13687=ORIENTED_EDGE('',*,*,#9648,.F.);
#13688=ORIENTED_EDGE('',*,*,#9649,.F.);
#13689=ORIENTED_EDGE('',*,*,#9646,.T.);
#13690=ORIENTED_EDGE('',*,*,#9650,.F.);
#13691=ORIENTED_EDGE('',*,*,#9365,.F.);
#13692=ORIENTED_EDGE('',*,*,#9606,.F.);
#13693=ORIENTED_EDGE('',*,*,#9537,.F.);
#13694=ORIENTED_EDGE('',*,*,#9648,.T.);
#13695=ORIENTED_EDGE('',*,*,#9595,.F.);
#13696=ORIENTED_EDGE('',*,*,#9388,.F.);
#13697=ORIENTED_EDGE('',*,*,#9651,.T.);
#13698=ORIENTED_EDGE('',*,*,#9652,.T.);
#13699=ORIENTED_EDGE('',*,*,#9390,.T.);
#13700=ORIENTED_EDGE('',*,*,#9597,.T.);
#13701=ORIENTED_EDGE('',*,*,#9601,.T.);
#13702=ORIENTED_EDGE('',*,*,#9598,.T.);
#13703=ORIENTED_EDGE('',*,*,#9538,.T.);
#13704=ORIENTED_EDGE('',*,*,#9443,.T.);
#13705=ORIENTED_EDGE('',*,*,#9653,.F.);
#13706=ORIENTED_EDGE('',*,*,#9654,.F.);
#13707=ORIENTED_EDGE('',*,*,#9655,.F.);
#13708=ORIENTED_EDGE('',*,*,#9654,.T.);
#13709=ORIENTED_EDGE('',*,*,#9656,.F.);
#13710=ORIENTED_EDGE('',*,*,#9383,.F.);
#13711=ORIENTED_EDGE('',*,*,#9657,.F.);
#13712=ORIENTED_EDGE('',*,*,#9658,.T.);
#13713=ORIENTED_EDGE('',*,*,#9659,.T.);
#13714=ORIENTED_EDGE('',*,*,#9635,.T.);
#13715=ORIENTED_EDGE('',*,*,#9660,.T.);
#13716=ORIENTED_EDGE('',*,*,#9637,.T.);
#13717=ORIENTED_EDGE('',*,*,#9380,.T.);
#13718=ORIENTED_EDGE('',*,*,#9659,.F.);
#13719=ORIENTED_EDGE('',*,*,#9661,.F.);
#13720=ORIENTED_EDGE('',*,*,#9636,.T.);
#13721=ORIENTED_EDGE('',*,*,#9662,.F.);
#13722=ORIENTED_EDGE('',*,*,#9658,.F.);
#13723=ORIENTED_EDGE('',*,*,#9379,.F.);
#13724=ORIENTED_EDGE('',*,*,#9410,.F.);
#13725=ORIENTED_EDGE('',*,*,#9631,.T.);
#13726=ORIENTED_EDGE('',*,*,#9633,.T.);
#13727=ORIENTED_EDGE('',*,*,#9397,.F.);
#13728=ORIENTED_EDGE('',*,*,#9412,.F.);
#13729=ORIENTED_EDGE('',*,*,#9660,.F.);
#13730=ORIENTED_EDGE('',*,*,#9634,.F.);
#13731=ORIENTED_EDGE('',*,*,#9663,.T.);
#13732=ORIENTED_EDGE('',*,*,#9664,.T.);
#13733=ORIENTED_EDGE('',*,*,#9665,.F.);
#13734=ORIENTED_EDGE('',*,*,#9402,.T.);
#13735=ORIENTED_EDGE('',*,*,#9661,.T.);
#13736=ORIENTED_EDGE('',*,*,#9662,.T.);
#13737=ORIENTED_EDGE('',*,*,#9407,.T.);
#13738=ORIENTED_EDGE('',*,*,#9416,.T.);
#13739=ORIENTED_EDGE('',*,*,#9418,.T.);
#13740=ORIENTED_EDGE('',*,*,#9622,.F.);
#13741=ORIENTED_EDGE('',*,*,#9666,.T.);
#13742=ORIENTED_EDGE('',*,*,#9336,.F.);
#13743=ORIENTED_EDGE('',*,*,#9643,.F.);
#13744=ORIENTED_EDGE('',*,*,#9374,.F.);
#13745=ORIENTED_EDGE('',*,*,#9324,.F.);
#13746=ORIENTED_EDGE('',*,*,#9327,.F.);
#13747=ORIENTED_EDGE('',*,*,#9326,.F.);
#13748=ORIENTED_EDGE('',*,*,#9377,.T.);
#13749=ORIENTED_EDGE('',*,*,#9419,.F.);
#13750=ORIENTED_EDGE('',*,*,#9414,.F.);
#13751=ORIENTED_EDGE('',*,*,#9667,.F.);
#13752=ORIENTED_EDGE('',*,*,#9308,.F.);
#13753=ORIENTED_EDGE('',*,*,#9307,.F.);
#13754=ORIENTED_EDGE('',*,*,#9668,.F.);
#13755=ORIENTED_EDGE('',*,*,#9294,.F.);
#13756=ORIENTED_EDGE('',*,*,#9642,.F.);
#13757=ORIENTED_EDGE('',*,*,#9313,.F.);
#13758=ORIENTED_EDGE('',*,*,#9312,.F.);
#13759=ORIENTED_EDGE('',*,*,#9669,.F.);
#13760=ORIENTED_EDGE('',*,*,#9664,.F.);
#13761=ORIENTED_EDGE('',*,*,#9670,.T.);
#13762=ORIENTED_EDGE('',*,*,#9310,.T.);
#13763=ORIENTED_EDGE('',*,*,#9671,.F.);
#13764=ORIENTED_EDGE('',*,*,#9627,.F.);
#13765=ORIENTED_EDGE('',*,*,#9665,.T.);
#13766=ORIENTED_EDGE('',*,*,#9669,.T.);
#13767=ORIENTED_EDGE('',*,*,#9311,.T.);
#13768=ORIENTED_EDGE('',*,*,#9670,.F.);
#13769=ORIENTED_EDGE('',*,*,#9626,.F.);
#13770=ORIENTED_EDGE('',*,*,#9403,.T.);
#13771=ORIENTED_EDGE('',*,*,#9542,.T.);
#13772=ORIENTED_EDGE('',*,*,#9672,.F.);
#13773=ORIENTED_EDGE('',*,*,#9673,.F.);
#13774=ORIENTED_EDGE('',*,*,#9608,.F.);
#13775=ORIENTED_EDGE('',*,*,#9644,.F.);
#13776=ORIENTED_EDGE('',*,*,#9609,.F.);
#13777=ORIENTED_EDGE('',*,*,#9674,.T.);
#13778=ORIENTED_EDGE('',*,*,#9675,.F.);
#13779=ORIENTED_EDGE('',*,*,#9676,.F.);
#13780=ORIENTED_EDGE('',*,*,#9677,.F.);
#13781=ORIENTED_EDGE('',*,*,#9674,.F.);
#13782=ORIENTED_EDGE('',*,*,#9673,.T.);
#13783=ORIENTED_EDGE('',*,*,#9604,.T.);
#13784=ORIENTED_EDGE('',*,*,#9678,.T.);
#13785=ORIENTED_EDGE('',*,*,#9386,.F.);
#13786=ORIENTED_EDGE('',*,*,#9445,.T.);
#13787=ORIENTED_EDGE('',*,*,#9586,.T.);
#13788=ORIENTED_EDGE('',*,*,#9578,.T.);
#13789=ORIENTED_EDGE('',*,*,#9576,.T.);
#13790=ORIENTED_EDGE('',*,*,#9589,.T.);
#13791=ORIENTED_EDGE('',*,*,#9679,.F.);
#13792=ORIENTED_EDGE('',*,*,#9680,.F.);
#13793=ORIENTED_EDGE('',*,*,#9613,.F.);
#13794=ORIENTED_EDGE('',*,*,#9559,.T.);
#13795=ORIENTED_EDGE('',*,*,#9607,.T.);
#13796=ORIENTED_EDGE('',*,*,#9363,.T.);
#13797=ORIENTED_EDGE('',*,*,#9536,.T.);
#13798=ORIENTED_EDGE('',*,*,#9599,.T.);
#13799=ORIENTED_EDGE('',*,*,#9681,.T.);
#13800=ORIENTED_EDGE('',*,*,#9531,.T.);
#13801=ORIENTED_EDGE('',*,*,#9682,.T.);
#13802=ORIENTED_EDGE('',*,*,#9616,.T.);
#13803=ORIENTED_EDGE('',*,*,#9683,.T.);
#13804=ORIENTED_EDGE('',*,*,#9351,.T.);
#13805=ORIENTED_EDGE('',*,*,#9684,.T.);
#13806=ORIENTED_EDGE('',*,*,#9685,.T.);
#13807=ORIENTED_EDGE('',*,*,#9686,.T.);
#13808=ORIENTED_EDGE('',*,*,#9342,.T.);
#13809=ORIENTED_EDGE('',*,*,#9687,.T.);
#13810=ORIENTED_EDGE('',*,*,#9688,.T.);
#13811=ORIENTED_EDGE('',*,*,#9689,.T.);
#13812=ORIENTED_EDGE('',*,*,#9690,.T.);
#13813=ORIENTED_EDGE('',*,*,#9484,.F.);
#13814=ORIENTED_EDGE('',*,*,#9470,.F.);
#13815=ORIENTED_EDGE('',*,*,#9573,.T.);
#13816=ORIENTED_EDGE('',*,*,#9435,.T.);
#13817=ORIENTED_EDGE('',*,*,#9568,.T.);
#13818=ORIENTED_EDGE('',*,*,#9577,.T.);
#13819=ORIENTED_EDGE('',*,*,#9583,.T.);
#13820=ORIENTED_EDGE('',*,*,#9439,.T.);
#13821=ORIENTED_EDGE('',*,*,#9571,.T.);
#13822=ORIENTED_EDGE('',*,*,#9580,.T.);
#13823=ORIENTED_EDGE('',*,*,#9685,.F.);
#13824=ORIENTED_EDGE('',*,*,#9691,.T.);
#13825=ORIENTED_EDGE('',*,*,#9692,.T.);
#13826=ORIENTED_EDGE('',*,*,#9587,.T.);
#13827=ORIENTED_EDGE('',*,*,#9569,.T.);
#13828=ORIENTED_EDGE('',*,*,#9564,.T.);
#13829=ORIENTED_EDGE('',*,*,#9693,.T.);
#13830=ORIENTED_EDGE('',*,*,#9694,.T.);
#13831=ORIENTED_EDGE('',*,*,#9652,.F.);
#13832=ORIENTED_EDGE('',*,*,#9602,.T.);
#13833=ORIENTED_EDGE('',*,*,#9600,.T.);
#13834=ORIENTED_EDGE('',*,*,#9590,.T.);
#13835=ORIENTED_EDGE('',*,*,#9695,.T.);
#13836=ORIENTED_EDGE('',*,*,#9653,.T.);
#13837=ORIENTED_EDGE('',*,*,#9582,.T.);
#13838=ORIENTED_EDGE('',*,*,#9585,.T.);
#13839=ORIENTED_EDGE('',*,*,#9309,.F.);
#13840=ORIENTED_EDGE('',*,*,#9667,.T.);
#13841=ORIENTED_EDGE('',*,*,#9663,.F.);
#13842=ORIENTED_EDGE('',*,*,#9417,.T.);
#13843=ORIENTED_EDGE('',*,*,#9405,.F.);
#13844=ORIENTED_EDGE('',*,*,#9628,.T.);
#13845=ORIENTED_EDGE('',*,*,#9671,.T.);
#13846=ORIENTED_EDGE('',*,*,#9649,.T.);
#13847=ORIENTED_EDGE('',*,*,#9539,.T.);
#13848=ORIENTED_EDGE('',*,*,#9535,.T.);
#13849=ORIENTED_EDGE('',*,*,#9650,.T.);
#13850=ORIENTED_EDGE('',*,*,#9696,.T.);
#13851=ORIENTED_EDGE('',*,*,#9697,.T.);
#13852=ORIENTED_EDGE('',*,*,#9698,.F.);
#13853=ORIENTED_EDGE('',*,*,#9679,.T.);
#13854=ORIENTED_EDGE('',*,*,#9384,.T.);
#13855=ORIENTED_EDGE('',*,*,#9656,.T.);
#13856=ORIENTED_EDGE('',*,*,#9695,.F.);
#13857=ORIENTED_EDGE('',*,*,#9446,.T.);
#13858=ORIENTED_EDGE('',*,*,#9618,.T.);
#13859=ORIENTED_EDGE('',*,*,#9699,.T.);
#13860=ORIENTED_EDGE('',*,*,#9513,.F.);
#13861=ORIENTED_EDGE('',*,*,#9504,.T.);
#13862=ORIENTED_EDGE('',*,*,#9467,.T.);
#13863=ORIENTED_EDGE('',*,*,#9700,.T.);
#13864=ORIENTED_EDGE('',*,*,#9701,.T.);
#13865=ORIENTED_EDGE('',*,*,#9546,.T.);
#13866=ORIENTED_EDGE('',*,*,#9605,.T.);
#13867=ORIENTED_EDGE('',*,*,#9554,.T.);
#13868=ORIENTED_EDGE('',*,*,#9702,.T.);
#13869=ORIENTED_EDGE('',*,*,#9703,.T.);
#13870=ORIENTED_EDGE('',*,*,#9704,.T.);
#13871=ORIENTED_EDGE('',*,*,#9614,.F.);
#13872=ORIENTED_EDGE('',*,*,#9705,.T.);
#13873=ORIENTED_EDGE('',*,*,#9611,.F.);
#13874=ORIENTED_EDGE('',*,*,#9680,.T.);
#13875=ORIENTED_EDGE('',*,*,#9698,.T.);
#13876=ORIENTED_EDGE('',*,*,#9332,.F.);
#13877=ORIENTED_EDGE('',*,*,#9706,.T.);
#13878=ORIENTED_EDGE('',*,*,#9707,.F.);
#13879=ORIENTED_EDGE('',*,*,#9305,.F.);
#13880=ORIENTED_EDGE('',*,*,#9708,.T.);
#13881=ORIENTED_EDGE('',*,*,#9638,.F.);
#13882=ORIENTED_EDGE('',*,*,#9473,.F.);
#13883=ORIENTED_EDGE('',*,*,#9333,.F.);
#13884=ORIENTED_EDGE('',*,*,#9396,.F.);
#13885=ORIENTED_EDGE('',*,*,#9709,.T.);
#13886=ORIENTED_EDGE('',*,*,#9338,.F.);
#13887=ORIENTED_EDGE('',*,*,#9337,.F.);
#13888=ORIENTED_EDGE('',*,*,#9666,.F.);
#13889=ORIENTED_EDGE('',*,*,#9621,.F.);
#13890=ORIENTED_EDGE('',*,*,#9710,.T.);
#13891=ORIENTED_EDGE('',*,*,#9303,.F.);
#13892=ORIENTED_EDGE('',*,*,#9352,.F.);
#13893=ORIENTED_EDGE('',*,*,#9711,.T.);
#13894=ORIENTED_EDGE('',*,*,#9712,.F.);
#13895=ORIENTED_EDGE('',*,*,#9703,.F.);
#13896=ORIENTED_EDGE('',*,*,#9713,.F.);
#13897=ORIENTED_EDGE('',*,*,#9320,.F.);
#13898=ORIENTED_EDGE('',*,*,#9712,.T.);
#13899=ORIENTED_EDGE('',*,*,#9702,.F.);
#13900=ORIENTED_EDGE('',*,*,#9697,.F.);
#13901=ORIENTED_EDGE('',*,*,#9714,.F.);
#13902=ORIENTED_EDGE('',*,*,#9321,.F.);
#13903=ORIENTED_EDGE('',*,*,#9713,.T.);
#13904=ORIENTED_EDGE('',*,*,#9692,.F.);
#13905=ORIENTED_EDGE('',*,*,#9715,.T.);
#13906=ORIENTED_EDGE('',*,*,#9696,.F.);
#13907=ORIENTED_EDGE('',*,*,#9588,.F.);
#13908=ORIENTED_EDGE('',*,*,#9350,.T.);
#13909=ORIENTED_EDGE('',*,*,#9323,.F.);
#13910=ORIENTED_EDGE('',*,*,#9716,.F.);
#13911=ORIENTED_EDGE('',*,*,#9691,.F.);
#13912=ORIENTED_EDGE('',*,*,#9684,.F.);
#13913=ORIENTED_EDGE('',*,*,#9346,.F.);
#13914=ORIENTED_EDGE('',*,*,#9328,.F.);
#13915=ORIENTED_EDGE('',*,*,#9349,.T.);
#13916=ORIENTED_EDGE('',*,*,#9356,.F.);
#13917=ORIENTED_EDGE('',*,*,#9355,.F.);
#13918=ORIENTED_EDGE('',*,*,#9714,.T.);
#13919=ORIENTED_EDGE('',*,*,#9715,.F.);
#13920=ORIENTED_EDGE('',*,*,#9716,.T.);
#13921=ORIENTED_EDGE('',*,*,#9322,.F.);
#13922=ORIENTED_EDGE('',*,*,#9705,.F.);
#13923=ORIENTED_EDGE('',*,*,#9619,.F.);
#13924=ORIENTED_EDGE('',*,*,#9558,.F.);
#13925=ORIENTED_EDGE('',*,*,#9612,.F.);
#13926=ORIENTED_EDGE('',*,*,#9387,.F.);
#13927=ORIENTED_EDGE('',*,*,#9678,.F.);
#13928=ORIENTED_EDGE('',*,*,#9603,.T.);
#13929=ORIENTED_EDGE('',*,*,#9651,.F.);
#13930=ORIENTED_EDGE('',*,*,#9711,.F.);
#13931=ORIENTED_EDGE('',*,*,#9683,.F.);
#13932=ORIENTED_EDGE('',*,*,#9615,.F.);
#13933=ORIENTED_EDGE('',*,*,#9704,.F.);
#13934=ORIENTED_EDGE('',*,*,#9717,.F.);
#13935=ORIENTED_EDGE('',*,*,#9718,.T.);
#13936=ORIENTED_EDGE('',*,*,#9693,.F.);
#13937=ORIENTED_EDGE('',*,*,#9563,.F.);
#13938=ORIENTED_EDGE('',*,*,#9682,.F.);
#13939=ORIENTED_EDGE('',*,*,#9530,.T.);
#13940=ORIENTED_EDGE('',*,*,#9699,.F.);
#13941=ORIENTED_EDGE('',*,*,#9617,.F.);
#13942=ORIENTED_EDGE('',*,*,#9719,.F.);
#13943=ORIENTED_EDGE('',*,*,#9700,.F.);
#13944=ORIENTED_EDGE('',*,*,#9343,.T.);
#13945=ORIENTED_EDGE('',*,*,#9686,.F.);
#13946=ORIENTED_EDGE('',*,*,#9694,.F.);
#13947=ORIENTED_EDGE('',*,*,#9718,.F.);
#13948=ORIENTED_EDGE('',*,*,#9512,.F.);
#13949=ORIENTED_EDGE('',*,*,#9529,.T.);
#13950=ORIENTED_EDGE('',*,*,#9681,.F.);
#13951=ORIENTED_EDGE('',*,*,#9720,.F.);
#13952=ORIENTED_EDGE('',*,*,#9720,.T.);
#13953=ORIENTED_EDGE('',*,*,#9690,.F.);
#13954=ORIENTED_EDGE('',*,*,#9721,.F.);
#13955=ORIENTED_EDGE('',*,*,#9510,.F.);
#13956=ORIENTED_EDGE('',*,*,#9721,.T.);
#13957=ORIENTED_EDGE('',*,*,#9689,.F.);
#13958=ORIENTED_EDGE('',*,*,#9722,.F.);
#13959=ORIENTED_EDGE('',*,*,#9508,.F.);
#13960=ORIENTED_EDGE('',*,*,#9722,.T.);
#13961=ORIENTED_EDGE('',*,*,#9688,.F.);
#13962=ORIENTED_EDGE('',*,*,#9723,.F.);
#13963=ORIENTED_EDGE('',*,*,#9500,.F.);
#13964=ORIENTED_EDGE('',*,*,#9687,.F.);
#13965=ORIENTED_EDGE('',*,*,#9341,.T.);
#13966=ORIENTED_EDGE('',*,*,#9497,.F.);
#13967=ORIENTED_EDGE('',*,*,#9723,.T.);
#13968=ORIENTED_EDGE('',*,*,#9708,.F.);
#13969=ORIENTED_EDGE('',*,*,#9304,.F.);
#13970=ORIENTED_EDGE('',*,*,#9710,.F.);
#13971=ORIENTED_EDGE('',*,*,#9620,.F.);
#13972=ORIENTED_EDGE('',*,*,#9490,.F.);
#13973=ORIENTED_EDGE('',*,*,#9359,.F.);
#13974=ORIENTED_EDGE('',*,*,#9358,.F.);
#13975=ORIENTED_EDGE('',*,*,#9357,.F.);
#13976=ORIENTED_EDGE('',*,*,#9494,.F.);
#13977=ORIENTED_EDGE('',*,*,#9639,.F.);
#13978=ORIENTED_EDGE('',*,*,#9395,.F.);
#13979=ORIENTED_EDGE('',*,*,#9296,.F.);
#13980=ORIENTED_EDGE('',*,*,#9724,.F.);
#13981=ORIENTED_EDGE('',*,*,#9706,.F.);
#13982=ORIENTED_EDGE('',*,*,#9339,.F.);
#13983=ORIENTED_EDGE('',*,*,#9709,.F.);
#13984=ORIENTED_EDGE('',*,*,#9330,.F.);
#13985=ORIENTED_EDGE('',*,*,#9428,.F.);
#13986=ORIENTED_EDGE('',*,*,#9707,.T.);
#13987=ORIENTED_EDGE('',*,*,#9724,.T.);
#13988=ORIENTED_EDGE('',*,*,#9295,.F.);
#13989=ORIENTED_EDGE('',*,*,#9668,.T.);
#13990=ORIENTED_EDGE('',*,*,#9306,.F.);
#13991=ORIENTED_EDGE('',*,*,#9317,.F.);
#13992=ORIENTED_EDGE('',*,*,#9526,.T.);
#13993=ORIENTED_EDGE('',*,*,#9272,.F.);
#13994=ORIENTED_EDGE('',*,*,#9285,.F.);
#13995=ORIENTED_EDGE('',*,*,#9725,.T.);
#13996=ORIENTED_EDGE('',*,*,#9726,.T.);
#13997=ORIENTED_EDGE('',*,*,#9394,.F.);
#13998=ORIENTED_EDGE('',*,*,#9725,.F.);
#13999=ORIENTED_EDGE('',*,*,#9284,.F.);
#14000=ORIENTED_EDGE('',*,*,#9519,.T.);
#14001=ORIENTED_EDGE('',*,*,#9263,.T.);
#14002=ORIENTED_EDGE('',*,*,#9641,.F.);
#14003=ORIENTED_EDGE('',*,*,#9292,.F.);
#14004=ORIENTED_EDGE('',*,*,#9726,.F.);
#14005=ORIENTED_EDGE('',*,*,#9283,.F.);
#14006=ORIENTED_EDGE('',*,*,#9276,.F.);
#14007=ORIENTED_EDGE('',*,*,#9727,.F.);
#14008=ORIENTED_EDGE('',*,*,#9280,.F.);
#14009=ORIENTED_EDGE('',*,*,#9728,.F.);
#14010=ORIENTED_EDGE('',*,*,#9729,.F.);
#14011=ORIENTED_EDGE('',*,*,#9455,.T.);
#14012=ORIENTED_EDGE('',*,*,#9265,.T.);
#14013=ORIENTED_EDGE('',*,*,#9518,.T.);
#14014=ORIENTED_EDGE('',*,*,#9459,.T.);
#14015=ORIENTED_EDGE('',*,*,#9525,.T.);
#14016=ORIENTED_EDGE('',*,*,#9528,.T.);
#14017=ORIENTED_EDGE('',*,*,#9457,.T.);
#14018=ORIENTED_EDGE('',*,*,#9462,.T.);
#14019=ORIENTED_EDGE('',*,*,#9523,.T.);
#14020=ORIENTED_EDGE('',*,*,#9730,.F.);
#14021=ORIENTED_EDGE('',*,*,#9729,.T.);
#14022=ORIENTED_EDGE('',*,*,#9515,.F.);
#14023=ORIENTED_EDGE('',*,*,#9288,.T.);
#14024=ORIENTED_EDGE('',*,*,#9281,.F.);
#14025=ORIENTED_EDGE('',*,*,#9727,.T.);
#14026=ORIENTED_EDGE('',*,*,#9730,.T.);
#14027=ORIENTED_EDGE('',*,*,#9728,.T.);
#14028=ORIENTED_EDGE('',*,*,#9279,.F.);
#14029=ORIENTED_EDGE('',*,*,#9287,.T.);
#14030=ORIENTED_EDGE('',*,*,#9655,.T.);
#14031=ORIENTED_EDGE('',*,*,#9657,.T.);
#14032=ORIENTED_EDGE('',*,*,#9382,.T.);
#14033=ORIENTED_EDGE('',*,*,#9392,.T.);
#14034=ORIENTED_EDGE('',*,*,#9592,.T.);
#14035=ORIENTED_EDGE('',*,*,#9596,.T.);
#14036=ORIENTED_EDGE('',*,*,#9647,.T.);
#14037=ORIENTED_EDGE('',*,*,#9675,.T.);
#14038=ORIENTED_EDGE('',*,*,#9677,.T.);
#14039=ORIENTED_EDGE('',*,*,#9731,.F.);
#14040=ORIENTED_EDGE('',*,*,#9732,.T.);
#14041=ORIENTED_EDGE('',*,*,#9733,.F.);
#14042=ORIENTED_EDGE('',*,*,#9562,.T.);
#14043=ORIENTED_EDGE('',*,*,#9437,.T.);
#14044=ORIENTED_EDGE('',*,*,#9441,.T.);
#14045=ORIENTED_EDGE('',*,*,#9734,.T.);
#14046=ORIENTED_EDGE('',*,*,#9732,.F.);
#14047=ORIENTED_EDGE('',*,*,#9701,.F.);
#14048=ORIENTED_EDGE('',*,*,#9719,.T.);
#14049=ORIENTED_EDGE('',*,*,#9717,.T.);
#14050=ORIENTED_EDGE('',*,*,#9733,.T.);
#14051=ORIENTED_EDGE('',*,*,#9734,.F.);
#14052=ORIENTED_EDGE('',*,*,#9731,.T.);
#14053=ORIENTED_EDGE('',*,*,#9676,.T.);
#14054=ORIENTED_EDGE('',*,*,#9672,.T.);
#14055=ORIENTED_EDGE('',*,*,#9547,.T.);
#14056=ORIENTED_EDGE('',*,*,#9425,.F.);
#14296=TOROIDAL_SURFACE('',#16489,17.0599057548774,0.5);
#14297=TOROIDAL_SURFACE('',#16502,2.20465088114115,0.3);
#14298=TOROIDAL_SURFACE('',#16510,16.5,3.);
#14299=TOROIDAL_SURFACE('',#16527,19.5,0.5);
#14300=TOROIDAL_SURFACE('',#16532,4.5,1.);
#14301=TOROIDAL_SURFACE('',#16537,19.5,0.5);
#14302=TOROIDAL_SURFACE('',#16543,17.5,1.);
#14303=TOROIDAL_SURFACE('',#16551,1.,0.5);
#14304=TOROIDAL_SURFACE('',#16561,6.,0.5);
#14305=TOROIDAL_SURFACE('',#16572,19.5,3.);
#14306=TOROIDAL_SURFACE('',#16632,19.5,5.);
#14307=TOROIDAL_SURFACE('',#16637,16.5,1.);
#14308=TOROIDAL_SURFACE('',#16671,17.,0.5);
#14309=TOROIDAL_SURFACE('',#16676,20.,1.);
#14310=TOROIDAL_SURFACE('',#16761,6.,0.5);
#14311=TOROIDAL_SURFACE('',#16767,19.5,3.);
#14312=TOROIDAL_SURFACE('',#16771,1.,0.5);
#14313=TOROIDAL_SURFACE('',#16820,17.5,1.);
#14314=TOROIDAL_SURFACE('',#16834,4.5,1.);
#14315=TOROIDAL_SURFACE('',#16838,20.,1.);
#14316=TOROIDAL_SURFACE('',#16842,19.5,3.);
#14317=TOROIDAL_SURFACE('',#16845,2.30308838114115,0.3);
#14962=ADVANCED_FACE('',(#4327),#14296,.F.);
#14963=ADVANCED_FACE('',(#4328),#3606,.T.);
#14964=ADVANCED_FACE('',(#4329),#1045,.T.);
#14965=ADVANCED_FACE('',(#4330),#14297,.T.);
#14966=ADVANCED_FACE('',(#4331),#1046,.T.);
#14967=ADVANCED_FACE('',(#4332),#14298,.T.);
#14968=ADVANCED_FACE('',(#4333,#258,#259),#3607,.T.);
#14969=ADVANCED_FACE('',(#4334),#14299,.T.);
#14970=ADVANCED_FACE('',(#4335),#3608,.T.);
#14971=ADVANCED_FACE('',(#4336),#14300,.T.);
#14972=ADVANCED_FACE('',(#4337),#14301,.T.);
#14973=ADVANCED_FACE('',(#4338),#168,.F.);
#14974=ADVANCED_FACE('',(#4339),#14302,.F.);
#14975=ADVANCED_FACE('',(#4340),#3609,.T.);
#14976=ADVANCED_FACE('',(#4341),#3610,.T.);
#14977=ADVANCED_FACE('',(#4342),#14303,.F.);
#14978=ADVANCED_FACE('',(#4343,#260,#261),#3611,.F.);
#14979=ADVANCED_FACE('',(#4344),#169,.F.);
#14980=ADVANCED_FACE('',(#4345),#14304,.T.);
#14981=ADVANCED_FACE('',(#4346),#3612,.F.);
#14982=ADVANCED_FACE('',(#4347),#3613,.T.);
#14983=ADVANCED_FACE('',(#4348),#3614,.T.);
#14984=ADVANCED_FACE('',(#4349),#14305,.F.);
#14985=ADVANCED_FACE('',(#4350),#3615,.T.);
#14986=ADVANCED_FACE('',(#4351),#3616,.T.);
#14987=ADVANCED_FACE('',(#4352),#3617,.T.);
#14988=ADVANCED_FACE('',(#4353),#3618,.F.);
#14989=ADVANCED_FACE('',(#4354),#3619,.F.);
#14990=ADVANCED_FACE('',(#4355),#3620,.F.);
#14991=ADVANCED_FACE('',(#4356),#83,.T.);
#14992=ADVANCED_FACE('',(#4357),#3621,.T.);
#14993=ADVANCED_FACE('',(#4358),#3622,.T.);
#14994=ADVANCED_FACE('',(#4359),#84,.T.);
#14995=ADVANCED_FACE('',(#4360),#3623,.T.);
#14996=ADVANCED_FACE('',(#4361),#85,.T.);
#14997=ADVANCED_FACE('',(#4362),#3624,.F.);
#14998=ADVANCED_FACE('',(#4363),#3625,.T.);
#14999=ADVANCED_FACE('',(#4364),#3626,.T.);
#15000=ADVANCED_FACE('',(#4365),#3627,.F.);
#15001=ADVANCED_FACE('',(#4366),#3628,.F.);
#15002=ADVANCED_FACE('',(#4367),#3629,.T.);
#15003=ADVANCED_FACE('',(#4368),#3630,.F.);
#15004=ADVANCED_FACE('',(#4369),#3631,.F.);
#15005=ADVANCED_FACE('',(#4370),#3632,.F.);
#15006=ADVANCED_FACE('',(#4371),#14306,.T.);
#15007=ADVANCED_FACE('',(#4372),#1047,.F.);
#15008=ADVANCED_FACE('',(#4373),#14307,.F.);
#15009=ADVANCED_FACE('',(#4374),#3633,.F.);
#15010=ADVANCED_FACE('',(#4375),#3634,.F.);
#15011=ADVANCED_FACE('',(#4376),#669,.F.);
#15012=ADVANCED_FACE('',(#4377),#670,.F.);
#15013=ADVANCED_FACE('',(#4378),#671,.F.);
#15014=ADVANCED_FACE('',(#4379),#3635,.F.);
#15015=ADVANCED_FACE('',(#4380),#3636,.F.);
#15016=ADVANCED_FACE('',(#4381),#672,.T.);
#15017=ADVANCED_FACE('',(#4382),#3637,.T.);
#15018=ADVANCED_FACE('',(#4383,#262,#263,#264),#673,.F.);
#15019=ADVANCED_FACE('',(#4384),#674,.T.);
#15020=ADVANCED_FACE('',(#4385),#3638,.T.);
#15021=ADVANCED_FACE('',(#4386),#675,.T.);
#15022=ADVANCED_FACE('',(#4387),#3639,.T.);
#15023=ADVANCED_FACE('',(#4388),#676,.F.);
#15024=ADVANCED_FACE('',(#4389),#170,.F.);
#15025=ADVANCED_FACE('',(#4390),#171,.F.);
#15026=ADVANCED_FACE('',(#4391),#172,.F.);
#15027=ADVANCED_FACE('',(#4392),#173,.F.);
#15028=ADVANCED_FACE('',(#4393),#174,.F.);
#15029=ADVANCED_FACE('',(#4394),#14308,.F.);
#15030=ADVANCED_FACE('',(#4395),#175,.F.);
#15031=ADVANCED_FACE('',(#4396),#86,.T.);
#15032=ADVANCED_FACE('',(#4397),#677,.F.);
#15033=ADVANCED_FACE('',(#4398),#14309,.T.);
#15034=ADVANCED_FACE('',(#4399),#87,.T.);
#15035=ADVANCED_FACE('',(#4400),#3640,.T.);
#15036=ADVANCED_FACE('',(#4401),#3641,.T.);
#15037=ADVANCED_FACE('',(#4402),#88,.T.);
#15038=ADVANCED_FACE('',(#4403),#3642,.T.);
#15039=ADVANCED_FACE('',(#4404),#3643,.T.);
#15040=ADVANCED_FACE('',(#4405),#89,.T.);
#15041=ADVANCED_FACE('',(#4406),#3644,.T.);
#15042=ADVANCED_FACE('',(#4407),#3645,.T.);
#15043=ADVANCED_FACE('',(#4408),#90,.T.);
#15044=ADVANCED_FACE('',(#4409),#3646,.T.);
#15045=ADVANCED_FACE('',(#4410),#3647,.T.);
#15046=ADVANCED_FACE('',(#4411),#91,.T.);
#15047=ADVANCED_FACE('',(#4412),#3648,.T.);
#15048=ADVANCED_FACE('',(#4413),#3649,.T.);
#15049=ADVANCED_FACE('',(#4414),#92,.T.);
#15050=ADVANCED_FACE('',(#4415),#3650,.T.);
#15051=ADVANCED_FACE('',(#4416),#3651,.T.);
#15052=ADVANCED_FACE('',(#4417),#3652,.T.);
#15053=ADVANCED_FACE('',(#4418),#93,.T.);
#15054=ADVANCED_FACE('',(#4419),#3653,.T.);
#15055=ADVANCED_FACE('',(#4420),#3654,.T.);
#15056=ADVANCED_FACE('',(#4421),#94,.T.);
#15057=ADVANCED_FACE('',(#4422),#3655,.T.);
#15058=ADVANCED_FACE('',(#4423),#95,.T.);
#15059=ADVANCED_FACE('',(#4424),#3656,.T.);
#15060=ADVANCED_FACE('',(#4425),#3657,.T.);
#15061=ADVANCED_FACE('',(#4426),#3658,.T.);
#15062=ADVANCED_FACE('',(#4427),#3659,.T.);
#15063=ADVANCED_FACE('',(#4428),#678,.F.);
#15064=ADVANCED_FACE('',(#4429),#679,.T.);
#15065=ADVANCED_FACE('',(#4430),#680,.F.);
#15066=ADVANCED_FACE('',(#4431,#265),#681,.F.);
#15067=ADVANCED_FACE('',(#4432),#682,.T.);
#15068=ADVANCED_FACE('',(#4433),#3660,.T.);
#15069=ADVANCED_FACE('',(#4434,#266),#683,.F.);
#15070=ADVANCED_FACE('',(#4435),#684,.T.);
#15071=ADVANCED_FACE('',(#4436),#3661,.T.);
#15072=ADVANCED_FACE('',(#4437,#267),#685,.F.);
#15073=ADVANCED_FACE('',(#4438),#14310,.T.);
#15074=ADVANCED_FACE('',(#4439),#176,.T.);
#15075=ADVANCED_FACE('',(#4440),#686,.T.);
#15076=ADVANCED_FACE('',(#4441),#14311,.F.);
#15077=ADVANCED_FACE('',(#4442,#268),#687,.T.);
#15078=ADVANCED_FACE('',(#4443,#269,#270),#688,.F.);
#15079=ADVANCED_FACE('',(#4444),#14312,.F.);
#15080=ADVANCED_FACE('',(#4445),#3662,.T.);
#15081=ADVANCED_FACE('',(#4446),#3663,.F.);
#15082=ADVANCED_FACE('',(#4447),#96,.T.);
#15083=ADVANCED_FACE('',(#4448),#689,.T.);
#15084=ADVANCED_FACE('',(#4449),#690,.T.);
#15085=ADVANCED_FACE('',(#4450),#3664,.T.);
#15086=ADVANCED_FACE('',(#4451),#3665,.T.);
#15087=ADVANCED_FACE('',(#4452),#691,.T.);
#15088=ADVANCED_FACE('',(#4453),#177,.T.);
#15089=ADVANCED_FACE('',(#4454),#178,.T.);
#15090=ADVANCED_FACE('',(#4455),#3666,.T.);
#15091=ADVANCED_FACE('',(#4456),#179,.T.);
#15092=ADVANCED_FACE('',(#4457),#3667,.T.);
#15093=ADVANCED_FACE('',(#4458),#3668,.F.);
#15094=ADVANCED_FACE('',(#4459),#180,.F.);
#15095=ADVANCED_FACE('',(#4460),#181,.F.);
#15096=ADVANCED_FACE('',(#4461),#692,.T.);
#15097=ADVANCED_FACE('',(#4462),#693,.T.);
#15098=ADVANCED_FACE('',(#4463),#3669,.T.);
#15099=ADVANCED_FACE('',(#4464),#3670,.F.);
#15100=ADVANCED_FACE('',(#4465),#182,.F.);
#15101=ADVANCED_FACE('',(#4466),#694,.F.);
#15102=ADVANCED_FACE('',(#4467,#271,#272),#695,.T.);
#15103=ADVANCED_FACE('',(#4468),#696,.F.);
#15104=ADVANCED_FACE('',(#4469),#697,.T.);
#15105=ADVANCED_FACE('',(#4470),#698,.F.);
#15106=ADVANCED_FACE('',(#4471),#699,.T.);
#15107=ADVANCED_FACE('',(#4472),#700,.T.);
#15108=ADVANCED_FACE('',(#4473),#701,.F.);
#15109=ADVANCED_FACE('',(#4474),#702,.F.);
#15110=ADVANCED_FACE('',(#4475),#703,.F.);
#15111=ADVANCED_FACE('',(#4476),#704,.T.);
#15112=ADVANCED_FACE('',(#4477),#705,.T.);
#15113=ADVANCED_FACE('',(#4478),#706,.F.);
#15114=ADVANCED_FACE('',(#4479),#183,.F.);
#15115=ADVANCED_FACE('',(#4480),#184,.F.);
#15116=ADVANCED_FACE('',(#4481),#97,.F.);
#15117=ADVANCED_FACE('',(#4482),#3671,.F.);
#15118=ADVANCED_FACE('',(#4483),#14313,.F.);
#15119=ADVANCED_FACE('',(#4484),#3672,.T.);
#15120=ADVANCED_FACE('',(#4485),#3673,.F.);
#15121=ADVANCED_FACE('',(#4486),#185,.F.);
#15122=ADVANCED_FACE('',(#4487),#186,.F.);
#15123=ADVANCED_FACE('',(#4488),#3674,.T.);
#15124=ADVANCED_FACE('',(#4489),#3675,.T.);
#15125=ADVANCED_FACE('',(#4490),#3676,.F.);
#15126=ADVANCED_FACE('',(#4491),#3677,.T.);
#15127=ADVANCED_FACE('',(#4492),#3678,.T.);
#15128=ADVANCED_FACE('',(#4493),#3679,.T.);
#15129=ADVANCED_FACE('',(#4494),#3680,.T.);
#15130=ADVANCED_FACE('',(#4495),#14314,.T.);
#15131=ADVANCED_FACE('',(#4496),#3681,.T.);
#15132=ADVANCED_FACE('',(#4497),#14315,.T.);
#15133=ADVANCED_FACE('',(#4498),#3682,.T.);
#15134=ADVANCED_FACE('',(#4499),#187,.F.);
#15135=ADVANCED_FACE('',(#4500),#188,.F.);
#15136=ADVANCED_FACE('',(#4501,#273),#707,.F.);
#15137=ADVANCED_FACE('',(#4502),#14316,.F.);
#15138=ADVANCED_FACE('',(#4503),#189,.F.);
#15139=ADVANCED_FACE('',(#4504),#190,.F.);
#15140=ADVANCED_FACE('',(#4505),#191,.F.);
#15141=ADVANCED_FACE('',(#4506),#14317,.T.);
#15142=ADVANCED_FACE('',(#4507),#708,.F.);
#15143=ADVANCED_FACE('',(#4508),#709,.F.);
#15144=ADVANCED_FACE('',(#4509),#710,.F.);
#15145=ADVANCED_FACE('',(#4510),#711,.T.);
#15146=ADVANCED_FACE('',(#4511),#712,.F.);
#15147=ADVANCED_FACE('',(#4512),#3683,.F.);
#15148=ADVANCED_FACE('',(#4513,#274),#713,.F.);
#15200=CLOSED_SHELL('',(#14962,#14963,#14964,#14965,#14966,#14967,#14968,
#14969,#14970,#14971,#14972,#14973,#14974,#14975,#14976,#14977,#14978,#14979,
#14980,#14981,#14982,#14983,#14984,#14985,#14986,#14987,#14988,#14989,#14990,
#14991,#14992,#14993,#14994,#14995,#14996,#14997,#14998,#14999,#15000,#15001,
#15002,#15003,#15004,#15005,#15006,#15007,#15008,#15009,#15010,#15011,#15012,
#15013,#15014,#15015,#15016,#15017,#15018,#15019,#15020,#15021,#15022,#15023,
#15024,#15025,#15026,#15027,#15028,#15029,#15030,#15031,#15032,#15033,#15034,
#15035,#15036,#15037,#15038,#15039,#15040,#15041,#15042,#15043,#15044,#15045,
#15046,#15047,#15048,#15049,#15050,#15051,#15052,#15053,#15054,#15055,#15056,
#15057,#15058,#15059,#15060,#15061,#15062,#15063,#15064,#15065,#15066,#15067,
#15068,#15069,#15070,#15071,#15072,#15073,#15074,#15075,#15076,#15077,#15078,
#15079,#15080,#15081,#15082,#15083,#15084,#15085,#15086,#15087,#15088,#15089,
#15090,#15091,#15092,#15093,#15094,#15095,#15096,#15097,#15098,#15099,#15100,
#15101,#15102,#15103,#15104,#15105,#15106,#15107,#15108,#15109,#15110,#15111,
#15112,#15113,#15114,#15115,#15116,#15117,#15118,#15119,#15120,#15121,#15122,
#15123,#15124,#15125,#15126,#15127,#15128,#15129,#15130,#15131,#15132,#15133,
#15134,#15135,#15136,#15137,#15138,#15139,#15140,#15141,#15142,#15143,#15144,
#15145,#15146,#15147,#15148));
#16488=AXIS2_PLACEMENT_3D('',#45568,#20245,#20246);
#16489=AXIS2_PLACEMENT_3D('',#45569,#20247,#20248);
#16490=AXIS2_PLACEMENT_3D('',#45585,#20249,#20250);
#16491=AXIS2_PLACEMENT_3D('',#45587,#20251,#20252);
#16492=AXIS2_PLACEMENT_3D('',#45589,#20253,#20254);
#16493=AXIS2_PLACEMENT_3D('',#45591,#20255,#20256);
#16494=AXIS2_PLACEMENT_3D('',#45592,#20257,#20258);
#16495=AXIS2_PLACEMENT_3D('',#45593,#20259,#20260);
#16496=AXIS2_PLACEMENT_3D('',#45595,#20261,#20262);
#16497=AXIS2_PLACEMENT_3D('',#45598,#20264,#20265);
#16498=AXIS2_PLACEMENT_3D('',#45599,#20266,#20267);
#16499=AXIS2_PLACEMENT_3D('',#46088,#20269,#20270);
#16500=AXIS2_PLACEMENT_3D('',#46099,#20271,#20272);
#16501=AXIS2_PLACEMENT_3D('',#46111,#20273,#20274);
#16502=AXIS2_PLACEMENT_3D('',#46340,#20275,#20276);
#16503=AXIS2_PLACEMENT_3D('',#46343,#20277,#20278);
#16504=AXIS2_PLACEMENT_3D('',#46364,#20279,#20280);
#16505=AXIS2_PLACEMENT_3D('',#46366,#20281,#20282);
#16506=AXIS2_PLACEMENT_3D('',#46370,#20284,#20285);
#16507=AXIS2_PLACEMENT_3D('',#46656,#20286,#20287);
#16508=AXIS2_PLACEMENT_3D('',#46681,#20288,#20289);
#16509=AXIS2_PLACEMENT_3D('',#47026,#20290,#20291);
#16510=AXIS2_PLACEMENT_3D('',#47027,#20292,#20293);
#16511=AXIS2_PLACEMENT_3D('',#47029,#20294,#20295);
#16512=AXIS2_PLACEMENT_3D('',#47030,#20296,#20297);
#16513=AXIS2_PLACEMENT_3D('',#47031,#20298,#20299);
#16514=AXIS2_PLACEMENT_3D('',#47034,#20300,#20301);
#16515=AXIS2_PLACEMENT_3D('',#47038,#20303,#20304);
#16516=AXIS2_PLACEMENT_3D('',#48229,#20305,#20306);
#16517=AXIS2_PLACEMENT_3D('',#48367,#20307,#20308);
#16518=AXIS2_PLACEMENT_3D('',#48371,#20310,#20311);
#16519=AXIS2_PLACEMENT_3D('',#48398,#20312,#20313);
#16520=AXIS2_PLACEMENT_3D('',#48400,#20314,#20315);
#16521=AXIS2_PLACEMENT_3D('',#48566,#20316,#20317);
#16522=AXIS2_PLACEMENT_3D('',#48905,#20318,#20319);
#16523=AXIS2_PLACEMENT_3D('',#48907,#20320,#20321);
#16524=AXIS2_PLACEMENT_3D('',#48911,#20323,#20324);
#16525=AXIS2_PLACEMENT_3D('',#49046,#20326,#20327);
#16526=AXIS2_PLACEMENT_3D('',#49470,#20328,#20329);
#16527=AXIS2_PLACEMENT_3D('',#50107,#20330,#20331);
#16528=AXIS2_PLACEMENT_3D('',#50109,#20332,#20333);
#16529=AXIS2_PLACEMENT_3D('',#50110,#20334,#20335);
#16530=AXIS2_PLACEMENT_3D('',#50111,#20336,#20337);
#16531=AXIS2_PLACEMENT_3D('',#50242,#20339,#20340);
#16532=AXIS2_PLACEMENT_3D('',#50702,#20342,#20343);
#16533=AXIS2_PLACEMENT_3D('',#50705,#20344,#20345);
#16534=AXIS2_PLACEMENT_3D('',#50707,#20346,#20347);
#16535=AXIS2_PLACEMENT_3D('',#50709,#20348,#20349);
#16536=AXIS2_PLACEMENT_3D('',#50710,#20350,#20351);
#16537=AXIS2_PLACEMENT_3D('',#50711,#20352,#20353);
#16538=AXIS2_PLACEMENT_3D('',#50713,#20354,#20355);
#16539=AXIS2_PLACEMENT_3D('',#50714,#20356,#20357);
#16540=AXIS2_PLACEMENT_3D('',#51502,#20358,#20359);
#16541=AXIS2_PLACEMENT_3D('',#51504,#20360,#20361);
#16542=AXIS2_PLACEMENT_3D('',#51625,#20362,#20363);
#16543=AXIS2_PLACEMENT_3D('',#51626,#20364,#20365);
#16544=AXIS2_PLACEMENT_3D('',#51641,#20366,#20367);
#16545=AXIS2_PLACEMENT_3D('',#51642,#20368,#20369);
#16546=AXIS2_PLACEMENT_3D('',#51643,#20370,#20371);
#16547=AXIS2_PLACEMENT_3D('',#51645,#20372,#20373);
#16548=AXIS2_PLACEMENT_3D('',#51774,#20375,#20376);
#16549=AXIS2_PLACEMENT_3D('',#51775,#20377,#20378);
#16550=AXIS2_PLACEMENT_3D('',#52121,#20380,#20381);
#16551=AXIS2_PLACEMENT_3D('',#52123,#20383,#20384);
#16552=AXIS2_PLACEMENT_3D('',#52133,#20385,#20386);
#16553=AXIS2_PLACEMENT_3D('',#52135,#20387,#20388);
#16554=AXIS2_PLACEMENT_3D('',#52136,#20389,#20390);
#16555=AXIS2_PLACEMENT_3D('',#52137,#20391,#20392);
#16556=AXIS2_PLACEMENT_3D('',#52139,#20393,#20394);
#16557=AXIS2_PLACEMENT_3D('',#52142,#20396,#20397);
#16558=AXIS2_PLACEMENT_3D('',#53020,#20398,#20399);
#16559=AXIS2_PLACEMENT_3D('',#53420,#20400,#20401);
#16560=AXIS2_PLACEMENT_3D('',#53421,#20402,#20403);
#16561=AXIS2_PLACEMENT_3D('',#53422,#20404,#20405);
#16562=AXIS2_PLACEMENT_3D('',#53425,#20406,#20407);
#16563=AXIS2_PLACEMENT_3D('',#53427,#20408,#20409);
#16564=AXIS2_PLACEMENT_3D('',#53429,#20410,#20411);
#16565=AXIS2_PLACEMENT_3D('',#53430,#20412,#20413);
#16566=AXIS2_PLACEMENT_3D('',#53431,#20414,#20415);
#16567=AXIS2_PLACEMENT_3D('',#53434,#20416,#20417);
#16568=AXIS2_PLACEMENT_3D('',#53460,#20419,#20420);
#16569=AXIS2_PLACEMENT_3D('',#53484,#20422,#20423);
#16570=AXIS2_PLACEMENT_3D('',#53488,#20425,#20426);
#16571=AXIS2_PLACEMENT_3D('',#53490,#20428,#20429);
#16572=AXIS2_PLACEMENT_3D('',#53492,#20431,#20432);
#16573=AXIS2_PLACEMENT_3D('',#53567,#20433,#20434);
#16574=AXIS2_PLACEMENT_3D('',#53685,#20435,#20436);
#16575=AXIS2_PLACEMENT_3D('',#53710,#20438,#20439);
#16576=AXIS2_PLACEMENT_3D('',#53834,#20441,#20442);
#16577=AXIS2_PLACEMENT_3D('',#53837,#20443,#20444);
#16578=AXIS2_PLACEMENT_3D('',#54036,#20445,#20446);
#16579=AXIS2_PLACEMENT_3D('',#54037,#20447,#20448);
#16580=AXIS2_PLACEMENT_3D('',#54039,#20449,#20450);
#16581=AXIS2_PLACEMENT_3D('',#54065,#20452,#20453);
#16582=AXIS2_PLACEMENT_3D('',#54499,#20454,#20455);
#16583=AXIS2_PLACEMENT_3D('',#54502,#20456,#20457);
#16584=AXIS2_PLACEMENT_3D('',#54504,#20458,#20459);
#16585=AXIS2_PLACEMENT_3D('',#54505,#20460,#20461);
#16586=AXIS2_PLACEMENT_3D('',#54508,#20463,#20464);
#16587=AXIS2_PLACEMENT_3D('',#54509,#20465,#20466);
#16588=AXIS2_PLACEMENT_3D('',#54511,#20467,#20468);
#16589=AXIS2_PLACEMENT_3D('',#54514,#20470,#20471);
#16590=AXIS2_PLACEMENT_3D('',#54515,#20472,#20473);
#16591=AXIS2_PLACEMENT_3D('',#54517,#20474,#20475);
#16592=AXIS2_PLACEMENT_3D('',#54520,#20477,#20478);
#16593=AXIS2_PLACEMENT_3D('',#54521,#20479,#20480);
#16594=AXIS2_PLACEMENT_3D('',#54524,#20481,#20482);
#16595=AXIS2_PLACEMENT_3D('',#54526,#20483,#20484);
#16596=AXIS2_PLACEMENT_3D('',#54527,#20485,#20486);
#16597=AXIS2_PLACEMENT_3D('',#54528,#20487,#20488);
#16598=AXIS2_PLACEMENT_3D('',#54531,#20489,#20490);
#16599=AXIS2_PLACEMENT_3D('',#54535,#20492,#20493);
#16600=AXIS2_PLACEMENT_3D('',#54537,#20495,#20496);
#16601=AXIS2_PLACEMENT_3D('',#54539,#20497,#20498);
#16602=AXIS2_PLACEMENT_3D('',#54543,#20500,#20501);
#16603=AXIS2_PLACEMENT_3D('',#54545,#20503,#20504);
#16604=AXIS2_PLACEMENT_3D('',#54547,#20505,#20506);
#16605=AXIS2_PLACEMENT_3D('',#54548,#20507,#20508);
#16606=AXIS2_PLACEMENT_3D('',#54549,#20509,#20510);
#16607=AXIS2_PLACEMENT_3D('',#54552,#20511,#20512);
#16608=AXIS2_PLACEMENT_3D('',#54555,#20515,#20516);
#16609=AXIS2_PLACEMENT_3D('',#54557,#20517,#20518);
#16610=AXIS2_PLACEMENT_3D('',#54558,#20519,#20520);
#16611=AXIS2_PLACEMENT_3D('',#54559,#20521,#20522);
#16612=AXIS2_PLACEMENT_3D('',#54561,#20523,#20524);
#16613=AXIS2_PLACEMENT_3D('',#54564,#20526,#20527);
#16614=AXIS2_PLACEMENT_3D('',#54565,#20528,#20529);
#16615=AXIS2_PLACEMENT_3D('',#54691,#20531,#20532);
#16616=AXIS2_PLACEMENT_3D('',#54693,#20534,#20535);
#16617=AXIS2_PLACEMENT_3D('',#54694,#20536,#20537);
#16618=AXIS2_PLACEMENT_3D('',#54966,#20540,#20541);
#16619=AXIS2_PLACEMENT_3D('',#54968,#20542,#20543);
#16620=AXIS2_PLACEMENT_3D('',#54970,#20545,#20546);
#16621=AXIS2_PLACEMENT_3D('',#54973,#20548,#20549);
#16622=AXIS2_PLACEMENT_3D('',#54974,#20550,#20551);
#16623=AXIS2_PLACEMENT_3D('',#54978,#20553,#20554);
#16624=AXIS2_PLACEMENT_3D('',#54980,#20556,#20557);
#16625=AXIS2_PLACEMENT_3D('',#54982,#20558,#20559);
#16626=AXIS2_PLACEMENT_3D('',#54985,#20561,#20562);
#16627=AXIS2_PLACEMENT_3D('',#54986,#20563,#20564);
#16628=AXIS2_PLACEMENT_3D('',#55000,#20566,#20567);
#16629=AXIS2_PLACEMENT_3D('',#55001,#20568,#20569);
#16630=AXIS2_PLACEMENT_3D('',#55003,#20570,#20571);
#16631=AXIS2_PLACEMENT_3D('',#55006,#20573,#20574);
#16632=AXIS2_PLACEMENT_3D('',#55007,#20575,#20576);
#16633=AXIS2_PLACEMENT_3D('',#55009,#20577,#20578);
#16634=AXIS2_PLACEMENT_3D('',#55010,#20579,#20580);
#16635=AXIS2_PLACEMENT_3D('',#55011,#20581,#20582);
#16636=AXIS2_PLACEMENT_3D('',#55014,#20584,#20585);
#16637=AXIS2_PLACEMENT_3D('',#55015,#20586,#20587);
#16638=AXIS2_PLACEMENT_3D('',#55016,#20588,#20589);
#16639=AXIS2_PLACEMENT_3D('',#55017,#20590,#20591);
#16640=AXIS2_PLACEMENT_3D('',#55019,#20592,#20593);
#16641=AXIS2_PLACEMENT_3D('',#55022,#20595,#20596);
#16642=AXIS2_PLACEMENT_3D('',#55023,#20597,#20598);
#16643=AXIS2_PLACEMENT_3D('',#55025,#20599,#20600);
#16644=AXIS2_PLACEMENT_3D('',#55028,#20602,#20603);
#16645=AXIS2_PLACEMENT_3D('',#55029,#20604,#20605);
#16646=AXIS2_PLACEMENT_3D('',#55030,#20606,#20607);
#16647=AXIS2_PLACEMENT_3D('',#55031,#20608,#20609);
#16648=AXIS2_PLACEMENT_3D('',#55032,#20610,#20611);
#16649=AXIS2_PLACEMENT_3D('',#55103,#20613,#20614);
#16650=AXIS2_PLACEMENT_3D('',#55104,#20615,#20616);
#16651=AXIS2_PLACEMENT_3D('',#55118,#20618,#20619);
#16652=AXIS2_PLACEMENT_3D('',#55119,#20620,#20621);
#16653=AXIS2_PLACEMENT_3D('',#55125,#20625,#20626);
#16654=AXIS2_PLACEMENT_3D('',#55129,#20628,#20629);
#16655=AXIS2_PLACEMENT_3D('',#55130,#20630,#20631);
#16656=AXIS2_PLACEMENT_3D('',#55131,#20632,#20633);
#16657=AXIS2_PLACEMENT_3D('',#55134,#20634,#20635);
#16658=AXIS2_PLACEMENT_3D('',#55139,#20638,#20639);
#16659=AXIS2_PLACEMENT_3D('',#55141,#20641,#20642);
#16660=AXIS2_PLACEMENT_3D('',#55145,#20645,#20646);
#16661=AXIS2_PLACEMENT_3D('',#55148,#20648,#20649);
#16662=AXIS2_PLACEMENT_3D('',#55149,#20650,#20651);
#16663=AXIS2_PLACEMENT_3D('',#55153,#20654,#20655);
#16664=AXIS2_PLACEMENT_3D('',#55156,#20657,#20658);
#16665=AXIS2_PLACEMENT_3D('',#55157,#20659,#20660);
#16666=AXIS2_PLACEMENT_3D('',#55243,#20662,#20663);
#16667=AXIS2_PLACEMENT_3D('',#55353,#20664,#20665);
#16668=AXIS2_PLACEMENT_3D('',#55618,#20666,#20667);
#16669=AXIS2_PLACEMENT_3D('',#55632,#20668,#20669);
#16670=AXIS2_PLACEMENT_3D('',#55776,#20670,#20671);
#16671=AXIS2_PLACEMENT_3D('',#55883,#20672,#20673);
#16672=AXIS2_PLACEMENT_3D('',#55884,#20674,#20675);
#16673=AXIS2_PLACEMENT_3D('',#55885,#20676,#20677);
#16674=AXIS2_PLACEMENT_3D('',#56054,#20678,#20679);
#16675=AXIS2_PLACEMENT_3D('',#56055,#20680,#20681);
#16676=AXIS2_PLACEMENT_3D('',#56056,#20682,#20683);
#16677=AXIS2_PLACEMENT_3D('',#56058,#20684,#20685);
#16678=AXIS2_PLACEMENT_3D('',#56060,#20686,#20687);
#16679=AXIS2_PLACEMENT_3D('',#56061,#20688,#20689);
#16680=AXIS2_PLACEMENT_3D('',#56062,#20690,#20691);
#16681=AXIS2_PLACEMENT_3D('',#56065,#20692,#20693);
#16682=AXIS2_PLACEMENT_3D('',#56067,#20694,#20695);
#16683=AXIS2_PLACEMENT_3D('',#56068,#20696,#20697);
#16684=AXIS2_PLACEMENT_3D('',#56069,#20698,#20699);
#16685=AXIS2_PLACEMENT_3D('',#56072,#20702,#20703);
#16686=AXIS2_PLACEMENT_3D('',#56075,#20704,#20705);
#16687=AXIS2_PLACEMENT_3D('',#56078,#20708,#20709);
#16688=AXIS2_PLACEMENT_3D('',#56081,#20710,#20711);
#16689=AXIS2_PLACEMENT_3D('',#56083,#20712,#20713);
#16690=AXIS2_PLACEMENT_3D('',#56084,#20714,#20715);
#16691=AXIS2_PLACEMENT_3D('',#56085,#20716,#20717);
#16692=AXIS2_PLACEMENT_3D('',#56088,#20718,#20719);
#16693=AXIS2_PLACEMENT_3D('',#56091,#20722,#20723);
#16694=AXIS2_PLACEMENT_3D('',#56094,#20724,#20725);
#16695=AXIS2_PLACEMENT_3D('',#56097,#20728,#20729);
#16696=AXIS2_PLACEMENT_3D('',#56099,#20730,#20731);
#16697=AXIS2_PLACEMENT_3D('',#56100,#20732,#20733);
#16698=AXIS2_PLACEMENT_3D('',#56101,#20734,#20735);
#16699=AXIS2_PLACEMENT_3D('',#56104,#20736,#20737);
#16700=AXIS2_PLACEMENT_3D('',#56107,#20740,#20741);
#16701=AXIS2_PLACEMENT_3D('',#56110,#20742,#20743);
#16702=AXIS2_PLACEMENT_3D('',#56113,#20746,#20747);
#16703=AXIS2_PLACEMENT_3D('',#56115,#20748,#20749);
#16704=AXIS2_PLACEMENT_3D('',#56116,#20750,#20751);
#16705=AXIS2_PLACEMENT_3D('',#56117,#20752,#20753);
#16706=AXIS2_PLACEMENT_3D('',#56120,#20754,#20755);
#16707=AXIS2_PLACEMENT_3D('',#56123,#20758,#20759);
#16708=AXIS2_PLACEMENT_3D('',#56127,#20761,#20762);
#16709=AXIS2_PLACEMENT_3D('',#56129,#20764,#20765);
#16710=AXIS2_PLACEMENT_3D('',#56132,#20766,#20767);
#16711=AXIS2_PLACEMENT_3D('',#56134,#20768,#20769);
#16712=AXIS2_PLACEMENT_3D('',#56135,#20770,#20771);
#16713=AXIS2_PLACEMENT_3D('',#56136,#20772,#20773);
#16714=AXIS2_PLACEMENT_3D('',#56139,#20776,#20777);
#16715=AXIS2_PLACEMENT_3D('',#56142,#20778,#20779);
#16716=AXIS2_PLACEMENT_3D('',#56144,#20781,#20782);
#16717=AXIS2_PLACEMENT_3D('',#56146,#20784,#20785);
#16718=AXIS2_PLACEMENT_3D('',#56148,#20786,#20787);
#16719=AXIS2_PLACEMENT_3D('',#56149,#20788,#20789);
#16720=AXIS2_PLACEMENT_3D('',#56150,#20790,#20791);
#16721=AXIS2_PLACEMENT_3D('',#56153,#20794,#20795);
#16722=AXIS2_PLACEMENT_3D('',#56157,#20797,#20798);
#16723=AXIS2_PLACEMENT_3D('',#56159,#20800,#20801);
#16724=AXIS2_PLACEMENT_3D('',#56161,#20802,#20803);
#16725=AXIS2_PLACEMENT_3D('',#56164,#20806,#20807);
#16726=AXIS2_PLACEMENT_3D('',#56165,#20808,#20809);
#16727=AXIS2_PLACEMENT_3D('',#56166,#20810,#20811);
#16728=AXIS2_PLACEMENT_3D('',#56169,#20814,#20815);
#16729=AXIS2_PLACEMENT_3D('',#56173,#20817,#20818);
#16730=AXIS2_PLACEMENT_3D('',#56175,#20820,#20821);
#16731=AXIS2_PLACEMENT_3D('',#56176,#20822,#20823);
#16732=AXIS2_PLACEMENT_3D('',#56180,#20825,#20826);
#16733=AXIS2_PLACEMENT_3D('',#56182,#20828,#20829);
#16734=AXIS2_PLACEMENT_3D('',#56184,#20830,#20831);
#16735=AXIS2_PLACEMENT_3D('',#56185,#20832,#20833);
#16736=AXIS2_PLACEMENT_3D('',#56186,#20834,#20835);
#16737=AXIS2_PLACEMENT_3D('',#56188,#20836,#20837);
#16738=AXIS2_PLACEMENT_3D('',#56191,#20840,#20841);
#16739=AXIS2_PLACEMENT_3D('',#56194,#20844,#20845);
#16740=AXIS2_PLACEMENT_3D('',#56197,#20848,#20849);
#16741=AXIS2_PLACEMENT_3D('',#56201,#20851,#20852);
#16742=AXIS2_PLACEMENT_3D('',#56203,#20854,#20855);
#16743=AXIS2_PLACEMENT_3D('',#56205,#20857,#20858);
#16744=AXIS2_PLACEMENT_3D('',#56213,#20863,#20864);
#16745=AXIS2_PLACEMENT_3D('',#56214,#20865,#20866);
#16746=AXIS2_PLACEMENT_3D('',#56220,#20870,#20871);
#16747=AXIS2_PLACEMENT_3D('',#56225,#20873,#20874);
#16748=AXIS2_PLACEMENT_3D('',#56229,#20876,#20877);
#16749=AXIS2_PLACEMENT_3D('',#56232,#20880,#20881);
#16750=AXIS2_PLACEMENT_3D('',#56234,#20882,#20883);
#16751=AXIS2_PLACEMENT_3D('',#56236,#20884,#20885);
#16752=AXIS2_PLACEMENT_3D('',#56240,#20888,#20889);
#16753=AXIS2_PLACEMENT_3D('',#56246,#20890,#20891);
#16754=AXIS2_PLACEMENT_3D('',#56247,#20892,#20893);
#16755=AXIS2_PLACEMENT_3D('',#56253,#20897,#20898);
#16756=AXIS2_PLACEMENT_3D('',#56257,#20901,#20902);
#16757=AXIS2_PLACEMENT_3D('',#56258,#20903,#20904);
#16758=AXIS2_PLACEMENT_3D('',#56259,#20905,#20906);
#16759=AXIS2_PLACEMENT_3D('',#56260,#20907,#20908);
#16760=AXIS2_PLACEMENT_3D('',#56261,#20909,#20910);
#16761=AXIS2_PLACEMENT_3D('',#56262,#20911,#20912);
#16762=AXIS2_PLACEMENT_3D('',#56264,#20913,#20914);
#16763=AXIS2_PLACEMENT_3D('',#56266,#20915,#20916);
#16764=AXIS2_PLACEMENT_3D('',#56267,#20917,#20918);
#16765=AXIS2_PLACEMENT_3D('',#56395,#20919,#20920);
#16766=AXIS2_PLACEMENT_3D('',#56397,#20921,#20922);
#16767=AXIS2_PLACEMENT_3D('',#56405,#20924,#20925);
#16768=AXIS2_PLACEMENT_3D('',#56442,#20926,#20927);
#16769=AXIS2_PLACEMENT_3D('',#56443,#20928,#20929);
#16770=AXIS2_PLACEMENT_3D('',#56444,#20930,#20931);
#16771=AXIS2_PLACEMENT_3D('',#56445,#20932,#20933);
#16772=AXIS2_PLACEMENT_3D('',#56447,#20934,#20935);
#16773=AXIS2_PLACEMENT_3D('',#56449,#20936,#20937);
#16774=AXIS2_PLACEMENT_3D('',#56450,#20938,#20939);
#16775=AXIS2_PLACEMENT_3D('',#56451,#20940,#20941);
#16776=AXIS2_PLACEMENT_3D('',#56453,#20943,#20944);
#16777=AXIS2_PLACEMENT_3D('',#56455,#20946,#20947);
#16778=AXIS2_PLACEMENT_3D('',#56457,#20949,#20950);
#16779=AXIS2_PLACEMENT_3D('',#56458,#20951,#20952);
#16780=AXIS2_PLACEMENT_3D('',#56461,#20955,#20956);
#16781=AXIS2_PLACEMENT_3D('',#56462,#20957,#20958);
#16782=AXIS2_PLACEMENT_3D('',#56466,#20960,#20961);
#16783=AXIS2_PLACEMENT_3D('',#56468,#20963,#20964);
#16784=AXIS2_PLACEMENT_3D('',#56471,#20967,#20968);
#16785=AXIS2_PLACEMENT_3D('',#56961,#20969,#20970);
#16786=AXIS2_PLACEMENT_3D('',#57046,#20971,#20972);
#16787=AXIS2_PLACEMENT_3D('',#57273,#20975,#20976);
#16788=AXIS2_PLACEMENT_3D('',#58841,#20977,#20978);
#16789=AXIS2_PLACEMENT_3D('',#58850,#20979,#20980);
#16790=AXIS2_PLACEMENT_3D('',#58851,#20981,#20982);
#16791=AXIS2_PLACEMENT_3D('',#58854,#20985,#20986);
#16792=AXIS2_PLACEMENT_3D('',#58855,#20987,#20988);
#16793=AXIS2_PLACEMENT_3D('',#58858,#20990,#20991);
#16794=AXIS2_PLACEMENT_3D('',#58859,#20992,#20993);
#16795=AXIS2_PLACEMENT_3D('',#58861,#20994,#20995);
#16796=AXIS2_PLACEMENT_3D('',#58992,#20997,#20998);
#16797=AXIS2_PLACEMENT_3D('',#58993,#20999,#21000);
#16798=AXIS2_PLACEMENT_3D('',#58998,#21004,#21005);
#16799=AXIS2_PLACEMENT_3D('',#59004,#21009,#21010);
#16800=AXIS2_PLACEMENT_3D('',#59011,#21014,#21015);
#16801=AXIS2_PLACEMENT_3D('',#59014,#21017,#21018);
#16802=AXIS2_PLACEMENT_3D('',#59015,#21019,#21020);
#16803=AXIS2_PLACEMENT_3D('',#59016,#21021,#21022);
#16804=AXIS2_PLACEMENT_3D('',#59017,#21023,#21024);
#16805=AXIS2_PLACEMENT_3D('',#59023,#21028,#21029);
#16806=AXIS2_PLACEMENT_3D('',#59024,#21030,#21031);
#16807=AXIS2_PLACEMENT_3D('',#59025,#21032,#21033);
#16808=AXIS2_PLACEMENT_3D('',#59027,#21035,#21036);
#16809=AXIS2_PLACEMENT_3D('',#59028,#21037,#21038);
#16810=AXIS2_PLACEMENT_3D('',#59029,#21039,#21040);
#16811=AXIS2_PLACEMENT_3D('',#59033,#21042,#21043);
#16812=AXIS2_PLACEMENT_3D('',#59035,#21045,#21046);
#16813=AXIS2_PLACEMENT_3D('',#59036,#21047,#21048);
#16814=AXIS2_PLACEMENT_3D('',#59041,#21052,#21053);
#16815=AXIS2_PLACEMENT_3D('',#59052,#21056,#21057);
#16816=AXIS2_PLACEMENT_3D('',#59661,#21058,#21059);
#16817=AXIS2_PLACEMENT_3D('',#59662,#21060,#21061);
#16818=AXIS2_PLACEMENT_3D('',#59663,#21062,#21063);
#16819=AXIS2_PLACEMENT_3D('',#59664,#21064,#21065);
#16820=AXIS2_PLACEMENT_3D('',#59673,#21066,#21067);
#16821=AXIS2_PLACEMENT_3D('',#59674,#21068,#21069);
#16822=AXIS2_PLACEMENT_3D('',#59675,#21070,#21071);
#16823=AXIS2_PLACEMENT_3D('',#59770,#21072,#21073);
#16824=AXIS2_PLACEMENT_3D('',#59771,#21074,#21075);
#16825=AXIS2_PLACEMENT_3D('',#60708,#21076,#21077);
#16826=AXIS2_PLACEMENT_3D('',#60709,#21078,#21079);
#16827=AXIS2_PLACEMENT_3D('',#60710,#21080,#21081);
#16828=AXIS2_PLACEMENT_3D('',#60711,#21082,#21083);
#16829=AXIS2_PLACEMENT_3D('',#60726,#21085,#21086);
#16830=AXIS2_PLACEMENT_3D('',#60727,#21087,#21088);
#16831=AXIS2_PLACEMENT_3D('',#60728,#21089,#21090);
#16832=AXIS2_PLACEMENT_3D('',#60729,#21091,#21092);
#16833=AXIS2_PLACEMENT_3D('',#60730,#21093,#21094);
#16834=AXIS2_PLACEMENT_3D('',#60731,#21095,#21096);
#16835=AXIS2_PLACEMENT_3D('',#60732,#21097,#21098);
#16836=AXIS2_PLACEMENT_3D('',#60733,#21099,#21100);
#16837=AXIS2_PLACEMENT_3D('',#60734,#21101,#21102);
#16838=AXIS2_PLACEMENT_3D('',#60735,#21103,#21104);
#16839=AXIS2_PLACEMENT_3D('',#60736,#21105,#21106);
#16840=AXIS2_PLACEMENT_3D('',#60737,#21107,#21108);
#16841=AXIS2_PLACEMENT_3D('',#61909,#21109,#21110);
#16842=AXIS2_PLACEMENT_3D('',#61910,#21111,#21112);
#16843=AXIS2_PLACEMENT_3D('',#62259,#21113,#21114);
#16844=AXIS2_PLACEMENT_3D('',#62296,#21115,#21116);
#16845=AXIS2_PLACEMENT_3D('',#62603,#21117,#21118);
#16846=AXIS2_PLACEMENT_3D('',#62626,#21119,#21120);
#16847=AXIS2_PLACEMENT_3D('',#62627,#21121,#21122);
#16848=AXIS2_PLACEMENT_3D('',#62628,#21123,#21124);
#16849=AXIS2_PLACEMENT_3D('',#62629,#21125,#21126);
#16850=AXIS2_PLACEMENT_3D('',#62631,#21128,#21129);
#16851=AXIS2_PLACEMENT_3D('',#62632,#21130,#21131);
#16852=AXIS2_PLACEMENT_3D('',#62636,#21133,#21134);
#16853=AXIS2_PLACEMENT_3D('',#62638,#21136,#21137);
#16854=AXIS2_PLACEMENT_3D('',#62639,#21138,#21139);
#16855=AXIS2_PLACEMENT_3D('',#62640,#21140,#21141);
#20245=DIRECTION('axis',(0.,0.,1.));
#20246=DIRECTION('refdir',(1.,0.,0.));
#20247=DIRECTION('center_axis',(0.,-1.,0.));
#20248=DIRECTION('ref_axis',(0.,0.,-1.));
#20249=DIRECTION('center_axis',(0.616244820322966,0.0279867525047081,-0.787057217176334));
#20250=DIRECTION('ref_axis',(0.787551815229396,-0.0245787495049397,0.615758088376967));
#20251=DIRECTION('center_axis',(0.,1.,0.));
#20252=DIRECTION('ref_axis',(0.,0.,1.));
#20253=DIRECTION('center_axis',(0.0586169709474566,1.30991163966162E-16,
0.998280547099334));
#20254=DIRECTION('ref_axis',(0.998280547099334,-9.82981897176464E-33,-0.0586169709474566));
#20255=DIRECTION('center_axis',(0.0586169709474566,1.30991163966162E-16,
0.998280547099334));
#20256=DIRECTION('ref_axis',(0.998280547099334,-9.82981897176464E-33,-0.0586169709474566));
#20257=DIRECTION('center_axis',(0.,-1.,0.));
#20258=DIRECTION('ref_axis',(0.,0.,1.));
#20259=DIRECTION('center_axis',(0.,1.,0.));
#20260=DIRECTION('ref_axis',(0.,0.,-1.));
#20261=DIRECTION('center_axis',(-6.12303176911189E-17,-1.,3.41304790901886E-16));
#20262=DIRECTION('ref_axis',(-8.90039129279581E-34,3.41304790901886E-16,
1.));
#20263=DIRECTION('',(0.,-1.,0.));
#20264=DIRECTION('center_axis',(6.12303176911189E-17,1.,-3.41304790901886E-16));
#20265=DIRECTION('ref_axis',(2.09156632226363E-34,-3.41304790901886E-16,
-1.));
#20266=DIRECTION('center_axis',(1.,-6.12303176911189E-17,0.));
#20267=DIRECTION('ref_axis',(6.12303176911189E-17,1.,0.));
#20268=DIRECTION('',(-0.999877952034695,0.0156230930005404,1.91327708358932E-18));
#20269=DIRECTION('center_axis',(1.,-6.12303176911189E-17,0.));
#20270=DIRECTION('ref_axis',(6.12303176911189E-17,1.,0.));
#20271=DIRECTION('center_axis',(1.,-6.12303176911189E-17,0.));
#20272=DIRECTION('ref_axis',(6.12303176911189E-17,1.,0.));
#20273=DIRECTION('center_axis',(1.,-6.12303176911189E-17,0.));
#20274=DIRECTION('ref_axis',(6.12303176911189E-17,1.,0.));
#20275=DIRECTION('center_axis',(1.,0.,0.));
#20276=DIRECTION('ref_axis',(0.,0.,-1.));
#20277=DIRECTION('center_axis',(-1.,0.,0.));
#20278=DIRECTION('ref_axis',(0.,0.,-1.));
#20279=DIRECTION('center_axis',(0.,-1.,0.));
#20280=DIRECTION('ref_axis',(0.,0.,-1.));
#20281=DIRECTION('center_axis',(0.,1.,0.));
#20282=DIRECTION('ref_axis',(0.,0.,-1.));
#20283=DIRECTION('',(4.30002198846826E-17,0.936329177569045,-0.351123441588391));
#20284=DIRECTION('center_axis',(0.,-1.,0.));
#20285=DIRECTION('ref_axis',(0.,0.,-1.));
#20286=DIRECTION('center_axis',(0.,-1.,0.));
#20287=DIRECTION('ref_axis',(0.,0.,-1.));
#20288=DIRECTION('center_axis',(0.,-1.,0.));
#20289=DIRECTION('ref_axis',(0.,0.,-1.));
#20290=DIRECTION('center_axis',(0.,-1.,0.));
#20291=DIRECTION('ref_axis',(0.,0.,-1.));
#20292=DIRECTION('center_axis',(0.,-1.,0.));
#20293=DIRECTION('ref_axis',(0.,0.,-1.));
#20294=DIRECTION('center_axis',(0.,-1.,0.));
#20295=DIRECTION('ref_axis',(0.,0.,-1.));
#20296=DIRECTION('center_axis',(-1.,0.,-1.22464679914735E-16));
#20297=DIRECTION('ref_axis',(-1.22464679914735E-16,0.,1.));
#20298=DIRECTION('center_axis',(0.,1.,0.));
#20299=DIRECTION('ref_axis',(0.,0.,-1.));
#20300=DIRECTION('center_axis',(0.,-1.,0.));
#20301=DIRECTION('ref_axis',(0.,0.,-1.));
#20302=DIRECTION('',(0.,-1.,0.));
#20303=DIRECTION('center_axis',(0.,1.,0.));
#20304=DIRECTION('ref_axis',(0.,0.,1.));
#20305=DIRECTION('center_axis',(0.,1.,0.));
#20306=DIRECTION('ref_axis',(0.,0.,1.));
#20307=DIRECTION('center_axis',(0.,1.,0.));
#20308=DIRECTION('ref_axis',(0.,0.,-1.));
#20309=DIRECTION('',(0.,1.,0.));
#20310=DIRECTION('center_axis',(0.,1.,0.));
#20311=DIRECTION('ref_axis',(0.,0.,-1.));
#20312=DIRECTION('center_axis',(-0.0992537560260724,-0.0678968120752535,
0.992743025573454));
#20313=DIRECTION('ref_axis',(-0.78073602976301,-0.613230529687184,-0.119998205359365));
#20314=DIRECTION('center_axis',(0.,1.,0.));
#20315=DIRECTION('ref_axis',(0.,0.,1.));
#20316=DIRECTION('center_axis',(0.,1.,0.));
#20317=DIRECTION('ref_axis',(0.,0.,-1.));
#20318=DIRECTION('center_axis',(0.,1.,0.));
#20319=DIRECTION('ref_axis',(0.,0.,1.));
#20320=DIRECTION('center_axis',(0.,-1.,0.));
#20321=DIRECTION('ref_axis',(0.,0.,-1.));
#20322=DIRECTION('',(0.,-1.,0.));
#20323=DIRECTION('center_axis',(0.,-1.,-3.65204942310907E-16));
#20324=DIRECTION('ref_axis',(0.,-3.65204942310907E-16,1.));
#20325=DIRECTION('',(0.,1.,0.));
#20326=DIRECTION('center_axis',(-0.0235708115402593,-0.177622508721337,
0.983816375772874));
#20327=DIRECTION('ref_axis',(-0.0102596870461854,-0.983994984048997,-0.177900562641405));
#20328=DIRECTION('center_axis',(-0.0365025544384845,0.274626243368348,0.960857944741497));
#20329=DIRECTION('ref_axis',(-0.126726318578374,0.952464399007476,-0.277041529022093));
#20330=DIRECTION('center_axis',(-6.12303176911189E-17,-1.,3.41304790901886E-16));
#20331=DIRECTION('ref_axis',(0.,-3.41393580072236E-16,-1.));
#20332=DIRECTION('center_axis',(0.,1.,0.));
#20333=DIRECTION('ref_axis',(1.,0.,0.));
#20334=DIRECTION('center_axis',(-1.,6.12303176911189E-17,-1.22464679914735E-16));
#20335=DIRECTION('ref_axis',(-1.22464679914735E-16,3.40005801291454E-16,
1.));
#20336=DIRECTION('center_axis',(1.,0.,0.));
#20337=DIRECTION('ref_axis',(0.,-0.919145030018057,0.393919298579168));
#20338=DIRECTION('',(1.,0.,0.));
#20339=DIRECTION('center_axis',(-1.,6.12303176911189E-17,0.));
#20340=DIRECTION('ref_axis',(6.12303176911189E-17,1.,0.));
#20341=DIRECTION('',(-1.,0.,0.));
#20342=DIRECTION('center_axis',(0.,-1.,0.));
#20343=DIRECTION('ref_axis',(0.,0.,-1.));
#20344=DIRECTION('center_axis',(0.,1.,0.));
#20345=DIRECTION('ref_axis',(0.,0.,-1.));
#20346=DIRECTION('center_axis',(0.645833333333334,0.,0.763478425075362));
#20347=DIRECTION('ref_axis',(0.763478425075362,0.,-0.645833333333334));
#20348=DIRECTION('center_axis',(0.,-1.,0.));
#20349=DIRECTION('ref_axis',(0.,0.,-1.));
#20350=DIRECTION('center_axis',(-0.645833333333332,3.20901901721091E-15,
0.763478425075363));
#20351=DIRECTION('ref_axis',(0.763478425075363,1.69290416562703E-30,0.645833333333332));
#20352=DIRECTION('center_axis',(-6.12303176911189E-17,-1.,3.41304790901886E-16));
#20353=DIRECTION('ref_axis',(0.,-3.5527136788005E-16,-1.));
#20354=DIRECTION('center_axis',(-1.,6.12303176911189E-17,-1.22464679914735E-16));
#20355=DIRECTION('ref_axis',(-1.22464679914735E-16,3.33066907387547E-16,
1.));
#20356=DIRECTION('center_axis',(6.12303176911189E-17,1.,-3.41304790901886E-16));
#20357=DIRECTION('ref_axis',(8.90039129279581E-34,-3.41304790901886E-16,
-1.));
#20358=DIRECTION('center_axis',(-0.0528173258599627,0.994670318915973,-0.0885510404038205));
#20359=DIRECTION('ref_axis',(5.77315972805033E-14,-0.0886748135151963,-0.996060629403675));
#20360=DIRECTION('center_axis',(-0.830210692183039,-5.0361934159377E-5,
0.557449732306542));
#20361=DIRECTION('ref_axis',(0.554262125429395,0.106713543884745,0.825473025522971));
#20362=DIRECTION('center_axis',(-0.0514510747169759,-0.994945252858774,
0.0862364814000291));
#20363=DIRECTION('ref_axis',(-6.66133814775061E-14,0.0863508516932711,0.996264789306461));
#20364=DIRECTION('center_axis',(0.,-1.,0.));
#20365=DIRECTION('ref_axis',(0.491127762261646,0.,0.87108755078687));
#20366=DIRECTION('center_axis',(0.,1.,0.));
#20367=DIRECTION('ref_axis',(0.,0.,-1.));
#20368=DIRECTION('center_axis',(0.777751862218069,-1.11075125232563E-14,
-0.628571428571428));
#20369=DIRECTION('ref_axis',(0.628571428571428,-5.32211583197118E-30,0.777751862218069));
#20370=DIRECTION('center_axis',(-1.,0.,0.));
#20371=DIRECTION('ref_axis',(0.,0.,-1.));
#20372=DIRECTION('center_axis',(-1.,6.12303176911189E-17,0.));
#20373=DIRECTION('ref_axis',(6.12303176911189E-17,1.,0.));
#20374=DIRECTION('',(1.,0.,0.));
#20375=DIRECTION('center_axis',(-0.830143860196626,4.61445617944268E-5,
-0.557549252755776));
#20376=DIRECTION('ref_axis',(0.554525958306133,-0.103929478609263,-0.825651031029861));
#20377=DIRECTION('center_axis',(1.,0.,0.));
#20378=DIRECTION('ref_axis',(0.,0.919145030018077,-0.393919298579124));
#20379=DIRECTION('',(1.,0.,0.));
#20380=DIRECTION('center_axis',(-1.,6.12303176911189E-17,0.));
#20381=DIRECTION('ref_axis',(6.12303176911189E-17,1.,0.));
#20382=DIRECTION('',(-1.,0.,0.));
#20383=DIRECTION('center_axis',(-1.,6.12303176911189E-17,0.));
#20384=DIRECTION('ref_axis',(0.,-1.,0.));
#20385=DIRECTION('center_axis',(1.,-6.12303176911189E-17,0.));
#20386=DIRECTION('ref_axis',(-6.12303176911189E-17,-1.,0.));
#20387=DIRECTION('center_axis',(0.,0.844082777626921,-0.536212891036408));
#20388=DIRECTION('ref_axis',(0.,0.536212891036408,0.844082777626921));
#20389=DIRECTION('center_axis',(-1.,6.12303176911189E-17,0.));
#20390=DIRECTION('ref_axis',(-6.12303176911189E-17,-1.,0.));
#20391=DIRECTION('center_axis',(6.12303176911189E-17,1.,-5.4780741346636E-16));
#20392=DIRECTION('ref_axis',(-4.24099588001204E-33,-5.4780741346636E-16,
-1.));
#20393=DIRECTION('center_axis',(-6.12303176911189E-17,-1.,5.4780741346636E-16));
#20394=DIRECTION('ref_axis',(-4.24099588001204E-33,-5.4780741346636E-16,
-1.));
#20395=DIRECTION('',(6.12303176911189E-17,1.,-5.4780741346636E-16));
#20396=DIRECTION('center_axis',(-6.12303176911189E-17,-1.,5.4780741346636E-16));
#20397=DIRECTION('ref_axis',(-4.24099588001204E-33,-5.4780741346636E-16,
-1.));
#20398=DIRECTION('center_axis',(-0.993081091300346,-0.108852122504348,-0.0440586146855738));
#20399=DIRECTION('ref_axis',(-0.0460861135957196,0.706355459430216,-0.706355459430145));
#20400=DIRECTION('center_axis',(0.0392783824307495,-0.24484604714314,-0.968766030510981));
#20401=DIRECTION('ref_axis',(-0.0234136567132537,0.969022486825046,-0.245860164944867));
#20402=DIRECTION('center_axis',(0.997833402867506,0.0628604513358008,0.0194181301806716));
#20403=DIRECTION('ref_axis',(0.0307704812544108,-0.706771949600093,0.706771949600333));
#20404=DIRECTION('center_axis',(1.,-6.12303176911189E-17,0.));
#20405=DIRECTION('ref_axis',(0.,1.,0.));
#20406=DIRECTION('center_axis',(-1.,6.12303176911189E-17,0.));
#20407=DIRECTION('ref_axis',(6.12303176911189E-17,1.,0.));
#20408=DIRECTION('center_axis',(5.76857827429812E-17,0.942111439531992,
-0.335299918733898));
#20409=DIRECTION('ref_axis',(8.70539504324123E-32,-0.335299918733898,-0.942111439531992));
#20410=DIRECTION('center_axis',(1.,-6.12303176911189E-17,0.));
#20411=DIRECTION('ref_axis',(6.12303176911189E-17,1.,0.));
#20412=DIRECTION('center_axis',(0.,-0.942111439531976,-0.335299918733941));
#20413=DIRECTION('ref_axis',(0.,0.335299918733941,-0.942111439531976));
#20414=DIRECTION('center_axis',(0.,-0.844082777626919,0.53621289103641));
#20415=DIRECTION('ref_axis',(1.,1.81846874723086E-15,2.82341200227949E-15));
#20416=DIRECTION('center_axis',(0.,-0.844082777626919,0.53621289103641));
#20417=DIRECTION('ref_axis',(-1.,0.,0.));
#20418=DIRECTION('',(0.,0.844082777626919,-0.53621289103641));
#20419=DIRECTION('center_axis',(0.,-0.844082777626919,0.53621289103641));
#20420=DIRECTION('ref_axis',(0.,0.53621289103641,0.844082777626919));
#20421=DIRECTION('',(0.,0.844082777626919,-0.53621289103641));
#20422=DIRECTION('center_axis',(-1.,-3.40699396374318E-16,-5.3631402309558E-16));
#20423=DIRECTION('ref_axis',(5.3631402309558E-16,1.82721863935746E-31,-1.));
#20424=DIRECTION('',(1.,3.40699396374318E-16,5.3631402309558E-16));
#20425=DIRECTION('center_axis',(-0.707106781186508,0.379159771411456,0.596856655942839));
#20426=DIRECTION('ref_axis',(0.707106781186587,0.379159771411817,0.596856655942516));
#20427=DIRECTION('',(-1.,-3.40699396374318E-16,-5.3631402309558E-16));
#20428=DIRECTION('center_axis',(0.,1.,0.));
#20429=DIRECTION('ref_axis',(0.,0.,-1.));
#20430=DIRECTION('',(0.,-1.,0.));
#20431=DIRECTION('center_axis',(0.,1.,0.));
#20432=DIRECTION('ref_axis',(0.,0.,1.));
#20433=DIRECTION('center_axis',(-1.,0.,0.));
#20434=DIRECTION('ref_axis',(0.,0.,-1.));
#20435=DIRECTION('center_axis',(-1.,6.12303176911189E-17,0.));
#20436=DIRECTION('ref_axis',(6.12303176911189E-17,1.,0.));
#20437=DIRECTION('',(1.,0.,0.));
#20438=DIRECTION('center_axis',(1.,-6.12303176911189E-17,0.));
#20439=DIRECTION('ref_axis',(6.12303176911189E-17,1.,0.));
#20440=DIRECTION('',(1.,0.,0.));
#20441=DIRECTION('center_axis',(0.,0.,1.));
#20442=DIRECTION('ref_axis',(0.502661025164392,0.864483599486238,0.));
#20443=DIRECTION('center_axis',(0.,0.,-1.));
#20444=DIRECTION('ref_axis',(1.,0.,0.));
#20445=DIRECTION('center_axis',(8.47625784656822E-14,0.707106781186507,
0.707106781186588));
#20446=DIRECTION('ref_axis',(-2.64990011864105E-13,-0.707106781186588,0.707106781186507));
#20447=DIRECTION('center_axis',(0.,0.707106781186548,0.707106781186548));
#20448=DIRECTION('ref_axis',(0.,0.707106781186548,-0.707106781186548));
#20449=DIRECTION('center_axis',(0.0242120578352017,0.225844330253542,-0.973862472193951));
#20450=DIRECTION('ref_axis',(0.0389083137551034,-0.973622857458564,-0.224821428149));
#20451=DIRECTION('',(0.,-0.707106781186548,-0.707106781186548));
#20452=DIRECTION('center_axis',(1.96528009851118E-14,-1.,-3.48447557928277E-14));
#20453=DIRECTION('ref_axis',(8.37468481768744E-12,3.48447557929923E-14,
-1.));
#20454=DIRECTION('center_axis',(0.,0.,1.));
#20455=DIRECTION('ref_axis',(-1.,0.,0.));
#20456=DIRECTION('center_axis',(0.,0.,1.));
#20457=DIRECTION('ref_axis',(-1.,0.,0.));
#20458=DIRECTION('center_axis',(0.,-0.707106781186553,-0.707106781186542));
#20459=DIRECTION('ref_axis',(-1.91958678679309E-15,0.707106781186542,-0.707106781186553));
#20460=DIRECTION('center_axis',(0.,0.,1.));
#20461=DIRECTION('ref_axis',(-1.,0.,0.));
#20462=DIRECTION('',(0.,0.,1.));
#20463=DIRECTION('center_axis',(0.,0.,1.));
#20464=DIRECTION('ref_axis',(-1.,0.,0.));
#20465=DIRECTION('center_axis',(0.,0.,1.));
#20466=DIRECTION('ref_axis',(-1.,0.,0.));
#20467=DIRECTION('center_axis',(0.,0.,-1.));
#20468=DIRECTION('ref_axis',(1.,0.,0.));
#20469=DIRECTION('',(0.,0.,1.));
#20470=DIRECTION('center_axis',(0.,0.,-1.));
#20471=DIRECTION('ref_axis',(-1.,0.,0.));
#20472=DIRECTION('center_axis',(6.12303176911189E-17,1.,-5.4780741346636E-16));
#20473=DIRECTION('ref_axis',(-9.26409749374061E-33,-5.4780741346636E-16,
-1.));
#20474=DIRECTION('center_axis',(-6.12303176911189E-17,-1.,5.4780741346636E-16));
#20475=DIRECTION('ref_axis',(1.47760280201776E-47,-5.4780741346636E-16,
-1.));
#20476=DIRECTION('',(6.12303176911189E-17,1.,-5.4780741346636E-16));
#20477=DIRECTION('center_axis',(-6.12303176911189E-17,-1.,5.4780741346636E-16));
#20478=DIRECTION('ref_axis',(2.87506473943675E-33,-5.4780741346636E-16,
-1.));
#20479=DIRECTION('center_axis',(0.,1.,0.));
#20480=DIRECTION('ref_axis',(1.,0.,0.));
#20481=DIRECTION('center_axis',(-1.17140016801371E-14,-0.844082777626922,
0.536212891036405));
#20482=DIRECTION('ref_axis',(-7.91994057259303E-30,-0.536212891036405,-0.844082777626922));
#20483=DIRECTION('center_axis',(0.,-0.536212891036385,-0.844082777626935));
#20484=DIRECTION('ref_axis',(0.,-0.844082777626935,0.536212891036385));
#20485=DIRECTION('center_axis',(-0.707106781186563,-0.379159771411482,-0.596856655942757));
#20486=DIRECTION('ref_axis',(-0.645019472682982,9.40542767458206E-16,0.764166133677598));
#20487=DIRECTION('center_axis',(-1.,0.,0.));
#20488=DIRECTION('ref_axis',(0.,0.,-1.));
#20489=DIRECTION('center_axis',(-1.,0.,0.));
#20490=DIRECTION('ref_axis',(0.,0.,-1.));
#20491=DIRECTION('',(1.,0.,0.));
#20492=DIRECTION('center_axis',(-1.,0.,0.));
#20493=DIRECTION('ref_axis',(0.,0.,1.));
#20494=DIRECTION('',(-1.,0.,0.));
#20495=DIRECTION('center_axis',(-0.707106781186547,0.379159771411489,0.596856655942772));
#20496=DIRECTION('ref_axis',(-0.645019472683,-1.15352107484122E-15,-0.764166133677583));
#20497=DIRECTION('center_axis',(-0.707106781186548,0.379159771411488,0.596856655942771));
#20498=DIRECTION('ref_axis',(-0.645019472682999,-1.68179175522602E-15,-0.764166133677584));
#20499=DIRECTION('',(0.707106781186547,-0.379159771411489,-0.596856655942772));
#20500=DIRECTION('center_axis',(-0.707106781186554,0.379159771411484,0.596856655942767));
#20501=DIRECTION('ref_axis',(0.645019472682992,-2.55583619520875E-15,0.76416613367759));
#20502=DIRECTION('',(-0.707106781186547,0.379159771411489,0.596856655942772));
#20503=DIRECTION('center_axis',(0.,1.,0.));
#20504=DIRECTION('ref_axis',(1.,0.,0.));
#20505=DIRECTION('center_axis',(-1.1714001680137E-14,0.84408277762692,-0.536212891036409));
#20506=DIRECTION('ref_axis',(-1.67319991007564E-29,0.536212891036409,0.84408277762692));
#20507=DIRECTION('center_axis',(0.,0.536212891036392,0.844082777626931));
#20508=DIRECTION('ref_axis',(0.,0.844082777626931,-0.536212891036392));
#20509=DIRECTION('center_axis',(1.,0.,0.));
#20510=DIRECTION('ref_axis',(0.,0.,1.));
#20511=DIRECTION('center_axis',(-0.707106781186233,-0.379159771411426,-0.596856655943184));
#20512=DIRECTION('ref_axis',(0.707106781186862,-0.379159771413722,-0.59685665594098));
#20513=DIRECTION('',(-1.,0.,0.));
#20514=DIRECTION('',(1.,0.,0.));
#20515=DIRECTION('center_axis',(0.,1.,0.));
#20516=DIRECTION('ref_axis',(1.,0.,0.));
#20517=DIRECTION('center_axis',(0.,-0.536212891036408,-0.844082777626921));
#20518=DIRECTION('ref_axis',(0.,0.844082777626921,-0.536212891036408));
#20519=DIRECTION('center_axis',(0.,0.844082777626921,-0.536212891036408));
#20520=DIRECTION('ref_axis',(0.,0.536212891036408,0.844082777626921));
#20521=DIRECTION('center_axis',(-1.,6.12303176911189E-17,0.));
#20522=DIRECTION('ref_axis',(-6.12303176911189E-17,-1.,0.));
#20523=DIRECTION('center_axis',(-1.,6.12303176911189E-17,0.));
#20524=DIRECTION('ref_axis',(-6.12303176911189E-17,-1.,0.));
#20525=DIRECTION('',(-1.,6.12303176911189E-17,0.));
#20526=DIRECTION('center_axis',(1.,-6.12303176911189E-17,0.));
#20527=DIRECTION('ref_axis',(-6.12303176911189E-17,-1.,0.));
#20528=DIRECTION('center_axis',(-1.,0.,0.));
#20529=DIRECTION('ref_axis',(0.,0.,-1.));
#20530=DIRECTION('',(1.,0.,0.));
#20531=DIRECTION('center_axis',(1.,0.,0.));
#20532=DIRECTION('ref_axis',(0.,0.,-1.));
#20533=DIRECTION('',(-1.,0.,0.));
#20534=DIRECTION('center_axis',(0.,0.,1.));
#20535=DIRECTION('ref_axis',(-1.,0.,0.));
#20536=DIRECTION('center_axis',(8.67361737988403E-16,0.,-1.));
#20537=DIRECTION('ref_axis',(-1.,0.,-8.67361737988403E-16));
#20538=DIRECTION('',(0.,0.,-1.));
#20539=DIRECTION('',(0.,0.,1.));
#20540=DIRECTION('center_axis',(-1.,6.12303176911189E-17,0.));
#20541=DIRECTION('ref_axis',(6.12303176911189E-17,1.,0.));
#20542=DIRECTION('center_axis',(-1.,6.12303176911189E-17,0.));
#20543=DIRECTION('ref_axis',(-6.12303176911189E-17,-1.,0.));
#20544=DIRECTION('',(-1.,6.12303176911189E-17,0.));
#20545=DIRECTION('center_axis',(-1.,6.12303176911189E-17,0.));
#20546=DIRECTION('ref_axis',(6.12303176911189E-17,1.,0.));
#20547=DIRECTION('',(-1.,6.12303176911189E-17,0.));
#20548=DIRECTION('center_axis',(-1.,6.12303176911189E-17,0.));
#20549=DIRECTION('ref_axis',(-6.12303176911189E-17,-1.,0.));
#20550=DIRECTION('center_axis',(0.,1.,0.));
#20551=DIRECTION('ref_axis',(0.,0.,-1.));
#20552=DIRECTION('',(0.,-1.,0.));
#20553=DIRECTION('center_axis',(0.,-1.,0.));
#20554=DIRECTION('ref_axis',(-1.,0.,0.));
#20555=DIRECTION('',(0.,-1.,0.));
#20556=DIRECTION('center_axis',(0.,1.,0.));
#20557=DIRECTION('ref_axis',(0.,0.,-1.));
#20558=DIRECTION('center_axis',(0.,-1.,0.));
#20559=DIRECTION('ref_axis',(-1.,0.,0.));
#20560=DIRECTION('',(0.,1.,0.));
#20561=DIRECTION('center_axis',(0.,-1.,0.));
#20562=DIRECTION('ref_axis',(0.,0.,-1.));
#20563=DIRECTION('center_axis',(1.,0.,0.));
#20564=DIRECTION('ref_axis',(0.,0.,1.));
#20565=DIRECTION('',(-1.,0.,0.));
#20566=DIRECTION('center_axis',(-1.,6.12303176911189E-17,0.));
#20567=DIRECTION('ref_axis',(-6.12303176911189E-17,-1.,0.));
#20568=DIRECTION('center_axis',(1.,-9.50125619344947E-18,-2.21695977847154E-17));
#20569=DIRECTION('ref_axis',(-2.21695977847154E-17,2.10639028258311E-34,
-1.));
#20570=DIRECTION('center_axis',(1.,-9.50125619344947E-18,-2.21695977847154E-17));
#20571=DIRECTION('ref_axis',(-2.21695977847154E-17,2.10639028258311E-34,
-1.));
#20572=DIRECTION('',(1.,-9.50125619344947E-18,-2.21695977847154E-17));
#20573=DIRECTION('center_axis',(-1.,9.50125619344947E-18,2.21695977847154E-17));
#20574=DIRECTION('ref_axis',(-2.21695977847154E-17,2.10639028258311E-34,
-1.));
#20575=DIRECTION('center_axis',(-6.12303176911189E-17,-1.,5.4780741346636E-16));
#20576=DIRECTION('ref_axis',(0.,-5.80034886334776E-16,-1.));
#20577=DIRECTION('center_axis',(-1.,6.12303176911188E-17,-1.22464679914735E-16));
#20578=DIRECTION('ref_axis',(-1.22464679914735E-16,5.43782705938852E-16,
1.));
#20579=DIRECTION('center_axis',(-6.12303176911189E-17,-1.,5.4780741346636E-16));
#20580=DIRECTION('ref_axis',(-4.87050097983572E-33,-5.4780741346636E-16,
-1.));
#20581=DIRECTION('center_axis',(-6.12303176911189E-17,-1.,5.4780741346636E-16));
#20582=DIRECTION('ref_axis',(3.00804750808099E-33,-5.4780741346636E-16,
-1.));
#20583=DIRECTION('',(-1.00331952890699E-16,-0.936329177569045,0.351123441588391));
#20584=DIRECTION('center_axis',(-6.12303176911189E-17,-1.,5.4780741346636E-16));
#20585=DIRECTION('ref_axis',(3.00804750808099E-33,-5.4780741346636E-16,
-1.));
#20586=DIRECTION('center_axis',(-6.12303176911189E-17,-1.,5.4780741346636E-16));
#20587=DIRECTION('ref_axis',(0.,-5.07530525542929E-16,-1.));
#20588=DIRECTION('center_axis',(1.,-6.12303176911188E-17,1.22464679914735E-16));
#20589=DIRECTION('ref_axis',(-1.22464679914735E-16,5.07530525542929E-16,
1.));
#20590=DIRECTION('center_axis',(0.,1.,0.));
#20591=DIRECTION('ref_axis',(0.,0.,-1.));
#20592=DIRECTION('center_axis',(0.,-1.,0.));
#20593=DIRECTION('ref_axis',(-1.,0.,0.));
#20594=DIRECTION('',(0.,1.,0.));
#20595=DIRECTION('center_axis',(0.,-1.,0.));
#20596=DIRECTION('ref_axis',(0.,0.,-1.));
#20597=DIRECTION('center_axis',(0.,0.707106781186548,0.707106781186548));
#20598=DIRECTION('ref_axis',(0.,0.707106781186548,-0.707106781186548));
#20599=DIRECTION('center_axis',(0.,0.707106781186548,0.707106781186548));
#20600=DIRECTION('ref_axis',(-1.,0.,0.));
#20601=DIRECTION('',(0.,0.707106781186548,0.707106781186548));
#20602=DIRECTION('center_axis',(0.,0.707106781186548,0.707106781186548));
#20603=DIRECTION('ref_axis',(-1.,0.,0.));
#20604=DIRECTION('center_axis',(0.,0.,1.));
#20605=DIRECTION('ref_axis',(1.,0.,0.));
#20606=DIRECTION('center_axis',(0.,0.707106781186548,0.707106781186548));
#20607=DIRECTION('ref_axis',(1.,0.,0.));
#20608=DIRECTION('center_axis',(-1.,9.50125619344947E-18,2.21695977847154E-17));
#20609=DIRECTION('ref_axis',(9.50125619344947E-18,1.,-1.28981852722485E-50));
#20610=DIRECTION('center_axis',(1.,0.,0.));
#20611=DIRECTION('ref_axis',(0.,0.296692407913666,-0.954973096524918));
#20612=DIRECTION('',(-1.,0.,0.));
#20613=DIRECTION('center_axis',(-1.,6.12303176911189E-17,0.));
#20614=DIRECTION('ref_axis',(-6.12303176911189E-17,-1.,0.));
#20615=DIRECTION('center_axis',(1.,0.,0.));
#20616=DIRECTION('ref_axis',(0.,0.,1.));
#20617=DIRECTION('',(1.,0.,0.));
#20618=DIRECTION('center_axis',(-1.,6.12303176911189E-17,0.));
#20619=DIRECTION('ref_axis',(-6.12303176911189E-17,-1.,0.));
#20620=DIRECTION('center_axis',(0.763478425075362,0.,-0.645833333333334));
#20621=DIRECTION('ref_axis',(0.,-1.,0.));
#20622=DIRECTION('',(0.,-1.,0.));
#20623=DIRECTION('',(-0.645833333333334,0.,-0.763478425075362));
#20624=DIRECTION('',(0.645833333333334,0.,0.763478425075362));
#20625=DIRECTION('center_axis',(0.,1.,0.));
#20626=DIRECTION('ref_axis',(0.,0.,-1.));
#20627=DIRECTION('',(0.,-1.,0.));
#20628=DIRECTION('center_axis',(0.,1.,0.));
#20629=DIRECTION('ref_axis',(0.,0.,-1.));
#20630=DIRECTION('center_axis',(0.,-1.,0.));
#20631=DIRECTION('ref_axis',(-1.,0.,0.));
#20632=DIRECTION('center_axis',(0.,-1.,0.));
#20633=DIRECTION('ref_axis',(0.,0.,-1.));
#20634=DIRECTION('center_axis',(0.,-1.,0.));
#20635=DIRECTION('ref_axis',(-1.,0.,0.));
#20636=DIRECTION('',(-0.645833333333333,0.,0.763478425075362));
#20637=DIRECTION('',(0.645833333333334,0.,-0.763478425075362));
#20638=DIRECTION('center_axis',(0.,-1.,0.));
#20639=DIRECTION('ref_axis',(1.,0.,0.));
#20640=DIRECTION('',(-0.645833333333334,0.,-0.763478425075362));
#20641=DIRECTION('center_axis',(0.763478425075362,0.,0.645833333333333));
#20642=DIRECTION('ref_axis',(0.,-1.,0.));
#20643=DIRECTION('',(0.,-1.,0.));
#20644=DIRECTION('',(0.645833333333333,0.,-0.763478425075362));
#20645=DIRECTION('center_axis',(0.,1.,0.));
#20646=DIRECTION('ref_axis',(3.21624529935327E-16,0.,1.));
#20647=DIRECTION('',(0.,-1.,0.));
#20648=DIRECTION('center_axis',(0.,1.,0.));
#20649=DIRECTION('ref_axis',(0.,0.,-1.));
#20650=DIRECTION('center_axis',(-0.763478425075362,0.,0.645833333333334));
#20651=DIRECTION('ref_axis',(0.,1.,0.));
#20652=DIRECTION('',(0.,-1.,0.));
#20653=DIRECTION('',(0.645833333333334,0.,0.763478425075362));
#20654=DIRECTION('center_axis',(0.,1.,0.));
#20655=DIRECTION('ref_axis',(0.,0.,-1.));
#20656=DIRECTION('',(0.,-1.,0.));
#20657=DIRECTION('center_axis',(0.,1.,0.));
#20658=DIRECTION('ref_axis',(0.,0.,-1.));
#20659=DIRECTION('center_axis',(1.,0.,0.));
#20660=DIRECTION('ref_axis',(0.,1.,0.));
#20661=DIRECTION('',(0.,0.939692620785908,-0.342020143325669));
#20662=DIRECTION('center_axis',(0.00295110397743048,-0.889977818593701,
0.45599426903911));
#20663=DIRECTION('ref_axis',(-7.26976717678396E-18,0.455996254682473,0.88998169403396));
#20664=DIRECTION('center_axis',(0.999864261635529,0.,-0.0164759917467061));
#20665=DIRECTION('ref_axis',(0.0164759917467061,0.,0.999864261635529));
#20666=DIRECTION('center_axis',(0.999864261635529,0.,-0.0164759917467083));
#20667=DIRECTION('ref_axis',(-0.0164759917467083,0.,-0.999864261635529));
#20668=DIRECTION('center_axis',(0.999865821664235,1.8733920536864E-13,-0.0163810459893322));
#20669=DIRECTION('ref_axis',(-0.0163810459893322,1.88332865382296E-28,-0.999865821664235));
#20670=DIRECTION('center_axis',(-0.189008920572759,0.,-0.981975370334674));
#20671=DIRECTION('ref_axis',(-0.981975370334674,0.,0.189008920572759));
#20672=DIRECTION('center_axis',(0.,-1.,0.));
#20673=DIRECTION('ref_axis',(0.,0.,-1.));
#20674=DIRECTION('center_axis',(-0.0588235294117643,8.6585981177414E-16,
-0.998268396969244));
#20675=DIRECTION('ref_axis',(-0.998268396969244,-2.36797261535997E-32,0.0588235294117643));
#20676=DIRECTION('center_axis',(0.,-1.,0.));
#20677=DIRECTION('ref_axis',(0.,0.,-1.));
#20678=DIRECTION('center_axis',(0.,1.,0.));
#20679=DIRECTION('ref_axis',(1.,0.,0.));
#20680=DIRECTION('center_axis',(1.,-6.12303176911189E-17,0.));
#20681=DIRECTION('ref_axis',(-6.12303176911189E-17,-1.,0.));
#20682=DIRECTION('center_axis',(0.,-1.,0.));
#20683=DIRECTION('ref_axis',(0.,0.,-1.));
#20684=DIRECTION('center_axis',(0.645833333333334,0.,0.763478425075362));
#20685=DIRECTION('ref_axis',(-0.763478425075362,0.,0.645833333333334));
#20686=DIRECTION('center_axis',(0.645833333333334,0.,-0.763478425075362));
#20687=DIRECTION('ref_axis',(-0.763478425075362,0.,-0.645833333333334));
#20688=DIRECTION('center_axis',(0.,-1.,0.));
#20689=DIRECTION('ref_axis',(0.,0.,-1.));
#20690=DIRECTION('center_axis',(0.,1.,0.));
#20691=DIRECTION('ref_axis',(1.,0.,0.));
#20692=DIRECTION('center_axis',(-1.,-7.44144872161806E-15,-1.1714001680137E-14));
#20693=DIRECTION('ref_axis',(-1.1714001680137E-14,1.61017035136602E-29,
1.));
#20694=DIRECTION('center_axis',(2.91984586184824E-15,-0.844082777626921,
0.536212891036408));
#20695=DIRECTION('ref_axis',(1.11963091130469E-29,-0.536212891036408,-0.844082777626921));
#20696=DIRECTION('center_axis',(-0.707106781186551,-0.379159771411502,-0.596856655942759));
#20697=DIRECTION('ref_axis',(0.645019472682989,9.66631051215658E-16,-0.764166133677592));
#20698=DIRECTION('center_axis',(-1.,0.,0.));
#20699=DIRECTION('ref_axis',(0.,-0.21769688453124,0.976016427354269));
#20700=DIRECTION('',(1.,0.,0.));
#20701=DIRECTION('',(-1.,0.,0.));
#20702=DIRECTION('center_axis',(-1.06260198549818E-16,-0.844082777626919,
0.53621289103641));
#20703=DIRECTION('ref_axis',(3.01348942600866E-31,0.53621289103641,0.844082777626919));
#20704=DIRECTION('center_axis',(-3.74339213057462E-16,-0.844082777626916,
0.536212891036415));
#20705=DIRECTION('ref_axis',(-1.14237476972092E-30,0.536212891036415,0.844082777626916));
#20706=DIRECTION('',(7.1769990995421E-17,0.844082777626919,-0.53621289103641));
#20707=DIRECTION('',(-1.06260198549818E-16,-0.844082777626919,0.53621289103641));
#20708=DIRECTION('center_axis',(0.,1.,0.));
#20709=DIRECTION('ref_axis',(1.,0.,0.));
#20710=DIRECTION('center_axis',(0.,0.,-1.));
#20711=DIRECTION('ref_axis',(-1.,0.,0.));
#20712=DIRECTION('center_axis',(-1.,0.,0.));
#20713=DIRECTION('ref_axis',(0.,0.,1.));
#20714=DIRECTION('center_axis',(0.,-1.,0.));
#20715=DIRECTION('ref_axis',(0.,0.,1.));
#20716=DIRECTION('center_axis',(0.,0.,-1.));
#20717=DIRECTION('ref_axis',(1.,0.,0.));
#20718=DIRECTION('center_axis',(0.,0.,-1.));
#20719=DIRECTION('ref_axis',(1.,0.,0.));
#20720=DIRECTION('',(0.,0.,1.));
#20721=DIRECTION('',(0.,0.,-1.));
#20722=DIRECTION('center_axis',(-1.,0.,0.));
#20723=DIRECTION('ref_axis',(0.,0.,-1.));
#20724=DIRECTION('center_axis',(0.763478425075353,-1.69136608464776E-14,
0.645833333333344));
#20725=DIRECTION('ref_axis',(0.645833333333344,-3.74756545942938E-12,-0.763478425075353));
#20726=DIRECTION('',(1.,0.,0.));
#20727=DIRECTION('',(-1.,0.,0.));
#20728=DIRECTION('center_axis',(0.,1.,0.));
#20729=DIRECTION('ref_axis',(1.,0.,0.));
#20730=DIRECTION('center_axis',(0.,1.,0.));
#20731=DIRECTION('ref_axis',(0.,0.,1.));
#20732=DIRECTION('center_axis',(-1.,0.,0.));
#20733=DIRECTION('ref_axis',(0.,0.,1.));
#20734=DIRECTION('center_axis',(6.12303176911189E-17,1.,0.));
#20735=DIRECTION('ref_axis',(1.,-6.12303176911189E-17,0.));
#20736=DIRECTION('center_axis',(0.,1.,0.));
#20737=DIRECTION('ref_axis',(0.,0.,-1.));
#20738=DIRECTION('',(-6.12303176911189E-17,-1.,0.));
#20739=DIRECTION('',(6.12303176911189E-17,1.,0.));
#20740=DIRECTION('center_axis',(-1.,0.,0.));
#20741=DIRECTION('ref_axis',(0.,0.,-1.));
#20742=DIRECTION('center_axis',(0.763478425075345,1.20977462004704E-13,
0.645833333333353));
#20743=DIRECTION('ref_axis',(0.645833333333353,2.41075408440725E-12,-0.763478425075345));
#20744=DIRECTION('',(1.,0.,0.));
#20745=DIRECTION('',(-1.,0.,0.));
#20746=DIRECTION('center_axis',(0.,1.,0.));
#20747=DIRECTION('ref_axis',(1.,0.,0.));
#20748=DIRECTION('center_axis',(0.,-1.38777878078144E-14,1.));
#20749=DIRECTION('ref_axis',(0.,-1.,-1.38777878078144E-14));
#20750=DIRECTION('center_axis',(-1.,0.,0.));
#20751=DIRECTION('ref_axis',(0.,0.,1.));
#20752=DIRECTION('center_axis',(-8.49741356322415E-31,-1.38777878078145E-14,
1.));
#20753=DIRECTION('ref_axis',(-4.72949161117447E-59,1.,1.38777878078145E-14));
#20754=DIRECTION('center_axis',(1.2440942836624E-13,0.844082777626929,-0.536212891036395));
#20755=DIRECTION('ref_axis',(-6.70739907751221E-13,0.536212891036395,0.844082777626929));
#20756=DIRECTION('',(8.49741356322415E-31,1.38777878078145E-14,-1.));
#20757=DIRECTION('',(-8.49741356322415E-31,-1.38777878078145E-14,1.));
#20758=DIRECTION('center_axis',(3.28324856682327E-17,0.53621289103641,0.844082777626919));
#20759=DIRECTION('ref_axis',(-9.30104503460367E-32,0.844082777626919,-0.53621289103641));
#20760=DIRECTION('',(-3.28324856682327E-17,-0.53621289103641,-0.844082777626919));
#20761=DIRECTION('center_axis',(1.05472713558318E-13,-0.876416821790961,
-0.481553272735044));
#20762=DIRECTION('ref_axis',(-1.50588472234195E-12,0.481553272735044,-0.876416821790961));
#20763=DIRECTION('',(3.28324856682327E-17,0.53621289103641,0.844082777626919));
#20764=DIRECTION('center_axis',(0.,0.,1.));
#20765=DIRECTION('ref_axis',(1.,0.,0.));
#20766=DIRECTION('center_axis',(0.,0.844082777626921,-0.536212891036408));
#20767=DIRECTION('ref_axis',(0.,-0.536212891036408,-0.844082777626921));
#20768=DIRECTION('center_axis',(0.,-0.536212891036408,-0.844082777626921));
#20769=DIRECTION('ref_axis',(0.,0.844082777626921,-0.536212891036408));
#20770=DIRECTION('center_axis',(-1.,0.,0.));
#20771=DIRECTION('ref_axis',(0.,0.,-1.));
#20772=DIRECTION('center_axis',(5.16834566316983E-17,0.844082777626919,
-0.536212891036411));
#20773=DIRECTION('ref_axis',(-1.89077532649189E-31,-0.536212891036411,-0.844082777626919));
#20774=DIRECTION('',(-5.16834566316983E-17,-0.844082777626919,0.536212891036411));
#20775=DIRECTION('',(5.16834566316983E-17,0.844082777626919,-0.536212891036411));
#20776=DIRECTION('center_axis',(7.85046229341887E-17,0.844082777626919,
-0.536212891036411));
#20777=DIRECTION('ref_axis',(-2.87429797914763E-31,-0.536212891036411,-0.844082777626919));
#20778=DIRECTION('center_axis',(5.54022035325046E-15,0.84408277762691,-0.536212891036424));
#20779=DIRECTION('ref_axis',(-1.55850943745324E-30,-0.536212891036424,-0.84408277762691));
#20780=DIRECTION('',(-5.55111512312579E-17,-0.844082777626919,0.536212891036411));
#20781=DIRECTION('center_axis',(-3.06958154707117E-15,0.844082777626921,
-0.536212891036408));
#20782=DIRECTION('ref_axis',(-1.81691724756689E-31,0.536212891036408,0.844082777626921));
#20783=DIRECTION('',(7.85046229341887E-17,0.844082777626919,-0.536212891036411));
#20784=DIRECTION('center_axis',(0.,0.,1.));
#20785=DIRECTION('ref_axis',(1.,0.,0.));
#20786=DIRECTION('center_axis',(-1.,2.34280033602742E-14,-1.48828974432361E-14));
#20787=DIRECTION('ref_axis',(-2.34280033602742E-14,-1.,6.44068140546378E-29));
#20788=DIRECTION('center_axis',(-0.707106781186557,0.379159771411482,0.596856655942765));
#20789=DIRECTION('ref_axis',(-0.645019472682989,1.25388061323787E-15,-0.764166133677592));
#20790=DIRECTION('center_axis',(-1.,0.,0.));
#20791=DIRECTION('ref_axis',(0.,0.,-1.));
#20792=DIRECTION('',(1.,0.,0.));
#20793=DIRECTION('',(-1.,0.,0.));
#20794=DIRECTION('center_axis',(0.707106781186547,-0.379159771411489,-0.596856655942772));
#20795=DIRECTION('ref_axis',(0.645019472683,1.15352107484122E-15,0.764166133677583));
#20796=DIRECTION('',(0.707106781186547,-0.379159771411489,-0.596856655942772));
#20797=DIRECTION('center_axis',(-0.707106781186551,0.37915977141147,0.596856655942779));
#20798=DIRECTION('ref_axis',(0.645019472683002,9.5350569374018E-17,0.764166133677581));
#20799=DIRECTION('',(-0.707106781186547,0.379159771411489,0.596856655942772));
#20800=DIRECTION('center_axis',(5.16834566316983E-17,0.844082777626919,
-0.536212891036411));
#20801=DIRECTION('ref_axis',(-7.00354623150013E-33,-0.536212891036411,-0.844082777626919));
#20802=DIRECTION('center_axis',(0.,0.844082777626919,-0.53621289103641));
#20803=DIRECTION('ref_axis',(0.,-0.53621289103641,-0.844082777626919));
#20804=DIRECTION('',(-5.16834566316983E-17,-0.844082777626919,0.536212891036411));
#20805=DIRECTION('',(2.77555756156288E-17,0.844082777626919,-0.536212891036411));
#20806=DIRECTION('center_axis',(0.,1.,0.));
#20807=DIRECTION('ref_axis',(-0.9069232251638,0.,0.42129593358884));
#20808=DIRECTION('center_axis',(-1.32984495616866E-14,-0.536212891036413,
-0.844082777626917));
#20809=DIRECTION('ref_axis',(-6.77246941118238E-30,0.844082777626917,-0.536212891036413));
#20810=DIRECTION('center_axis',(3.28324856682327E-17,0.53621289103641,0.844082777626919));
#20811=DIRECTION('ref_axis',(1.02431542274941E-31,0.844082777626919,-0.53621289103641));
#20812=DIRECTION('',(3.28324856682327E-17,0.53621289103641,0.844082777626919));
#20813=DIRECTION('',(-3.28324856682327E-17,-0.53621289103641,-0.844082777626919));
#20814=DIRECTION('center_axis',(-3.28324856682327E-17,-0.53621289103641,
-0.844082777626919));
#20815=DIRECTION('ref_axis',(9.30104503460367E-32,-0.844082777626919,0.53621289103641));
#20816=DIRECTION('',(-3.28324856682327E-17,-0.53621289103641,-0.844082777626919));
#20817=DIRECTION('center_axis',(-1.2947686397577E-14,-0.279210693180882,
-0.960229862487858));
#20818=DIRECTION('ref_axis',(-1.21180702059432E-11,0.960229862487858,-0.279210693180882));
#20819=DIRECTION('',(3.28324856682327E-17,0.53621289103641,0.844082777626919));
#20820=DIRECTION('center_axis',(0.,1.,0.));
#20821=DIRECTION('ref_axis',(1.,0.,0.));
#20822=DIRECTION('center_axis',(-3.28324856682327E-17,-0.53621289103641,
-0.844082777626919));
#20823=DIRECTION('ref_axis',(-1.02431542274941E-31,-0.844082777626919,0.53621289103641));
#20824=DIRECTION('',(-3.28324856682327E-17,-0.53621289103641,-0.844082777626919));
#20825=DIRECTION('center_axis',(-5.85700084006849E-15,0.536212891036413,
0.844082777626917));
#20826=DIRECTION('ref_axis',(-2.92088988510645E-30,-0.844082777626917,0.536212891036413));
#20827=DIRECTION('',(3.28324856682327E-17,0.53621289103641,0.844082777626919));
#20828=DIRECTION('center_axis',(0.,1.,0.));
#20829=DIRECTION('ref_axis',(-0.906923225163802,0.,-0.421295933588834));
#20830=DIRECTION('center_axis',(-0.707106781186551,-0.379159771411477,-0.596856655942775));
#20831=DIRECTION('ref_axis',(-0.645019472682999,-2.94711224947621E-16,0.764166133677583));
#20832=DIRECTION('center_axis',(0.,-0.844082777626922,0.536212891036405));
#20833=DIRECTION('ref_axis',(0.,0.536212891036405,0.844082777626922));
#20834=DIRECTION('center_axis',(0.707106781186547,0.379159771411489,0.596856655942772));
#20835=DIRECTION('ref_axis',(-0.645019472683,1.15352107484122E-15,0.764166133677583));
#20836=DIRECTION('center_axis',(-0.707106781186541,-0.379159771411494,-0.596856655942776));
#20837=DIRECTION('ref_axis',(0.645019472683004,1.45000042130455E-15,-0.764166133677579));
#20838=DIRECTION('',(0.707106781186547,0.379159771411489,0.596856655942772));
#20839=DIRECTION('',(-0.707106781186547,-0.379159771411489,-0.596856655942772));
#20840=DIRECTION('center_axis',(-0.707106781186547,-0.379159771411489,-0.596856655942772));
#20841=DIRECTION('ref_axis',(-0.499999999999993,-0.32875021042458,0.801201160224947));
#20842=DIRECTION('',(0.707106781186547,0.379159771411489,0.596856655942772));
#20843=DIRECTION('',(-0.707106781186546,-0.37915977141149,-0.596856655942772));
#20844=DIRECTION('center_axis',(-5.16834566316983E-17,-0.844082777626919,
0.53621289103641));
#20845=DIRECTION('ref_axis',(4.60389737147646E-33,0.53621289103641,0.844082777626919));
#20846=DIRECTION('',(5.16834566316983E-17,0.844082777626919,-0.53621289103641));
#20847=DIRECTION('',(-5.55111512312577E-17,-0.844082777626919,0.53621289103641));
#20848=DIRECTION('center_axis',(3.28324856682327E-17,0.53621289103641,0.844082777626919));
#20849=DIRECTION('ref_axis',(1.02431542274941E-31,0.844082777626919,-0.53621289103641));
#20850=DIRECTION('',(3.28324856682327E-17,0.53621289103641,0.844082777626919));
#20851=DIRECTION('center_axis',(0.707106781186648,-0.379159771411277,-0.596856655942787));
#20852=DIRECTION('ref_axis',(0.707106781186447,0.379159771409511,0.596856655944146));
#20853=DIRECTION('',(-3.28324856682327E-17,-0.53621289103641,-0.844082777626919));
#20854=DIRECTION('center_axis',(0.,-1.,0.));
#20855=DIRECTION('ref_axis',(0.,0.,-1.));
#20856=DIRECTION('',(-0.645833333333334,0.,0.763478425075362));
#20857=DIRECTION('center_axis',(-1.,6.12303176911189E-17,0.));
#20858=DIRECTION('ref_axis',(0.,0.,1.));
#20859=DIRECTION('',(-5.16834566316983E-17,-0.844082777626919,0.53621289103641));
#20860=DIRECTION('',(3.28324856682327E-17,0.53621289103641,0.844082777626919));
#20861=DIRECTION('',(-6.12303176911189E-17,-1.,0.));
#20862=DIRECTION('',(3.28324856682327E-17,0.53621289103641,0.844082777626919));
#20863=DIRECTION('center_axis',(-1.,6.12303176911189E-17,0.));
#20864=DIRECTION('ref_axis',(-6.12303176911189E-17,-1.,0.));
#20865=DIRECTION('center_axis',(0.,1.,1.38777878078145E-14));
#20866=DIRECTION('ref_axis',(0.,1.38777878078145E-14,-1.));
#20867=DIRECTION('',(-8.49741356322415E-31,-1.38777878078145E-14,1.));
#20868=DIRECTION('',(-1.,0.,0.));
#20869=DIRECTION('',(1.,0.,0.));
#20870=DIRECTION('center_axis',(0.,0.,-1.));
#20871=DIRECTION('ref_axis',(0.,-1.,0.));
#20872=DIRECTION('',(6.12303176911189E-17,1.,0.));
#20873=DIRECTION('center_axis',(0.,0.,1.));
#20874=DIRECTION('ref_axis',(-1.,0.,0.));
#20875=DIRECTION('',(1.,0.,0.));
#20876=DIRECTION('center_axis',(4.09272608780354E-15,5.36063096661746E-15,
-1.));
#20877=DIRECTION('ref_axis',(1.,8.41575319003231E-13,4.09272608780805E-15));
#20878=DIRECTION('',(0.,-1.,0.));
#20879=DIRECTION('',(1.,0.,0.));
#20880=DIRECTION('center_axis',(0.,0.393919298579167,0.919145030018058));
#20881=DIRECTION('ref_axis',(1.,0.,0.));
#20882=DIRECTION('center_axis',(-2.8065169850844E-7,0.393919438749702,0.919144969944916));
#20883=DIRECTION('ref_axis',(-0.918388540903831,0.36368697754103,-0.155866193587968));
#20884=DIRECTION('center_axis',(-2.74470711777249E-6,0.393918529530603,
0.919145359605821));
#20885=DIRECTION('ref_axis',(0.773783494589027,0.582233610477103,-0.249525802939077));
#20886=DIRECTION('',(1.,0.,0.));
#20887=DIRECTION('',(5.62795421922187E-17,0.919145030018058,-0.393919298579167));
#20888=DIRECTION('center_axis',(0.,0.707106781186548,0.707106781186548));
#20889=DIRECTION('ref_axis',(-0.0433996118379072,-0.706440540205727,0.706440540205727));
#20890=DIRECTION('center_axis',(0.,0.707106781186548,0.707106781186548));
#20891=DIRECTION('ref_axis',(1.,0.,0.));
#20892=DIRECTION('center_axis',(1.,-6.12303176911189E-17,0.));
#20893=DIRECTION('ref_axis',(-6.12303176911189E-17,-1.,0.));
#20894=DIRECTION('',(0.,0.,1.));
#20895=DIRECTION('',(0.,1.,0.));
#20896=DIRECTION('',(0.,0.,1.));
#20897=DIRECTION('center_axis',(0.,0.,-1.));
#20898=DIRECTION('ref_axis',(0.,-1.,0.));
#20899=DIRECTION('',(1.,0.,0.));
#20900=DIRECTION('',(1.,0.,0.));
#20901=DIRECTION('center_axis',(-1.63807337386231E-14,2.73218531703445E-14,
1.));
#20902=DIRECTION('ref_axis',(-6.24102255372086E-12,-1.,2.73218531702423E-14));
#20903=DIRECTION('center_axis',(0.,0.,1.));
#20904=DIRECTION('ref_axis',(-1.,0.,0.));
#20905=DIRECTION('center_axis',(5.57758659674859E-13,0.707106781185667,
0.707106781187428));
#20906=DIRECTION('ref_axis',(1.7011908926004E-10,-0.707106781187428,0.707106781185667));
#20907=DIRECTION('center_axis',(0.,0.707106781186548,0.707106781186548));
#20908=DIRECTION('ref_axis',(1.,0.,0.));
#20909=DIRECTION('center_axis',(0.,0.707106781186548,0.707106781186548));
#20910=DIRECTION('ref_axis',(1.,0.,0.));
#20911=DIRECTION('center_axis',(1.,-6.12303176911189E-17,0.));
#20912=DIRECTION('ref_axis',(0.,-1.,-3.82599934640054E-15));
#20913=DIRECTION('center_axis',(-5.76857827429812E-17,-0.942111439531993,
0.335299918733896));
#20914=DIRECTION('ref_axis',(-2.18993762695094E-31,0.335299918733896,0.942111439531992));
#20915=DIRECTION('center_axis',(1.,-6.12303176911189E-17,0.));
#20916=DIRECTION('ref_axis',(6.12303176911189E-17,1.,0.));
#20917=DIRECTION('center_axis',(0.,0.942111439531991,0.335299918733899));
#20918=DIRECTION('ref_axis',(0.,-0.335299918733899,0.942111439531991));
#20919=DIRECTION('center_axis',(0.,-0.393919298579169,-0.919145030018057));
#20920=DIRECTION('ref_axis',(0.,-0.919145030018057,0.393919298579169));
#20921=DIRECTION('center_axis',(-4.29577406892133E-7,-0.393919484948488,
-0.919144950145369));
#20922=DIRECTION('ref_axis',(0.716472147339189,-0.641210067193636,0.274804133550978));
#20923=DIRECTION('',(-5.62795421922186E-17,-0.919145030018057,0.393919298579169));
#20924=DIRECTION('center_axis',(0.,1.,0.));
#20925=DIRECTION('ref_axis',(-0.733899982512709,0.,-0.679257547376432));
#20926=DIRECTION('center_axis',(-1.,6.12303176911189E-17,0.));
#20927=DIRECTION('ref_axis',(0.,0.,1.));
#20928=DIRECTION('center_axis',(-1.,6.12303176911189E-17,0.));
#20929=DIRECTION('ref_axis',(0.,0.,1.));
#20930=DIRECTION('center_axis',(-1.,6.12303176911189E-17,0.));
#20931=DIRECTION('ref_axis',(-6.12303176911189E-17,-1.,0.));
#20932=DIRECTION('center_axis',(-1.,6.12303176911189E-17,0.));
#20933=DIRECTION('ref_axis',(0.,0.976016427354256,0.217696884531301));
#20934=DIRECTION('center_axis',(0.,-0.536212891036408,-0.844082777626921));
#20935=DIRECTION('ref_axis',(0.,0.844082777626921,-0.536212891036408));
#20936=DIRECTION('center_axis',(-1.,6.12303176911189E-17,0.));
#20937=DIRECTION('ref_axis',(-6.12303176911189E-17,-1.,0.));
#20938=DIRECTION('center_axis',(0.,0.844082777626921,-0.536212891036408));
#20939=DIRECTION('ref_axis',(0.,-0.536212891036408,-0.844082777626921));
#20940=DIRECTION('center_axis',(-1.,0.,0.));
#20941=DIRECTION('ref_axis',(0.,0.,-1.));
#20942=DIRECTION('',(1.,0.,0.));
#20943=DIRECTION('center_axis',(-1.,0.,0.));
#20944=DIRECTION('ref_axis',(0.,0.,1.));
#20945=DIRECTION('',(-1.,0.,0.));
#20946=DIRECTION('center_axis',(-5.16834566316983E-17,-0.844082777626919,
0.53621289103641));
#20947=DIRECTION('ref_axis',(1.42644336347277E-31,0.53621289103641,0.844082777626919));
#20948=DIRECTION('',(5.16834566316983E-17,0.844082777626919,-0.53621289103641));
#20949=DIRECTION('center_axis',(0.,0.,1.));
#20950=DIRECTION('ref_axis',(1.,0.,0.));
#20951=DIRECTION('center_axis',(6.35380838599017E-16,-0.53621289103641,
-0.844082777626919));
#20952=DIRECTION('ref_axis',(-2.25177327489712E-32,-0.844082777626919,0.53621289103641));
#20953=DIRECTION('',(-1.,-3.40699396374318E-16,-5.3631402309558E-16));
#20954=DIRECTION('',(0.,0.844082777626919,-0.53621289103641));
#20955=DIRECTION('center_axis',(-0.707106781186548,0.379159771411488,0.596856655942771));
#20956=DIRECTION('ref_axis',(0.472562808991505,0.881296993957235,-5.26365224320196E-17));
#20957=DIRECTION('center_axis',(-3.28324856682327E-17,-0.53621289103641,
-0.844082777626919));
#20958=DIRECTION('ref_axis',(-1.02431542274941E-31,-0.844082777626919,0.53621289103641));
#20959=DIRECTION('',(-3.28324856682327E-17,-0.53621289103641,-0.844082777626919));
#20960=DIRECTION('center_axis',(0.707106781186624,0.37915977141133,0.596856655942782));
#20961=DIRECTION('ref_axis',(0.707106781186471,-0.379159771411251,-0.596856655943013));
#20962=DIRECTION('',(3.28324856682327E-17,0.53621289103641,0.844082777626919));
#20963=DIRECTION('center_axis',(1.,0.,0.));
#20964=DIRECTION('ref_axis',(0.,0.,1.));
#20965=DIRECTION('',(-1.,0.,0.));
#20966=DIRECTION('',(1.,0.,0.));
#20967=DIRECTION('center_axis',(1.,-6.12303176911189E-17,0.));
#20968=DIRECTION('ref_axis',(-6.12303176911189E-17,-1.,0.));
#20969=DIRECTION('center_axis',(0.,0.707106781186548,0.707106781186548));
#20970=DIRECTION('ref_axis',(0.,0.707106781186548,-0.707106781186548));
#20971=DIRECTION('center_axis',(0.,0.,1.));
#20972=DIRECTION('ref_axis',(1.,1.22464679914735E-16,0.));
#20973=DIRECTION('',(0.,0.,1.));
#20974=DIRECTION('',(0.,0.,1.));
#20975=DIRECTION('center_axis',(1.,0.,0.));
#20976=DIRECTION('ref_axis',(0.,0.,1.));
#20977=DIRECTION('center_axis',(-1.07888181684715E-8,1.,-7.76704436521076E-9));
#20978=DIRECTION('ref_axis',(0.988419917866598,9.48528488113968E-9,-0.151743421487022));
#20979=DIRECTION('center_axis',(-4.24666173856902E-7,-0.999999999999844,
3.63117712421864E-7));
#20980=DIRECTION('ref_axis',(0.988473455373134,-4.74745184886749E-7,-0.151394280019001));
#20981=DIRECTION('center_axis',(-0.641555200491106,0.,0.76707687015241));
#20982=DIRECTION('ref_axis',(0.,1.,0.));
#20983=DIRECTION('',(0.76707687015241,0.,0.641555200491106));
#20984=DIRECTION('',(0.76707687015241,0.,0.641555200491106));
#20985=DIRECTION('center_axis',(0.,-1.,0.));
#20986=DIRECTION('ref_axis',(0.,0.,-1.));
#20987=DIRECTION('center_axis',(-6.12303176911189E-17,-1.,0.));
#20988=DIRECTION('ref_axis',(-1.,6.12303176911189E-17,0.));
#20989=DIRECTION('',(6.12303176911189E-17,1.,0.));
#20990=DIRECTION('center_axis',(-9.15914568528454E-14,-0.618483918322797,
0.785797456585397));
#20991=DIRECTION('ref_axis',(6.57167920551881E-13,-0.785797456585397,-0.618483918322797));
#20992=DIRECTION('center_axis',(3.28324856682327E-17,0.53621289103641,0.844082777626919));
#20993=DIRECTION('ref_axis',(-9.30104503460367E-32,0.844082777626919,-0.53621289103641));
#20994=DIRECTION('center_axis',(0.,-0.536212891036408,-0.844082777626921));
#20995=DIRECTION('ref_axis',(0.,0.844082777626921,-0.536212891036408));
#20996=DIRECTION('',(-3.28324856682327E-17,-0.53621289103641,-0.844082777626919));
#20997=DIRECTION('center_axis',(-3.63890463093118E-14,-0.844082777626962,
0.536212891036343));
#20998=DIRECTION('ref_axis',(-1.84413742032711E-5,-0.536212890945164,-0.844082777483432));
#20999=DIRECTION('center_axis',(0.,0.844082777626919,-0.53621289103641));
#21000=DIRECTION('ref_axis',(-1.,0.,0.));
#21001=DIRECTION('',(1.,3.40699396374318E-16,5.3631402309558E-16));
#21002=DIRECTION('',(1.,0.,0.));
#21003=DIRECTION('',(-3.28324856682327E-17,-0.53621289103641,-0.844082777626919));
#21004=DIRECTION('center_axis',(0.,-1.,0.));
#21005=DIRECTION('ref_axis',(0.,0.,-1.));
#21006=DIRECTION('',(-0.645833333333334,0.,-0.763478425075362));
#21007=DIRECTION('',(0.645833333333334,0.,-0.763478425075362));
#21008=DIRECTION('',(0.,0.,1.));
#21009=DIRECTION('center_axis',(0.,-1.,0.));
#21010=DIRECTION('ref_axis',(0.,0.,-1.));
#21011=DIRECTION('',(0.,0.,-1.));
#21012=DIRECTION('',(0.645833333333334,0.,-0.763478425075362));
#21013=DIRECTION('',(0.645833333333334,0.,0.763478425075362));
#21014=DIRECTION('center_axis',(0.,-1.,0.));
#21015=DIRECTION('ref_axis',(0.,0.,-1.));
#21016=DIRECTION('',(-0.645833333333333,0.,0.763478425075362));
#21017=DIRECTION('center_axis',(0.,-1.,0.));
#21018=DIRECTION('ref_axis',(0.,0.,-1.));
#21019=DIRECTION('center_axis',(0.,0.536212891036411,0.844082777626919));
#21020=DIRECTION('ref_axis',(1.,0.,0.));
#21021=DIRECTION('center_axis',(-0.707106781186548,-0.379159771411489,-0.596856655942771));
#21022=DIRECTION('ref_axis',(-0.645019472682998,-1.54058679206033E-17,0.764166133677584));
#21023=DIRECTION('center_axis',(-1.,6.12303176911189E-17,3.08148791101958E-33));
#21024=DIRECTION('ref_axis',(3.08148791101958E-33,0.,1.));
#21025=DIRECTION('',(-6.12303176911189E-17,-1.,1.88680483753071E-49));
#21026=DIRECTION('',(1.9280126729044E-32,3.65204942310907E-16,-1.));
#21027=DIRECTION('',(6.12303176911189E-17,1.,0.));
#21028=DIRECTION('center_axis',(-1.,-4.06251537009573E-12,-1.06264377235447E-13));
#21029=DIRECTION('ref_axis',(4.06239277484557E-12,-0.999999999824389,1.87409114472015E-5));
#21030=DIRECTION('center_axis',(-1.,6.12303176911189E-17,3.08148791101958E-33));
#21031=DIRECTION('ref_axis',(3.08148791101958E-33,0.,1.));
#21032=DIRECTION('center_axis',(-1.,6.12303176911189E-17,3.08148791101958E-33));
#21033=DIRECTION('ref_axis',(3.08148791101958E-33,0.,1.));
#21034=DIRECTION('',(0.,0.844082777626919,-0.53621289103641));
#21035=DIRECTION('center_axis',(0.,-1.,0.));
#21036=DIRECTION('ref_axis',(0.,0.,-1.));
#21037=DIRECTION('center_axis',(0.,-0.53621289103641,-0.844082777626919));
#21038=DIRECTION('ref_axis',(0.,-0.844082777626919,0.53621289103641));
#21039=DIRECTION('center_axis',(0.,1.,3.65204942310907E-16));
#21040=DIRECTION('ref_axis',(0.,3.65204942310907E-16,-1.));
#21041=DIRECTION('',(-1.9280126729044E-32,-3.65204942310907E-16,1.));
#21042=DIRECTION('center_axis',(0.,1.,3.65204942310907E-16));
#21043=DIRECTION('ref_axis',(0.,-3.65204942310907E-16,1.));
#21044=DIRECTION('',(-2.23616146400636E-32,-3.65204942310907E-16,1.));
#21045=DIRECTION('center_axis',(0.,0.53621289103641,0.844082777626919));
#21046=DIRECTION('ref_axis',(1.,0.,0.));
#21047=DIRECTION('center_axis',(-0.763478425075362,0.,-0.645833333333334));
#21048=DIRECTION('ref_axis',(-0.645833333333334,0.,0.763478425075362));
#21049=DIRECTION('',(-0.645833333333334,0.,0.763478425075362));
#21050=DIRECTION('',(-0.645833333333334,0.,0.763478425075362));
#21051=DIRECTION('',(0.,1.,0.));
#21052=DIRECTION('center_axis',(1.,-6.12303176911189E-17,0.));
#21053=DIRECTION('ref_axis',(-6.12303176911189E-17,-1.,0.));
#21054=DIRECTION('',(6.12303176911189E-17,1.,0.));
#21055=DIRECTION('',(0.,0.,-1.));
#21056=DIRECTION('center_axis',(1.,-6.12303176911189E-17,0.));
#21057=DIRECTION('ref_axis',(6.12303176911189E-17,1.,0.));
#21058=DIRECTION('center_axis',(0.,1.,0.));
#21059=DIRECTION('ref_axis',(1.,0.,0.));
#21060=DIRECTION('center_axis',(6.93889390390724E-15,0.,-1.));
#21061=DIRECTION('ref_axis',(-1.,0.,-6.93889390390724E-15));
#21062=DIRECTION('center_axis',(0.,1.,0.));
#21063=DIRECTION('ref_axis',(0.,0.,-1.));
#21064=DIRECTION('center_axis',(0.,1.,0.));
#21065=DIRECTION('ref_axis',(0.,0.,-1.));
#21066=DIRECTION('center_axis',(0.,1.,3.65204942310907E-16));
#21067=DIRECTION('ref_axis',(0.,-3.84077154464919E-16,1.));
#21068=DIRECTION('center_axis',(-0.928461531958395,0.,0.371428571428572));
#21069=DIRECTION('ref_axis',(0.371428571428572,0.,0.928461531958395));
#21070=DIRECTION('center_axis',(1.9280126729044E-32,3.65204942310907E-16,
-1.));
#21071=DIRECTION('ref_axis',(7.04119756982749E-48,-1.,-3.65204942310907E-16));
#21072=DIRECTION('center_axis',(0.,1.,0.));
#21073=DIRECTION('ref_axis',(-0.597614304667194,0.,0.801783725737275));
#21074=DIRECTION('center_axis',(0.,1.,0.));
#21075=DIRECTION('ref_axis',(0.,0.,1.));
#21076=DIRECTION('center_axis',(-1.,0.,0.));
#21077=DIRECTION('ref_axis',(0.,0.,-1.));
#21078=DIRECTION('center_axis',(-1.,-3.40699396374318E-16,-5.3631402309558E-16));
#21079=DIRECTION('ref_axis',(5.3631402309558E-16,1.82721863935746E-31,-1.));
#21080=DIRECTION('center_axis',(0.,0.,1.));
#21081=DIRECTION('ref_axis',(-1.,0.,0.));
#21082=DIRECTION('center_axis',(6.12303176911189E-17,1.,0.));
#21083=DIRECTION('ref_axis',(1.,-6.12303176911189E-17,0.));
#21084=DIRECTION('',(-6.12303176911189E-17,-1.,0.));
#21085=DIRECTION('center_axis',(-0.645833333333334,0.,0.763478425075362));
#21086=DIRECTION('ref_axis',(-0.763478425075362,0.,-0.645833333333334));
#21087=DIRECTION('center_axis',(-0.645833333333334,0.,0.763478425075362));
#21088=DIRECTION('ref_axis',(-0.763478425075362,0.,-0.645833333333334));
#21089=DIRECTION('center_axis',(5.8100520420011E-14,2.63746680760317E-14,
1.));
#21090=DIRECTION('ref_axis',(1.,1.73652799098504E-12,-5.81005204200568E-14));
#21091=DIRECTION('center_axis',(0.645833333333334,0.,0.763478425075362));
#21092=DIRECTION('ref_axis',(-0.763478425075362,0.,0.645833333333334));
#21093=DIRECTION('center_axis',(0.645833333333335,-8.40256683676267E-16,
0.763478425075361));
#21094=DIRECTION('ref_axis',(0.763478425075361,-4.92693589372649E-33,-0.645833333333335));
#21095=DIRECTION('center_axis',(0.,-1.,0.));
#21096=DIRECTION('ref_axis',(-1.22464679914735E-16,0.,1.));
#21097=DIRECTION('center_axis',(0.645833333333334,2.80085561225422E-16,
-0.763478425075361));
#21098=DIRECTION('ref_axis',(-0.763478425075361,-2.0725839158777E-31,-0.645833333333334));
#21099=DIRECTION('center_axis',(0.645833333333333,0.,-0.763478425075362));
#21100=DIRECTION('ref_axis',(0.763478425075362,0.,0.645833333333333));
#21101=DIRECTION('center_axis',(0.645833333333334,-3.36102673470506E-15,
-0.763478425075362));
#21102=DIRECTION('ref_axis',(-0.763478425075362,-1.51941949277112E-30,-0.645833333333334));
#21103=DIRECTION('center_axis',(0.,-1.,0.));
#21104=DIRECTION('ref_axis',(0.,0.,-1.));
#21105=DIRECTION('center_axis',(-0.645833333333334,0.,-0.763478425075362));
#21106=DIRECTION('ref_axis',(-0.763478425075362,0.,0.645833333333334));
#21107=DIRECTION('center_axis',(-0.645833333333334,0.,-0.763478425075362));
#21108=DIRECTION('ref_axis',(0.763478425075362,0.,-0.645833333333334));
#21109=DIRECTION('center_axis',(0.,1.,0.));
#21110=DIRECTION('ref_axis',(1.,0.,0.));
#21111=DIRECTION('center_axis',(0.,1.,0.));
#21112=DIRECTION('ref_axis',(0.,0.,1.));
#21113=DIRECTION('center_axis',(-0.0936591325004365,-0.988529372823465,
-0.11848057209734));
#21114=DIRECTION('ref_axis',(1.42799135152678E-16,0.119003673873871,-0.992893813861544));
#21115=DIRECTION('center_axis',(-0.564981881496666,-0.784698449006113,-0.255036894797377));
#21116=DIRECTION('ref_axis',(0.811534832728152,-0.58430404351578,-3.34937223530467E-16));
#21117=DIRECTION('center_axis',(1.,0.,0.));
#21118=DIRECTION('ref_axis',(0.,0.342020143325671,0.939692620785908));
#21119=DIRECTION('center_axis',(-1.,0.,0.));
#21120=DIRECTION('ref_axis',(0.,0.,-1.));
#21121=DIRECTION('center_axis',(0.,1.,0.));
#21122=DIRECTION('ref_axis',(1.,0.,0.));
#21123=DIRECTION('center_axis',(0.,-1.,0.));
#21124=DIRECTION('ref_axis',(0.,0.,-1.));
#21125=DIRECTION('center_axis',(1.,0.,0.));
#21126=DIRECTION('ref_axis',(0.,1.,0.));
#21127=DIRECTION('',(0.,0.939692620785908,-0.342020143325669));
#21128=DIRECTION('center_axis',(0.,0.342020143325669,0.939692620785908));
#21129=DIRECTION('ref_axis',(1.,0.,0.));
#21130=DIRECTION('center_axis',(0.,-0.844082777626919,0.53621289103641));
#21131=DIRECTION('ref_axis',(-1.,0.,0.));
#21132=DIRECTION('',(-1.,0.,0.));
#21133=DIRECTION('center_axis',(0.,-0.84408277762692,0.536212891036408));
#21134=DIRECTION('ref_axis',(-3.60441158372807E-15,-0.536212891036408,-0.84408277762692));
#21135=DIRECTION('',(-1.,0.,0.));
#21136=DIRECTION('center_axis',(0.,0.,-1.));
#21137=DIRECTION('ref_axis',(1.,0.,0.));
#21138=DIRECTION('center_axis',(0.,0.,1.));
#21139=DIRECTION('ref_axis',(1.,0.,0.));
#21140=DIRECTION('center_axis',(0.,0.,1.));
#21141=DIRECTION('ref_axis',(1.,0.,0.));
#45568=CARTESIAN_POINT('',(0.,0.,0.));
#45569=CARTESIAN_POINT('Origin',(6.61325378140121E-15,20.,8.67361737988404E-16));
#45570=CARTESIAN_POINT('',(-16.4311231709604,20.4751899333702,3.97184757758869));
#45571=CARTESIAN_POINT('',(-16.2371390735994,19.8911995661135,3.31402377493683));
#45572=CARTESIAN_POINT('Ctrl Pts',(-16.2371391035607,19.8912002375752,3.31402203697616));
#45573=CARTESIAN_POINT('Ctrl Pts',(-16.2259081885633,19.9279846491836,3.32803992581055));
#45574=CARTESIAN_POINT('Ctrl Pts',(-16.21610893629,19.9659892577548,3.35699075210906));
#45575=CARTESIAN_POINT('Ctrl Pts',(-16.2047647575198,20.0287863583858,3.41123974011251));
#45576=CARTESIAN_POINT('Ctrl Pts',(-16.2015113087813,20.0572758839873,3.43881950477961));
#45577=CARTESIAN_POINT('Ctrl Pts',(-16.1982197044851,20.1365633601703,3.5193334688907));
#45578=CARTESIAN_POINT('Ctrl Pts',(-16.2034921724796,20.187761246405,3.5761654848116));
#45579=CARTESIAN_POINT('Ctrl Pts',(-16.2318237402137,20.2873087487659,3.69280893423355));
#45580=CARTESIAN_POINT('Ctrl Pts',(-16.2566681168736,20.3365098327336,3.75433106955588));
#45581=CARTESIAN_POINT('Ctrl Pts',(-16.3283879292358,20.4193612299745,3.86971862334388));
#45582=CARTESIAN_POINT('Ctrl Pts',(-16.374261882323,20.45337712185,3.92346367802565));
#45583=CARTESIAN_POINT('Ctrl Pts',(-16.4311231758819,20.4751899320956,3.97184757096493));
#45584=CARTESIAN_POINT('',(-16.6268429955203,20.5,3.81948640102502));
#45585=CARTESIAN_POINT('Origin',(-16.6034196622342,20.0095539027816,3.82038660784234));
#45586=CARTESIAN_POINT('',(-17.0305720504421,20.5,1.));
#45587=CARTESIAN_POINT('Origin',(6.61325378140121E-15,20.5,8.67361737988404E-16));
#45588=CARTESIAN_POINT('',(-16.5314317768924,20.,0.970691514526271));
#45589=CARTESIAN_POINT('Origin',(-17.0305720504421,20.,1.));
#45590=CARTESIAN_POINT('',(-16.5433923268431,19.8911992509365,0.971393813304911));
#45591=CARTESIAN_POINT('Origin',(-17.0305720504421,20.,1.));
#45592=CARTESIAN_POINT('Origin',(6.61325378140121E-15,19.8911992509365,
8.67361737988404E-16));
#45593=CARTESIAN_POINT('Origin',(0.,12.,0.));
#45594=CARTESIAN_POINT('',(2.38806125833734E-15,8.00000000000001,19.5));
#45595=CARTESIAN_POINT('Origin',(4.8984254152895E-16,8.,1.70652395450943E-16));
#45596=CARTESIAN_POINT('',(2.38806125833734E-15,0.999999999999994,19.5));
#45597=CARTESIAN_POINT('',(2.38806125833734E-15,12.,19.5));
#45598=CARTESIAN_POINT('Origin',(6.12303176911187E-17,1.,3.29879455650267E-15));
#45599=CARTESIAN_POINT('Origin',(-6.,21.,7.));
#45600=CARTESIAN_POINT('',(-16.0233918507227,23.8433850776541,7.00000000000931));
#45601=CARTESIAN_POINT('',(-17.1604382595081,21.8496676031881,4.3051562348531));
#45602=CARTESIAN_POINT('Ctrl Pts',(-16.0233918597094,23.8433856528354,7.00000000001199));
#45603=CARTESIAN_POINT('Ctrl Pts',(-16.0284377251753,23.8433069425452,6.99144636015799));
#45604=CARTESIAN_POINT('Ctrl Pts',(-16.0334726453492,23.843189782176,6.98288622959523));
#45605=CARTESIAN_POINT('Ctrl Pts',(-16.0384965994218,23.843033968243,6.97431959907794));
#45606=CARTESIAN_POINT('Ctrl Pts',(-16.067918697475,23.8421214653128,6.92415030226116));
#45607=CARTESIAN_POINT('Ctrl Pts',(-16.0969646771329,23.8398833271083,6.87375808053725));
#45608=CARTESIAN_POINT('Ctrl Pts',(-16.1256302786017,23.8362782231697,6.82314031829582));
#45609=CARTESIAN_POINT('Ctrl Pts',(-16.1442199635033,23.8339403079396,6.79031462470237));
#45610=CARTESIAN_POINT('Ctrl Pts',(-16.1626496774753,23.8310276912692,6.75739407907483));
#45611=CARTESIAN_POINT('Ctrl Pts',(-16.1809181459987,23.8275229657671,6.72437791675892));
#45612=CARTESIAN_POINT('Ctrl Pts',(-16.2041375205119,23.8230684306814,6.68241410152068));
#45613=CARTESIAN_POINT('Ctrl Pts',(-16.2270964121805,23.8176574074361,6.6402960321563));
#45614=CARTESIAN_POINT('Ctrl Pts',(-16.2497921838513,23.8112536349832,6.59802202944585));
#45615=CARTESIAN_POINT('Ctrl Pts',(-16.2561057824771,23.809472208489,6.58626208185338));
#45616=CARTESIAN_POINT('Ctrl Pts',(-16.2623990192776,23.8076139509515,6.57449005186631));
#45617=CARTESIAN_POINT('Ctrl Pts',(-16.2686718368427,23.8056780738639,6.5627059101453));
#45618=CARTESIAN_POINT('Ctrl Pts',(-16.2736736063734,23.8041344595419,6.55330956466016));
#45619=CARTESIAN_POINT('Ctrl Pts',(-16.2786623917353,23.8025413849404,6.54390551776014));
#45620=CARTESIAN_POINT('Ctrl Pts',(-16.2836381623927,23.8008983485357,6.53449375383592));
#45621=CARTESIAN_POINT('Ctrl Pts',(-16.2901995856383,23.7987317178766,6.52208269817312));
#45622=CARTESIAN_POINT('Ctrl Pts',(-16.2967376415088,23.7964784648201,6.50965962858277));
#45623=CARTESIAN_POINT('Ctrl Pts',(-16.3032535167685,23.7941370090411,6.49722211474457));
#45624=CARTESIAN_POINT('Ctrl Pts',(-16.3078757650997,23.7924760211254,6.48839915922591));
#45625=CARTESIAN_POINT('Ctrl Pts',(-16.3124894944245,23.7907696002991,6.47956383625479));
#45626=CARTESIAN_POINT('Ctrl Pts',(-16.3170869282503,23.7890203161444,6.47073105701516));
#45627=CARTESIAN_POINT('Ctrl Pts',(-16.318180251042,23.7886043161957,6.46863052023255));
#45628=CARTESIAN_POINT('Ctrl Pts',(-16.3192726250444,23.7881859023917,6.46653017992206));
#45629=CARTESIAN_POINT('Ctrl Pts',(-16.320363939594,23.7877651117504,6.46443024841133));
#45630=CARTESIAN_POINT('Ctrl Pts',(-16.3260389472779,23.7855769340861,6.45351027354005));
#45631=CARTESIAN_POINT('Ctrl Pts',(-16.3316845634806,23.7833249057076,6.44260286155155));
#45632=CARTESIAN_POINT('Ctrl Pts',(-16.3373010110403,23.7810090011584,6.43170801330259));
#45633=CARTESIAN_POINT('Ctrl Pts',(-16.3597169306986,23.7717659467615,6.38822535982041));
#45634=CARTESIAN_POINT('Ctrl Pts',(-16.3816683400294,23.7615059125948,6.34494266243544));
#45635=CARTESIAN_POINT('Ctrl Pts',(-16.4031683995334,23.7502232140424,6.30186134796477));
#45636=CARTESIAN_POINT('Ctrl Pts',(-16.4172323732936,23.7428427890555,6.27368028752822));
#45637=CARTESIAN_POINT('Ctrl Pts',(-16.4311033535401,23.7350253864853,6.24558518657362));
#45638=CARTESIAN_POINT('Ctrl Pts',(-16.4447844323403,23.7267668059867,6.21757733753011));
#45639=CARTESIAN_POINT('Ctrl Pts',(-16.4727067748196,23.7099114894986,6.1604148312306));
#45640=CARTESIAN_POINT('Ctrl Pts',(-16.4998355812374,23.6912200670357,6.10362158299839));
#45641=CARTESIAN_POINT('Ctrl Pts',(-16.5261925108193,23.6706610942453,6.04721999865201));
#45642=CARTESIAN_POINT('Ctrl Pts',(-16.5383895772972,23.6611471196732,6.02111931527783));
#45643=CARTESIAN_POINT('Ctrl Pts',(-16.5504213408844,23.6512332657452,5.99510248283814));
#45644=CARTESIAN_POINT('Ctrl Pts',(-16.5622894775869,23.6409135376314,5.96917275294547));
#45645=CARTESIAN_POINT('Ctrl Pts',(-16.5883707008436,23.6182350717835,5.91219000230245));
#45646=CARTESIAN_POINT('Ctrl Pts',(-16.613662202772,23.593596548317,5.85562799479922));
#45647=CARTESIAN_POINT('Ctrl Pts',(-16.6381830439851,23.5669338767108,5.79952074742108));
#45648=CARTESIAN_POINT('Ctrl Pts',(-16.6489320806676,23.5552459402058,5.77492538974222));
#45649=CARTESIAN_POINT('Ctrl Pts',(-16.6595330305966,23.543169167367,5.75041737025986));
#45650=CARTESIAN_POINT('Ctrl Pts',(-16.6699871278393,23.5306950852284,5.72600068773709));
#45651=CARTESIAN_POINT('Ctrl Pts',(-16.687138187239,23.510230025573,5.68594252082273));
#45652=CARTESIAN_POINT('Ctrl Pts',(-16.7038942239911,23.4886956751937,5.64613036475662));
#45653=CARTESIAN_POINT('Ctrl Pts',(-16.7202610350444,23.4660543595333,5.60658198567009));
#45654=CARTESIAN_POINT('Ctrl Pts',(-16.7268161206599,23.4569862666644,5.59074243024164));
#45655=CARTESIAN_POINT('Ctrl Pts',(-16.7333087571338,23.4477405918434,5.57494516833557));
#45656=CARTESIAN_POINT('Ctrl Pts',(-16.7397393243964,23.4383148767634,5.55919131448836));
#45657=CARTESIAN_POINT('Ctrl Pts',(-16.7413367132527,23.4359734764459,5.55527796912543));
#45658=CARTESIAN_POINT('Ctrl Pts',(-16.7429302691987,23.433620942759,5.55136731108168));
#45659=CARTESIAN_POINT('Ctrl Pts',(-16.7445199969512,23.4312572278318,5.54745936122601));
#45660=CARTESIAN_POINT('Ctrl Pts',(-16.7485147239046,23.425317597153,5.53763931965202));
#45661=CARTESIAN_POINT('Ctrl Pts',(-16.7524852872413,23.4193073729298,5.52783639310678));
#45662=CARTESIAN_POINT('Ctrl Pts',(-16.7564317657962,23.4132257989771,5.51805092053644));
#45663=CARTESIAN_POINT('Ctrl Pts',(-16.7588161175821,23.4095514823646,5.51213881214064));
#45664=CARTESIAN_POINT('Ctrl Pts',(-16.7611918475176,23.4058508582643,5.50623265323961));
#45665=CARTESIAN_POINT('Ctrl Pts',(-16.7635588441968,23.4021239495519,5.50033283496077));
#45666=CARTESIAN_POINT('Ctrl Pts',(-16.7651096006317,23.3996822360849,5.49646752275275));
#45667=CARTESIAN_POINT('Ctrl Pts',(-16.7666564028141,23.3972295317442,5.49260543324729));
#45668=CARTESIAN_POINT('Ctrl Pts',(-16.7681985799081,23.3947669372142,5.48874830563239));
#45669=CARTESIAN_POINT('Ctrl Pts',(-16.7705519340973,23.3910090308258,5.48286234904143));
#45670=CARTESIAN_POINT('Ctrl Pts',(-16.7728944619133,23.3872281839827,5.47698808791221));
#45671=CARTESIAN_POINT('Ctrl Pts',(-16.7752239052603,23.3834281185936,5.47113139231683));
#45672=CARTESIAN_POINT('Ctrl Pts',(-16.7790773875821,23.3771418593388,5.46144295195627));
#45673=CARTESIAN_POINT('Ctrl Pts',(-16.7828979733183,23.3707984623358,5.45179534097987));
#45674=CARTESIAN_POINT('Ctrl Pts',(-16.7866861214173,23.3643980243537,5.44218853694711));
#45675=CARTESIAN_POINT('Ctrl Pts',(-16.8018147227821,23.338836807564,5.40382216245424));
#45676=CARTESIAN_POINT('Ctrl Pts',(-16.8164262027409,23.3123662713952,5.36610626913502));
#45677=CARTESIAN_POINT('Ctrl Pts',(-16.8305477690303,23.2849889629749,5.3290423500846));
#45678=CARTESIAN_POINT('Ctrl Pts',(-16.8390627181896,23.2684811348389,5.3066937394637));
#45679=CARTESIAN_POINT('Ctrl Pts',(-16.8473998107328,23.2516441263546,5.28458176432105));
#45680=CARTESIAN_POINT('Ctrl Pts',(-16.8555640341602,23.2344766403772,5.26270826111354));
#45681=CARTESIAN_POINT('Ctrl Pts',(-16.8743784114623,23.1949143278836,5.21230097548252));
#45682=CARTESIAN_POINT('Ctrl Pts',(-16.8922740093455,23.1536002626368,5.16316463641716));
#45683=CARTESIAN_POINT('Ctrl Pts',(-16.9093101088097,23.1105258117712,5.11532790787435));
#45684=CARTESIAN_POINT('Ctrl Pts',(-16.916852396087,23.091455725721,5.09414944799066));
#45685=CARTESIAN_POINT('Ctrl Pts',(-16.9242262045456,23.0720406582638,5.0732256601497));
#45686=CARTESIAN_POINT('Ctrl Pts',(-16.9314355358393,23.0522772513815,5.05256120178904));
#45687=CARTESIAN_POINT('Ctrl Pts',(-16.9474705650594,23.0083193870615,5.00659921445182));
#45688=CARTESIAN_POINT('Ctrl Pts',(-16.9626931835324,22.9626383608009,4.96192034827594));
#45689=CARTESIAN_POINT('Ctrl Pts',(-16.977149247726,22.9151967856811,4.91857454139849));
#45690=CARTESIAN_POINT('Ctrl Pts',(-16.9838731661397,22.8931303866773,4.89841319837217));
#45691=CARTESIAN_POINT('Ctrl Pts',(-16.99043100828,22.8706825154872,4.8785407471639));
#45692=CARTESIAN_POINT('Ctrl Pts',(-16.9968265198859,22.8478469378767,4.85896430688065));
#45693=CARTESIAN_POINT('Ctrl Pts',(-17.0003660793906,22.8352087173936,4.84812983740528));
#45694=CARTESIAN_POINT('Ctrl Pts',(-17.0038557015822,22.8224526137342,4.83738677511585));
#45695=CARTESIAN_POINT('Ctrl Pts',(-17.0072962876948,22.809576737179,4.82673558374586));
#45696=CARTESIAN_POINT('Ctrl Pts',(-17.0121178529662,22.7915327536236,4.81180922738465));
#45697=CARTESIAN_POINT('Ctrl Pts',(-17.0168430837008,22.7732534583247,4.79706337239252));
#45698=CARTESIAN_POINT('Ctrl Pts',(-17.021474163257,22.7547327835074,4.78250002849357));
#45699=CARTESIAN_POINT('Ctrl Pts',(-17.0229427117219,22.748859744998,4.77788188793504));
#45700=CARTESIAN_POINT('Ctrl Pts',(-17.0244024446751,22.7429597062764,4.77328002892413));
#45701=CARTESIAN_POINT('Ctrl Pts',(-17.0258519078165,22.7370387750722,4.76869934923281));
#45702=CARTESIAN_POINT('Ctrl Pts',(-17.0266859568084,22.7336317572868,4.76606353796613));
#45703=CARTESIAN_POINT('Ctrl Pts',(-17.0275165314831,22.7302181246644,4.76343497366233));
#45704=CARTESIAN_POINT('Ctrl Pts',(-17.0283433567152,22.726799039008,4.7608145820925));
#45705=CARTESIAN_POINT('Ctrl Pts',(-17.0306064360811,22.7174407588067,4.75364238431455));
#45706=CARTESIAN_POINT('Ctrl Pts',(-17.0328406947071,22.7080449324597,4.74653378214495));
#45707=CARTESIAN_POINT('Ctrl Pts',(-17.035046758628,22.6986113109312,4.73948821377146));
#45708=CARTESIAN_POINT('Ctrl Pts',(-17.0365196257533,22.6923130024866,4.73478427661965));
#45709=CARTESIAN_POINT('Ctrl Pts',(-17.0379799702854,22.6859978859778,4.73010837023522));
#45710=CARTESIAN_POINT('Ctrl Pts',(-17.039427949088,22.6796658611914,4.72546037207139));
#45711=CARTESIAN_POINT('Ctrl Pts',(-17.043837088838,22.6603846520101,4.71130707547284));
#45712=CARTESIAN_POINT('Ctrl Pts',(-17.0481310680966,22.640947326536,4.69741303542798));
#45713=CARTESIAN_POINT('Ctrl Pts',(-17.0523146503055,22.6213547488622,4.68377752410598));
#45714=CARTESIAN_POINT('Ctrl Pts',(-17.0631983357952,22.570384206709,4.648304427294));
#45715=CARTESIAN_POINT('Ctrl Pts',(-17.0733323397321,22.5183633805738,4.61458142439873));
#45716=CARTESIAN_POINT('Ctrl Pts',(-17.0827819382676,22.4653091749687,4.58259528972156));
#45717=CARTESIAN_POINT('Ctrl Pts',(-17.0878616725955,22.4367893105069,4.56540079561412));
#45718=CARTESIAN_POINT('Ctrl Pts',(-17.0927435475338,22.4079708208665,4.54870821341221));
#45719=CARTESIAN_POINT('Ctrl Pts',(-17.0974346071329,22.3788534273067,4.53252048432898));
#45720=CARTESIAN_POINT('Ctrl Pts',(-17.1058978315018,22.3263222177721,4.50331591330117));
#45721=CARTESIAN_POINT('Ctrl Pts',(-17.1137418031168,22.2728181444527,4.47575463281059));
#45722=CARTESIAN_POINT('Ctrl Pts',(-17.1210087870872,22.2183386823111,4.44985278433895));
#45723=CARTESIAN_POINT('Ctrl Pts',(-17.125262903816,22.1864462229058,4.43468975558594));
#45724=CARTESIAN_POINT('Ctrl Pts',(-17.1293192739918,22.154219575904,4.42009527073905));
#45725=CARTESIAN_POINT('Ctrl Pts',(-17.1331830538353,22.1216546244272,4.40607883828957));
#45726=CARTESIAN_POINT('Ctrl Pts',(-17.1384150443394,22.0775580340953,4.38709901944727));
#45727=CARTESIAN_POINT('Ctrl Pts',(-17.1432952592276,22.0328413580963,4.36917924964466));
#45728=CARTESIAN_POINT('Ctrl Pts',(-17.1478360657817,21.9874939088656,4.35234281173029));
#45729=CARTESIAN_POINT('Ctrl Pts',(-17.1488284826203,21.9775829884882,4.34866312084493));
#45730=CARTESIAN_POINT('Ctrl Pts',(-17.1498047181489,21.9676413186292,4.34503494964224));
#45731=CARTESIAN_POINT('Ctrl Pts',(-17.1507648504972,21.9576696303041,4.34145885652359));
#45732=CARTESIAN_POINT('Ctrl Pts',(-17.1518385084627,21.946518894034,4.3374599277622));
#45733=CARTESIAN_POINT('Ctrl Pts',(-17.1528919489068,21.9353305256573,4.33352628632849));
#45734=CARTESIAN_POINT('Ctrl Pts',(-17.1539252278949,21.924105493081,4.32965880561775));
#45735=CARTESIAN_POINT('Ctrl Pts',(-17.1540818609778,21.9224039086308,4.32907254050056));
#45736=CARTESIAN_POINT('Ctrl Pts',(-17.1542380525564,21.9207012217312,4.32848771335121));
#45737=CARTESIAN_POINT('Ctrl Pts',(-17.1543937822607,21.9189976751517,4.32790440467035));
#45738=CARTESIAN_POINT('Ctrl Pts',(-17.1552641853424,21.9094762277235,4.32464418096637));
#45739=CARTESIAN_POINT('Ctrl Pts',(-17.1561212020475,21.8999164524419,4.32142744214349));
#45740=CARTESIAN_POINT('Ctrl Pts',(-17.1569616836063,21.8903543830217,4.31826660511824));
#45741=CARTESIAN_POINT('Ctrl Pts',(-17.1571359480896,21.8883717945047,4.31761124079123));
#45742=CARTESIAN_POINT('Ctrl Pts',(-17.1573095927471,21.8863881041705,4.31695793879396));
#45743=CARTESIAN_POINT('Ctrl Pts',(-17.1574826225619,21.8844032604135,4.31630668534007));
#45744=CARTESIAN_POINT('Ctrl Pts',(-17.1584901791008,21.8728454701626,4.31251442169526));
#45745=CARTESIAN_POINT('Ctrl Pts',(-17.1594752876153,21.8612669031643,4.30879763630566));
#45746=CARTESIAN_POINT('Ctrl Pts',(-17.1604382596112,21.8496676051728,4.30515622855862));
#45747=CARTESIAN_POINT('',(-28.4921884534998,21.8412135273285,4.48858057664302));
#45748=CARTESIAN_POINT('Ctrl Pts',(-17.1604382594737,21.8496676025262,4.30515623695262));
#45749=CARTESIAN_POINT('Ctrl Pts',(-20.937690036586,21.8469996129353,4.36619867482251));
#45750=CARTESIAN_POINT('Ctrl Pts',(-24.7149401916638,21.8441900251035,4.42733521081778));
#45751=CARTESIAN_POINT('Ctrl Pts',(-28.4921884534998,21.8412135273285,4.48858057664302));
#45752=CARTESIAN_POINT('',(-28.492188453501,20.1587864726715,4.48858057664304));
#45753=CARTESIAN_POINT('Ctrl Pts',(-28.4921884534998,21.8412135273285,4.48858057664302));
#45754=CARTESIAN_POINT('Ctrl Pts',(-28.5227165270159,21.8411894664569,4.48907556589413));
#45755=CARTESIAN_POINT('Ctrl Pts',(-28.5530697764421,21.839992183168,4.4891736621749));
#45756=CARTESIAN_POINT('Ctrl Pts',(-28.5832520807999,21.8376467249157,4.48888855370485));
#45757=CARTESIAN_POINT('Ctrl Pts',(-28.5858424780989,21.8374454258814,4.48886408426071));
#45758=CARTESIAN_POINT('Ctrl Pts',(-28.5884316135345,21.8372356594637,4.48883678885867));
#45759=CARTESIAN_POINT('Ctrl Pts',(-28.5910194901533,21.8370174426294,4.4888066765942));
#45760=CARTESIAN_POINT('Ctrl Pts',(-28.6185845479042,21.8346930815706,4.48848593243537));
#45761=CARTESIAN_POINT('Ctrl Pts',(-28.6460068811572,21.8314097542959,4.48784553144024));
#45762=CARTESIAN_POINT('Ctrl Pts',(-28.6732861919453,21.8271634702414,4.48689681709569));
#45763=CARTESIAN_POINT('Ctrl Pts',(-28.6782462125312,21.8263913958848,4.48672431850452));
#45764=CARTESIAN_POINT('Ctrl Pts',(-28.6832014941128,21.8255874235304,4.48654160704114));
#45765=CARTESIAN_POINT('Ctrl Pts',(-28.6881520409208,21.8247515308658,4.48634875274379));
#45766=CARTESIAN_POINT('Ctrl Pts',(-28.7129848589572,21.8205585454759,4.485381361492));
#45767=CARTESIAN_POINT('Ctrl Pts',(-28.7376985199429,21.8155624946819,4.48415871300685));
#45768=CARTESIAN_POINT('Ctrl Pts',(-28.7622902462614,21.8097419383589,4.48269023678948));
#45769=CARTESIAN_POINT('Ctrl Pts',(-28.7694071606622,21.8080574530739,4.48226525566358));
#45770=CARTESIAN_POINT('Ctrl Pts',(-28.7765112054826,21.8063044074594,4.48181980291049));
#45771=CARTESIAN_POINT('Ctrl Pts',(-28.7836050970554,21.8044816528127,4.48135395516118));
#45772=CARTESIAN_POINT('Ctrl Pts',(-28.7912106045476,21.8025274399551,4.48085451017937));
#45773=CARTESIAN_POINT('Ctrl Pts',(-28.7988145600856,21.8004896679887,4.48033076967421));
#45774=CARTESIAN_POINT('Ctrl Pts',(-28.8063988576059,21.7983729620984,4.4797845327618));
#45775=CARTESIAN_POINT('Ctrl Pts',(-28.8137280605548,21.7963274506966,4.47925666829203));
#45776=CARTESIAN_POINT('Ctrl Pts',(-28.8210440935422,21.794206699072,4.47870739914648));
#45777=CARTESIAN_POINT('Ctrl Pts',(-28.8283192684753,21.7920178352031,4.47813911019099));
#45778=CARTESIAN_POINT('Ctrl Pts',(-28.8290919422524,21.7917853627569,4.47807875398269));
#45779=CARTESIAN_POINT('Ctrl Pts',(-28.829864237367,21.7915520981649,4.47801817707474));
#45780=CARTESIAN_POINT('Ctrl Pts',(-28.8306361287375,21.7913180475491,4.47795738170932));
#45781=CARTESIAN_POINT('Ctrl Pts',(-28.8371320454856,21.7893483749078,4.47744575319842));
#45782=CARTESIAN_POINT('Ctrl Pts',(-28.8436017105944,21.7873228425933,4.47691861764328));
#45783=CARTESIAN_POINT('Ctrl Pts',(-28.8500445700105,21.7852417342137,4.47637649647148));
#45784=CARTESIAN_POINT('Ctrl Pts',(-28.8589452391665,21.782366728573,4.47562756794751));
#45785=CARTESIAN_POINT('Ctrl Pts',(-28.867795030091,21.7793853473532,4.47484994645555));
#45786=CARTESIAN_POINT('Ctrl Pts',(-28.8765942156564,21.7762977216211,4.47404486510076));
#45787=CARTESIAN_POINT('Ctrl Pts',(-28.8963000577746,21.769382960619,4.47224187936397));
#45788=CARTESIAN_POINT('Ctrl Pts',(-28.9157526841421,21.761936297264,4.47030119654534));
#45789=CARTESIAN_POINT('Ctrl Pts',(-28.9349503511768,21.7539513728655,4.46823635605871));
#45790=CARTESIAN_POINT('Ctrl Pts',(-28.9450156597226,21.7497648887661,4.46715376323334));
#45791=CARTESIAN_POINT('Ctrl Pts',(-28.9550106747551,21.7454301254848,4.46603695502191));
#45792=CARTESIAN_POINT('Ctrl Pts',(-28.964935373711,21.740946115794,4.46488795892171));
#45793=CARTESIAN_POINT('Ctrl Pts',(-28.9823926751867,21.7330588529822,4.46286690302823));
#45794=CARTESIAN_POINT('Ctrl Pts',(-28.999632408897,21.7247098510798,4.46074616568145));
#45795=CARTESIAN_POINT('Ctrl Pts',(-29.0166492430745,21.7158853181679,4.45853674003619));
#45796=CARTESIAN_POINT('Ctrl Pts',(-29.0273929158853,21.7103139002811,4.45714180687854));
#45797=CARTESIAN_POINT('Ctrl Pts',(-29.0380469194319,21.7045529828368,4.45571153450151));
#45798=CARTESIAN_POINT('Ctrl Pts',(-29.0486108330097,21.6985982905204,4.45424862705299));
#45799=CARTESIAN_POINT('Ctrl Pts',(-29.0621240238921,21.6909811424507,4.45237729902201));
#45800=CARTESIAN_POINT('Ctrl Pts',(-29.0754894651515,21.6830463951951,4.45045254736087));
#45801=CARTESIAN_POINT('Ctrl Pts',(-29.088703716323,21.6747809730397,4.44848022524981));
#45802=CARTESIAN_POINT('Ctrl Pts',(-29.0908231994901,21.6734552510672,4.44816387712988));
#45803=CARTESIAN_POINT('Ctrl Pts',(-29.0929392811997,21.6721206654223,4.44784622555517));
#45804=CARTESIAN_POINT('Ctrl Pts',(-29.0950506645488,21.6707780193494,4.44752749694437));
#45805=CARTESIAN_POINT('Ctrl Pts',(-29.0994868545906,21.6679570095404,4.44685782192305));
#45806=CARTESIAN_POINT('Ctrl Pts',(-29.1039021069988,21.6651005315295,4.44618341803519));
#45807=CARTESIAN_POINT('Ctrl Pts',(-29.1082854328805,21.6622153371953,4.44550622678895));
#45808=CARTESIAN_POINT('Ctrl Pts',(-29.1102174113624,21.6609436696259,4.44520775048323));
#45809=CARTESIAN_POINT('Ctrl Pts',(-29.1121438952947,21.6596659942202,4.44490862929262));
#45810=CARTESIAN_POINT('Ctrl Pts',(-29.1140649936888,21.6583822331944,4.44460887284627));
#45811=CARTESIAN_POINT('Ctrl Pts',(-29.1185508902551,21.6553845631138,4.44390892097626));
#45812=CARTESIAN_POINT('Ctrl Pts',(-29.1230068386011,21.6523541042434,4.44320559705709));
#45813=CARTESIAN_POINT('Ctrl Pts',(-29.1274327932882,21.6492907567066,4.44249923281721));
#45814=CARTESIAN_POINT('Ctrl Pts',(-29.129202666098,21.6480657700323,4.44221676836596));
#45815=CARTESIAN_POINT('Ctrl Pts',(-29.1309677573007,21.6468355354338,4.44193381959285));
#45816=CARTESIAN_POINT('Ctrl Pts',(-29.1327280554723,21.6456000401895,4.44165040684993));
#45817=CARTESIAN_POINT('Ctrl Pts',(-29.1450526742288,21.6369497966643,4.43966611006221));
#45818=CARTESIAN_POINT('Ctrl Pts',(-29.157142362216,21.6280416455197,4.43765903675389));
#45819=CARTESIAN_POINT('Ctrl Pts',(-29.168996237874,21.6188730413405,4.43563686577132));
#45820=CARTESIAN_POINT('Ctrl Pts',(-29.1793869162976,21.6108361747184,4.43386430386807));
#45821=CARTESIAN_POINT('Ctrl Pts',(-29.1895954231523,21.6025984363405,4.43207994577978));
#45822=CARTESIAN_POINT('Ctrl Pts',(-29.1996207750758,21.5941571047765,4.43028895762304));
#45823=CARTESIAN_POINT('Ctrl Pts',(-29.2124696321858,21.5833383860013,4.42799356180181));
#45824=CARTESIAN_POINT('Ctrl Pts',(-29.2250176217377,21.5721852553999,4.42568718330686));
#45825=CARTESIAN_POINT('Ctrl Pts',(-29.237256114022,21.5606866723982,4.42338074627525));
#45826=CARTESIAN_POINT('Ctrl Pts',(-29.2466554289126,21.5518556170755,4.42160937383559));
#45827=CARTESIAN_POINT('Ctrl Pts',(-29.2558718272431,21.5428205251124,4.41983791271102));
#45828=CARTESIAN_POINT('Ctrl Pts',(-29.264901681043,21.53357566893,4.41807146387376));
#45829=CARTESIAN_POINT('Ctrl Pts',(-29.2768030222565,21.5213909547215,4.41574328549854));
#45830=CARTESIAN_POINT('Ctrl Pts',(-29.2883804475871,21.5088419871408,4.41342370773151));
#45831=CARTESIAN_POINT('Ctrl Pts',(-29.299617742575,21.4959091454236,4.41112518095054));
#45832=CARTESIAN_POINT('Ctrl Pts',(-29.3045585725327,21.4902228150511,4.41011456140285));
#45833=CARTESIAN_POINT('Ctrl Pts',(-29.3094337349238,21.4844622768702,4.40910802533679));
#45834=CARTESIAN_POINT('Ctrl Pts',(-29.3142416822275,21.4786255847451,4.40810663827177));
#45835=CARTESIAN_POINT('Ctrl Pts',(-29.3172794243947,21.4749378642554,4.40747394504097));
#45836=CARTESIAN_POINT('Ctrl Pts',(-29.3202907592376,21.4712191361926,4.40684320370065));
#45837=CARTESIAN_POINT('Ctrl Pts',(-29.3232747701016,21.4674695968391,4.40621481258309));
#45838=CARTESIAN_POINT('Ctrl Pts',(-29.325013664013,21.4652846010567,4.40584862574996));
#45839=CARTESIAN_POINT('Ctrl Pts',(-29.3267406732683,21.4630923936772,4.40548379116715));
#45840=CARTESIAN_POINT('Ctrl Pts',(-29.3284556614909,21.4608931100365,4.4051203821878));
#45841=CARTESIAN_POINT('Ctrl Pts',(-29.3377716134452,21.4489464269854,4.40314631580824));
#45842=CARTESIAN_POINT('Ctrl Pts',(-29.3467234992276,21.4368026456522,4.40121620315188));
#45843=CARTESIAN_POINT('Ctrl Pts',(-29.3553119242716,21.4244611435133,4.39933786704563));
#45844=CARTESIAN_POINT('Ctrl Pts',(-29.3616566833125,21.4153437725315,4.39795023311611));
#45845=CARTESIAN_POINT('Ctrl Pts',(-29.3678027743186,21.4061172031824,4.39659065710816));
#45846=CARTESIAN_POINT('Ctrl Pts',(-29.3737481428319,21.3967828893906,4.39526271743198));
#45847=CARTESIAN_POINT('Ctrl Pts',(-29.3838983743266,21.380846880442,4.39299559217406));
#45848=CARTESIAN_POINT('Ctrl Pts',(-29.3934673651695,21.3645919103031,4.39081973562068));
#45849=CARTESIAN_POINT('Ctrl Pts',(-29.4024399499354,21.3480104267181,4.38875131818053));
#45850=CARTESIAN_POINT('Ctrl Pts',(-29.4069596931346,21.3396578672694,4.38770939816504));
#45851=CARTESIAN_POINT('Ctrl Pts',(-29.4113277352643,21.331222226145,4.38669471346358));
#45852=CARTESIAN_POINT('Ctrl Pts',(-29.4155423013294,21.3227021231074,4.38570936360752));
#45853=CARTESIAN_POINT('Ctrl Pts',(-29.4245951987033,21.3044009226462,4.38359282990357));
#45854=CARTESIAN_POINT('Ctrl Pts',(-29.4329402271217,21.2857101671811,4.3816114641524));
#45855=CARTESIAN_POINT('Ctrl Pts',(-29.4405414932869,21.2666089081952,4.37978733052507));
#45856=CARTESIAN_POINT('Ctrl Pts',(-29.4433583616853,21.2595303857965,4.37911134520135));
#45857=CARTESIAN_POINT('Ctrl Pts',(-29.446072864589,21.2523953721124,4.37845695150955));
#45858=CARTESIAN_POINT('Ctrl Pts',(-29.4486830987638,21.2452026419165,4.3778253136806));
#45859=CARTESIAN_POINT('Ctrl Pts',(-29.4512342841163,21.2381726259518,4.37720796478796));
#45860=CARTESIAN_POINT('Ctrl Pts',(-29.4536856689904,21.2310874002537,4.37661236210478));
#45861=CARTESIAN_POINT('Ctrl Pts',(-29.4560347196898,21.2239455260892,4.37603966694944));
#45862=CARTESIAN_POINT('Ctrl Pts',(-29.45808264445,21.2177191722093,4.37554038586156));
#45863=CARTESIAN_POINT('Ctrl Pts',(-29.4600529077877,21.2114495063001,4.37505849678349));
#45864=CARTESIAN_POINT('Ctrl Pts',(-29.4619435946022,21.2051358286219,4.37459481009537));
#45865=CARTESIAN_POINT('Ctrl Pts',(-29.4622466982348,21.2041236574763,4.37452047461133));
#45866=CARTESIAN_POINT('Ctrl Pts',(-29.462547565049,21.2031109894319,4.37444665410515));
#45867=CARTESIAN_POINT('Ctrl Pts',(-29.4628461926641,21.2020978304696,4.37437335042911));
#45868=CARTESIAN_POINT('Ctrl Pts',(-29.4650075867848,21.1947648320685,4.37384279623265));
#45869=CARTESIAN_POINT('Ctrl Pts',(-29.4670484442119,21.1874164428921,4.37334005434292));
#45870=CARTESIAN_POINT('Ctrl Pts',(-29.4689700849412,21.1800528117656,4.37286547380907));
#45871=CARTESIAN_POINT('Ctrl Pts',(-29.4703195306758,21.1748818032293,4.37253220616575));
#45872=CARTESIAN_POINT('Ctrl Pts',(-29.4716100602321,21.1697029993436,4.37221280780103));
#45873=CARTESIAN_POINT('Ctrl Pts',(-29.4728416797525,21.164517221623,4.37190746254535));
#45874=CARTESIAN_POINT('Ctrl Pts',(-29.478625474554,21.1401643482511,4.37047353406884));
#45875=CARTESIAN_POINT('Ctrl Pts',(-29.4831166515775,21.1156432655594,4.36934845920679));
#45876=CARTESIAN_POINT('Ctrl Pts',(-29.4863141901159,21.0909577508463,4.36854519159516));
#45877=CARTESIAN_POINT('Ctrl Pts',(-29.4866678555618,21.0882273963985,4.36845634575493));
#45878=CARTESIAN_POINT('Ctrl Pts',(-29.4870056852833,21.0854950132696,4.36837143579129));
#45879=CARTESIAN_POINT('Ctrl Pts',(-29.4873276786664,21.0827605984085,4.36829047900386));
#45880=CARTESIAN_POINT('Ctrl Pts',(-29.4905367896416,21.0555083590705,4.36748363225269));
#45881=CARTESIAN_POINT('Ctrl Pts',(-29.4921729809254,21.0280543316155,4.36706935322525));
#45882=CARTESIAN_POINT('Ctrl Pts',(-29.4921883426906,21.0003922828609,4.3670654720775));
#45883=CARTESIAN_POINT('Ctrl Pts',(-29.4921883566808,21.0003670905664,4.36706546854288));
#45884=CARTESIAN_POINT('Ctrl Pts',(-29.4921883693259,21.000341898099,4.36706546534868));
#45885=CARTESIAN_POINT('Ctrl Pts',(-29.4921883806259,21.0003167054589,4.36706546249491));
#45886=CARTESIAN_POINT('Ctrl Pts',(-29.4921917825163,20.9927323980165,4.3670646033626));
#45887=CARTESIAN_POINT('Ctrl Pts',(-29.4920730566502,20.9851324156375,4.3670946013449));
#45888=CARTESIAN_POINT('Ctrl Pts',(-29.4918305391955,20.9775165461871,4.36715584865301));
#45889=CARTESIAN_POINT('Ctrl Pts',(-29.4916325392323,20.9712986767451,4.36720585315584));
#45890=CARTESIAN_POINT('Ctrl Pts',(-29.491351642387,20.9650645241479,4.36727677879092));
#45891=CARTESIAN_POINT('Ctrl Pts',(-29.4909881144146,20.9588345028022,4.36736851454079));
#45892=CARTESIAN_POINT('Ctrl Pts',(-29.4909049012731,20.9574084236909,4.36738951325482));
#45893=CARTESIAN_POINT('Ctrl Pts',(-29.4908173655457,20.955982561579,4.3674116001301));
#45894=CARTESIAN_POINT('Ctrl Pts',(-29.4907255238541,20.9545571623216,4.3674347698338));
#45895=CARTESIAN_POINT('Ctrl Pts',(-29.4903701470481,20.9490416515945,4.36752442383679));
#45896=CARTESIAN_POINT('Ctrl Pts',(-29.4899501892045,20.9435311774064,4.36763032274499));
#45897=CARTESIAN_POINT('Ctrl Pts',(-29.4894659444528,20.938027187658,4.36775233853024));
#45898=CARTESIAN_POINT('Ctrl Pts',(-29.4892783277562,20.9358947115263,4.36779961255538));
#45899=CARTESIAN_POINT('Ctrl Pts',(-29.4890809366929,20.933762242885,4.36784933719275));
#45900=CARTESIAN_POINT('Ctrl Pts',(-29.4888739485811,20.9316311318625,4.36790146339755));
#45901=CARTESIAN_POINT('Ctrl Pts',(-29.488405606424,20.9268091683002,4.36801940688222));
#45902=CARTESIAN_POINT('Ctrl Pts',(-29.4878877219468,20.9219900447715,4.36814974506808));
#45903=CARTESIAN_POINT('Ctrl Pts',(-29.4873219268749,20.9171880702865,4.36829200382837));
#45904=CARTESIAN_POINT('Ctrl Pts',(-29.4869922550241,20.9143901035059,4.36837489374934));
#45905=CARTESIAN_POINT('Ctrl Pts',(-29.4866463833471,20.911597564513,4.36846182241841));
#45906=CARTESIAN_POINT('Ctrl Pts',(-29.4862844141115,20.9088103872103,4.36855274501376));
#45907=CARTESIAN_POINT('Ctrl Pts',(-29.4830395682688,20.8838249470327,4.36936781374468));
#45908=CARTESIAN_POINT('Ctrl Pts',(-29.4785025352126,20.8592571813233,4.37050416053162));
#45909=CARTESIAN_POINT('Ctrl Pts',(-29.4727464080655,20.8350828641766,4.37193103596413));
#45910=CARTESIAN_POINT('Ctrl Pts',(-29.4715260666181,20.8299577304844,4.37223354408915));
#45911=CARTESIAN_POINT('Ctrl Pts',(-29.470250901937,20.8248502902165,4.37254912127071));
#45912=CARTESIAN_POINT('Ctrl Pts',(-29.4689212596439,20.8197603930924,4.37287749430385));
#45913=CARTESIAN_POINT('Ctrl Pts',(-29.4632121945934,20.7979059786151,4.37428742464127));
#45914=CARTESIAN_POINT('Ctrl Pts',(-29.4565005209999,20.7763746296517,4.37593323382873));
#45915=CARTESIAN_POINT('Ctrl Pts',(-29.4488131569132,20.7551568610949,4.37779376198798));
#45916=CARTESIAN_POINT('Ctrl Pts',(-29.4462651977887,20.7481242805658,4.37841042976204));
#45917=CARTESIAN_POINT('Ctrl Pts',(-29.4436100535821,20.7411261537694,4.3790507017421));
#45918=CARTESIAN_POINT('Ctrl Pts',(-29.4408477969706,20.7341623429493,4.37971382159266));
#45919=CARTESIAN_POINT('Ctrl Pts',(-29.4352997116543,20.7201752946803,4.38104572011743));
#45920=CARTESIAN_POINT('Ctrl Pts',(-29.429320357937,20.7063265823598,4.38246980672111));
#45921=CARTESIAN_POINT('Ctrl Pts',(-29.422910812072,20.6926154355498,4.38398004522345));
#45922=CARTESIAN_POINT('Ctrl Pts',(-29.4205280402512,20.6875182672109,4.38454148184031));
#45923=CARTESIAN_POINT('Ctrl Pts',(-29.4180857816454,20.6824403569271,4.38511479576126));
#45924=CARTESIAN_POINT('Ctrl Pts',(-29.4155840016469,20.6773812076774,4.38569973530258));
#45925=CARTESIAN_POINT('Ctrl Pts',(-29.4147209454693,20.6756359183169,4.38590152590167));
#45926=CARTESIAN_POINT('Ctrl Pts',(-29.413850662798,20.6738927337401,4.38610472707077));
#45927=CARTESIAN_POINT('Ctrl Pts',(-29.4129733677328,20.6721520011351,4.38630927694907));
#45928=CARTESIAN_POINT('Ctrl Pts',(-29.4095530177616,20.6653653281535,4.38710676481617));
#45929=CARTESIAN_POINT('Ctrl Pts',(-29.4060207796651,20.65860648416,4.38792593542571));
#45930=CARTESIAN_POINT('Ctrl Pts',(-29.4024066083896,20.6519284466736,4.38875907393075));
#45931=CARTESIAN_POINT('Ctrl Pts',(-29.4001371996232,20.647735176444,4.38928221787797));
#45932=CARTESIAN_POINT('Ctrl Pts',(-29.3978321856955,20.6435672740895,4.38981165055932));
#45933=CARTESIAN_POINT('Ctrl Pts',(-29.3954948265902,20.6394299308394,4.39034642994758));
#45934=CARTESIAN_POINT('Ctrl Pts',(-29.3884220722315,20.6269104970744,4.39196465080228));
#45935=CARTESIAN_POINT('Ctrl Pts',(-29.3810364699,20.6146350685622,4.39363574521622));
#45936=CARTESIAN_POINT('Ctrl Pts',(-29.3733525338789,20.6025957810371,4.39535118824676));
#45937=CARTESIAN_POINT('Ctrl Pts',(-29.3673996050382,20.5932686573166,4.39668018295247));
#45938=CARTESIAN_POINT('Ctrl Pts',(-29.3612679862125,20.5840830647999,4.39803579888286));
#45939=CARTESIAN_POINT('Ctrl Pts',(-29.3549625690452,20.5750364056405,4.39941427356976));
#45940=CARTESIAN_POINT('Ctrl Pts',(-29.3447906773285,20.5604423454973,4.40163802734804));
#45941=CARTESIAN_POINT('Ctrl Pts',(-29.3341654427046,20.5462068647962,4.40392168341668));
#45942=CARTESIAN_POINT('Ctrl Pts',(-29.3231032810787,20.5323157427589,4.40625078658438));
#45943=CARTESIAN_POINT('Ctrl Pts',(-29.3155317896742,20.5228079707103,4.40784494016942));
#45944=CARTESIAN_POINT('Ctrl Pts',(-29.3077555903465,20.5134615445095,4.40946043956847));
#45945=CARTESIAN_POINT('Ctrl Pts',(-29.2997767506546,20.5042737135194,4.41109279276069));
#45946=CARTESIAN_POINT('Ctrl Pts',(-29.2885663431556,20.4913646523768,4.41338627717365));
#45947=CARTESIAN_POINT('Ctrl Pts',(-29.2769568348822,20.4787683533196,4.41571308352564));
#45948=CARTESIAN_POINT('Ctrl Pts',(-29.2649547579802,20.4664781747352,4.41806118409384));
#45949=CARTESIAN_POINT('Ctrl Pts',(-29.2559339982298,20.4572408777904,4.41982601623651));
#45950=CARTESIAN_POINT('Ctrl Pts',(-29.246690765677,20.4481765788377,4.42160290420698));
#45951=CARTESIAN_POINT('Ctrl Pts',(-29.2372257463337,20.4392844579056,4.42338663097564));
#45952=CARTESIAN_POINT('Ctrl Pts',(-29.2357824384442,20.4379285105134,4.42365862903761));
#45953=CARTESIAN_POINT('Ctrl Pts',(-29.2343339292738,20.4365765234704,4.42393079522064));
#45954=CARTESIAN_POINT('Ctrl Pts',(-29.2328802517791,20.4352285214994,4.42420310602461));
#45955=CARTESIAN_POINT('Ctrl Pts',(-29.228779764045,20.4314261199573,4.42497123177162));
#45956=CARTESIAN_POINT('Ctrl Pts',(-29.224649830871,20.4276662781706,4.42573831030471));
#45957=CARTESIAN_POINT('Ctrl Pts',(-29.2204919524299,20.4239491692082,4.4265037708607));
#45958=CARTESIAN_POINT('Ctrl Pts',(-29.2148600507244,20.4189142956299,4.42754059737495));
#45959=CARTESIAN_POINT('Ctrl Pts',(-29.2091763097764,20.4139573124958,4.42857455648857));
#45960=CARTESIAN_POINT('Ctrl Pts',(-29.2034417856259,20.4090764056792,4.42960472148362));
#45961=CARTESIAN_POINT('Ctrl Pts',(-29.2019739526209,20.4078270681698,4.42986840686372));
#45962=CARTESIAN_POINT('Ctrl Pts',(-29.2005027900015,20.4065827309674,4.43013184020828));
#45963=CARTESIAN_POINT('Ctrl Pts',(-29.1990283323788,20.4053433739984,4.43039500427588));
#45964=CARTESIAN_POINT('Ctrl Pts',(-29.1889819796394,20.3968989012052,4.43218809687529));
#45965=CARTESIAN_POINT('Ctrl Pts',(-29.1787816675667,20.3886839680143,4.43396892744536));
#45966=CARTESIAN_POINT('Ctrl Pts',(-29.1684325608492,20.3806911215074,4.4357329453857));
#45967=CARTESIAN_POINT('Ctrl Pts',(-29.154829586387,20.3701852401901,4.43805158907628));
#45968=CARTESIAN_POINT('Ctrl Pts',(-29.1409683057726,20.3600635818434,4.44034101948239));
#45969=CARTESIAN_POINT('Ctrl Pts',(-29.1268573005585,20.3503117232733,4.44259090921445));
#45970=CARTESIAN_POINT('Ctrl Pts',(-29.1163458403702,20.343047444679,4.4442668795644));
#45971=CARTESIAN_POINT('Ctrl Pts',(-29.1056957917177,20.3359883984724,4.44592095804887));
#45972=CARTESIAN_POINT('Ctrl Pts',(-29.0949083371168,20.3291312146284,4.44754895806742));
#45973=CARTESIAN_POINT('Ctrl Pts',(-29.0797948733191,20.3195241475662,4.44982982229845));
#45974=CARTESIAN_POINT('Ctrl Pts',(-29.0644122897058,20.3103127098318,4.45205964031271));
#45975=CARTESIAN_POINT('Ctrl Pts',(-29.0487649387269,20.3014886351646,4.45422727163098));
#45976=CARTESIAN_POINT('Ctrl Pts',(-29.0382506909112,20.2955592923691,4.45568381292568));
#45977=CARTESIAN_POINT('Ctrl Pts',(-29.0276166084402,20.2898051592413,4.45711226285544));
#45978=CARTESIAN_POINT('Ctrl Pts',(-29.016862654098,20.2842252122415,4.45850921188307));
#45979=CARTESIAN_POINT('Ctrl Pts',(-29.0137406770345,20.2826052996034,4.45891475971082));
#45980=CARTESIAN_POINT('Ctrl Pts',(-29.0106091998765,20.2810003697014,4.45931757794315));
#45981=CARTESIAN_POINT('Ctrl Pts',(-29.0074679133908,20.2794102180322,4.45971762954353));
#45982=CARTESIAN_POINT('Ctrl Pts',(-28.9971474318437,20.2741858836601,4.46103197167007));
#45983=CARTESIAN_POINT('Ctrl Pts',(-28.9867108167574,20.2691163199733,4.46231765695496));
#45984=CARTESIAN_POINT('Ctrl Pts',(-28.9761693954237,20.2642067288857,4.46357037351109));
#45985=CARTESIAN_POINT('Ctrl Pts',(-28.9723369419537,20.2624217912759,4.46402581284516));
#45986=CARTESIAN_POINT('Ctrl Pts',(-28.9684910649499,20.2606582186039,4.46447684003569));
#45987=CARTESIAN_POINT('Ctrl Pts',(-28.9646329082511,20.2589165824116,4.46492316881479));
#45988=CARTESIAN_POINT('Ctrl Pts',(-28.961569978256,20.257533924798,4.46527750222113));
#45989=CARTESIAN_POINT('Ctrl Pts',(-28.9585030873642,20.256166717489,4.46562844571048));
#45990=CARTESIAN_POINT('Ctrl Pts',(-28.9554323067952,20.2548148767914,4.46597595326881));
#45991=CARTESIAN_POINT('Ctrl Pts',(-28.9484934807138,20.2517602177952,4.46676119156735));
#45992=CARTESIAN_POINT('Ctrl Pts',(-28.9415314764778,20.2487826803726,4.46752922468682));
#45993=CARTESIAN_POINT('Ctrl Pts',(-28.9345467044577,20.2458807444744,4.46827970500645));
#45994=CARTESIAN_POINT('Ctrl Pts',(-28.9151642248849,20.2378279815343,4.47036225965865));
#45995=CARTESIAN_POINT('Ctrl Pts',(-28.8956059486648,20.2303585263828,4.4723092627131));
#45996=CARTESIAN_POINT('Ctrl Pts',(-28.8758774726147,20.2234510771608,4.47411036362058));
#45997=CARTESIAN_POINT('Ctrl Pts',(-28.8671681201616,20.2204017078292,4.47490547939976));
#45998=CARTESIAN_POINT('Ctrl Pts',(-28.8584255903597,20.2174618973078,4.47567217444019));
#45999=CARTESIAN_POINT('Ctrl Pts',(-28.8496499871138,20.2146308023702,4.47640958818901));
#46000=CARTESIAN_POINT('Ctrl Pts',(-28.8279227455547,20.2076213829761,4.478235327822));
#46001=CARTESIAN_POINT('Ctrl Pts',(-28.8059933800392,20.2012769372787,4.47988199179129));
#46002=CARTESIAN_POINT('Ctrl Pts',(-28.7838646067432,20.1955853468773,4.48133681237158));
#46003=CARTESIAN_POINT('Ctrl Pts',(-28.776809684112,20.1937707984886,4.48180062690387));
#46004=CARTESIAN_POINT('Ctrl Pts',(-28.769734499636,20.1920226012458,4.48224495215947));
#46005=CARTESIAN_POINT('Ctrl Pts',(-28.7626389680079,20.1903408137018,4.4826693708897));
#46006=CARTESIAN_POINT('Ctrl Pts',(-28.7381896799774,20.1845458274732,4.4841318033507));
#46007=CARTESIAN_POINT('Ctrl Pts',(-28.7134995184439,20.1795376786906,4.48535837645559));
#46008=CARTESIAN_POINT('Ctrl Pts',(-28.6885669332602,20.1753183905708,4.48633263463277));
#46009=CARTESIAN_POINT('Ctrl Pts',(-28.6835676332246,20.1744723697073,4.48652798577281));
#46010=CARTESIAN_POINT('Ctrl Pts',(-28.6785585585997,20.1736581381179,4.48671319150791));
#46011=CARTESIAN_POINT('Ctrl Pts',(-28.6735396612379,20.1728758059763,4.4868881172469));
#46012=CARTESIAN_POINT('Ctrl Pts',(-28.6704354517054,20.1723919301931,4.48699630956632));
#46013=CARTESIAN_POINT('Ctrl Pts',(-28.667328116131,20.1719203450063,4.48710055087429));
#46014=CARTESIAN_POINT('Ctrl Pts',(-28.6642171269454,20.1714609861963,4.48720083066601));
#46015=CARTESIAN_POINT('Ctrl Pts',(-28.6597994044565,20.1708086792854,4.4873432317689));
#46016=CARTESIAN_POINT('Ctrl Pts',(-28.6553706485648,20.1701805791297,4.48747773248562));
#46017=CARTESIAN_POINT('Ctrl Pts',(-28.6509366884823,20.1695774849372,4.48760410629557));
#46018=CARTESIAN_POINT('Ctrl Pts',(-28.647181504148,20.169066715823,4.48771113408621));
#46019=CARTESIAN_POINT('Ctrl Pts',(-28.6434213870889,20.1685737240394,4.48781236546092));
#46020=CARTESIAN_POINT('Ctrl Pts',(-28.6396608841676,20.1680991871688,4.48790761646221));
#46021=CARTESIAN_POINT('Ctrl Pts',(-28.6358543008539,20.1676188354257,4.48800403464875));
#46022=CARTESIAN_POINT('Ctrl Pts',(-28.6320482362219,20.1671574287393,4.48809432417053));
#46023=CARTESIAN_POINT('Ctrl Pts',(-28.6282428208247,20.1667148882399,4.48817848501042));
#46024=CARTESIAN_POINT('Ctrl Pts',(-28.6156464496165,20.1652500272923,4.48845706725958));
#46025=CARTESIAN_POINT('Ctrl Pts',(-28.603052964721,20.1639913732817,4.48866859713531));
#46026=CARTESIAN_POINT('Ctrl Pts',(-28.590462340133,20.1629357314628,4.48881310846486));
#46027=CARTESIAN_POINT('Ctrl Pts',(-28.5879303379186,20.1627234395781,4.48884217001013));
#46028=CARTESIAN_POINT('Ctrl Pts',(-28.5853984512941,20.1625193432353,4.4888685206279));
#46029=CARTESIAN_POINT('Ctrl Pts',(-28.5828666801655,20.1623234310325,4.488892161079));
#46030=CARTESIAN_POINT('Ctrl Pts',(-28.5526241869252,20.1599832220774,4.48917455081571));
#46031=CARTESIAN_POINT('Ctrl Pts',(-28.5223981639468,20.1588102781325,4.48907040538594));
#46032=CARTESIAN_POINT('Ctrl Pts',(-28.492188453501,20.1587864726715,4.48858057664305));
#46033=CARTESIAN_POINT('',(-17.2867694013439,20.1504205562397,4.30719763801101));
#46034=CARTESIAN_POINT('Ctrl Pts',(-28.492188453501,20.1587864726715,4.48858057664304));
#46035=CARTESIAN_POINT('Ctrl Pts',(-24.7570506191739,20.1558431582048,4.42801800113474));
#46036=CARTESIAN_POINT('Ctrl Pts',(-21.0219109331918,20.1530630626027,4.36756184755652));
#46037=CARTESIAN_POINT('Ctrl Pts',(-17.2867696586256,20.1504216822361,4.30719785610076));
#46038=CARTESIAN_POINT('',(-17.2461080117266,18.1757197899201,7.));
#46039=CARTESIAN_POINT('Ctrl Pts',(-17.2867699753103,20.1504209513526,4.30719809188305));
#46040=CARTESIAN_POINT('Ctrl Pts',(-17.3208257192627,20.071822958759,4.33255373642374));
#46041=CARTESIAN_POINT('Ctrl Pts',(-17.3535476746569,19.9938851605761,4.36146905604493));
#46042=CARTESIAN_POINT('Ctrl Pts',(-17.4004272525326,19.8779754334467,4.41045157774795));
#46043=CARTESIAN_POINT('Ctrl Pts',(-17.4233147516175,19.8202699530577,4.43634776622695));
#46044=CARTESIAN_POINT('Ctrl Pts',(-17.4453203036792,19.7629423461442,4.46442773366274));
#46045=CARTESIAN_POINT('Ctrl Pts',(-17.4597874908418,19.7248085032196,4.48364358525879));
#46046=CARTESIAN_POINT('Ctrl Pts',(-17.4669273739776,19.7057623714905,4.4935111894555));
#46047=CARTESIAN_POINT('Ctrl Pts',(-17.5019467009911,19.6111618337293,4.54389102196789));
#46048=CARTESIAN_POINT('Ctrl Pts',(-17.5278706528003,19.537295520511,4.58761089528929));
#46049=CARTESIAN_POINT('Ctrl Pts',(-17.5752369806953,19.3931873285045,4.68200405571982));
#46050=CARTESIAN_POINT('Ctrl Pts',(-17.5966805850057,19.3229450588183,4.73267627680039));
#46051=CARTESIAN_POINT('Ctrl Pts',(-17.6346156200307,19.1861771553916,4.84130234246955));
#46052=CARTESIAN_POINT('Ctrl Pts',(-17.6511094474768,19.1196505679119,4.8992538406938));
#46053=CARTESIAN_POINT('Ctrl Pts',(-17.6681966114296,19.0389449588237,4.97660963956145));
#46054=CARTESIAN_POINT('Ctrl Pts',(-17.6714220915483,19.0229959339583,4.99226140241664));
#46055=CARTESIAN_POINT('Ctrl Pts',(-17.6774786818592,18.9915153566521,5.02388879094697));
#46056=CARTESIAN_POINT('Ctrl Pts',(-17.6859756358375,18.9449029840238,5.07183293884616));
#46057=CARTESIAN_POINT('Ctrl Pts',(-17.6926947074833,18.9001035758318,5.12127726254189));
#46058=CARTESIAN_POINT('Ctrl Pts',(-17.703709514897,18.8129042024216,5.22215494584585));
#46059=CARTESIAN_POINT('Ctrl Pts',(-17.7078275163219,18.7579651770337,5.29205430864768));
#46060=CARTESIAN_POINT('Ctrl Pts',(-17.7091952476915,18.6545099125253,5.43719659709591));
#46061=CARTESIAN_POINT('Ctrl Pts',(-17.7064463567172,18.6059930873587,5.51243899701703));
#46062=CARTESIAN_POINT('Ctrl Pts',(-17.6991407639401,18.5551445709081,5.60020358607968));
#46063=CARTESIAN_POINT('Ctrl Pts',(-17.6982694593839,18.5495414765602,5.61000793743428));
#46064=CARTESIAN_POINT('Ctrl Pts',(-17.6964128600498,18.5384679700224,5.62965390264442));
#46065=CARTESIAN_POINT('Ctrl Pts',(-17.6934584932203,18.5220630392232,5.65916663843846));
#46066=CARTESIAN_POINT('Ctrl Pts',(-17.685384085205,18.4852072119293,5.72833147537855));
#46067=CARTESIAN_POINT('Ctrl Pts',(-17.676455706464,18.4560061760419,5.78811746154919));
#46068=CARTESIAN_POINT('Ctrl Pts',(-17.6559536600445,18.4006832919842,5.90832310966332));
#46069=CARTESIAN_POINT('Ctrl Pts',(-17.6387627137838,18.3679005667132,5.98930349659442));
#46070=CARTESIAN_POINT('Ctrl Pts',(-17.5973924447825,18.3101371654525,6.15280666091991));
#46071=CARTESIAN_POINT('Ctrl Pts',(-17.5732126955704,18.2851576196246,6.23532979134612));
#46072=CARTESIAN_POINT('Ctrl Pts',(-17.5385754612136,18.2586835344225,6.33938793190696));
#46073=CARTESIAN_POINT('Ctrl Pts',(-17.5314210668692,18.2536232472437,6.36026115366522));
#46074=CARTESIAN_POINT('Ctrl Pts',(-17.5167222918182,18.2440104157202,6.4019466819254));
#46075=CARTESIAN_POINT('Ctrl Pts',(-17.5091735113904,18.2394538697671,6.42277317881695));
#46076=CARTESIAN_POINT('Ctrl Pts',(-17.4975544336796,18.2329867994005,6.45398810171667));
#46077=CARTESIAN_POINT('Ctrl Pts',(-17.4936310903107,18.2308919767749,6.46439142406025));
#46078=CARTESIAN_POINT('Ctrl Pts',(-17.4857011391769,18.2268311508652,6.48515121686447));
#46079=CARTESIAN_POINT('Ctrl Pts',(-17.4736763159107,18.2209302438205,6.51623424645934));
#46080=CARTESIAN_POINT('Ctrl Pts',(-17.4281734265522,18.20135436499,6.62958911199627));
#46081=CARTESIAN_POINT('Ctrl Pts',(-17.3826445834544,18.1895780498687,6.73081934613577));
#46082=CARTESIAN_POINT('Ctrl Pts',(-17.3127519420792,18.1788281172695,6.87449306774556));
#46083=CARTESIAN_POINT('Ctrl Pts',(-17.2801713026602,18.1762507473026,6.93757304535173));
#46084=CARTESIAN_POINT('Ctrl Pts',(-17.2461080117266,18.1757197899201,7.));
#46085=CARTESIAN_POINT('',(-37.7046869279002,18.4953857332484,7.));
#46086=CARTESIAN_POINT('',(-6.,18.,7.));
#46087=CARTESIAN_POINT('',(-37.7046869279001,23.4998565514917,7.15430439779759));
#46088=CARTESIAN_POINT('Origin',(-37.7046869279001,21.,7.));
#46089=CARTESIAN_POINT('',(-31.4046869279001,23.6003888166982,7.11771364567903));
#46090=CARTESIAN_POINT('Ctrl Pts',(-37.7046869279001,23.4998565514917,7.15430439779759));
#46091=CARTESIAN_POINT('Ctrl Pts',(-36.1624028751846,23.524555494072,7.14531471788049));
#46092=CARTESIAN_POINT('Ctrl Pts',(-34.620117596862,23.5491869331956,7.13634960721236));
#46093=CARTESIAN_POINT('Ctrl Pts',(-33.0778312194337,23.5737573593539,7.12740670344752));
#46094=CARTESIAN_POINT('Ctrl Pts',(-32.6184875763975,23.5810752409274,7.12474321237687));
#46095=CARTESIAN_POINT('Ctrl Pts',(-32.0607728361779,23.5899537087511,7.12151171436315));
#46096=CARTESIAN_POINT('Ctrl Pts',(-31.503057956262,23.5988244202026,7.11828303943805));
#46097=CARTESIAN_POINT('Ctrl Pts',(-31.4046869279001,23.6003888166982,7.11771364567903));
#46098=CARTESIAN_POINT('',(-31.4046869279001,19.0836514699531,8.76167159589278));
#46099=CARTESIAN_POINT('Origin',(-31.4046869279001,21.,7.));
#46100=CARTESIAN_POINT('',(-37.7046869279002,19.1841837351597,8.72508084377422));
#46101=CARTESIAN_POINT('Ctrl Pts',(-31.4046869279001,19.0836514699531,8.76167159589278));
#46102=CARTESIAN_POINT('Ctrl Pts',(-31.503057956262,19.0852158664487,8.76110220213375));
#46103=CARTESIAN_POINT('Ctrl Pts',(-31.601428980305,19.0867805027715,8.76053272108482));
#46104=CARTESIAN_POINT('Ctrl Pts',(-31.6998,19.0883453804229,8.75996315219946));
#46105=CARTESIAN_POINT('Ctrl Pts',(-33.4052019268744,19.1154747663967,8.75008886323108));
#46106=CARTESIAN_POINT('Ctrl Pts',(-35.1106025511401,19.1426765782906,8.74018821338358));
#46107=CARTESIAN_POINT('Ctrl Pts',(-36.8160017078461,19.1699592983337,8.73025811537809));
#46108=CARTESIAN_POINT('Ctrl Pts',(-37.1122301591213,19.1746983166879,8.72853325375751));
#46109=CARTESIAN_POINT('Ctrl Pts',(-37.4084585661232,19.1794397794108,8.72680750245948));
#46110=CARTESIAN_POINT('Ctrl Pts',(-37.7046869279002,19.1841837351597,8.72508084377422));
#46111=CARTESIAN_POINT('Origin',(-37.7046869279001,21.,7.));
#46112=CARTESIAN_POINT('',(-13.9943709817605,20.1406244663727,9.74364801533398));
#46113=CARTESIAN_POINT('Ctrl Pts',(-17.2461080117266,18.1757197899201,7.));
#46114=CARTESIAN_POINT('Ctrl Pts',(-17.2374845700418,18.1755853730772,7.01580396926482));
#46115=CARTESIAN_POINT('Ctrl Pts',(-17.2287661057066,18.1755821101472,7.03156608650189));
#46116=CARTESIAN_POINT('Ctrl Pts',(-17.1763326909695,18.1763288548473,7.12510606643033));
#46117=CARTESIAN_POINT('Ctrl Pts',(-17.130413388618,18.1801068975316,7.20191231344627));
#46118=CARTESIAN_POINT('Ctrl Pts',(-17.0702785978487,18.1885224733183,7.29671107593985));
#46119=CARTESIAN_POINT('Ctrl Pts',(-17.0581024000519,18.1903928724755,7.31562872420576));
#46120=CARTESIAN_POINT('Ctrl Pts',(-17.0335791359912,18.1944811541833,7.35319187234959));
#46121=CARTESIAN_POINT('Ctrl Pts',(-16.9965140945174,18.2011373096274,7.40916741270535));
#46122=CARTESIAN_POINT('Ctrl Pts',(-16.9586325955796,18.2093134720725,7.46406874755071));
#46123=CARTESIAN_POINT('Ctrl Pts',(-16.881837046061,18.2275755679313,7.57251632857413));
#46124=CARTESIAN_POINT('Ctrl Pts',(-16.8292652167036,18.2422918218164,7.64301081819979));
#46125=CARTESIAN_POINT('Ctrl Pts',(-16.7216151897572,18.276322662728,7.78072073500009));
#46126=CARTESIAN_POINT('Ctrl Pts',(-16.6665364004662,18.2956386676755,7.84793529715628));
#46127=CARTESIAN_POINT('Ctrl Pts',(-16.5540588873242,18.3385266250333,7.97932936266556));
#46128=CARTESIAN_POINT('Ctrl Pts',(-16.496659786943,18.362099434901,8.04350832782672));
#46129=CARTESIAN_POINT('Ctrl Pts',(-16.4089303610114,18.4004724064477,8.13763727160809));
#46130=CARTESIAN_POINT('Ctrl Pts',(-16.3794151366119,18.4137664344875,8.16865656743358));
#46131=CARTESIAN_POINT('Ctrl Pts',(-16.33474556304,18.4344457762559,8.21466361265896));
#46132=CARTESIAN_POINT('Ctrl Pts',(-16.3197785925108,18.4414672349154,8.22992330103603));
#46133=CARTESIAN_POINT('Ctrl Pts',(-16.2897774767356,18.4557238173284,8.26020696428227));
#46134=CARTESIAN_POINT('Ctrl Pts',(-16.2146133970836,18.4918961529488,8.33532057783537));
#46135=CARTESIAN_POINT('Ctrl Pts',(-16.0779109948858,18.5616689299404,8.46530633625082));
#46136=CARTESIAN_POINT('Ctrl Pts',(-15.8929500681926,18.6639819795036,8.62836707437087));
#46137=CARTESIAN_POINT('Ctrl Pts',(-15.7055634000057,18.7751395847501,8.78182921325318));
#46138=CARTESIAN_POINT('Ctrl Pts',(-15.5159845124422,18.8948891297535,8.92617004052537));
#46139=CARTESIAN_POINT('Ctrl Pts',(-15.3882781701595,18.9803912140309,9.01653479984028));
#46140=CARTESIAN_POINT('Ctrl Pts',(-15.2920527636081,19.0466610460811,9.08215821710572));
#46141=CARTESIAN_POINT('Ctrl Pts',(-15.2438286045929,19.0803323938859,9.11443187566169));
#46142=CARTESIAN_POINT('Ctrl Pts',(-15.1954462683221,19.1148173577572,9.14590290763911));
#46143=CARTESIAN_POINT('Ctrl Pts',(-15.1631572166934,19.1379895449502,9.16670540807019));
#46144=CARTESIAN_POINT('Ctrl Pts',(-15.1469886722597,19.1496718364991,9.17702188510648));
#46145=CARTESIAN_POINT('Ctrl Pts',(-15.0662279656308,19.2084219980857,9.22805559353009));
#46146=CARTESIAN_POINT('Ctrl Pts',(-14.9373315528598,19.3047303334721,9.30633637519877));
#46147=CARTESIAN_POINT('Ctrl Pts',(-14.745157724316,19.456198658285,9.4139193981442));
#46148=CARTESIAN_POINT('Ctrl Pts',(-14.554399737518,19.6148926439594,9.51177846055287));
#46149=CARTESIAN_POINT('Ctrl Pts',(-14.3653491692332,19.7811828464356,9.59985942251706));
#46150=CARTESIAN_POINT('Ctrl Pts',(-14.2406886289955,19.8974714244525,9.65190302383858));
#46151=CARTESIAN_POINT('Ctrl Pts',(-14.1168602614401,20.0167316186446,9.70045488642478));
#46152=CARTESIAN_POINT('Ctrl Pts',(-14.0553617214042,20.0778465000411,9.72298583483569));
#46153=CARTESIAN_POINT('Ctrl Pts',(-13.9943709817605,20.1406244663727,9.74364801533398));
#46154=CARTESIAN_POINT('',(-13.7129564349448,20.6615335048058,9.85952349485951));
#46155=CARTESIAN_POINT('Ctrl Pts',(-13.9943709817604,20.1406244663728,9.74364801533398));
#46156=CARTESIAN_POINT('Ctrl Pts',(-13.9678155062267,20.1679580970929,9.7526443631144));
#46157=CARTESIAN_POINT('Ctrl Pts',(-13.9423330747277,20.1962188425863,9.76146424305687));
#46158=CARTESIAN_POINT('Ctrl Pts',(-13.9181306824652,20.2255898589142,9.77006745101129));
#46159=CARTESIAN_POINT('Ctrl Pts',(-13.9106257065011,20.2346975855055,9.77273523972456));
#46160=CARTESIAN_POINT('Ctrl Pts',(-13.9032441390017,20.2439122365762,9.77538212412262));
#46161=CARTESIAN_POINT('Ctrl Pts',(-13.8959930675324,20.2532397371734,9.77800670735638));
#46162=CARTESIAN_POINT('Ctrl Pts',(-13.894459989469,20.2552118300721,9.77856161720638));
#46163=CARTESIAN_POINT('Ctrl Pts',(-13.8929328029768,20.2571889081341,9.77911551270585));
#46164=CARTESIAN_POINT('Ctrl Pts',(-13.8914115564317,20.2591710522661,9.77966838704705));
#46165=CARTESIAN_POINT('Ctrl Pts',(-13.8777336839485,20.276992959417,9.78463940555978));
#46166=CARTESIAN_POINT('Ctrl Pts',(-13.8645321513175,20.2952317214795,9.78952955576498));
#46167=CARTESIAN_POINT('Ctrl Pts',(-13.8518728105507,20.3139384256743,9.79432607313674));
#46168=CARTESIAN_POINT('Ctrl Pts',(-13.8500982491222,20.3165606945848,9.79499843948473));
#46169=CARTESIAN_POINT('Ctrl Pts',(-13.848334638917,20.3191917804785,9.79566886174757));
#46170=CARTESIAN_POINT('Ctrl Pts',(-13.846582196565,20.321831792061,9.79633729347187));
#46171=CARTESIAN_POINT('Ctrl Pts',(-13.8413886567631,20.3296557328692,9.79831825835845));
#46172=CARTESIAN_POINT('Ctrl Pts',(-13.8363073992497,20.3375366388824,9.80027632033235));
#46173=CARTESIAN_POINT('Ctrl Pts',(-13.8313424796597,20.3454770830741,9.80221067100469));
#46174=CARTESIAN_POINT('Ctrl Pts',(-13.8229125974778,20.3589590756412,9.8054949836649));
#46175=CARTESIAN_POINT('Ctrl Pts',(-13.8148176348778,20.372613333958,9.80871112397037));
#46176=CARTESIAN_POINT('Ctrl Pts',(-13.8070804182788,20.3864513682538,9.81185433149902));
#46177=CARTESIAN_POINT('Ctrl Pts',(-13.7965338154804,20.4053139979037,9.81613883884006));
#46178=CARTESIAN_POINT('Ctrl Pts',(-13.7866491922786,20.4245175913989,9.82028832080854));
#46179=CARTESIAN_POINT('Ctrl Pts',(-13.7774996931455,20.4440988084439,9.82428825257612));
#46180=CARTESIAN_POINT('Ctrl Pts',(-13.7669251796949,20.466729756872,9.82891116489764));
#46181=CARTESIAN_POINT('Ctrl Pts',(-13.7573319687151,20.4898647835373,9.83333444164274));
#46182=CARTESIAN_POINT('Ctrl Pts',(-13.7488489882647,20.5135706416344,9.83753261467546));
#46183=CARTESIAN_POINT('Ctrl Pts',(-13.7480286665604,20.5158630470016,9.83793858666573));
#46184=CARTESIAN_POINT('Ctrl Pts',(-13.7472187561872,20.5181608018945,9.8383424508099));
#46185=CARTESIAN_POINT('Ctrl Pts',(-13.7464193789805,20.520463975649,9.83874418260543));
#46186=CARTESIAN_POINT('Ctrl Pts',(-13.7430855599168,20.530069409111,9.84041961331223));
#46187=CARTESIAN_POINT('Ctrl Pts',(-13.7399346038681,20.5397690428386,9.84205802015337));
#46188=CARTESIAN_POINT('Ctrl Pts',(-13.7369778918466,20.5495685335625,9.84365718794162));
#46189=CARTESIAN_POINT('Ctrl Pts',(-13.7346205393843,20.5573815547226,9.84493218601245));
#46190=CARTESIAN_POINT('Ctrl Pts',(-13.7323843611739,20.5652681120244,9.84618372560941));
#46191=CARTESIAN_POINT('Ctrl Pts',(-13.7302881581844,20.5731813035807,9.8474030924272));
#46192=CARTESIAN_POINT('Ctrl Pts',(-13.7291247796699,20.5775730714983,9.84807983278311));
#46193=CARTESIAN_POINT('Ctrl Pts',(-13.7280038555256,20.58197485668,9.8487469873088));
#46194=CARTESIAN_POINT('Ctrl Pts',(-13.726925950927,20.5863867852498,9.84940444264791));
#46195=CARTESIAN_POINT('Ctrl Pts',(-13.7208857536075,20.6111096773842,9.85308859056077));
#46196=CARTESIAN_POINT('Ctrl Pts',(-13.7161966218325,20.6361508131826,9.85646810013119));
#46197=CARTESIAN_POINT('Ctrl Pts',(-13.7129564349448,20.6615335048058,9.8595234948595));
#46198=CARTESIAN_POINT('Ctrl Pts',(-13.7129564349448,20.6615335048058,9.85952349485952));
#46199=CARTESIAN_POINT('Ctrl Pts',(-13.7036527253464,20.7344160883897,9.86829660154869));
#46200=CARTESIAN_POINT('Ctrl Pts',(-13.6973734530137,20.8072675266628,9.87419602162833));
#46201=CARTESIAN_POINT('Ctrl Pts',(-13.6940900143325,20.8800864282419,9.87728216942434));
#46202=CARTESIAN_POINT('Ctrl Pts',(-13.6930332737108,20.9035224350612,9.87827541402463));
#46203=CARTESIAN_POINT('Ctrl Pts',(-13.6922868437377,20.9269551735342,9.87897686532106));
#46204=CARTESIAN_POINT('Ctrl Pts',(-13.691849770872,20.9503848193212,9.87938741553639));
#46205=CARTESIAN_POINT('Ctrl Pts',(-13.6904743566214,21.0241150168119,9.88067936628678));
#46206=CARTESIAN_POINT('Ctrl Pts',(-13.6921624494699,21.0978128650641,9.87909442673253));
#46207=CARTESIAN_POINT('Ctrl Pts',(-13.6969164901419,21.1714789657059,9.87462563650867));
#46208=CARTESIAN_POINT('Ctrl Pts',(-13.6983671737571,21.1939579919851,9.87326199635393));
#46209=CARTESIAN_POINT('Ctrl Pts',(-13.7001033430898,21.2164340423875,9.87162946024555));
#46210=CARTESIAN_POINT('Ctrl Pts',(-13.7021250674901,21.2389070262678,9.86972686788085));
#46211=CARTESIAN_POINT('Ctrl Pts',(-13.7042868487285,21.2629368470063,9.86769247166067));
#46212=CARTESIAN_POINT('Ctrl Pts',(-13.7067754665188,21.2869632334582,9.865349303113));
#46213=CARTESIAN_POINT('Ctrl Pts',(-13.7095917140698,21.3109861711179,9.86269533148285));
#46214=CARTESIAN_POINT('Ctrl Pts',(-13.7109998378453,21.3229976399478,9.86136834566778));
#46215=CARTESIAN_POINT('Ctrl Pts',(-13.712489868911,21.3350082454893,9.85996364954342));
#46216=CARTESIAN_POINT('Ctrl Pts',(-13.7140619415434,21.3470179869437,9.85848092966431));
#46217=CARTESIAN_POINT('Ctrl Pts',(-13.7156340141758,21.3590277283981,9.8569982097852));
#46218=CARTESIAN_POINT('Ctrl Pts',(-13.717289175782,21.3710435001363,9.85543647401904));
#46219=CARTESIAN_POINT('Ctrl Pts',(-13.7190227227906,21.3830328711285,9.85379994855188));
#46220=CARTESIAN_POINT('Ctrl Pts',(-13.7207562697992,21.3950222421207,9.85216342308471));
#46221=CARTESIAN_POINT('Ctrl Pts',(-13.7225685411701,21.406988586054,9.85045178901428));
#46222=CARTESIAN_POINT('Ctrl Pts',(-13.7244588222449,21.4189320780816,9.84866549501998));
#46223=CARTESIAN_POINT('Ctrl Pts',(-13.7263491033196,21.4308755701092,9.84687920102567));
#46224=CARTESIAN_POINT('Ctrl Pts',(-13.7283185206183,21.4428026752592,9.84501718116659));
#46225=CARTESIAN_POINT('Ctrl Pts',(-13.7303624422929,21.4546908792916,9.84308357311477));
#46226=CARTESIAN_POINT('Ctrl Pts',(-13.734450285642,21.4784672873565,9.83921635701112));
#46227=CARTESIAN_POINT('Ctrl Pts',(-13.7388319210099,21.5020663604287,9.83506680074837));
#46228=CARTESIAN_POINT('Ctrl Pts',(-13.7434962067534,21.5254941628828,9.83064342694144));
#46229=CARTESIAN_POINT('Ctrl Pts',(-13.7561476228294,21.5890397715551,9.81864546078576));
#46230=CARTESIAN_POINT('Ctrl Pts',(-13.7708718347572,21.6513304844594,9.80463565324319));
#46231=CARTESIAN_POINT('Ctrl Pts',(-13.7874862060043,21.7124593155382,9.78875075720091));
#46232=CARTESIAN_POINT('Ctrl Pts',(-13.7953731789483,21.7414776533159,9.7812100718846));
#46233=CARTESIAN_POINT('Ctrl Pts',(-13.8036860947034,21.7702343158064,9.77324607590147));
#46234=CARTESIAN_POINT('Ctrl Pts',(-13.8124054158604,21.7987397797719,9.764869356201));
#46235=CARTESIAN_POINT('Ctrl Pts',(-13.8322758179319,21.8637006890019,9.74577970627396));
#46236=CARTESIAN_POINT('Ctrl Pts',(-13.8542587234846,21.9273544229971,9.72455068576793));
#46237=CARTESIAN_POINT('Ctrl Pts',(-13.878183283974,21.989781098824,9.70127867312322));
#46238=CARTESIAN_POINT('Ctrl Pts',(-13.8868723841143,22.0124536840915,9.69282657017131));
#46239=CARTESIAN_POINT('Ctrl Pts',(-13.8958175984909,22.0349644128231,9.68410448289681));
#46240=CARTESIAN_POINT('Ctrl Pts',(-13.9050107423846,22.0573170274346,9.67511534283697));
#46241=CARTESIAN_POINT('Ctrl Pts',(-13.9136371268844,22.0782915983152,9.66668038528867));
#46242=CARTESIAN_POINT('Ctrl Pts',(-13.9224824295412,22.099126578146,9.65801041030057));
#46243=CARTESIAN_POINT('Ctrl Pts',(-13.931541052428,22.1198243299877,9.64910743888102));
#46244=CARTESIAN_POINT('Ctrl Pts',(-13.9405996753149,22.1405220818294,9.64020446746147));
#46245=CARTESIAN_POINT('Ctrl Pts',(-13.9498749785272,22.1610898312997,9.63106517933433));
#46246=CARTESIAN_POINT('Ctrl Pts',(-13.9593514650354,22.181507469896,9.6217012642152));
#46247=CARTESIAN_POINT('Ctrl Pts',(-13.9783044380518,22.2223427470887,9.60297343397693));
#46248=CARTESIAN_POINT('Ctrl Pts',(-13.9979239435683,22.2622844146239,9.58348365750646));
#46249=CARTESIAN_POINT('Ctrl Pts',(-14.0181458571129,22.301397033398,9.56327145460671));
#46250=CARTESIAN_POINT('Ctrl Pts',(-14.047012829478,22.3572306656996,9.53441834427864));
#46251=CARTESIAN_POINT('Ctrl Pts',(-14.077103469815,22.4113789550291,9.50409285299139));
#46252=CARTESIAN_POINT('Ctrl Pts',(-14.1082729868791,22.4639803192505,9.4723797919722));
#46253=CARTESIAN_POINT('Ctrl Pts',(-14.1207732576489,22.4850756507655,9.4596615375038));
#46254=CARTESIAN_POINT('Ctrl Pts',(-14.1334470488101,22.5059220937757,9.44671952479236));
#46255=CARTESIAN_POINT('Ctrl Pts',(-14.1462850211486,22.5265281049559,9.4335569387938));
#46256=CARTESIAN_POINT('Ctrl Pts',(-14.1808678364504,22.582036393957,9.39809968211153));
#46257=CARTESIAN_POINT('Ctrl Pts',(-14.2166436653731,22.6357989151547,9.3610466312961));
#46258=CARTESIAN_POINT('Ctrl Pts',(-14.2534796534065,22.6879277922558,9.3224484691866));
#46259=CARTESIAN_POINT('Ctrl Pts',(-14.26441529704,22.7034034955946,9.31098968205277));
#46260=CARTESIAN_POINT('Ctrl Pts',(-14.2754443768594,22.7187351039292,9.29939438604579));
#46261=CARTESIAN_POINT('Ctrl Pts',(-14.2865634167636,22.7339252276024,9.28766309180211));
#46262=CARTESIAN_POINT('Ctrl Pts',(-14.2987066132822,22.75051448877,9.27485124719641));
#46263=CARTESIAN_POINT('Ctrl Pts',(-14.3109575323814,22.7669347099736,9.26187741306074));
#46264=CARTESIAN_POINT('Ctrl Pts',(-14.323312446271,22.7831885697824,9.24874219114853));
#46265=CARTESIAN_POINT('Ctrl Pts',(-14.3356673601605,22.7994424295911,9.23560696923631));
#46266=CARTESIAN_POINT('Ctrl Pts',(-14.3481294639689,22.8155339721094,9.22230693586296));
#46267=CARTESIAN_POINT('Ctrl Pts',(-14.3606854713469,22.8314530437744,9.20885290917389));
#46268=CARTESIAN_POINT('Ctrl Pts',(-14.385797486103,22.8632911871044,9.18194485579574));
#46269=CARTESIAN_POINT('Ctrl Pts',(-14.4111704750995,22.8942958355665,9.15454372686061));
#46270=CARTESIAN_POINT('Ctrl Pts',(-14.4367746827933,22.9245107320554,9.12666136044781));
#46271=CARTESIAN_POINT('Ctrl Pts',(-14.4773471154067,22.9723892630523,9.08247895707439));
#46272=CARTESIAN_POINT('Ctrl Pts',(-14.5184980614865,23.0182881012217,9.03708818117602));
#46273=CARTESIAN_POINT('Ctrl Pts',(-14.5601330700439,23.0623326230404,8.99051784601957));
#46274=CARTESIAN_POINT('Ctrl Pts',(-14.5710476049953,23.0738788071163,8.9783095249846));
#46275=CARTESIAN_POINT('Ctrl Pts',(-14.5819954054864,23.0852974233284,8.96601989905037));
#46276=CARTESIAN_POINT('Ctrl Pts',(-14.5929747699614,23.0965904242636,8.95364898597441));
#46277=CARTESIAN_POINT('Ctrl Pts',(-14.6373231856493,23.1422056965305,8.90367975535227));
#46278=CARTESIAN_POINT('Ctrl Pts',(-14.6821873492953,23.185772764633,8.85238878137541));
#46279=CARTESIAN_POINT('Ctrl Pts',(-14.7274828084958,23.2273755535218,8.79977569903656));
#46280=CARTESIAN_POINT('Ctrl Pts',(-14.7361778644479,23.2353617530998,8.78967592959335));
#46281=CARTESIAN_POINT('Ctrl Pts',(-14.7448888135656,23.2432754682488,8.77952732413173));
#46282=CARTESIAN_POINT('Ctrl Pts',(-14.7536150584491,23.2511171438068,8.76932972001199));
#46283=CARTESIAN_POINT('Ctrl Pts',(-14.8003253341024,23.2930924529792,8.71474347979135));
#46284=CARTESIAN_POINT('Ctrl Pts',(-14.8474743525417,23.3330060160619,8.65875697852264));
#46285=CARTESIAN_POINT('Ctrl Pts',(-14.8949923923289,23.3708917389166,8.60133801834855));
#46286=CARTESIAN_POINT('Ctrl Pts',(-14.9025955410729,23.376953663765,8.59215066767327));
#46287=CARTESIAN_POINT('Ctrl Pts',(-14.9102081374154,23.3829635840753,8.58292658058977));
#46288=CARTESIAN_POINT('Ctrl Pts',(-14.9178298957478,23.38892153554,8.57366555667347));
#46289=CARTESIAN_POINT('Ctrl Pts',(-14.9247369087521,23.394320768427,8.56527300342887));
#46290=CARTESIAN_POINT('Ctrl Pts',(-14.9316514833144,23.3996773155833,8.55685012467997));
#46291=CARTESIAN_POINT('Ctrl Pts',(-14.9385734378949,23.4049911793944,8.54839676378748));
#46292=CARTESIAN_POINT('Ctrl Pts',(-14.9454953924754,23.4103050432056,8.539943402895));
#46293=CARTESIAN_POINT('Ctrl Pts',(-14.9524262363533,23.4155773244076,8.53145769055019));
#46294=CARTESIAN_POINT('Ctrl Pts',(-14.959353285948,23.4207986878509,8.5229548624532));
#46295=CARTESIAN_POINT('Ctrl Pts',(-14.9732073851374,23.4312414147376,8.50594920625923));
#46296=CARTESIAN_POINT('Ctrl Pts',(-14.9870564533274,23.4414883605791,8.48886276682353));
#46297=CARTESIAN_POINT('Ctrl Pts',(-15.0008990793685,23.4515418985906,8.47169540755511));
#46298=CARTESIAN_POINT('Ctrl Pts',(-15.0285843314506,23.4716489746137,8.43736068901826));
#46299=CARTESIAN_POINT('Ctrl Pts',(-15.056243820486,23.4909827221071,8.40270247677271));
#46300=CARTESIAN_POINT('Ctrl Pts',(-15.0838673340348,23.5095574077922,8.36771880146978));
#46301=CARTESIAN_POINT('Ctrl Pts',(-15.1327946316088,23.5424572477151,8.30575504408032));
#46302=CARTESIAN_POINT('Ctrl Pts',(-15.1816083488692,23.5729787208378,8.24277073945841));
#46303=CARTESIAN_POINT('Ctrl Pts',(-15.2302598345825,23.6011583270334,8.17874455125467));
#46304=CARTESIAN_POINT('Ctrl Pts',(-15.236543938669,23.6047981661021,8.17047456268122));
#46305=CARTESIAN_POINT('Ctrl Pts',(-15.2428253361195,23.6083988711168,8.16218715798696));
#46306=CARTESIAN_POINT('Ctrl Pts',(-15.2491039220922,23.6119604639728,8.15388226311987));
#46307=CARTESIAN_POINT('Ctrl Pts',(-15.2980136097019,23.6397049903268,8.08918778965834));
#46308=CARTESIAN_POINT('Ctrl Pts',(-15.3467526858593,23.6650797342656,8.02343413429301));
#46309=CARTESIAN_POINT('Ctrl Pts',(-15.3952795899614,23.688065012956,7.95658226498493));
#46310=CARTESIAN_POINT('Ctrl Pts',(-15.4012104696617,23.6908742365261,7.94841173768804));
#46311=CARTESIAN_POINT('Ctrl Pts',(-15.4071381800772,23.6936477058343,7.94022479030037));
#46312=CARTESIAN_POINT('Ctrl Pts',(-15.4130626453345,23.6963853325483,7.93202133999328));
#46313=CARTESIAN_POINT('Ctrl Pts',(-15.4603402908521,23.7182317844597,7.86655723499836));
#46314=CARTESIAN_POINT('Ctrl Pts',(-15.5074112844545,23.7377996181745,7.80004345203389));
#46315=CARTESIAN_POINT('Ctrl Pts',(-15.5542428903708,23.7550185268095,7.73242656333141));
#46316=CARTESIAN_POINT('Ctrl Pts',(-15.5612969456177,23.7576121413231,7.7222417050674));
#46317=CARTESIAN_POINT('Ctrl Pts',(-15.5683455695944,23.7601523666281,7.71203181680802));
#46318=CARTESIAN_POINT('Ctrl Pts',(-15.5753886504285,23.762638858942,7.70179671648233));
#46319=CARTESIAN_POINT('Ctrl Pts',(-15.602289564448,23.7721359693005,7.66270394439485));
#46320=CARTESIAN_POINT('Ctrl Pts',(-15.6291097206323,23.780849799148,7.6232429531147));
#46321=CARTESIAN_POINT('Ctrl Pts',(-15.6558435641724,23.7887579153097,7.58340079166616));
#46322=CARTESIAN_POINT('Ctrl Pts',(-15.6625270250574,23.7907349443502,7.57344025130403));
#46323=CARTESIAN_POINT('Ctrl Pts',(-15.6692027203841,23.7926608334869,7.56345938084566));
#46324=CARTESIAN_POINT('Ctrl Pts',(-15.6758600778727,23.794532483472,7.55347386171613));
#46325=CARTESIAN_POINT('Ctrl Pts',(-15.6825174353613,23.7964041334571,7.54348834258661));
#46326=CARTESIAN_POINT('Ctrl Pts',(-15.689159444701,23.798222436163,7.53349372486578));
#46327=CARTESIAN_POINT('Ctrl Pts',(-15.6957860766278,23.7999874133985,7.52348999736768));
#46328=CARTESIAN_POINT('Ctrl Pts',(-15.7090393404816,23.8035173678694,7.50348254237147));
#46329=CARTESIAN_POINT('Ctrl Pts',(-15.7222310949942,23.8068340407154,7.48343864760626));
#46330=CARTESIAN_POINT('Ctrl Pts',(-15.7353611064557,23.8099373932428,7.4633580913403));
#46331=CARTESIAN_POINT('Ctrl Pts',(-15.7827318779681,23.8211337432174,7.39091097691843));
#46332=CARTESIAN_POINT('Ctrl Pts',(-15.829299054463,23.8295572844193,7.31798752817788));
#46333=CARTESIAN_POINT('Ctrl Pts',(-15.8750507541838,23.8351723271489,7.24458053382367));
#46334=CARTESIAN_POINT('Ctrl Pts',(-15.8800240329711,23.8357826907652,7.23660108278487));
#46335=CARTESIAN_POINT('Ctrl Pts',(-15.8849876760702,23.8363598183367,7.22861591935028));
#46336=CARTESIAN_POINT('Ctrl Pts',(-15.8899416682199,23.8369036267558,7.22062503629825));
#46337=CARTESIAN_POINT('Ctrl Pts',(-15.935236133316,23.8418756797414,7.14756420726362));
#46338=CARTESIAN_POINT('Ctrl Pts',(-15.979723815376,23.8440668153845,7.07402507537809));
#46339=CARTESIAN_POINT('Ctrl Pts',(-16.0233918417347,23.8433845024729,7.00000000000883));
#46340=CARTESIAN_POINT('Origin',(-37.7,21.,7.));
#46341=CARTESIAN_POINT('',(-38.,23.1883393165246,7.26768739878651));
#46342=CARTESIAN_POINT('',(-38.,19.4957009701268,8.6116978427853));
#46343=CARTESIAN_POINT('Origin',(-38.,21.,7.));
#46344=CARTESIAN_POINT('Ctrl Pts',(-37.7046869279001,23.4998565514917,7.15430439779761));
#46345=CARTESIAN_POINT('Ctrl Pts',(-37.7395316670408,23.4992985296346,7.15450750114366));
#46346=CARTESIAN_POINT('Ctrl Pts',(-37.7794800415659,23.4909398979206,7.15754979428675));
#46347=CARTESIAN_POINT('Ctrl Pts',(-37.8454177694196,23.4639858105548,7.16736027977971));
#46348=CARTESIAN_POINT('Ctrl Pts',(-37.8821059412057,23.4393962497117,7.17631014800026));
#46349=CARTESIAN_POINT('Ctrl Pts',(-37.9354044401321,23.3865174575227,7.19555645438101));
#46350=CARTESIAN_POINT('Ctrl Pts',(-37.9607107815143,23.3482518128805,7.20948401002579));
#46351=CARTESIAN_POINT('Ctrl Pts',(-37.9908311196217,23.2758954359896,7.23581957747343));
#46352=CARTESIAN_POINT('Ctrl Pts',(-38.,23.2284905615032,7.25307354074558));
#46353=CARTESIAN_POINT('Ctrl Pts',(-38.,23.1883393165246,7.26768739878653));
#46354=CARTESIAN_POINT('Ctrl Pts',(-38.,19.4957009701268,8.61169784278532));
#46355=CARTESIAN_POINT('Ctrl Pts',(-38.,19.4555497251481,8.62631170082627));
#46356=CARTESIAN_POINT('Ctrl Pts',(-37.9908311196217,19.4081448506618,8.64356566409842));
#46357=CARTESIAN_POINT('Ctrl Pts',(-37.9607107815143,19.3357884737709,8.66990123154606));
#46358=CARTESIAN_POINT('Ctrl Pts',(-37.9354044401321,19.2975228291287,8.68382878719084));
#46359=CARTESIAN_POINT('Ctrl Pts',(-37.8821059412057,19.2446440369396,8.70307509357159));
#46360=CARTESIAN_POINT('Ctrl Pts',(-37.8454177694196,19.2200544760966,8.71202496179214));
#46361=CARTESIAN_POINT('Ctrl Pts',(-37.7794800415659,19.1931003887308,8.7218354472851));
#46362=CARTESIAN_POINT('Ctrl Pts',(-37.7395316670409,19.1847417570168,8.72487774042819));
#46363=CARTESIAN_POINT('Ctrl Pts',(-37.7046869279002,19.1841837351597,8.72508084377424));
#46364=CARTESIAN_POINT('Origin',(6.61287431064084E-15,12.,8.67361737988404E-16));
#46365=CARTESIAN_POINT('',(4.24820533297024E-15,12.5093665794476,19.3089875327072));
#46366=CARTESIAN_POINT('Origin',(3.30643715532042E-15,12.5093665794476,
4.33680868994202E-16));
#46367=CARTESIAN_POINT('',(4.568814811381E-15,19.4906334205533,16.6910124672925));
#46368=CARTESIAN_POINT('',(4.2248130523035E-15,12.,19.5));
#46369=CARTESIAN_POINT('',(-13.2658111744658,19.4906334205523,10.1295681579593));
#46370=CARTESIAN_POINT('Origin',(6.61325378140121E-15,19.4906334205523,
8.67361737988404E-16));
#46371=CARTESIAN_POINT('',(-16.3856910571095,19.4906334689658,3.17789711507297));
#46372=CARTESIAN_POINT('Ctrl Pts',(-13.2658111744658,19.4906334205523,10.1295681579593));
#46373=CARTESIAN_POINT('Ctrl Pts',(-13.3267563717861,19.4032674929026,10.1037375593391));
#46374=CARTESIAN_POINT('Ctrl Pts',(-13.3884259101566,19.3179204250404,10.075220655976));
#46375=CARTESIAN_POINT('Ctrl Pts',(-13.4507036432112,19.2344246756853,10.0441518788645));
#46376=CARTESIAN_POINT('Ctrl Pts',(-13.4570523134828,19.2259130142016,10.0409846887317));
#46377=CARTESIAN_POINT('Ctrl Pts',(-13.4634073117058,19.2174206253153,10.0377909469459));
#46378=CARTESIAN_POINT('Ctrl Pts',(-13.469768514267,19.2089473264459,10.0345707988203));
#46379=CARTESIAN_POINT('Ctrl Pts',(-13.5258079811479,19.1343011967558,10.0062026746325));
#46380=CARTESIAN_POINT('Ctrl Pts',(-13.5823298738816,19.0611374216604,9.97578381795668));
#46381=CARTESIAN_POINT('Ctrl Pts',(-13.6392670213906,18.9893727845524,9.94336645117775));
#46382=CARTESIAN_POINT('Ctrl Pts',(-13.6519731092965,18.9733577956124,9.93613219498486));
#46383=CARTESIAN_POINT('Ctrl Pts',(-13.6646999196863,18.9574126170077,9.9287982659174));
#46384=CARTESIAN_POINT('Ctrl Pts',(-13.6774467134566,18.9415362896475,9.92136524837809));
#46385=CARTESIAN_POINT('Ctrl Pts',(-13.7283032803252,18.8781936547406,9.89170933957969));
#46386=CARTESIAN_POINT('Ctrl Pts',(-13.7794782156711,18.8159476034485,9.86047564177073));
#46387=CARTESIAN_POINT('Ctrl Pts',(-13.8309330026652,18.7547608624783,9.82767434435942));
#46388=CARTESIAN_POINT('Ctrl Pts',(-13.8499593369977,18.732135962864,9.81554547380052));
#46389=CARTESIAN_POINT('Ctrl Pts',(-13.8690240359903,18.7096562047432,9.80320192369851));
#46390=CARTESIAN_POINT('Ctrl Pts',(-13.8881251733158,18.6873196376304,9.79064419604015));
#46391=CARTESIAN_POINT('Ctrl Pts',(-13.9336285571146,18.6341087021369,9.76072874694729));
#46392=CARTESIAN_POINT('Ctrl Pts',(-13.9793388662965,18.5817106162214,9.72959770180917));
#46393=CARTESIAN_POINT('Ctrl Pts',(-14.0252343603869,18.5301127159014,9.69724126768515));
#46394=CARTESIAN_POINT('Ctrl Pts',(-14.0505071373545,18.5016998563687,9.67942389891539));
#46395=CARTESIAN_POINT('Ctrl Pts',(-14.0758362191046,18.4735300880598,9.66123443518788));
#46396=CARTESIAN_POINT('Ctrl Pts',(-14.1012180543646,18.4456012371598,9.64267109998932));
#46397=CARTESIAN_POINT('Ctrl Pts',(-14.1412786350688,18.4015206585098,9.61337227347639));
#46398=CARTESIAN_POINT('Ctrl Pts',(-14.1814707003173,18.3580402718792,9.58314214870423));
#46399=CARTESIAN_POINT('Ctrl Pts',(-14.2217824291453,18.3151599459258,9.55196286685991));
#46400=CARTESIAN_POINT('Ctrl Pts',(-14.2531968841308,18.2817438134852,9.52766522013385));
#46401=CARTESIAN_POINT('Ctrl Pts',(-14.2846839504599,18.2486918389125,9.50279141917903));
#46402=CARTESIAN_POINT('Ctrl Pts',(-14.3162385566473,18.2160051198467,9.47733130486547));
#46403=CARTESIAN_POINT('Ctrl Pts',(-14.3177571907933,18.2144320003028,9.47610598141418));
#46404=CARTESIAN_POINT('Ctrl Pts',(-14.3192759817155,18.2128597284681,9.47487929772981));
#46405=CARTESIAN_POINT('Ctrl Pts',(-14.3207949288989,18.2112883047585,9.47365125229762));
#46406=CARTESIAN_POINT('Ctrl Pts',(-14.3372603013804,18.1942540872504,9.46033925192903));
#46407=CARTESIAN_POINT('Ctrl Pts',(-14.3537439534659,18.1773193481409,9.44686748678888));
#46408=CARTESIAN_POINT('Ctrl Pts',(-14.3702452789957,18.160484438606,9.43323407054952));
#46409=CARTESIAN_POINT('Ctrl Pts',(-14.3703200984053,18.160408106678,9.43317225465766));
#46410=CARTESIAN_POINT('Ctrl Pts',(-14.3703949181347,18.1603317768519,9.43311043547205));
#46411=CARTESIAN_POINT('Ctrl Pts',(-14.3704697381797,18.1602554491316,9.433048612996));
#46412=CARTESIAN_POINT('Ctrl Pts',(-14.3787578810354,18.1518002945171,9.42620026757015));
#46413=CARTESIAN_POINT('Ctrl Pts',(-14.3870535870957,18.1433672280733,9.41930847928004));
#46414=CARTESIAN_POINT('Ctrl Pts',(-14.3953439616599,18.1349691748069,9.41238384586159));
#46415=CARTESIAN_POINT('Ctrl Pts',(-14.4036343362241,18.1265711215405,9.40545921244314));
#46416=CARTESIAN_POINT('Ctrl Pts',(-14.4119193906067,18.1182081087496,9.39850171532258));
#46417=CARTESIAN_POINT('Ctrl Pts',(-14.4201990643658,18.1098799082598,9.39151134982619));
#46418=CARTESIAN_POINT('Ctrl Pts',(-14.421558271936,18.1085127344458,9.39036379764265));
#46419=CARTESIAN_POINT('Ctrl Pts',(-14.422917280404,18.1071465552667,9.38921540373944));
#46420=CARTESIAN_POINT('Ctrl Pts',(-14.4242760645572,18.1057813955388,9.38806618855738));
#46421=CARTESIAN_POINT('Ctrl Pts',(-14.4602193317155,18.0696694783551,9.35766654913436));
#46422=CARTESIAN_POINT('Ctrl Pts',(-14.4960648528319,18.0342100318951,9.32664377669584));
#46423=CARTESIAN_POINT('Ctrl Pts',(-14.5318017642789,17.9993986191631,9.29499961802803));
#46424=CARTESIAN_POINT('Ctrl Pts',(-14.5605504652558,17.9713944393194,9.26954334835129));
#46425=CARTESIAN_POINT('Ctrl Pts',(-14.5892289079274,17.943809019562,9.24368540990711));
#46426=CARTESIAN_POINT('Ctrl Pts',(-14.6178313776236,17.9166428216246,9.21742470121035));
#46427=CARTESIAN_POINT('Ctrl Pts',(-14.6602094841027,17.8763927298999,9.17851620410542));
#46428=CARTESIAN_POINT('Ctrl Pts',(-14.7024236203372,17.8370594141368,9.13872159295134));
#46429=CARTESIAN_POINT('Ctrl Pts',(-14.7444610537933,17.798639696996,9.09803104691099));
#46430=CARTESIAN_POINT('Ctrl Pts',(-14.7673987745469,17.7776759827358,9.07582825512162));
#46431=CARTESIAN_POINT('Ctrl Pts',(-14.7902838993704,17.7569842878885,9.05335872280684));
#46432=CARTESIAN_POINT('Ctrl Pts',(-14.8131141999115,17.7365661645866,9.03061927808011));
#46433=CARTESIAN_POINT('Ctrl Pts',(-14.8601963365352,17.6944585773839,8.98372451024983));
#46434=CARTESIAN_POINT('Ctrl Pts',(-14.9070453477554,17.6535123161777,8.93568335712758));
#46435=CARTESIAN_POINT('Ctrl Pts',(-14.9536422378279,17.6137407654663,8.88646686737394));
#46436=CARTESIAN_POINT('Ctrl Pts',(-14.9710496924444,17.5988830901374,8.86808079460306));
#46437=CARTESIAN_POINT('Ctrl Pts',(-14.9884219698747,17.5841893412295,8.84953071609024));
#46438=CARTESIAN_POINT('Ctrl Pts',(-15.005757957724,17.5696612078881,8.83081432981604));
#46439=CARTESIAN_POINT('Ctrl Pts',(-15.0571595476816,17.526584969063,8.77531982779415));
#46440=CARTESIAN_POINT('Ctrl Pts',(-15.1082422038154,17.4849616812795,8.71836542626731));
#46441=CARTESIAN_POINT('Ctrl Pts',(-15.1589777195974,17.4448351333286,8.65988924371568));
#46442=CARTESIAN_POINT('Ctrl Pts',(-15.1711577983194,17.4352019502349,8.64585086259621));
#46443=CARTESIAN_POINT('Ctrl Pts',(-15.1833178750539,17.4256550106342,8.63172479735828));
#46444=CARTESIAN_POINT('Ctrl Pts',(-15.1954574932711,17.416195331879,8.6175098489441));
#46445=CARTESIAN_POINT('Ctrl Pts',(-15.2507634646902,17.373098694612,8.55274903714184));
#46446=CARTESIAN_POINT('Ctrl Pts',(-15.3056449788749,17.3318093226852,8.48614625302313));
#46447=CARTESIAN_POINT('Ctrl Pts',(-15.3600600510067,17.2924229689497,8.4175851121417));
#46448=CARTESIAN_POINT('Ctrl Pts',(-15.3673414639574,17.2871525853053,8.40841077937746));
#46449=CARTESIAN_POINT('Ctrl Pts',(-15.3746145140432,17.281916335781,8.39920133086733));
#46450=CARTESIAN_POINT('Ctrl Pts',(-15.3818790846534,17.276714535136,8.38995641468225));
#46451=CARTESIAN_POINT('Ctrl Pts',(-15.4076486781805,17.2582622004526,8.35716194614907));
#46452=CARTESIAN_POINT('Ctrl Pts',(-15.433311892242,17.2402426999691,8.3239211011398));
#46453=CARTESIAN_POINT('Ctrl Pts',(-15.458862852334,17.2226705080983,8.29021899737143));
#46454=CARTESIAN_POINT('Ctrl Pts',(-15.4638276648221,17.2192560517597,8.28367033442248));
#46455=CARTESIAN_POINT('Ctrl Pts',(-15.4687883226332,17.2158584353545,8.27710413388084));
#46456=CARTESIAN_POINT('Ctrl Pts',(-15.4737447016702,17.2124778330333,8.27052037800331));
#46457=CARTESIAN_POINT('Ctrl Pts',(-15.4813606859533,17.2072831911478,8.26040376244317));
#46458=CARTESIAN_POINT('Ctrl Pts',(-15.4889666118216,17.2021286574388,8.25024566530342));
#46459=CARTESIAN_POINT('Ctrl Pts',(-15.4965623340349,17.1970147003122,8.24004557550053));
#46460=CARTESIAN_POINT('Ctrl Pts',(-15.500311300197,17.1944906411533,8.23501119029698));
#46461=CARTESIAN_POINT('Ctrl Pts',(-15.5040577922121,17.1919764550271,8.22996656269615));
#46462=CARTESIAN_POINT('Ctrl Pts',(-15.5078015824525,17.1894723340246,8.2249119185801));
#46463=CARTESIAN_POINT('Ctrl Pts',(-15.5116430275708,17.1869028942903,8.21972542662477));
#46464=CARTESIAN_POINT('Ctrl Pts',(-15.5154790323891,17.184345787301,8.21453189406302));
#46465=CARTESIAN_POINT('Ctrl Pts',(-15.5193093970066,17.1818011536978,8.20933156444055));
#46466=CARTESIAN_POINT('Ctrl Pts',(-15.5316884204386,17.1735773728976,8.1925250698434));
#46467=CARTESIAN_POINT('Ctrl Pts',(-15.5440097288867,17.1654831610244,8.17564589662492));
#46468=CARTESIAN_POINT('Ctrl Pts',(-15.5562729465418,17.1575189151244,8.15869371101957));
#46469=CARTESIAN_POINT('Ctrl Pts',(-15.5589949305578,17.1557511449805,8.1549309482968));
#46470=CARTESIAN_POINT('Ctrl Pts',(-15.5617140559427,17.1539897665543,8.15116459316442));
#46471=CARTESIAN_POINT('Ctrl Pts',(-15.5644303175793,17.1522347879277,8.14739464025237));
#46472=CARTESIAN_POINT('Ctrl Pts',(-15.6242451117547,17.1135884057392,8.06437651179032));
#46473=CARTESIAN_POINT('Ctrl Pts',(-15.6826710263357,17.0780463286275,7.97961348456311));
#46474=CARTESIAN_POINT('Ctrl Pts',(-15.739650238122,17.045710385027,7.89304092775047));
#46475=CARTESIAN_POINT('Ctrl Pts',(-15.7410835124827,17.0448969957674,7.89086325238204));
#46476=CARTESIAN_POINT('Ctrl Pts',(-15.7425158711234,17.0440856365664,7.88868443145153));
#46477=CARTESIAN_POINT('Ctrl Pts',(-15.7439473131389,17.0432763090081,7.88650446391694));
#46478=CARTESIAN_POINT('Ctrl Pts',(-15.7994222388065,17.0119111641728,7.80202075054952));
#46479=CARTESIAN_POINT('Ctrl Pts',(-15.8535208498676,16.9835963942817,7.71581549314315));
#46480=CARTESIAN_POINT('Ctrl Pts',(-15.9061702459269,16.9584917518482,7.62779804765074));
#46481=CARTESIAN_POINT('Ctrl Pts',(-15.9112471153019,16.956070964529,7.61931071243075));
#46482=CARTESIAN_POINT('Ctrl Pts',(-15.9163104996267,16.9536800690656,7.61080650848719));
#46483=CARTESIAN_POINT('Ctrl Pts',(-15.9213603339769,16.9513192076422,7.60228535346611));
#46484=CARTESIAN_POINT('Ctrl Pts',(-15.970030829791,16.9285651353192,7.52015813680427));
#46485=CARTESIAN_POINT('Ctrl Pts',(-16.017443148426,16.908599481043,7.43645711852202));
#46486=CARTESIAN_POINT('Ctrl Pts',(-16.0635184121896,16.891616430166,7.35107816654769));
#46487=CARTESIAN_POINT('Ctrl Pts',(-16.0717041578125,16.88859921609,7.33590971551069));
#46488=CARTESIAN_POINT('Ctrl Pts',(-16.0798476086457,16.8856763078134,7.32068835327566));
#46489=CARTESIAN_POINT('Ctrl Pts',(-16.0879483499438,16.88284880545,7.30541341996439));
#46490=CARTESIAN_POINT('Ctrl Pts',(-16.1147581040427,16.873491063944,7.25486036674568));
#46491=CARTESIAN_POINT('Ctrl Pts',(-16.1410995143865,16.8651800504117,7.20371978428443));
#46492=CARTESIAN_POINT('Ctrl Pts',(-16.16695329123,16.8579688556867,7.15196177803975));
#46493=CARTESIAN_POINT('Ctrl Pts',(-16.1798695718559,16.854366217075,7.12610401120998));
#46494=CARTESIAN_POINT('Ctrl Pts',(-16.1926640919658,16.8510382409624,7.10009206849362));
#46495=CARTESIAN_POINT('Ctrl Pts',(-16.2053341041957,16.8479925917601,7.07392174227086));
#46496=CARTESIAN_POINT('Ctrl Pts',(-16.207248100535,16.847532500537,7.06996831999477));
#46497=CARTESIAN_POINT('Ctrl Pts',(-16.2091593148357,16.8470788585248,7.06601112699843));
#46498=CARTESIAN_POINT('Ctrl Pts',(-16.2110675167977,16.8466317303188,7.06205063036694));
#46499=CARTESIAN_POINT('Ctrl Pts',(-16.217000474151,16.8452415249684,7.04973670444064));
#46500=CARTESIAN_POINT('Ctrl Pts',(-16.2229080555058,16.8439135616734,7.0373828841659));
#46501=CARTESIAN_POINT('Ctrl Pts',(-16.2287732539462,16.8426519143645,7.02502447530824));
#46502=CARTESIAN_POINT('Ctrl Pts',(-16.2335040116055,16.8416342936086,7.0150564174576));
#46503=CARTESIAN_POINT('Ctrl Pts',(-16.2382100622439,16.8406591492381,7.00507941805309));
#46504=CARTESIAN_POINT('Ctrl Pts',(-16.2428892811382,16.8397271892998,6.99509766222573));
#46505=CARTESIAN_POINT('Ctrl Pts',(-16.2440113628681,16.839503704303,6.99270402642913));
#46506=CARTESIAN_POINT('Ctrl Pts',(-16.24513203341,16.8392826651952,6.9903098519872));
#46507=CARTESIAN_POINT('Ctrl Pts',(-16.2462513124443,16.8390640709198,6.98791509430535));
#46508=CARTESIAN_POINT('Ctrl Pts',(-16.2578249331307,16.8368037523125,6.96315271048787));
#46509=CARTESIAN_POINT('Ctrl Pts',(-16.2692417829089,16.8348066794356,6.93834479185663));
#46510=CARTESIAN_POINT('Ctrl Pts',(-16.2805015918988,16.8330742819549,6.91349131223052));
#46511=CARTESIAN_POINT('Ctrl Pts',(-16.3030212098786,16.8296094869936,6.86378435297832));
#46512=CARTESIAN_POINT('Ctrl Pts',(-16.3249126668437,16.8272033934617,6.81389514748906));
#46513=CARTESIAN_POINT('Ctrl Pts',(-16.3461718488325,16.8258727062833,6.76382298919644));
#46514=CARTESIAN_POINT('Ctrl Pts',(-16.3585128827858,16.8251002374433,6.73475591568759));
#46515=CARTESIAN_POINT('Ctrl Pts',(-16.3706406252239,16.8246907899988,6.70562711760921));
#46516=CARTESIAN_POINT('Ctrl Pts',(-16.3825543362793,16.8246474124682,6.67643650814875));
#46517=CARTESIAN_POINT('Ctrl Pts',(-16.4116867405569,16.8245413420967,6.60505718461495));
#46518=CARTESIAN_POINT('Ctrl Pts',(-16.4395395922015,16.8266234509508,6.53330838124095));
#46519=CARTESIAN_POINT('Ctrl Pts',(-16.4660876043868,16.830974861643,6.46118444796423));
#46520=CARTESIAN_POINT('Ctrl Pts',(-16.4793737111767,16.8331525503806,6.42508960692901));
#46521=CARTESIAN_POINT('Ctrl Pts',(-16.4923325381101,16.835899902222,6.38890068074229));
#46522=CARTESIAN_POINT('Ctrl Pts',(-16.5049608875163,16.8392270469745,6.35261705451585));
#46523=CARTESIAN_POINT('Ctrl Pts',(-16.5278855658781,16.8452669276318,6.28675013602257));
#46524=CARTESIAN_POINT('Ctrl Pts',(-16.5497215555428,16.8532163974352,6.22057127274915));
#46525=CARTESIAN_POINT('Ctrl Pts',(-16.5704362939606,16.8631707652677,6.15407282388274));
#46526=CARTESIAN_POINT('Ctrl Pts',(-16.5839479628594,16.8696637327162,6.11069766725516));
#46527=CARTESIAN_POINT('Ctrl Pts',(-16.5969825403869,16.8770097708918,6.06718658073939));
#46528=CARTESIAN_POINT('Ctrl Pts',(-16.6095299784033,16.885238026301,6.0235372341579));
#46529=CARTESIAN_POINT('Ctrl Pts',(-16.6118991067048,16.8867916337176,6.01529563916504));
#46530=CARTESIAN_POINT('Ctrl Pts',(-16.614250835039,16.8883767774259,6.00704910784024));
#46531=CARTESIAN_POINT('Ctrl Pts',(-16.6165850775924,16.8899936994925,5.99879762134841));
#46532=CARTESIAN_POINT('Ctrl Pts',(-16.6181662314661,16.8910889595311,5.99320828368015));
#46533=CARTESIAN_POINT('Ctrl Pts',(-16.6197392455601,16.8921986796151,5.98761712958495));
#46534=CARTESIAN_POINT('Ctrl Pts',(-16.6213041889455,16.8933229998439,5.98202381843932));
#46535=CARTESIAN_POINT('Ctrl Pts',(-16.6233758056449,16.894811335194,5.97461959098788));
#46536=CARTESIAN_POINT('Ctrl Pts',(-16.6254340295377,16.8963258504435,5.96720881741333));
#46537=CARTESIAN_POINT('Ctrl Pts',(-16.6274776180581,16.897865794274,5.95979582904516));
#46538=CARTESIAN_POINT('Ctrl Pts',(-16.6292570586422,16.8992066897243,5.95334102064287));
#46539=CARTESIAN_POINT('Ctrl Pts',(-16.631025572609,16.9005669866222,5.94688392154869));
#46540=CARTESIAN_POINT('Ctrl Pts',(-16.6327818099178,16.9019457784013,5.94042932478974));
#46541=CARTESIAN_POINT('Ctrl Pts',(-16.6345661535421,16.9033466359665,5.93387143052549));
#46542=CARTESIAN_POINT('Ctrl Pts',(-16.6363372586855,16.9047660921804,5.92731827230297));
#46543=CARTESIAN_POINT('Ctrl Pts',(-16.6380947701799,16.9062037955367,5.92077133421867));
#46544=CARTESIAN_POINT('Ctrl Pts',(-16.6437740492813,16.9108496363473,5.89961534817929));
#46545=CARTESIAN_POINT('Ctrl Pts',(-16.6493146604464,16.9156889677414,5.87851181846174));
#46546=CARTESIAN_POINT('Ctrl Pts',(-16.6547182018872,16.9207206527441,5.85746057140922));
#46547=CARTESIAN_POINT('Ctrl Pts',(-16.6559507078088,16.9218683410943,5.85265894511777));
#46548=CARTESIAN_POINT('Ctrl Pts',(-16.6571760846858,16.9230260331474,5.8478600378164));
#46549=CARTESIAN_POINT('Ctrl Pts',(-16.6583943491292,16.9241937195169,5.8430638481694));
#46550=CARTESIAN_POINT('Ctrl Pts',(-16.6711840856364,16.9364524709472,5.79271188874387));
#46551=CARTESIAN_POINT('Ctrl Pts',(-16.6831889826383,16.949814692948,5.74265997630306));
#46552=CARTESIAN_POINT('Ctrl Pts',(-16.6944254022008,16.9642745561676,5.69290880673133));
#46553=CARTESIAN_POINT('Ctrl Pts',(-16.7062399084323,16.979478344453,5.64059805955267));
#46554=CARTESIAN_POINT('Ctrl Pts',(-16.7172058453786,16.9958937260294,5.58861931331693));
#46555=CARTESIAN_POINT('Ctrl Pts',(-16.7273360612814,17.013524763337,5.53697595623463));
#46556=CARTESIAN_POINT('Ctrl Pts',(-16.7383690919225,17.0327270959147,5.48073009271422));
#46557=CARTESIAN_POINT('Ctrl Pts',(-16.7484107574535,17.0533714712242,5.42488213752166));
#46558=CARTESIAN_POINT('Ctrl Pts',(-16.7574767467459,17.0754640501639,5.36943744760249));
#46559=CARTESIAN_POINT('Ctrl Pts',(-16.7646517241534,17.0929484911502,5.32555758135657));
#46560=CARTESIAN_POINT('Ctrl Pts',(-16.7712156377876,17.1113397698573,5.28193022356205));
#46561=CARTESIAN_POINT('Ctrl Pts',(-16.7771711177175,17.1306506982287,5.23856061432427));
#46562=CARTESIAN_POINT('Ctrl Pts',(-16.7857032969204,17.1583166971708,5.17642670029277));
#46563=CARTESIAN_POINT('Ctrl Pts',(-16.7929878087474,17.1878678868144,5.11482118509071));
#46564=CARTESIAN_POINT('Ctrl Pts',(-16.7990319439269,17.2193417178198,5.05376028262675));
#46565=CARTESIAN_POINT('Ctrl Pts',(-16.8025373454865,17.2375955147675,5.0183469478207));
#46566=CARTESIAN_POINT('Ctrl Pts',(-16.8056249923219,17.2564970784941,4.9831170877998));
#46567=CARTESIAN_POINT('Ctrl Pts',(-16.8082939481964,17.2760584841819,4.94807520570957));
#46568=CARTESIAN_POINT('Ctrl Pts',(-16.8095429904173,17.2852130085553,4.93167598733007));
#46569=CARTESIAN_POINT('Ctrl Pts',(-16.8107003335015,17.2945118620255,4.91531818116869));
#46570=CARTESIAN_POINT('Ctrl Pts',(-16.8117658798418,17.3039556942957,4.89900304955538));
#46571=CARTESIAN_POINT('Ctrl Pts',(-16.8122510098167,17.3082553534842,4.89157497337359));
#46572=CARTESIAN_POINT('Ctrl Pts',(-16.8127172005031,17.3125869477479,4.88415283348946));
#46573=CARTESIAN_POINT('Ctrl Pts',(-16.8131642431758,17.3169475780613,4.87674150730954));
#46574=CARTESIAN_POINT('Ctrl Pts',(-16.8138787099376,17.3239167682738,4.86489667338347));
#46575=CARTESIAN_POINT('Ctrl Pts',(-16.8145449498413,17.3309677138809,4.85306683516652));
#46576=CARTESIAN_POINT('Ctrl Pts',(-16.8151607441959,17.3380741191068,4.84129616134881));
#46577=CARTESIAN_POINT('Ctrl Pts',(-16.8154888696785,17.3418607609082,4.83502416811295));
#46578=CARTESIAN_POINT('Ctrl Pts',(-16.815802859543,17.345665122089,4.82876566522662));
#46579=CARTESIAN_POINT('Ctrl Pts',(-16.8161026019274,17.3494855415575,4.82252343039461));
#46580=CARTESIAN_POINT('Ctrl Pts',(-16.8163653872281,17.3528349179926,4.8170508391198));
#46581=CARTESIAN_POINT('Ctrl Pts',(-16.8166173448659,17.3561974209022,4.81158930335026));
#46582=CARTESIAN_POINT('Ctrl Pts',(-16.8168585431549,17.3595730738688,4.80613867917317));
#46583=CARTESIAN_POINT('Ctrl Pts',(-16.8177333839499,17.3718167715219,4.78636893533259));
#46584=CARTESIAN_POINT('Ctrl Pts',(-16.8184664384501,17.3842314930117,4.76674627660528));
#46585=CARTESIAN_POINT('Ctrl Pts',(-16.8190606453201,17.3968154028595,4.74726906352365));
#46586=CARTESIAN_POINT('Ctrl Pts',(-16.8198692059289,17.4139388228674,4.72076565526566));
#46587=CARTESIAN_POINT('Ctrl Pts',(-16.82042126738,17.4313747980671,4.69453101225618));
#46588=CARTESIAN_POINT('Ctrl Pts',(-16.8207228409782,17.4491203250095,4.66856224559516));
#46589=CARTESIAN_POINT('Ctrl Pts',(-16.8215560496239,17.4981489089408,4.59681391938496));
#46590=CARTESIAN_POINT('Ctrl Pts',(-16.820480330705,17.5495354930376,4.52709118335943));
#46591=CARTESIAN_POINT('Ctrl Pts',(-16.8176176508208,17.6032206644751,4.45933945087101));
#46592=CARTESIAN_POINT('Ctrl Pts',(-16.8168851937344,17.6169567739388,4.44200421305957));
#46593=CARTESIAN_POINT('Ctrl Pts',(-16.8160356997886,17.6308433811587,4.42479803834067));
#46594=CARTESIAN_POINT('Ctrl Pts',(-16.8150705444703,17.6448803145444,4.4077206653306));
#46595=CARTESIAN_POINT('Ctrl Pts',(-16.8108707290189,17.7059611878581,4.3334095014392));
#46596=CARTESIAN_POINT('Ctrl Pts',(-16.804484970729,17.7698819222335,4.26153195563804));
#46597=CARTESIAN_POINT('Ctrl Pts',(-16.7960260709805,17.836624529602,4.19206773199594));
#46598=CARTESIAN_POINT('Ctrl Pts',(-16.7949435260831,17.845166050508,4.18317790671273));
#46599=CARTESIAN_POINT('Ctrl Pts',(-16.7938269626664,17.8537538688681,4.1743276718339));
#46600=CARTESIAN_POINT('Ctrl Pts',(-16.7926765400346,17.8623880506822,4.16551706644754));
#46601=CARTESIAN_POINT('Ctrl Pts',(-16.7882774357282,17.8954043225738,4.13182616796633));
#46602=CARTESIAN_POINT('Ctrl Pts',(-16.7833836442642,17.9290978128492,4.09871424594278));
#46603=CARTESIAN_POINT('Ctrl Pts',(-16.7780042088693,17.9634716718842,4.06618342561398));
#46604=CARTESIAN_POINT('Ctrl Pts',(-16.7771839813685,17.9687128138295,4.06122330034071));
#46605=CARTESIAN_POINT('Ctrl Pts',(-16.7763524570089,17.9739697823373,4.05627669175243));
#46606=CARTESIAN_POINT('Ctrl Pts',(-16.7755096616605,17.9792425973972,4.05134361419153));
#46607=CARTESIAN_POINT('Ctrl Pts',(-16.774606322161,17.9848941973095,4.04605615760648));
#46608=CARTESIAN_POINT('Ctrl Pts',(-16.7736900416366,17.9905639652448,4.04078427420014));
#46609=CARTESIAN_POINT('Ctrl Pts',(-16.772760844743,17.9962519732155,4.03552793535613));
#46610=CARTESIAN_POINT('Ctrl Pts',(-16.7709635554923,18.0072539423928,4.02536091761548));
#46611=CARTESIAN_POINT('Ctrl Pts',(-16.7691170692686,18.0183290120654,4.0152478267625));
#46612=CARTESIAN_POINT('Ctrl Pts',(-16.7672278724432,18.0294413032003,4.00522090599292));
#46613=CARTESIAN_POINT('Ctrl Pts',(-16.7666499510457,18.0328406476918,4.00215358553933));
#46614=CARTESIAN_POINT('Ctrl Pts',(-16.7660679300489,18.0362441268367,3.99909371537179));
#46615=CARTESIAN_POINT('Ctrl Pts',(-16.7654818289922,18.0396517394221,3.99604126463338));
#46616=CARTESIAN_POINT('Ctrl Pts',(-16.7622326330158,18.0585426814793,3.97911925000119));
#46617=CARTESIAN_POINT('Ctrl Pts',(-16.758857941205,18.0775606054575,3.96242577932828));
#46618=CARTESIAN_POINT('Ctrl Pts',(-16.7553616195243,18.0967033857874,3.94595641211867));
#46619=CARTESIAN_POINT('Ctrl Pts',(-16.7550997309887,18.0981372569145,3.94472279037113));
#46620=CARTESIAN_POINT('Ctrl Pts',(-16.7548371621615,18.0995718268212,3.94349042298232));
#46621=CARTESIAN_POINT('Ctrl Pts',(-16.7545739143653,18.1010070948678,3.94225930848775));
#46622=CARTESIAN_POINT('Ctrl Pts',(-16.7394630496698,18.1833938862189,3.87159127318213));
#46623=CARTESIAN_POINT('Ctrl Pts',(-16.7221122255081,18.2680851147759,3.80505793177941));
#46624=CARTESIAN_POINT('Ctrl Pts',(-16.7027490566819,18.3549810994009,3.74243609542314));
#46625=CARTESIAN_POINT('Ctrl Pts',(-16.7011252984973,18.3622680299395,3.73718474838229));
#46626=CARTESIAN_POINT('Ctrl Pts',(-16.6994873679414,18.3695704916422,3.73196094643881));
#46627=CARTESIAN_POINT('Ctrl Pts',(-16.6978353988412,18.3768884221525,3.72676456101778));
#46628=CARTESIAN_POINT('Ctrl Pts',(-16.6797877865089,18.4568361481147,3.66999452240542));
#46629=CARTESIAN_POINT('Ctrl Pts',(-16.660063932005,18.5386304234911,3.61649763813193));
#46630=CARTESIAN_POINT('Ctrl Pts',(-16.6387816406185,18.6222388096108,3.56618605682596));
#46631=CARTESIAN_POINT('Ctrl Pts',(-16.6343665117779,18.6395838308854,3.55574864153051));
#46632=CARTESIAN_POINT('Ctrl Pts',(-16.6298845307761,18.6570058438323,3.54544919702397));
#46633=CARTESIAN_POINT('Ctrl Pts',(-16.6253365723563,18.6745052073658,3.53528656580386));
#46634=CARTESIAN_POINT('Ctrl Pts',(-16.6120568488463,18.725602136554,3.50561238669301));
#46635=CARTESIAN_POINT('Ctrl Pts',(-16.5982133624414,18.7773596411757,3.47710648804274));
#46636=CARTESIAN_POINT('Ctrl Pts',(-16.5838189315666,18.8297952185675,3.4497540158));
#46637=CARTESIAN_POINT('Ctrl Pts',(-16.5772052155726,18.8538874539513,3.43718655240246));
#46638=CARTESIAN_POINT('Ctrl Pts',(-16.5704722809959,18.8781329439034,3.42485779907269));
#46639=CARTESIAN_POINT('Ctrl Pts',(-16.5636289474838,18.9025052790382,3.4127811710977));
#46640=CARTESIAN_POINT('Ctrl Pts',(-16.5630150703628,18.9046915847181,3.41169784444109));
#46641=CARTESIAN_POINT('Ctrl Pts',(-16.562400271962,18.9068790266346,3.41061649162404));
#46642=CARTESIAN_POINT('Ctrl Pts',(-16.5617845583766,18.9090675860316,3.40953712293799));
#46643=CARTESIAN_POINT('Ctrl Pts',(-16.5543053966033,18.9356523328526,3.39642587574771));
#46644=CARTESIAN_POINT('Ctrl Pts',(-16.5467123462032,18.9623271295586,3.3836439251165));
#46645=CARTESIAN_POINT('Ctrl Pts',(-16.5390081804392,18.9890932965675,3.37118496984572));
#46646=CARTESIAN_POINT('Ctrl Pts',(-16.5196180850813,19.0564592576034,3.33982786536966));
#46647=CARTESIAN_POINT('Ctrl Pts',(-16.4995268262444,19.1244028255936,3.31051116810786));
#46648=CARTESIAN_POINT('Ctrl Pts',(-16.4787633867405,19.1929521614537,3.28316660603189));
#46649=CARTESIAN_POINT('Ctrl Pts',(-16.4665990140822,19.2331121583907,3.26714664733446));
#46650=CARTESIAN_POINT('Ctrl Pts',(-16.4542052664158,19.2734744522462,3.25180765814332));
#46651=CARTESIAN_POINT('Ctrl Pts',(-16.4415901717203,19.3140374655582,3.23713906453767));
#46652=CARTESIAN_POINT('Ctrl Pts',(-16.4234126569237,19.372486077516,3.21600259400401));
#46653=CARTESIAN_POINT('Ctrl Pts',(-16.4047752775749,19.4313515251799,3.19625859049243));
#46654=CARTESIAN_POINT('Ctrl Pts',(-16.3856913105911,19.4906335657926,3.17789716423366));
#46655=CARTESIAN_POINT('',(2.06506260776231,19.4906334205523,-16.5627719180504));
#46656=CARTESIAN_POINT('Origin',(6.61325378140121E-15,19.4906334205523,
8.67361737988404E-16));
#46657=CARTESIAN_POINT('',(6.78574855947105,19.4906334205522,-15.2493774847033));
#46658=CARTESIAN_POINT('Ctrl Pts',(2.06506260776273,19.4906334205533,-16.5627719180497));
#46659=CARTESIAN_POINT('Ctrl Pts',(2.41742332821393,19.349939283335,-16.5720080472377));
#46660=CARTESIAN_POINT('Ctrl Pts',(2.76269377024947,19.2344262533423,-16.5621715122885));
#46661=CARTESIAN_POINT('Ctrl Pts',(3.44112953030319,19.0724697614237,-16.495689659873));
#46662=CARTESIAN_POINT('Ctrl Pts',(3.75758071471907,19.0223948272706,-16.4459328577175));
#46663=CARTESIAN_POINT('Ctrl Pts',(4.22465776181844,18.9889208004819,-16.3426280057139));
#46664=CARTESIAN_POINT('Ctrl Pts',(4.37312530932789,18.984322683773,-16.3053159474107));
#46665=CARTESIAN_POINT('Ctrl Pts',(4.59196989806894,18.9864292907932,-16.2436668872455));
#46666=CARTESIAN_POINT('Ctrl Pts',(4.66297798251051,18.9885240740547,-16.2226078396245));
#46667=CARTESIAN_POINT('Ctrl Pts',(4.76322511787825,18.9934497272694,-16.1913920375261));
#46668=CARTESIAN_POINT('Ctrl Pts',(4.7927075198343,18.9951414505049,-16.1820279768777));
#46669=CARTESIAN_POINT('Ctrl Pts',(4.83538292817332,18.9979409897723,-16.1682080344538));
#46670=CARTESIAN_POINT('Ctrl Pts',(4.84862882894517,18.9988591807016,-16.1638812207154));
#46671=CARTESIAN_POINT('Ctrl Pts',(4.91979031300025,19.0040561695104,-16.1404359378585));
#46672=CARTESIAN_POINT('Ctrl Pts',(4.97741481102364,19.0092070140339,-16.1207366039373));
#46673=CARTESIAN_POINT('Ctrl Pts',(5.11930956255435,19.0241842792193,-16.0704800244993));
#46674=CARTESIAN_POINT('Ctrl Pts',(5.2031675870547,19.0350630426818,-16.0392332038417));
#46675=CARTESIAN_POINT('Ctrl Pts',(5.46110025027662,19.074570039631,-15.9384495833863));
#46676=CARTESIAN_POINT('Ctrl Pts',(5.63207967254321,19.1095004500619,-15.8648985157062));
#46677=CARTESIAN_POINT('Ctrl Pts',(6.14663187861032,19.2388854970279,-15.6241814045855));
#46678=CARTESIAN_POINT('Ctrl Pts',(6.46898077889003,19.3543537790241,-15.44627066688));
#46679=CARTESIAN_POINT('Ctrl Pts',(6.78574855947051,19.4906334205529,-15.2493774847029));
#46680=CARTESIAN_POINT('',(16.6906704142672,19.4906334305655,0.10686064282603));
#46681=CARTESIAN_POINT('Origin',(6.61325378140121E-15,19.4906334205523,
8.67361737988404E-16));
#46682=CARTESIAN_POINT('',(12.3247145833779,19.4906334205523,11.2557233273388));
#46683=CARTESIAN_POINT('Ctrl Pts',(16.6906704676692,19.4906334505918,0.106860643167889));
#46684=CARTESIAN_POINT('Ctrl Pts',(16.7554332564921,19.3173865856866,0.139157039459681));
#46685=CARTESIAN_POINT('Ctrl Pts',(16.8193252940415,19.1461031307759,0.178612921117866));
#46686=CARTESIAN_POINT('Ctrl Pts',(16.8822218893148,18.9767355755773,0.225223411409203));
#46687=CARTESIAN_POINT('Ctrl Pts',(16.8826470664552,18.9755906612543,0.225538495475169));
#46688=CARTESIAN_POINT('Ctrl Pts',(16.8830721981114,18.9744458344816,0.225853906539962));
#46689=CARTESIAN_POINT('Ctrl Pts',(16.8834972842449,18.9733010952449,0.226169644596096));
#46690=CARTESIAN_POINT('Ctrl Pts',(16.9459553307026,18.8051041798494,0.272561141813467));
#46691=CARTESIAN_POINT('Ctrl Pts',(17.007431128011,18.6387971651158,0.32601057224118));
#46692=CARTESIAN_POINT('Ctrl Pts',(17.0677324304234,18.474366967947,0.386698765732942));
#46693=CARTESIAN_POINT('Ctrl Pts',(17.0738247090014,18.4577544815209,0.392830132160528));
#46694=CARTESIAN_POINT('Ctrl Pts',(17.0799049883242,18.4411611794587,0.3990355131978));
#46695=CARTESIAN_POINT('Ctrl Pts',(17.0859730702553,18.424587051854,0.405315079357435));
#46696=CARTESIAN_POINT('Ctrl Pts',(17.110140279184,18.3585776589057,0.430324561609761));
#46697=CARTESIAN_POINT('Ctrl Pts',(17.134113158127,18.2928728040555,0.456513147980813));
#46698=CARTESIAN_POINT('Ctrl Pts',(17.1578750798263,18.2274735574929,0.483903109577319));
#46699=CARTESIAN_POINT('Ctrl Pts',(17.1666728977386,18.2032595789208,0.494044204131883));
#46700=CARTESIAN_POINT('Ctrl Pts',(17.1754417870569,18.1790875151221,0.504350093439007));
#46701=CARTESIAN_POINT('Ctrl Pts',(17.1841808989709,18.1549574369282,0.514821961053957));
#46702=CARTESIAN_POINT('Ctrl Pts',(17.1902067224447,18.1383191797416,0.522042560390655));
#46703=CARTESIAN_POINT('Ctrl Pts',(17.1962183712914,18.1217008914811,0.529342119502282));
#46704=CARTESIAN_POINT('Ctrl Pts',(17.2022155260639,18.1051026122299,0.536721137196537));
#46705=CARTESIAN_POINT('Ctrl Pts',(17.209562870631,18.0847674230431,0.545761455084535));
#46706=CARTESIAN_POINT('Ctrl Pts',(17.2168884661567,18.0644622546451,0.554920988090242));
#46707=CARTESIAN_POINT('Ctrl Pts',(17.2241917200914,18.0441871936411,0.564200691556757));
#46708=CARTESIAN_POINT('Ctrl Pts',(17.2269375825861,18.0365642176241,0.567689655508839));
#46709=CARTESIAN_POINT('Ctrl Pts',(17.229680508348,18.0289448827969,0.571195887923344));
#46710=CARTESIAN_POINT('Ctrl Pts',(17.2324204715755,18.0213291760418,0.574719454032397));
#46711=CARTESIAN_POINT('Ctrl Pts',(17.2369680718224,18.0086891560694,0.580567623798449));
#46712=CARTESIAN_POINT('Ctrl Pts',(17.2415029342496,17.9960718361261,0.586457709712012));
#46713=CARTESIAN_POINT('Ctrl Pts',(17.2460245379011,17.9834783465572,0.592389106278812));
#46714=CARTESIAN_POINT('Ctrl Pts',(17.2573836593269,17.9518411248512,0.60728989348185));
#46715=CARTESIAN_POINT('Ctrl Pts',(17.2686612397977,17.9203483203527,0.622454523538607));
#46716=CARTESIAN_POINT('Ctrl Pts',(17.2798485678208,17.8890190033201,0.637873157575821));
#46717=CARTESIAN_POINT('Ctrl Pts',(17.3257517832463,17.7604703109143,0.701138029966847));
#46718=CARTESIAN_POINT('Ctrl Pts',(17.3701969574651,17.6345118072375,0.768739601039109));
#46719=CARTESIAN_POINT('Ctrl Pts',(17.4130560019887,17.5110962940719,0.840715969915629));
#46720=CARTESIAN_POINT('Ctrl Pts',(17.4284574345146,17.4667468289871,0.866580736641848));
#46721=CARTESIAN_POINT('Ctrl Pts',(17.4436530655792,17.4227281768419,0.893011286951045));
#46722=CARTESIAN_POINT('Ctrl Pts',(17.4586365955835,17.3790389121479,0.920008840824794));
#46723=CARTESIAN_POINT('Ctrl Pts',(17.4955111628831,17.271519340273,0.986450001016147));
#46724=CARTESIAN_POINT('Ctrl Pts',(17.5311020607058,17.1659947086958,1.05632454162672));
#46725=CARTESIAN_POINT('Ctrl Pts',(17.5652760758296,17.0624873851863,1.12972562705538));
#46726=CARTESIAN_POINT('Ctrl Pts',(17.5834046144217,17.0075791017433,1.168663235208));
#46727=CARTESIAN_POINT('Ctrl Pts',(17.6011335450642,16.953240328626,1.20859594981807));
#46728=CARTESIAN_POINT('Ctrl Pts',(17.618442770531,16.8994741998413,1.24953825060211));
#46729=CARTESIAN_POINT('Ctrl Pts',(17.6470216890427,16.810702012075,1.31713727056023));
#46730=CARTESIAN_POINT('Ctrl Pts',(17.6744578871136,16.7234901850469,1.38748683629434));
#46731=CARTESIAN_POINT('Ctrl Pts',(17.7006253081176,16.637886306578,1.46071191763152));
#46732=CARTESIAN_POINT('Ctrl Pts',(17.7199827879829,16.5745604116187,1.51488053583065));
#46733=CARTESIAN_POINT('Ctrl Pts',(17.738646309133,16.5121137043897,1.5706217131087));
#46734=CARTESIAN_POINT('Ctrl Pts',(17.7565615957351,16.4505703505189,1.62799550309415));
#46735=CARTESIAN_POINT('Ctrl Pts',(17.7580891880836,16.4453227003659,1.63288762480768));
#46736=CARTESIAN_POINT('Ctrl Pts',(17.7596113167566,16.4400816395194,1.63779165267672));
#46737=CARTESIAN_POINT('Ctrl Pts',(17.7611279404093,16.4348471898327,1.64270763524448));
#46738=CARTESIAN_POINT('Ctrl Pts',(17.770039202122,16.4040910091567,1.67159259108592));
#46739=CARTESIAN_POINT('Ctrl Pts',(17.7787607516293,16.3735624005947,1.70088932840607));
#46740=CARTESIAN_POINT('Ctrl Pts',(17.7872844554273,16.3432652299643,1.73060714320661));
#46741=CARTESIAN_POINT('Ctrl Pts',(17.7879926300817,16.340748050948,1.73307618761802));
#46742=CARTESIAN_POINT('Ctrl Pts',(17.7886994386785,16.3382324698041,1.73554813918163));
#46743=CARTESIAN_POINT('Ctrl Pts',(17.7894048762293,16.335718489019,1.73802300370958));
#46744=CARTESIAN_POINT('Ctrl Pts',(17.7936629409595,16.3205439453602,1.75296143921885));
#46745=CARTESIAN_POINT('Ctrl Pts',(17.7978713134397,16.3054267654372,1.7680069588093));
#46746=CARTESIAN_POINT('Ctrl Pts',(17.8020281525554,16.2903702106543,1.78315803810895));
#46747=CARTESIAN_POINT('Ctrl Pts',(17.8023601028744,16.2891678479878,1.78436794916567));
#46748=CARTESIAN_POINT('Ctrl Pts',(17.8026917396659,16.2879658150709,1.78557859340076));
#46749=CARTESIAN_POINT('Ctrl Pts',(17.8030230558681,16.2867641364131,1.7867899461418));
#46750=CARTESIAN_POINT('Ctrl Pts',(17.8075032704746,16.2705144684552,1.80317043163647));
#46751=CARTESIAN_POINT('Ctrl Pts',(17.8119262462366,16.2543245055393,1.81968570898484));
#46752=CARTESIAN_POINT('Ctrl Pts',(17.8162742104404,16.2382558357076,1.83627399178503));
#46753=CARTESIAN_POINT('Ctrl Pts',(17.8162953962977,16.238177539629,1.8363548197259));
#46754=CARTESIAN_POINT('Ctrl Pts',(17.816316580384,16.2380992463939,1.83643564943822));
#46755=CARTESIAN_POINT('Ctrl Pts',(17.8163377626971,16.2380209560091,1.8365164809153));
#46756=CARTESIAN_POINT('Ctrl Pts',(17.8350686489185,16.168791109381,1.90799333949187));
#46757=CARTESIAN_POINT('Ctrl Pts',(17.8524671078719,16.1015998621785,1.98103401675485));
#46758=CARTESIAN_POINT('Ctrl Pts',(17.8684852965537,16.0364294729093,2.05563176347801));
#46759=CARTESIAN_POINT('Ctrl Pts',(17.8821901849448,15.9806708019961,2.11945632025969));
#46760=CARTESIAN_POINT('Ctrl Pts',(17.8948867344368,15.9263883328354,2.18441855727403));
#46761=CARTESIAN_POINT('Ctrl Pts',(17.9065346466881,15.8735871519442,2.25052542310617));
#46762=CARTESIAN_POINT('Ctrl Pts',(17.9220146524199,15.8034146982716,2.33838105250214));
#46763=CARTESIAN_POINT('Ctrl Pts',(17.9356436345352,15.735856243357,2.42825707097301));
#46764=CARTESIAN_POINT('Ctrl Pts',(17.9473244533597,15.6709250091733,2.52017572255856));
#46765=CARTESIAN_POINT('Ctrl Pts',(17.9547172544272,15.6298299708379,2.57835112239702));
#46766=CARTESIAN_POINT('Ctrl Pts',(17.9613282438511,15.5897895312754,2.6373462328043));
#46767=CARTESIAN_POINT('Ctrl Pts',(17.9671255285473,15.5508170878235,2.69717341994217));
#46768=CARTESIAN_POINT('Ctrl Pts',(17.9693245013501,15.5360344184021,2.71986651925895));
#46769=CARTESIAN_POINT('Ctrl Pts',(17.9714064145044,15.5214053613257,2.74267934384877));
#46770=CARTESIAN_POINT('Ctrl Pts',(17.9733695519132,15.5069305580775,2.7656125562293));
#46771=CARTESIAN_POINT('Ctrl Pts',(17.9780829256348,15.4721774343545,2.82067380670434));
#46772=CARTESIAN_POINT('Ctrl Pts',(17.9821116985938,15.4383134582655,2.87642898490496));
#46773=CARTESIAN_POINT('Ctrl Pts',(17.9854278507014,15.4053528371821,2.93289108280594));
#46774=CARTESIAN_POINT('Ctrl Pts',(17.9871214137631,15.3885198064447,2.96172634737995));
#46775=CARTESIAN_POINT('Ctrl Pts',(17.9886290074013,15.3719225948283,2.99074613159763));
#46776=CARTESIAN_POINT('Ctrl Pts',(17.9899468566142,15.3555631122618,3.01995223286669));
#46777=CARTESIAN_POINT('Ctrl Pts',(17.9922842524111,15.3265472086113,3.07175346906009));
#46778=CARTESIAN_POINT('Ctrl Pts',(17.9940248324192,15.2982790927692,3.12414077166325));
#46779=CARTESIAN_POINT('Ctrl Pts',(17.9951437711287,15.2707738254319,3.17712733298565));
#46780=CARTESIAN_POINT('Ctrl Pts',(17.9958860934773,15.2525263785625,3.21227948950411));
#46781=CARTESIAN_POINT('Ctrl Pts',(17.9963548145827,15.2346143329278,3.24769611805471));
#46782=CARTESIAN_POINT('Ctrl Pts',(17.9965424157188,15.217043464621,3.28337941396034));
#46783=CARTESIAN_POINT('Ctrl Pts',(17.9965759220781,15.2139052329469,3.28975260209714));
#46784=CARTESIAN_POINT('Ctrl Pts',(17.9966004535718,15.2107778316002,3.29613443020691));
#46785=CARTESIAN_POINT('Ctrl Pts',(17.996615963183,15.2076613246323,3.30252485909978));
#46786=CARTESIAN_POINT('Ctrl Pts',(17.9966671369206,15.1973784549953,3.32360998674614));
#46787=CARTESIAN_POINT('Ctrl Pts',(17.9966201386314,15.1872142054475,3.34478847787987));
#46788=CARTESIAN_POINT('Ctrl Pts',(17.996473262686,15.1771697287181,3.36606132847237));
#46789=CARTESIAN_POINT('Ctrl Pts',(17.9963998247132,15.1721474903534,3.37669775376862));
#46790=CARTESIAN_POINT('Ctrl Pts',(17.996301417629,15.1671551934491,3.38735776816199));
#46791=CARTESIAN_POINT('Ctrl Pts',(17.9961778220592,15.1621929880374,3.39804150044135));
#46792=CARTESIAN_POINT('Ctrl Pts',(17.9960987266352,15.1590174070552,3.404878592869));
#46793=CARTESIAN_POINT('Ctrl Pts',(17.9960093131326,15.1558540955849,3.41172551884406));
#46794=CARTESIAN_POINT('Ctrl Pts',(17.9959095368297,15.1527034975434,3.41858143252991));
#46795=CARTESIAN_POINT('Ctrl Pts',(17.9958534013443,15.1509309288511,3.42243866147377));
#46796=CARTESIAN_POINT('Ctrl Pts',(17.9957940138343,15.1491632483792,3.42629685157856));
#46797=CARTESIAN_POINT('Ctrl Pts',(17.9957313769541,15.1474005156812,3.43015585664521));
#46798=CARTESIAN_POINT('Ctrl Pts',(17.9950561047956,15.1283969460774,3.47175880159095));
#46799=CARTESIAN_POINT('Ctrl Pts',(17.9940028406359,15.1099587858533,3.51347756260468));
#46800=CARTESIAN_POINT('Ctrl Pts',(17.9925715579667,15.0920785076305,3.55530998373131));
#46801=CARTESIAN_POINT('Ctrl Pts',(17.9910529348596,15.0731071302408,3.59969512351652));
#46802=CARTESIAN_POINT('Ctrl Pts',(17.9891089067087,15.0547634660304,3.64420815159584));
#46803=CARTESIAN_POINT('Ctrl Pts',(17.9867385000125,15.0370405505643,3.68884690964006));
#46804=CARTESIAN_POINT('Ctrl Pts',(17.9842315841771,15.0182969917055,3.73605636512686));
#46805=CARTESIAN_POINT('Ctrl Pts',(17.98124774844,15.0002478006414,3.78340641977283));
#46806=CARTESIAN_POINT('Ctrl Pts',(17.9777857836728,14.9828847689785,3.83089464581435));
#46807=CARTESIAN_POINT('Ctrl Pts',(17.9710601427838,14.9491531964285,3.92315114646949));
#46808=CARTESIAN_POINT('Ctrl Pts',(17.9625299443818,14.9180114764903,4.01592917751899));
#46809=CARTESIAN_POINT('Ctrl Pts',(17.9521757527204,14.8894208769911,4.10921510859279));
#46810=CARTESIAN_POINT('Ctrl Pts',(17.9482813090824,14.8786673114816,4.14430203885945));
#46811=CARTESIAN_POINT('Ctrl Pts',(17.9441288257152,14.8682746592604,4.1794608228901));
#46812=CARTESIAN_POINT('Ctrl Pts',(17.939716716368,14.8582419102149,4.21469093389021));
#46813=CARTESIAN_POINT('Ctrl Pts',(17.9324154880939,14.8416395585428,4.27299027832925));
#46814=CARTESIAN_POINT('Ctrl Pts',(17.9244033804411,14.8260225892159,4.33148490202253));
#46815=CARTESIAN_POINT('Ctrl Pts',(17.9156731062911,14.8113863758173,4.39017270789179));
#46816=CARTESIAN_POINT('Ctrl Pts',(17.9016880401047,14.7879405584717,4.48418497317845));
#46817=CARTESIAN_POINT('Ctrl Pts',(17.8858601407598,14.7670114814837,4.57869298264017));
#46818=CARTESIAN_POINT('Ctrl Pts',(17.8681487343997,14.7485990793917,4.67369153702113));
#46819=CARTESIAN_POINT('Ctrl Pts',(17.8633275572532,14.7435870859692,4.69955085332978));
#46820=CARTESIAN_POINT('Ctrl Pts',(17.8583668179424,14.738761572283,4.72544651760255));
#46821=CARTESIAN_POINT('Ctrl Pts',(17.8532654706195,14.7341229139912,4.7513784911553));
#46822=CARTESIAN_POINT('Ctrl Pts',(17.8443802227101,14.7260435525441,4.79654538515573));
#46823=CARTESIAN_POINT('Ctrl Pts',(17.8350684710653,14.718530907793,4.8418224347108));
#46824=CARTESIAN_POINT('Ctrl Pts',(17.8253246718829,14.71158690184,4.88720951203339));
#46825=CARTESIAN_POINT('Ctrl Pts',(17.8204527722917,14.7081148988635,4.90990305069469));
#46826=CARTESIAN_POINT('Ctrl Pts',(17.8154728604565,14.704785055436,4.93262409639065));
#46827=CARTESIAN_POINT('Ctrl Pts',(17.8103841833282,14.7015977386771,4.95537266126419));
#46828=CARTESIAN_POINT('Ctrl Pts',(17.8100602652887,14.7013948510955,4.95682071354793));
#46829=CARTESIAN_POINT('Ctrl Pts',(17.8097359181445,14.7011925479494,4.95826882593874));
#46830=CARTESIAN_POINT('Ctrl Pts',(17.8094111397357,14.7009908278893,4.95971700764907));
#46831=CARTESIAN_POINT('Ctrl Pts',(17.8071848214802,14.6996080603154,4.96964412500633));
#46832=CARTESIAN_POINT('Ctrl Pts',(17.8049374293926,14.6982522836604,4.97957790799021));
#46833=CARTESIAN_POINT('Ctrl Pts',(17.8026694530977,14.6969237531007,4.98951614577323));
#46834=CARTESIAN_POINT('Ctrl Pts',(17.8000706212612,14.6954014146521,5.00090418752978));
#46835=CARTESIAN_POINT('Ctrl Pts',(17.7974433294583,14.6939141022485,5.01230419126638));
#46836=CARTESIAN_POINT('Ctrl Pts',(17.7947921859334,14.6924644235442,5.02369591713228));
#46837=CARTESIAN_POINT('Ctrl Pts',(17.7941791730066,14.6921292203472,5.02632997867901));
#46838=CARTESIAN_POINT('Ctrl Pts',(17.7935648422523,14.6917960048101,5.02896378380818));
#46839=CARTESIAN_POINT('Ctrl Pts',(17.7929492152684,14.6914647890424,5.03159723664596));
#46840=CARTESIAN_POINT('Ctrl Pts',(17.7873483284016,14.6884514350272,5.05555601655535));
#46841=CARTESIAN_POINT('Ctrl Pts',(17.7816424538296,14.6856043845632,5.07947678558384));
#46842=CARTESIAN_POINT('Ctrl Pts',(17.7758323461943,14.6829213594339,5.1033604314301));
#46843=CARTESIAN_POINT('Ctrl Pts',(17.7642105485492,14.6775545784573,5.15113422779961));
#46844=CARTESIAN_POINT('Ctrl Pts',(17.7521717712571,14.6728439394171,5.19875951427955));
#46845=CARTESIAN_POINT('Ctrl Pts',(17.7397212214228,14.6687729664596,5.24624310344624));
#46846=CARTESIAN_POINT('Ctrl Pts',(17.7354095133055,14.6673631614807,5.26268698581072));
#46847=CARTESIAN_POINT('Ctrl Pts',(17.7310484383225,14.6660300309743,5.27911388004275));
#46848=CARTESIAN_POINT('Ctrl Pts',(17.7266381601075,14.6647730057,5.29552405089601));
#46849=CARTESIAN_POINT('Ctrl Pts',(17.7055762871139,14.658769913517,5.37389301481793));
#46850=CARTESIAN_POINT('Ctrl Pts',(17.6833946055873,14.6545023082244,5.45187298840078));
#46851=CARTESIAN_POINT('Ctrl Pts',(17.6601166503744,14.6519096363622,5.52947233599578));
#46852=CARTESIAN_POINT('Ctrl Pts',(17.6566350859603,14.6515218637245,5.54107847256024));
#46853=CARTESIAN_POINT('Ctrl Pts',(17.6531289967112,14.6511715627669,5.55267609381828));
#46854=CARTESIAN_POINT('Ctrl Pts',(17.6495984426794,14.650858573625,5.56426522108234));
#46855=CARTESIAN_POINT('Ctrl Pts',(17.6245782873355,14.6486404976851,5.64639447383985));
#46856=CARTESIAN_POINT('Ctrl Pts',(17.5983297977291,14.6482953236228,5.72809730835287));
#46857=CARTESIAN_POINT('Ctrl Pts',(17.570874188347,14.6497664199344,5.80938132211805));
#46858=CARTESIAN_POINT('Ctrl Pts',(17.5685523256427,14.6498908274321,5.81625533891355));
#46859=CARTESIAN_POINT('Ctrl Pts',(17.5662218403192,14.650028201591,5.82312636385389));
#46860=CARTESIAN_POINT('Ctrl Pts',(17.5638827400639,14.6501785196801,5.82999439969799));
#46861=CARTESIAN_POINT('Ctrl Pts',(17.5038856589009,14.6540341246598,6.00615705156473));
#46862=CARTESIAN_POINT('Ctrl Pts',(17.4382229946775,14.6663995345244,6.18035414179747));
#46863=CARTESIAN_POINT('Ctrl Pts',(17.3670255340948,14.686885583319,6.35263285243815));
#46864=CARTESIAN_POINT('Ctrl Pts',(17.3660868151046,14.6871556862536,6.35490429998657));
#46865=CARTESIAN_POINT('Ctrl Pts',(17.3651471338108,14.6874272011641,6.35717541405588));
#46866=CARTESIAN_POINT('Ctrl Pts',(17.3642064905221,14.6877001271357,6.35944619474937));
#46867=CARTESIAN_POINT('Ctrl Pts',(17.3473112813971,14.6926022419129,6.40023244725639));
#46868=CARTESIAN_POINT('Ctrl Pts',(17.3301052356159,14.6979606564321,6.44091098042997));
#46869=CARTESIAN_POINT('Ctrl Pts',(17.3125892792668,14.7037719520379,6.4814821016378));
#46870=CARTESIAN_POINT('Ctrl Pts',(17.3106500215433,14.7044153425364,6.48597388379275));
#46871=CARTESIAN_POINT('Ctrl Pts',(17.3087068447073,14.7050643246938,6.49046462743921));
#46872=CARTESIAN_POINT('Ctrl Pts',(17.3067598265897,14.7057188695631,6.49495415327635));
#46873=CARTESIAN_POINT('Ctrl Pts',(17.2994242664377,14.7081849243048,6.51186883246479));
#46874=CARTESIAN_POINT('Ctrl Pts',(17.2920351878217,14.7107297252115,6.52876361629531));
#46875=CARTESIAN_POINT('Ctrl Pts',(17.2846071230498,14.7133476118522,6.54560651341641));
#46876=CARTESIAN_POINT('Ctrl Pts',(17.2821447655724,14.7142154250636,6.55118982952103));
#46877=CARTESIAN_POINT('Ctrl Pts',(17.2796776634466,14.7150914327112,6.55676849028774));
#46878=CARTESIAN_POINT('Ctrl Pts',(17.2772062480082,14.7159754625462,6.56234155089384));
#46879=CARTESIAN_POINT('Ctrl Pts',(17.2702434505644,14.7184660679616,6.57804271207401));
#46880=CARTESIAN_POINT('Ctrl Pts',(17.2632433558177,14.7210213662988,6.59370650751666));
#46881=CARTESIAN_POINT('Ctrl Pts',(17.2562075816311,14.7236401478524,6.60933047448542));
#46882=CARTESIAN_POINT('Ctrl Pts',(17.2532097516256,14.724755968473,6.61598759504413));
#46883=CARTESIAN_POINT('Ctrl Pts',(17.2502053634654,14.725883353374,6.62263765588774));
#46884=CARTESIAN_POINT('Ctrl Pts',(17.2471944427328,14.7270222483695,6.62928068697227));
#46885=CARTESIAN_POINT('Ctrl Pts',(17.2119064798966,14.7403700870687,6.7071369491747));
#46886=CARTESIAN_POINT('Ctrl Pts',(17.1757218111607,14.7552975107985,6.78402829646679));
#46887=CARTESIAN_POINT('Ctrl Pts',(17.1386772777326,14.7717276730342,6.85999798429434));
#46888=CARTESIAN_POINT('Ctrl Pts',(17.1333754037566,14.7740791846209,6.87087088978365));
#46889=CARTESIAN_POINT('Ctrl Pts',(17.1280559071385,14.7764615087316,6.8817249071209));
#46890=CARTESIAN_POINT('Ctrl Pts',(17.1227188965086,14.7788744200072,6.8925601603357));
#46891=CARTESIAN_POINT('Ctrl Pts',(17.0471123438152,14.8130568333759,7.04605735191772));
#46892=CARTESIAN_POINT('Ctrl Pts',(16.9679967584232,14.8533638693528,7.19579527946855));
#46893=CARTESIAN_POINT('Ctrl Pts',(16.8856109571811,14.8993231905961,7.342046713768));
#46894=CARTESIAN_POINT('Ctrl Pts',(16.8749530043552,14.9052687815881,7.36096673231486));
#46895=CARTESIAN_POINT('Ctrl Pts',(16.8642402649882,14.9113091728742,7.37982832651959));
#46896=CARTESIAN_POINT('Ctrl Pts',(16.8534732588058,14.9174433438549,7.3986320679054));
#46897=CARTESIAN_POINT('Ctrl Pts',(16.7751364249307,14.9620733482351,7.53544127375318));
#46898=CARTESIAN_POINT('Ctrl Pts',(16.6939260422893,15.0116699463912,7.66918665661123));
#46899=CARTESIAN_POINT('Ctrl Pts',(16.6099844685074,15.0659826559846,7.80002155565286));
#46900=CARTESIAN_POINT('Ctrl Pts',(16.5930199143405,15.0769592300746,7.82646322968525));
#46901=CARTESIAN_POINT('Ctrl Pts',(16.5759431813926,15.0881292937242,7.85278656828423));
#46902=CARTESIAN_POINT('Ctrl Pts',(16.558756936468,15.099489782043,7.87899055063023));
#46903=CARTESIAN_POINT('Ctrl Pts',(16.5517615237535,15.1041139046932,7.88965650308689));
#46904=CARTESIAN_POINT('Ctrl Pts',(16.5447473800273,15.1087700325058,7.90030346917402));
#46905=CARTESIAN_POINT('Ctrl Pts',(16.5377151519886,15.1134576667111,7.91093065893069));
#46906=CARTESIAN_POINT('Ctrl Pts',(16.5255606917866,15.1215597451814,7.92929862911696));
#46907=CARTESIAN_POINT('Ctrl Pts',(16.5133516708353,15.1297562440715,7.94760839472119));
#46908=CARTESIAN_POINT('Ctrl Pts',(16.5010884079715,15.1380466877915,7.96586027627348));
#46909=CARTESIAN_POINT('Ctrl Pts',(16.4944989617198,15.1425014103154,7.97566760029621));
#46910=CARTESIAN_POINT('Ctrl Pts',(16.4878941994145,15.1469830271346,7.98545769044203));
#46911=CARTESIAN_POINT('Ctrl Pts',(16.4812751499307,15.1514907998686,7.99522914710671));
#46912=CARTESIAN_POINT('Ctrl Pts',(16.4755758435728,15.1553721997383,8.00364282118959));
#46913=CARTESIAN_POINT('Ctrl Pts',(16.4698677621575,15.1592717459216,8.01204001683089));
#46914=CARTESIAN_POINT('Ctrl Pts',(16.4641513393775,15.1631890857729,8.02042025617386));
#46915=CARTESIAN_POINT('Ctrl Pts',(16.4437117286727,15.177195905184,8.05038459512734));
#46916=CARTESIAN_POINT('Ctrl Pts',(16.4231596967393,15.1914341799859,8.08014062779508));
#46917=CARTESIAN_POINT('Ctrl Pts',(16.4024974398753,15.2058999341082,8.10969210477789));
#46918=CARTESIAN_POINT('Ctrl Pts',(16.3731999518779,15.2264112587209,8.1515938218994));
#46919=CARTESIAN_POINT('Ctrl Pts',(16.3436809381474,15.2473796884686,8.19308445418479));
#46920=CARTESIAN_POINT('Ctrl Pts',(16.3139460336245,15.2687956713135,8.23417339797329));
#46921=CARTESIAN_POINT('Ctrl Pts',(16.2899592323926,15.2860716952971,8.26731937046929));
#46922=CARTESIAN_POINT('Ctrl Pts',(16.2658319325667,15.3036390269857,8.30020390682567));
#46923=CARTESIAN_POINT('Ctrl Pts',(16.2415670965676,15.3214927217308,8.33283183165488));
#46924=CARTESIAN_POINT('Ctrl Pts',(16.2145385429846,15.3413799175515,8.36917601360532));
#46925=CARTESIAN_POINT('Ctrl Pts',(16.1873393276794,15.361622446644,8.40520178115493));
#46926=CARTESIAN_POINT('Ctrl Pts',(16.159973040911,15.3822149926241,8.44091470888462));
#46927=CARTESIAN_POINT('Ctrl Pts',(16.1340058798433,15.4017547264134,8.47480178148602));
#46928=CARTESIAN_POINT('Ctrl Pts',(16.1078883340152,15.4216092771505,8.50840736974749));
#46929=CARTESIAN_POINT('Ctrl Pts',(16.0816234182085,15.4417746145561,8.54173588342655));
#46930=CARTESIAN_POINT('Ctrl Pts',(16.0798486235869,15.4431372434193,8.54398798532766));
#46931=CARTESIAN_POINT('Ctrl Pts',(16.0780731561048,15.4445012909336,8.54623882233379));
#46932=CARTESIAN_POINT('Ctrl Pts',(16.0762970167215,15.4458667556287,8.54848839592704));
#46933=CARTESIAN_POINT('Ctrl Pts',(16.0649307477388,15.454604943159,8.56288437115155));
#46934=CARTESIAN_POINT('Ctrl Pts',(16.0535369512196,15.4634012045553,8.57722858040296));
#46935=CARTESIAN_POINT('Ctrl Pts',(16.0421158599722,15.472255213642,8.59152137068278));
#46936=CARTESIAN_POINT('Ctrl Pts',(16.0395193741824,15.4742680956231,8.59477071227845));
#46937=CARTESIAN_POINT('Ctrl Pts',(16.0369214123754,15.4762840129575,8.59801747797031));
#46938=CARTESIAN_POINT('Ctrl Pts',(16.0343220133108,15.478302934371,8.60126162608156));
#46939=CARTESIAN_POINT('Ctrl Pts',(16.0237007979998,15.4865523022038,8.61451730354146));
#46940=CARTESIAN_POINT('Ctrl Pts',(16.0130541971412,15.4948529430825,8.62773092316722));
#46941=CARTESIAN_POINT('Ctrl Pts',(16.0023948674495,15.5031947937513,8.64088751525607));
#46942=CARTESIAN_POINT('Ctrl Pts',(15.998966260682,15.5058779761355,8.645119374292));
#46943=CARTESIAN_POINT('Ctrl Pts',(15.9955361555857,15.5085655671632,8.649345555432));
#46944=CARTESIAN_POINT('Ctrl Pts',(15.9921048908792,15.5112572959462,8.65356566263564));
#46945=CARTESIAN_POINT('Ctrl Pts',(15.963891155855,15.5333901621449,8.68826569210053));
#46946=CARTESIAN_POINT('Ctrl Pts',(15.9355795517899,15.5558177771029,8.72257963369553));
#46947=CARTESIAN_POINT('Ctrl Pts',(15.9071741212286,15.5785326177975,8.75651763111319));
#46948=CARTESIAN_POINT('Ctrl Pts',(15.8320856427827,15.6385782778068,8.84623120127341));
#46949=CARTESIAN_POINT('Ctrl Pts',(15.7563428898215,15.7006252473126,8.93332397978106));
#46950=CARTESIAN_POINT('Ctrl Pts',(15.6800121405069,15.7645675407892,9.01794758228341));
#46951=CARTESIAN_POINT('Ctrl Pts',(15.6406445808878,15.7975457582603,9.06159217828978));
#46952=CARTESIAN_POINT('Ctrl Pts',(15.6011197257036,15.8310304240877,9.10457977539739));
#46953=CARTESIAN_POINT('Ctrl Pts',(15.5614458176104,15.8650078553951,9.1469317593497));
#46954=CARTESIAN_POINT('Ctrl Pts',(15.4915558576705,15.9248628439017,9.22153944495621));
#46955=CARTESIAN_POINT('Ctrl Pts',(15.4212030312285,15.9862476883049,9.29417371478342));
#46956=CARTESIAN_POINT('Ctrl Pts',(15.3504255247275,16.0491202511077,9.36491710445505));
#46957=CARTESIAN_POINT('Ctrl Pts',(15.3028155108123,16.0914128344143,9.41250416895029));
#46958=CARTESIAN_POINT('Ctrl Pts',(15.2550134038353,16.1343797974888,9.45923461112119));
#46959=CARTESIAN_POINT('Ctrl Pts',(15.2070311136134,16.1780085379062,9.50513258392003));
#46960=CARTESIAN_POINT('Ctrl Pts',(15.1431905716113,16.2360566723789,9.56619993703555));
#46961=CARTESIAN_POINT('Ctrl Pts',(15.0790308535853,16.2952765226413,9.62579322207588));
#46962=CARTESIAN_POINT('Ctrl Pts',(15.0145773289901,16.35565810712,9.6839498613404));
#46963=CARTESIAN_POINT('Ctrl Pts',(14.9582797762188,16.4083989845189,9.73474733888037));
#46964=CARTESIAN_POINT('Ctrl Pts',(14.9017581147026,16.4620266993466,9.78444830855335));
#46965=CARTESIAN_POINT('Ctrl Pts',(14.8450296295046,16.51653473843,9.83307664083576));
#46966=CARTESIAN_POINT('Ctrl Pts',(14.7879974125538,16.5713346207062,9.88196533558943));
#46967=CARTESIAN_POINT('Ctrl Pts',(14.7307560003233,16.6270242276471,9.92976976812893));
#46968=CARTESIAN_POINT('Ctrl Pts',(14.673322350996,16.6836096033916,9.97650269153596));
#46969=CARTESIAN_POINT('Ctrl Pts',(14.6079377474624,16.7480285007138,10.0297051905017));
#46970=CARTESIAN_POINT('Ctrl Pts',(14.542303948576,16.8136074931285,10.0815196120906));
#46971=CARTESIAN_POINT('Ctrl Pts',(14.4764465245309,16.8803555924736,10.1319634598115));
#46972=CARTESIAN_POINT('Ctrl Pts',(14.4269140830284,16.930557925379,10.1699030994592));
#46973=CARTESIAN_POINT('Ctrl Pts',(14.3772551335397,16.9814228338856,10.2070663578355));
#46974=CARTESIAN_POINT('Ctrl Pts',(14.3274807199144,17.0329603662361,10.2434554339001));
#46975=CARTESIAN_POINT('Ctrl Pts',(14.314990397583,17.0458931231355,10.2525868581859));
#46976=CARTESIAN_POINT('Ctrl Pts',(14.3024946467154,17.05886631397,10.2616681973105));
#46977=CARTESIAN_POINT('Ctrl Pts',(14.2899914513039,17.07188234669,10.2707011041516));
#46978=CARTESIAN_POINT('Ctrl Pts',(14.2734763801558,17.0890748082458,10.2826323820567));
#46979=CARTESIAN_POINT('Ctrl Pts',(14.2569416682199,17.1063491334474,10.2944837091251));
#46980=CARTESIAN_POINT('Ctrl Pts',(14.2404003000471,17.1236924326205,10.3062463900494));
#46981=CARTESIAN_POINT('Ctrl Pts',(14.2257017395037,17.1391035842408,10.3166986377662));
#46982=CARTESIAN_POINT('Ctrl Pts',(14.2110064088285,17.1545603076558,10.3270748478657));
#46983=CARTESIAN_POINT('Ctrl Pts',(14.1963246412405,17.170052197827,10.3373681732381));
#46984=CARTESIAN_POINT('Ctrl Pts',(14.181975142211,17.1851934852533,10.3474285465246));
#46985=CARTESIAN_POINT('Ctrl Pts',(14.1676354439626,17.2003715773109,10.3574121351433));
#46986=CARTESIAN_POINT('Ctrl Pts',(14.1533036570002,17.2155887738345,10.3673208975942));
#46987=CARTESIAN_POINT('Ctrl Pts',(14.1364434248707,17.2334906214145,10.3789777855647));
#46988=CARTESIAN_POINT('Ctrl Pts',(14.1195959115965,17.2514448030669,10.3905298278396));
#46989=CARTESIAN_POINT('Ctrl Pts',(14.102761535583,17.2694513331259,10.4019778023782));
#46990=CARTESIAN_POINT('Ctrl Pts',(14.0616939791491,17.3133783660484,10.4299052016498));
#46991=CARTESIAN_POINT('Ctrl Pts',(14.0207043099312,17.357616068478,10.4572145106538));
#46992=CARTESIAN_POINT('Ctrl Pts',(13.9797992920512,17.4021669272979,10.4839136631712));
#46993=CARTESIAN_POINT('Ctrl Pts',(13.8963730378755,17.4930289159798,10.5383668916413));
#46994=CARTESIAN_POINT('Ctrl Pts',(13.8132979186715,17.5851917329795,10.5902846035054));
#46995=CARTESIAN_POINT('Ctrl Pts',(13.7306345084654,17.6786798143199,10.6397262633505));
#46996=CARTESIAN_POINT('Ctrl Pts',(13.6990070978718,17.7144487951397,10.658642875579));
#46997=CARTESIAN_POINT('Ctrl Pts',(13.6674398860713,17.7504117000158,10.6771970283303));
#46998=CARTESIAN_POINT('Ctrl Pts',(13.6359369836638,17.7865716688882,10.6953896284376));
#46999=CARTESIAN_POINT('Ctrl Pts',(13.5443304572451,17.8917203660138,10.7482914493811));
#47000=CARTESIAN_POINT('Ctrl Pts',(13.4532652978713,17.9985304127055,10.7981423054322));
#47001=CARTESIAN_POINT('Ctrl Pts',(13.362843952931,18.1070757677516,10.8449629340514));
#47002=CARTESIAN_POINT('Ctrl Pts',(13.3408972516745,18.133421455062,10.8563270466912));
#47003=CARTESIAN_POINT('Ctrl Pts',(13.3189884250314,18.1598692890699,10.8675126974676));
#47004=CARTESIAN_POINT('Ctrl Pts',(13.2971192937982,18.1864210638634,10.8785192895612));
#47005=CARTESIAN_POINT('Ctrl Pts',(13.1974886473656,18.3073847390275,10.9286627485591));
#47006=CARTESIAN_POINT('Ctrl Pts',(13.0986789283229,18.4304994909325,10.9750973239262));
#47007=CARTESIAN_POINT('Ctrl Pts',(13.0008637679413,18.555928374369,11.0177665156938));
#47008=CARTESIAN_POINT('Ctrl Pts',(12.9887483958524,18.5714639783347,11.0230515158204));
#47009=CARTESIAN_POINT('Ctrl Pts',(12.9766482540743,18.5870350362773,11.0282787901708));
#47010=CARTESIAN_POINT('Ctrl Pts',(12.9645637645202,18.6026420312121,11.0334480392572));
#47011=CARTESIAN_POINT('Ctrl Pts',(12.8572271761536,18.7412661396995,11.0793622302421));
#47012=CARTESIAN_POINT('Ctrl Pts',(12.7511223420231,18.8827189620378,11.1207063336849));
#47013=CARTESIAN_POINT('Ctrl Pts',(12.6465462824545,19.0273228911961,11.1572752841488));
#47014=CARTESIAN_POINT('Ctrl Pts',(12.644292060807,19.0304399459864,11.1580635574889));
#47015=CARTESIAN_POINT('Ctrl Pts',(12.6420385516737,19.0335584688927,11.1588496076951));
#47016=CARTESIAN_POINT('Ctrl Pts',(12.6397857586885,19.0366784643387,11.1596334314464));
#47017=CARTESIAN_POINT('Ctrl Pts',(12.5836913769038,19.1143661244414,11.1791505859489));
#47018=CARTESIAN_POINT('Ctrl Pts',(12.5281517057416,19.1928079324649,11.1972529590116));
#47019=CARTESIAN_POINT('Ctrl Pts',(12.4729858003008,19.2724054736595,11.2139668936264));
#47020=CARTESIAN_POINT('Ctrl Pts',(12.4443163748122,19.313771889349,11.2226530358955));
#47021=CARTESIAN_POINT('Ctrl Pts',(12.4157289692281,19.3554805340295,11.2309679359619));
#47022=CARTESIAN_POINT('Ctrl Pts',(12.3873311427962,19.39739837676,11.2388739303386));
#47023=CARTESIAN_POINT('Ctrl Pts',(12.3663714964643,19.428336771314,11.2447091250298));
#47024=CARTESIAN_POINT('Ctrl Pts',(12.3455020862917,19.4594076778139,11.2503257124173));
#47025=CARTESIAN_POINT('Ctrl Pts',(12.3247145835032,19.4906334206159,11.2557233274532));
#47026=CARTESIAN_POINT('Origin',(6.61325378140121E-15,19.4906334205523,
8.67361737988404E-16));
#47027=CARTESIAN_POINT('Origin',(3.30643715532042E-15,11.4559962546824,
4.33680868994202E-16));
#47028=CARTESIAN_POINT('',(9.18375896983081E-16,11.4559962546824,19.5));
#47029=CARTESIAN_POINT('Origin',(0.,11.4559962546824,0.));
#47030=CARTESIAN_POINT('Origin',(1.28576993672729E-15,11.4559962546824,
16.5));
#47031=CARTESIAN_POINT('Origin',(6.61363325216158E-15,52.,8.67361737988404E-16));
#47032=CARTESIAN_POINT('',(-4.71428571428571,51.,-15.8121949837485));
#47033=CARTESIAN_POINT('',(8.63430047075471E-15,51.,16.5));
#47034=CARTESIAN_POINT('Origin',(6.61363325216158E-15,51.,8.67361737988404E-16));
#47035=CARTESIAN_POINT('',(8.63430047075471E-15,20.5439967627459,16.5));
#47036=CARTESIAN_POINT('',(8.63430047075471E-15,52.,16.5));
#47037=CARTESIAN_POINT('',(12.0252610002882,20.5440037453176,11.2979244951432));
#47038=CARTESIAN_POINT('Origin',(6.61363325216158E-15,20.5440037453176,
8.67361737988404E-16));
#47039=CARTESIAN_POINT('',(15.4998953469709,26.9999999999978,5.65714310527842));
#47040=CARTESIAN_POINT('Ctrl Pts',(12.0252610013046,20.5440037453176,11.2979244960981));
#47041=CARTESIAN_POINT('Ctrl Pts',(12.0249308728691,20.548893260366,11.2982758756345));
#47042=CARTESIAN_POINT('Ctrl Pts',(12.0246060118186,20.5537834284514,11.2986216185138));
#47043=CARTESIAN_POINT('Ctrl Pts',(12.024286421815,20.5586742495714,11.298961724254));
#47044=CARTESIAN_POINT('Ctrl Pts',(12.0228356969254,20.5808753067053,11.3005055768679));
#47045=CARTESIAN_POINT('Ctrl Pts',(12.0214935973948,20.6030898283043,11.3019332419997));
#47046=CARTESIAN_POINT('Ctrl Pts',(12.0202605030161,20.6253178445758,11.3032445556378));
#47047=CARTESIAN_POINT('Ctrl Pts',(12.0196817441633,20.6357506722801,11.3038600270809));
#47048=CARTESIAN_POINT('Ctrl Pts',(12.0191271097146,20.6461843806063,11.3044497486797));
#47049=CARTESIAN_POINT('Ctrl Pts',(12.0185964357884,20.656622724066,11.3050139192154));
#47050=CARTESIAN_POINT('Ctrl Pts',(12.0177638774852,20.6729991260151,11.3058990293379));
#47051=CARTESIAN_POINT('Ctrl Pts',(12.0169903907423,20.6893867131252,11.3067211441569));
#47052=CARTESIAN_POINT('Ctrl Pts',(12.0162772436363,20.7057571332248,11.3074789941909));
#47053=CARTESIAN_POINT('Ctrl Pts',(12.0162631181461,20.7060813863941,11.3074940051237));
#47054=CARTESIAN_POINT('Ctrl Pts',(12.0162490161176,20.706405637056,11.307508991068));
#47055=CARTESIAN_POINT('Ctrl Pts',(12.0162349375449,20.7067298853232,11.3075239520309));
#47056=CARTESIAN_POINT('Ctrl Pts',(12.0155382159022,20.7227763120345,11.3082643414754));
#47057=CARTESIAN_POINT('Ctrl Pts',(12.0148990649862,20.738814572496,11.3089434156603));
#47058=CARTESIAN_POINT('Ctrl Pts',(12.0143172936214,20.7548446975429,11.3095614401351));
#47059=CARTESIAN_POINT('Ctrl Pts',(12.0129319285457,20.7930170393609,11.3110331343007));
#47060=CARTESIAN_POINT('Ctrl Pts',(12.0118718817328,20.8311432832627,11.3121590426822));
#47061=CARTESIAN_POINT('Ctrl Pts',(12.0111346855915,20.8692237895445,11.3129419381104));
#47062=CARTESIAN_POINT('Ctrl Pts',(12.0093466729179,20.9615851355062,11.3148407908979));
#47063=CARTESIAN_POINT('Ctrl Pts',(12.0094576599568,21.0536774553069,11.3147220486198));
#47064=CARTESIAN_POINT('Ctrl Pts',(12.01143572497,21.1455054304304,11.3126217927108));
#47065=CARTESIAN_POINT('Ctrl Pts',(12.0117737384095,21.1611970732783,11.3122628991866));
#47066=CARTESIAN_POINT('Ctrl Pts',(12.0121662715151,21.1768809958035,11.3118461408723));
#47067=CARTESIAN_POINT('Ctrl Pts',(12.0126131765915,21.1925572116773,11.3113716032014));
#47068=CARTESIAN_POINT('Ctrl Pts',(12.0156753838789,21.2999711235487,11.3081200565288));
#47069=CARTESIAN_POINT('Ctrl Pts',(12.0212890769295,21.4070235554608,11.3021571360844));
#47070=CARTESIAN_POINT('Ctrl Pts',(12.029405224626,21.5137197802307,11.293511875714));
#47071=CARTESIAN_POINT('Ctrl Pts',(12.0298842581913,21.5200172349913,11.2930016127108));
#47072=CARTESIAN_POINT('Ctrl Pts',(12.0303720112037,21.526313448837,11.292482003453));
#47073=CARTESIAN_POINT('Ctrl Pts',(12.0308684730983,21.5326084229108,11.2919530544105));
#47074=CARTESIAN_POINT('Ctrl Pts',(12.038783442791,21.6329676439405,11.2835201501216));
#47075=CARTESIAN_POINT('Ctrl Pts',(12.0489119741868,21.7330116990756,11.2727132659417));
#47076=CARTESIAN_POINT('Ctrl Pts',(12.0612142372056,21.8327433602281,11.2595345438906));
#47077=CARTESIAN_POINT('Ctrl Pts',(12.0646499496549,21.8605959032351,11.2558540584914));
#47078=CARTESIAN_POINT('Ctrl Pts',(12.0682552832817,21.8884240721786,11.2519884939938));
#47079=CARTESIAN_POINT('Ctrl Pts',(12.0720293911064,21.9162279265017,11.2479378723508));
#47080=CARTESIAN_POINT('Ctrl Pts',(12.0806670632113,21.9798616614262,11.2386673524827));
#47081=CARTESIAN_POINT('Ctrl Pts',(12.0901888787009,22.0433679653625,11.2284267261222));
#47082=CARTESIAN_POINT('Ctrl Pts',(12.1005853276592,22.1067471382375,11.217211539774));
#47083=CARTESIAN_POINT('Ctrl Pts',(12.1029321776561,22.1210540821047,11.2146798714946));
#47084=CARTESIAN_POINT('Ctrl Pts',(12.1053235973978,22.1353545469586,11.2120985328033));
#47085=CARTESIAN_POINT('Ctrl Pts',(12.1077594815789,22.1496485338453,11.2094674447032));
#47086=CARTESIAN_POINT('Ctrl Pts',(12.1107170104573,22.1670035786097,11.2062729089786));
#47087=CARTESIAN_POINT('Ctrl Pts',(12.1137401289893,22.1843493271757,11.2030049893633));
#47088=CARTESIAN_POINT('Ctrl Pts',(12.1168286615825,22.2016858050301,11.1996635300287));
#47089=CARTESIAN_POINT('Ctrl Pts',(12.1184242270949,22.2106419954981,11.1979373001397));
#47090=CARTESIAN_POINT('Ctrl Pts',(12.1200374772146,22.219596819521,11.1961911962994));
#47091=CARTESIAN_POINT('Ctrl Pts',(12.1216670572837,22.2285432875991,11.1944266373505));
#47092=CARTESIAN_POINT('Ctrl Pts',(12.1229129709795,22.235383409983,11.1930775240402));
#47093=CARTESIAN_POINT('Ctrl Pts',(12.1241684933701,22.2422189946054,11.191717554553));
#47094=CARTESIAN_POINT('Ctrl Pts',(12.1254330313338,22.2490469590199,11.1903473495079));
#47095=CARTESIAN_POINT('Ctrl Pts',(12.1283503922125,22.2647994605947,11.187186208673));
#47096=CARTESIAN_POINT('Ctrl Pts',(12.1313172199455,22.2805198972878,11.1839689876802));
#47097=CARTESIAN_POINT('Ctrl Pts',(12.1343330639684,22.2962091557006,11.1806959127187));
#47098=CARTESIAN_POINT('Ctrl Pts',(12.1350293696224,22.2998315311472,11.1799402169387));
#47099=CARTESIAN_POINT('Ctrl Pts',(12.1357282849766,22.303452247295,11.1791815485227));
#47100=CARTESIAN_POINT('Ctrl Pts',(12.136429805251,22.3070713144085,11.178419909148));
#47101=CARTESIAN_POINT('Ctrl Pts',(12.1465437361255,22.3592479883444,11.1674392315131));
#47102=CARTESIAN_POINT('Ctrl Pts',(12.1571983969572,22.411075698049,11.1558418062304));
#47103=CARTESIAN_POINT('Ctrl Pts',(12.1683725405619,22.4625644347832,11.1436401560417));
#47104=CARTESIAN_POINT('Ctrl Pts',(12.1832259279363,22.5310065614632,11.1274209411048));
#47105=CARTESIAN_POINT('Ctrl Pts',(12.1989982808949,22.5988489749547,11.1101329448993));
#47106=CARTESIAN_POINT('Ctrl Pts',(12.2156434245513,22.6661129579501,11.0918012840217));
#47107=CARTESIAN_POINT('Ctrl Pts',(12.2240424301989,22.7000538229085,11.0825512753454));
#47108=CARTESIAN_POINT('Ctrl Pts',(12.2326636902816,22.7338473804668,11.0730354852607));
#47109=CARTESIAN_POINT('Ctrl Pts',(12.2415021288752,22.7674955939997,11.0632558073106));
#47110=CARTESIAN_POINT('Ctrl Pts',(12.2641668096522,22.8537807461063,11.0381774774118));
#47111=CARTESIAN_POINT('Ctrl Pts',(12.2882575055527,22.9391117544965,11.0113662686165));
#47112=CARTESIAN_POINT('Ctrl Pts',(12.3136878264858,23.0235234978828,10.9828544610159));
#47113=CARTESIAN_POINT('Ctrl Pts',(12.3178278371292,23.0372655783292,10.9782127898692));
#47114=CARTESIAN_POINT('Ctrl Pts',(12.3220033536933,23.0509832918754,10.9735260433554));
#47115=CARTESIAN_POINT('Ctrl Pts',(12.3262140559314,23.0646767404433,10.9687942764753));
#47116=CARTESIAN_POINT('Ctrl Pts',(12.3562893074409,23.162483207494,10.9349972823026));
#47117=CARTESIAN_POINT('Ctrl Pts',(12.3881579513823,23.259053126514,10.8989055023022));
#47118=CARTESIAN_POINT('Ctrl Pts',(12.4217002577817,23.3544275618513,10.8605415533984));
#47119=CARTESIAN_POINT('Ctrl Pts',(12.4234325753308,23.3593532460336,10.8585602185091));
#47120=CARTESIAN_POINT('Ctrl Pts',(12.4251693574216,23.3642757416104,10.8565728222644));
#47121=CARTESIAN_POINT('Ctrl Pts',(12.4269105870875,23.3691950546363,10.854579368199));
#47122=CARTESIAN_POINT('Ctrl Pts',(12.4420267918443,23.411901277955,10.8372735179623));
#47123=CARTESIAN_POINT('Ctrl Pts',(12.4574784902714,23.4543673858017,10.8195106603123));
#47124=CARTESIAN_POINT('Ctrl Pts',(12.4732557741443,23.4965962769449,10.8012911523043));
#47125=CARTESIAN_POINT('Ctrl Pts',(12.4783984540648,23.5103609827268,10.7953524179347));
#47126=CARTESIAN_POINT('Ctrl Pts',(12.4835754560386,23.5240997521511,10.7893654779865));
#47127=CARTESIAN_POINT('Ctrl Pts',(12.4887867248453,23.5378134440997,10.7833300117045));
#47128=CARTESIAN_POINT('Ctrl Pts',(12.4924901191887,23.5475590955087,10.7790409004501));
#47129=CARTESIAN_POINT('Ctrl Pts',(12.4962117800455,23.55729444906,10.774726155287));
#47130=CARTESIAN_POINT('Ctrl Pts',(12.4999498795827,23.5670152413277,10.7703877686227));
#47131=CARTESIAN_POINT('Ctrl Pts',(12.504448981637,23.5787149930396,10.7651661729537));
#47132=CARTESIAN_POINT('Ctrl Pts',(12.5089736617026,23.590398206173,10.7599082780242));
#47133=CARTESIAN_POINT('Ctrl Pts',(12.5135167964196,23.6020472903523,10.7546221314614));
#47134=CARTESIAN_POINT('Ctrl Pts',(12.5159900547159,23.6083889896161,10.7517443814812));
#47135=CARTESIAN_POINT('Ctrl Pts',(12.5184694270114,23.6147222115016,10.7488575096783));
#47136=CARTESIAN_POINT('Ctrl Pts',(12.5209543788166,23.621045733523,10.7459620994861));
#47137=CARTESIAN_POINT('Ctrl Pts',(12.523034041566,23.6263379058562,10.7435389230253));
#47138=CARTESIAN_POINT('Ctrl Pts',(12.5251178344798,23.6316238943125,10.7411095107864));
#47139=CARTESIAN_POINT('Ctrl Pts',(12.5272057361195,23.6369037580822,10.7386738679465));
#47140=CARTESIAN_POINT('Ctrl Pts',(12.5359929025913,23.6591246525012,10.7284231939234));
#47141=CARTESIAN_POINT('Ctrl Pts',(12.5448522441492,23.6812349383611,10.7180628615953));
#47142=CARTESIAN_POINT('Ctrl Pts',(12.5537816116273,23.7032364478602,10.7075939056153));
#47143=CARTESIAN_POINT('Ctrl Pts',(12.5821071150075,23.773029054472,10.6743845603033));
#47144=CARTESIAN_POINT('Ctrl Pts',(12.6111358407004,23.8417290631451,10.6400837415979));
#47145=CARTESIAN_POINT('Ctrl Pts',(12.6408066531758,23.9093846481827,10.604716206553));
#47146=CARTESIAN_POINT('Ctrl Pts',(12.6573308096376,23.9470631402563,10.5850194529426));
#47147=CARTESIAN_POINT('Ctrl Pts',(12.6740544347473,23.9844172157351,10.5649914598182));
#47148=CARTESIAN_POINT('Ctrl Pts',(12.6909669667773,24.0214553684772,10.5446364303458));
#47149=CARTESIAN_POINT('Ctrl Pts',(12.7139959188659,24.0718883754,10.5169200010344));
#47150=CARTESIAN_POINT('Ctrl Pts',(12.7373752989098,24.1217354114684,10.4885970630843));
#47151=CARTESIAN_POINT('Ctrl Pts',(12.7610828922023,24.1710115636718,10.4596731584983));
#47152=CARTESIAN_POINT('Ctrl Pts',(12.7858766861947,24.2225453803435,10.4294240597008));
#47153=CARTESIAN_POINT('Ctrl Pts',(12.8110293324431,24.2734549676925,10.3985178216957));
#47154=CARTESIAN_POINT('Ctrl Pts',(12.8365157707695,24.3237575293058,10.3669601555514));
#47155=CARTESIAN_POINT('Ctrl Pts',(12.8532965490679,24.356877737138,10.3461819600108));
#47156=CARTESIAN_POINT('Ctrl Pts',(12.8702220812317,24.3897347297404,10.3251213217501));
#47157=CARTESIAN_POINT('Ctrl Pts',(12.8872863473921,24.4223316737733,10.3037784633077));
#47158=CARTESIAN_POINT('Ctrl Pts',(12.9207515320077,24.4862584046218,10.261922417974));
#47159=CARTESIAN_POINT('Ctrl Pts',(12.9547492668051,24.5491865853333,10.218982271535));
#47160=CARTESIAN_POINT('Ctrl Pts',(12.989234150632,24.6111411057364,10.1749592716658));
#47161=CARTESIAN_POINT('Ctrl Pts',(12.9990401875224,24.6287583410343,10.1624409995176));
#47162=CARTESIAN_POINT('Ctrl Pts',(13.0088856229381,24.6462968362974,10.1498351639255));
#47163=CARTESIAN_POINT('Ctrl Pts',(13.018769570305,24.6637569001809,10.137141572148));
#47164=CARTESIAN_POINT('Ctrl Pts',(13.0612011775983,24.7387126386645,10.0826482122126));
#47165=CARTESIAN_POINT('Ctrl Pts',(13.1043412580011,24.8122250522767,10.0265393117696));
#47166=CARTESIAN_POINT('Ctrl Pts',(13.1481190796857,24.8843211741588,9.96879955994731));
#47167=CARTESIAN_POINT('Ctrl Pts',(13.150400445733,24.8880782739477,9.96579060462879));
#47168=CARTESIAN_POINT('Ctrl Pts',(13.1526835438624,24.8918315272673,9.9627772203878));
#47169=CARTESIAN_POINT('Ctrl Pts',(13.1549683655095,24.8955809352535,9.95975940265458));
#47170=CARTESIAN_POINT('Ctrl Pts',(13.2010973193871,24.9712788647993,9.89883176954819));
#47171=CARTESIAN_POINT('Ctrl Pts',(13.2479284546171,25.0454100868088,9.83609760807509));
#47172=CARTESIAN_POINT('Ctrl Pts',(13.2953897478999,25.1179881253617,9.77152044143306));
#47173=CARTESIAN_POINT('Ctrl Pts',(13.3010243543399,25.1266045927006,9.7638538378943));
#47174=CARTESIAN_POINT('Ctrl Pts',(13.3066676460292,25.1351988393214,9.75616152364732));
#47175=CARTESIAN_POINT('Ctrl Pts',(13.3123196583909,25.1437711353646,9.74844322509082));
#47176=CARTESIAN_POINT('Ctrl Pts',(13.3261977499658,25.1648197640443,9.72949152305712));
#47177=CARTESIAN_POINT('Ctrl Pts',(13.34012850467,25.1857358948461,9.71038301825754));
#47178=CARTESIAN_POINT('Ctrl Pts',(13.354112658698,25.206523063251,9.69111320224889));
#47179=CARTESIAN_POINT('Ctrl Pts',(13.3584191706195,25.2129246080545,9.68517893606442));
#47180=CARTESIAN_POINT('Ctrl Pts',(13.3627307231837,25.2193138613263,9.67922939251358));
#47181=CARTESIAN_POINT('Ctrl Pts',(13.3670465731033,25.2256898232767,9.6732655098805));
#47182=CARTESIAN_POINT('Ctrl Pts',(13.3767333995054,25.2400005239987,9.65987971175828));
#47183=CARTESIAN_POINT('Ctrl Pts',(13.3864388290379,25.254239747419,9.64642588898842));
#47184=CARTESIAN_POINT('Ctrl Pts',(13.3961546301693,25.2683965644849,9.63291446679527));
#47185=CARTESIAN_POINT('Ctrl Pts',(13.4105486129811,25.2893699231161,9.6128972622249));
#47186=CARTESIAN_POINT('Ctrl Pts',(13.4249722375238,25.3101727876637,9.5927441957544));
#47187=CARTESIAN_POINT('Ctrl Pts',(13.4394268689906,25.3308108782405,9.57245033620673));
#47188=CARTESIAN_POINT('Ctrl Pts',(13.4531522150938,25.3504077068919,9.55318037095716));
#47189=CARTESIAN_POINT('Ctrl Pts',(13.4669038118876,25.3698533742983,9.53378584359692));
#47190=CARTESIAN_POINT('Ctrl Pts',(13.4806800176673,25.3891488043011,9.51426645944222));
#47191=CARTESIAN_POINT('Ctrl Pts',(13.5155059835076,25.4379272558502,9.4649218563875));
#47192=CARTESIAN_POINT('Ctrl Pts',(13.5504889007219,25.4857465093747,9.41477989849423));
#47193=CARTESIAN_POINT('Ctrl Pts',(13.5856048493766,25.5326144032833,9.36383157029569));
#47194=CARTESIAN_POINT('Ctrl Pts',(13.6074054038267,25.5617107572836,9.33220201604527));
#47195=CARTESIAN_POINT('Ctrl Pts',(13.6292572492356,25.5904404157791,9.30026164404338));
#47196=CARTESIAN_POINT('Ctrl Pts',(13.6511549037297,25.6188047072121,9.26800786546799));
#47197=CARTESIAN_POINT('Ctrl Pts',(13.6538698198203,25.6223213702058,9.26400897588554));
#47198=CARTESIAN_POINT('Ctrl Pts',(13.6565854424971,25.6258324098416,9.2600052645616));
#47199=CARTESIAN_POINT('Ctrl Pts',(13.6593017621577,25.6293378259766,9.25599672497029));
#47200=CARTESIAN_POINT('Ctrl Pts',(13.6708601828647,25.6442539917827,9.23893967984864));
#47201=CARTESIAN_POINT('Ctrl Pts',(13.6824315688055,25.6590689268798,9.22179469795511));
#47202=CARTESIAN_POINT('Ctrl Pts',(13.694014042668,25.6737812611331,9.20456296622561));
#47203=CARTESIAN_POINT('Ctrl Pts',(13.6947698389658,25.6747412915975,9.20343853640167));
#47204=CARTESIAN_POINT('Ctrl Pts',(13.6955256987437,25.6757009054187,9.20231371272741));
#47205=CARTESIAN_POINT('Ctrl Pts',(13.6962816185107,25.6766600985106,9.20118850000519));
#47206=CARTESIAN_POINT('Ctrl Pts',(13.7086219042892,25.6923187932376,9.18281955774556));
#47207=CARTESIAN_POINT('Ctrl Pts',(13.7209791439012,25.7078665937885,9.16434550060255));
#47208=CARTESIAN_POINT('Ctrl Pts',(13.7333406641673,25.7232888198184,9.1457834092639));
#47209=CARTESIAN_POINT('Ctrl Pts',(13.7345433154336,25.7247892468908,9.14397750495978));
#47210=CARTESIAN_POINT('Ctrl Pts',(13.7357459848049,25.726288457548,9.14217080098322));
#47211=CARTESIAN_POINT('Ctrl Pts',(13.7369486596423,25.7277864371561,9.14036331457088));
#47212=CARTESIAN_POINT('Ctrl Pts',(13.7655659843295,25.7634304595377,9.09735466092379));
#47213=CARTESIAN_POINT('Ctrl Pts',(13.7941628056774,25.7983490149194,9.05393888933006));
#47214=CARTESIAN_POINT('Ctrl Pts',(13.8227306450084,25.8325548745127,9.01011195910166));
#47215=CARTESIAN_POINT('Ctrl Pts',(13.842323756366,25.8560147941913,8.98005347569739));
#47216=CARTESIAN_POINT('Ctrl Pts',(13.8619031653407,25.8791397721896,8.94980169723303));
#47217=CARTESIAN_POINT('Ctrl Pts',(13.8814664318801,25.9019324890728,8.91935478464348));
#47218=CARTESIAN_POINT('Ctrl Pts',(13.9188560303246,25.9454942598026,8.86116420418492));
#47219=CARTESIAN_POINT('Ctrl Pts',(13.9561842683538,25.9878408888805,8.80226458048654));
#47220=CARTESIAN_POINT('Ctrl Pts',(13.9934294395427,26.0289848800641,8.74265020005614));
#47221=CARTESIAN_POINT('Ctrl Pts',(14.0052802435624,26.0420762248087,8.72368187968913));
#47222=CARTESIAN_POINT('Ctrl Pts',(14.0171226430049,26.0550458029487,8.70464119597399));
#47223=CARTESIAN_POINT('Ctrl Pts',(14.028956008926,26.0678936516663,8.68552782935395));
#47224=CARTESIAN_POINT('Ctrl Pts',(14.073645714307,26.1164146369712,8.6133445867516));
#47225=CARTESIAN_POINT('Ctrl Pts',(14.1182061758798,26.1632016095437,8.54012540763018));
#47226=CARTESIAN_POINT('Ctrl Pts',(14.1626036383006,26.2082576238332,8.46585247830341));
#47227=CARTESIAN_POINT('Ctrl Pts',(14.166909323044,26.2126271752164,8.45864945810322));
#47228=CARTESIAN_POINT('Ctrl Pts',(14.171213475128,26.2169804459483,8.45143652733002));
#47229=CARTESIAN_POINT('Ctrl Pts',(14.1755160662839,26.2213174218195,8.44421366298218));
#47230=CARTESIAN_POINT('Ctrl Pts',(14.2241842207673,26.2703745141725,8.36251324917115));
#47231=CARTESIAN_POINT('Ctrl Pts',(14.2726524536592,26.3173480640962,8.27954231106037));
#47232=CARTESIAN_POINT('Ctrl Pts',(14.3208797292034,26.3622200090052,8.19526716166835));
#47233=CARTESIAN_POINT('Ctrl Pts',(14.3238709484976,26.3650031193068,8.19004013090527));
#47234=CARTESIAN_POINT('Ctrl Pts',(14.3268612416092,26.3677781409806,8.1848080812505));
#47235=CARTESIAN_POINT('Ctrl Pts',(14.329850598655,26.3705450703243,8.17957100465716));
#47236=CARTESIAN_POINT('Ctrl Pts',(14.3750584922162,26.4123892011349,8.10037096345171));
#47237=CARTESIAN_POINT('Ctrl Pts',(14.4200523911715,26.4523826410612,8.02002135269682));
#47238=CARTESIAN_POINT('Ctrl Pts',(14.4648003758821,26.490492278629,7.93848543396106));
#47239=CARTESIAN_POINT('Ctrl Pts',(14.4748141458766,26.4990205095124,7.92023920585061));
#47240=CARTESIAN_POINT('Ctrl Pts',(14.4848156256028,26.5074542835796,7.90193352052972));
#47241=CARTESIAN_POINT('Ctrl Pts',(14.4948044563928,26.5157932364357,7.88356795942912));
#47242=CARTESIAN_POINT('Ctrl Pts',(14.5324037423552,26.547182162693,7.81443754785294));
#47243=CARTESIAN_POINT('Ctrl Pts',(14.5698238573549,26.5772277118277,7.74445888208727));
#47244=CARTESIAN_POINT('Ctrl Pts',(14.6070465811387,26.6058975693601,7.67360363343441));
#47245=CARTESIAN_POINT('Ctrl Pts',(14.6237799773867,26.6187860427897,7.64175080721871));
#47246=CARTESIAN_POINT('Ctrl Pts',(14.6404735352976,26.6313962194054,7.60972072029597));
#47247=CARTESIAN_POINT('Ctrl Pts',(14.6571256324194,26.6437250310917,7.57751068593594));
#47248=CARTESIAN_POINT('Ctrl Pts',(14.6839259713877,26.663567356647,7.52567097873781));
#47249=CARTESIAN_POINT('Ctrl Pts',(14.7106189563916,26.6826802627059,7.47336488375808));
#47250=CARTESIAN_POINT('Ctrl Pts',(14.7371979544204,26.7010468771463,7.42057925314658));
#47251=CARTESIAN_POINT('Ctrl Pts',(14.740599812746,26.703397628675,7.41382319572207));
#47252=CARTESIAN_POINT('Ctrl Pts',(14.7439998038026,26.7057361517508,7.40705928125229));
#47253=CARTESIAN_POINT('Ctrl Pts',(14.7473979137365,26.7080624063013,7.40028747986925));
#47254=CARTESIAN_POINT('Ctrl Pts',(14.7572628866864,26.7148157011212,7.38062842269809));
#47255=CARTESIAN_POINT('Ctrl Pts',(14.7671117981769,26.7214654268918,7.36090331359513));
#47256=CARTESIAN_POINT('Ctrl Pts',(14.7769448591095,26.7280110411829,7.3411103132182));
#47257=CARTESIAN_POINT('Ctrl Pts',(14.7786852863083,26.7291695985461,7.33760700164122));
#47258=CARTESIAN_POINT('Ctrl Pts',(14.7804252430215,26.7303249048412,7.3341015033297));
#47259=CARTESIAN_POINT('Ctrl Pts',(14.7821646285529,26.7314768936909,7.3305940181548));
#47260=CARTESIAN_POINT('Ctrl Pts',(14.78794790918,26.7353071398764,7.31893198538767));
#47261=CARTESIAN_POINT('Ctrl Pts',(14.7937273787648,26.7391023078568,7.3072429141235));
#47262=CARTESIAN_POINT('Ctrl Pts',(14.7994927953372,26.7428556865468,7.29554740361937));
#47263=CARTESIAN_POINT('Ctrl Pts',(14.8051580499374,26.7465438581858,7.28405507798198));
#47264=CARTESIAN_POINT('Ctrl Pts',(14.8108113279298,26.7501927519568,7.27255334308904));
#47265=CARTESIAN_POINT('Ctrl Pts',(14.816452375147,26.7538021411957,7.26104255703003));
#47266=CARTESIAN_POINT('Ctrl Pts',(14.8165521091315,26.75386595537,7.26083904578215));
#47267=CARTESIAN_POINT('Ctrl Pts',(14.8166518399196,26.7539297576608,7.26063553045111));
#47268=CARTESIAN_POINT('Ctrl Pts',(14.8167515675295,26.7539935480794,7.26043201099886));
#47269=CARTESIAN_POINT('Ctrl Pts',(14.8397132246179,26.7686808921284,7.21357293276645));
#47270=CARTESIAN_POINT('Ctrl Pts',(14.8624748126585,26.7827163343924,7.16655984206479));
#47271=CARTESIAN_POINT('Ctrl Pts',(14.8850347731502,26.7961020023305,7.11939232524414));
#47272=CARTESIAN_POINT('Ctrl Pts',(14.9301546941337,26.8228733382067,7.02505729160283));
#47273=CARTESIAN_POINT('Ctrl Pts',(14.9744681085358,26.8470455767767,6.93010455596954));
#47274=CARTESIAN_POINT('Ctrl Pts',(15.0179634542513,26.8686149665637,6.83452897348291));
#47275=CARTESIAN_POINT('Ctrl Pts',(15.0518694820136,26.8854290030292,6.76002471791515));
#47276=CARTESIAN_POINT('Ctrl Pts',(15.0852784766965,26.9006590046989,6.68514179979587));
#47277=CARTESIAN_POINT('Ctrl Pts',(15.11818516713,26.9142986900843,6.60987724941857));
#47278=CARTESIAN_POINT('Ctrl Pts',(15.1274918520523,26.9181562720121,6.58859089558124));
#47279=CARTESIAN_POINT('Ctrl Pts',(15.1367583557927,26.921886293869,6.5672739825884));
#47280=CARTESIAN_POINT('Ctrl Pts',(15.1459845498898,26.9254881988036,6.54592640551724));
#47281=CARTESIAN_POINT('Ctrl Pts',(15.1844555772193,26.9405072826993,6.45691210424756));
#47282=CARTESIAN_POINT('Ctrl Pts',(15.2222256053613,26.9533040744962,6.36736498601499));
#47283=CARTESIAN_POINT('Ctrl Pts',(15.2592854167753,26.963841419386,6.2772771620655));
#47284=CARTESIAN_POINT('Ctrl Pts',(15.2625387870946,26.964766461468,6.26936862067291));
#47285=CARTESIAN_POINT('Ctrl Pts',(15.2657866840963,26.965674091811,6.2614559125951));
#47286=CARTESIAN_POINT('Ctrl Pts',(15.269029101094,26.966564271014,6.25353903103056));
#47287=CARTESIAN_POINT('Ctrl Pts',(15.3092065579625,26.977594664871,6.15543932089992));
#47288=CARTESIAN_POINT('Ctrl Pts',(15.3485425859871,26.9859469157609,6.05669887485067));
#47289=CARTESIAN_POINT('Ctrl Pts',(15.3870245205822,26.9915481270336,5.9573044625394));
#47290=CARTESIAN_POINT('Ctrl Pts',(15.3892689468374,26.9918748129389,5.95150736759178));
#47291=CARTESIAN_POINT('Ctrl Pts',(15.3915104679287,26.9921921361717,5.94570804740638));
#47292=CARTESIAN_POINT('Ctrl Pts',(15.3937490813168,26.9925000827492,5.93990649938684));
#47293=CARTESIAN_POINT('Ctrl Pts',(15.4298927376898,26.9974720512608,5.84623728470405));
#47294=CARTESIAN_POINT('Ctrl Pts',(15.4652784277793,26.9999999999997,5.75198738946509));
#47295=CARTESIAN_POINT('Ctrl Pts',(15.4998946833985,27.,5.65714286308472));
#47296=CARTESIAN_POINT('',(16.4260329799192,25.1379309923314,1.56059116342174));
#47297=CARTESIAN_POINT('Ctrl Pts',(15.4998966741159,26.9999999999935,5.65714358966582));
#47298=CARTESIAN_POINT('Ctrl Pts',(15.4605694492474,27.0857112046842,5.76489474592549));
#47299=CARTESIAN_POINT('Ctrl Pts',(15.4207785141578,27.1734809441547,5.87042507646245));
#47300=CARTESIAN_POINT('Ctrl Pts',(15.3806244193455,27.2632762176172,5.97380887466604));
#47301=CARTESIAN_POINT('Ctrl Pts',(15.3782691166024,27.2685433032006,5.97987301693189));
#47302=CARTESIAN_POINT('Ctrl Pts',(15.3759125601364,27.2738173579326,5.98592977147193));
#47303=CARTESIAN_POINT('Ctrl Pts',(15.3735547702585,27.2790983825627,5.99197914719141));
#47304=CARTESIAN_POINT('Ctrl Pts',(15.3310004839505,27.3744123188118,6.10116057542921));
#47305=CARTESIAN_POINT('Ctrl Pts',(15.2880444697824,27.4719959961733,6.20793920008953));
#47306=CARTESIAN_POINT('Ctrl Pts',(15.2447991620941,27.5718319675762,6.31237932440066));
#47307=CARTESIAN_POINT('Ctrl Pts',(15.2015538544059,27.6716679389791,6.41681944871178));
#47308=CARTESIAN_POINT('Ctrl Pts',(15.1580191426619,27.7737562144739,6.51892100698712));
#47309=CARTESIAN_POINT('Ctrl Pts',(15.1143112165841,27.878098848085,6.61873074046543));
#47310=CARTESIAN_POINT('Ctrl Pts',(15.1126633328231,27.8820327920385,6.62249378423699));
#47311=CARTESIAN_POINT('Ctrl Pts',(15.1110152005509,27.8859699339714,6.62625357479283));
#47312=CARTESIAN_POINT('Ctrl Pts',(15.1093668257744,27.8899102732374,6.63001011493869));
#47313=CARTESIAN_POINT('Ctrl Pts',(15.067294250942,27.9904821947445,6.72589080824484));
#47314=CARTESIAN_POINT('Ctrl Pts',(15.0250644654567,28.0931422469056,6.81965016197501));
#47315=CARTESIAN_POINT('Ctrl Pts',(14.9827816132864,28.1979088402624,6.91131356524541));
#47316=CARTESIAN_POINT('Ctrl Pts',(14.9787573508417,28.207879980937,6.92003761228592));
#47317=CARTESIAN_POINT('Ctrl Pts',(14.9747326086664,28.2178702120797,6.92874266722994));
#47318=CARTESIAN_POINT('Ctrl Pts',(14.9707074756758,28.2278795472534,6.93742875118335));
#47319=CARTESIAN_POINT('Ctrl Pts',(14.952758123344,28.2725143665395,6.97616277105936));
#47320=CARTESIAN_POINT('Ctrl Pts',(14.9348010697903,28.317529336006,7.01451936651037));
#47321=CARTESIAN_POINT('Ctrl Pts',(14.9168444926374,28.3629268553635,7.05249958405971));
#47322=CARTESIAN_POINT('Ctrl Pts',(14.9115517161979,28.3763079646263,7.06369441250069));
#47323=CARTESIAN_POINT('Ctrl Pts',(14.9062586162459,28.3897232443503,7.07485731092418));
#47324=CARTESIAN_POINT('Ctrl Pts',(14.900965620398,28.4031722110485,7.08598783372623));
#47325=CARTESIAN_POINT('Ctrl Pts',(14.8952664954411,28.4176531107047,7.09797239636471));
#47326=CARTESIAN_POINT('Ctrl Pts',(14.8895690962475,28.4321690472932,7.10991600819615));
#47327=CARTESIAN_POINT('Ctrl Pts',(14.8838763075017,28.4467132589687,7.12181336541017));
#47328=CARTESIAN_POINT('Ctrl Pts',(14.877938180411,28.4618842728988,7.13422345514567));
#47329=CARTESIAN_POINT('Ctrl Pts',(14.8720042057682,28.4770882994026,7.14658502557187));
#47330=CARTESIAN_POINT('Ctrl Pts',(14.8660770570502,28.4923191860082,7.15889327576865));
#47331=CARTESIAN_POINT('Ctrl Pts',(14.8610446054279,28.5052509857072,7.16934360806462));
#47332=CARTESIAN_POINT('Ctrl Pts',(14.8560159746172,28.5182049390111,7.17975781925992));
#47333=CARTESIAN_POINT('Ctrl Pts',(14.8509911673286,28.5311814410601,7.19013639432679));
#47334=CARTESIAN_POINT('Ctrl Pts',(14.8444171067273,28.5481588704351,7.20371490142723));
#47335=CARTESIAN_POINT('Ctrl Pts',(14.8378500820084,28.5651738792742,7.21723139465462));
#47336=CARTESIAN_POINT('Ctrl Pts',(14.8312904741886,28.5822263963677,7.23068619636096));
#47337=CARTESIAN_POINT('Ctrl Pts',(14.7941745019158,28.678713986635,7.30681697441842));
#47338=CARTESIAN_POINT('Ctrl Pts',(14.7572952651303,28.7763985017568,7.38097825825209));
#47339=CARTESIAN_POINT('Ctrl Pts',(14.7207229839317,28.8752782662337,7.45321250522372));
#47340=CARTESIAN_POINT('Ctrl Pts',(14.6776871829316,28.9916333233289,7.53821290925047));
#47341=CARTESIAN_POINT('Ctrl Pts',(14.6350754185611,29.1096418353901,7.62054685582819));
#47342=CARTESIAN_POINT('Ctrl Pts',(14.5930071299595,29.2293096316852,7.70026989277396));
#47343=CARTESIAN_POINT('Ctrl Pts',(14.5814101538139,29.2622984844567,7.72224716326552));
#47344=CARTESIAN_POINT('Ctrl Pts',(14.5698545944106,29.2954136234644,7.74402578590885));
#47345=CARTESIAN_POINT('Ctrl Pts',(14.5583428293979,29.3286549581115,7.76560712769879));
#47346=CARTESIAN_POINT('Ctrl Pts',(14.5280954110866,29.4159973033722,7.82231258269372));
#47347=CARTESIAN_POINT('Ctrl Pts',(14.4981498437657,29.5042107576476,7.87765592020842));
#47348=CARTESIAN_POINT('Ctrl Pts',(14.4685529155124,29.5933054917983,7.93164594712575));
#47349=CARTESIAN_POINT('Ctrl Pts',(14.4276917901088,29.7163084964947,8.00618386003138));
#47350=CARTESIAN_POINT('Ctrl Pts',(14.3874934405528,29.8409884290493,8.0781455526749));
#47351=CARTESIAN_POINT('Ctrl Pts',(14.348083905333,29.9673763912336,8.14754584487634));
#47352=CARTESIAN_POINT('Ctrl Pts',(14.3318729112048,30.0193657004558,8.17609344695027));
#47353=CARTESIAN_POINT('Ctrl Pts',(14.3157957407696,30.0716445884368,8.20420699797485));
#47354=CARTESIAN_POINT('Ctrl Pts',(14.2998608525879,30.1242146835024,8.2318879727946));
#47355=CARTESIAN_POINT('Ctrl Pts',(14.2770574294696,30.1994444628066,8.27150048679177));
#47356=CARTESIAN_POINT('Ctrl Pts',(14.2545460134195,30.2752720256852,8.31022525165558));
#47357=CARTESIAN_POINT('Ctrl Pts',(14.2323537327013,30.3517071915215,8.34806018280675));
#47358=CARTESIAN_POINT('Ctrl Pts',(14.214138504925,30.4144444997552,8.37911475973689));
#47359=CARTESIAN_POINT('Ctrl Pts',(14.1961383970943,30.4775913242493,8.40956964533723));
#47360=CARTESIAN_POINT('Ctrl Pts',(14.1783685323836,30.5411531688201,8.43942330730726));
#47361=CARTESIAN_POINT('Ctrl Pts',(14.1593600597948,30.609145446752,8.47135785067454));
#47362=CARTESIAN_POINT('Ctrl Pts',(14.1406150048816,30.6776125759273,8.50260447704652));
#47363=CARTESIAN_POINT('Ctrl Pts',(14.1221532487268,30.7465637771849,8.53315820493967));
#47364=CARTESIAN_POINT('Ctrl Pts',(14.1022298693507,30.8209738674047,8.56613088137767));
#47365=CARTESIAN_POINT('Ctrl Pts',(14.0826363732492,30.8959476343974,8.59829668510921));
#47366=CARTESIAN_POINT('Ctrl Pts',(14.0633976982587,30.9714964270601,8.62964919221027));
#47367=CARTESIAN_POINT('Ctrl Pts',(14.0481434474469,31.0313986933219,8.65450844094409));
#47368=CARTESIAN_POINT('Ctrl Pts',(14.033112419075,31.0916627211746,8.67885607314034));
#47369=CARTESIAN_POINT('Ctrl Pts',(14.0183177786232,31.1522954179624,8.70268732550796));
#47370=CARTESIAN_POINT('Ctrl Pts',(14.015101549896,31.1654764494213,8.70786803663916));
#47371=CARTESIAN_POINT('Ctrl Pts',(14.0118965191854,31.1786747841575,8.71302430103908));
#47372=CARTESIAN_POINT('Ctrl Pts',(14.0087028170895,31.191890502718,8.71815607697348));
#47373=CARTESIAN_POINT('Ctrl Pts',(13.999750872967,31.2289341500401,8.73254044033435));
#47374=CARTESIAN_POINT('Ctrl Pts',(13.9908879533214,31.2661144055239,8.74673237050487));
#47375=CARTESIAN_POINT('Ctrl Pts',(13.9821170337287,31.303433206279,8.76073074892257));
#47376=CARTESIAN_POINT('Ctrl Pts',(13.9777432789681,31.3220428036803,8.76771125690659));
#47377=CARTESIAN_POINT('Ctrl Pts',(13.9733909131801,31.3406934119555,8.77464599131914));
#47378=CARTESIAN_POINT('Ctrl Pts',(13.9690630125404,31.3593734023405,8.78153052202542));
#47379=CARTESIAN_POINT('Ctrl Pts',(13.9650372173515,31.3767494517654,8.78793448387731));
#47380=CARTESIAN_POINT('Ctrl Pts',(13.961030484189,31.3941600858426,8.79429835191505));
#47381=CARTESIAN_POINT('Ctrl Pts',(13.9570487976368,31.4115807756301,8.80061298178852));
#47382=CARTESIAN_POINT('Ctrl Pts',(13.9567217978581,31.4130114662759,8.80113157674668));
#47383=CARTESIAN_POINT('Ctrl Pts',(13.9563949570268,31.4144422679483,8.80164985548056));
#47384=CARTESIAN_POINT('Ctrl Pts',(13.9560682763309,31.4158731763214,8.80216781630477));
#47385=CARTESIAN_POINT('Ctrl Pts',(13.9524171557598,31.4318656088748,8.80795676387294));
#47386=CARTESIAN_POINT('Ctrl Pts',(13.9487865760586,31.4478688324497,8.81370518755723));
#47387=CARTESIAN_POINT('Ctrl Pts',(13.9451764341561,31.4638840446531,8.81941354815297));
#47388=CARTESIAN_POINT('Ctrl Pts',(13.9373101220175,31.4987803621828,8.83185177010061));
#47389=CARTESIAN_POINT('Ctrl Pts',(13.92954125731,31.533731632952,8.84409912661643));
#47390=CARTESIAN_POINT('Ctrl Pts',(13.9218713056012,31.568737905583,8.85615636330126));
#47391=CARTESIAN_POINT('Ctrl Pts',(13.8999348550734,31.6688576190942,8.89064067116655));
#47392=CARTESIAN_POINT('Ctrl Pts',(13.8788078574992,31.7694274729138,8.92356928315047));
#47393=CARTESIAN_POINT('Ctrl Pts',(13.8585278428624,31.8704501006104,8.95495427283813));
#47394=CARTESIAN_POINT('Ctrl Pts',(13.8504447031737,31.9107153581073,8.96746359594845));
#47395=CARTESIAN_POINT('Ctrl Pts',(13.8424960957031,31.951052419582,8.97972818763168));
#47396=CARTESIAN_POINT('Ctrl Pts',(13.8346844161992,31.9914616384529,8.99174802005895));
#47397=CARTESIAN_POINT('Ctrl Pts',(13.807273796088,32.1332546737276,9.03392474534529));
#47398=CARTESIAN_POINT('Ctrl Pts',(13.7815485167864,32.2759361339262,9.0730889007526));
#47399=CARTESIAN_POINT('Ctrl Pts',(13.7576063783065,32.4195184154285,9.10924700295637));
#47400=CARTESIAN_POINT('Ctrl Pts',(13.7365494340305,32.5457980333979,9.14104780236572));
#47401=CARTESIAN_POINT('Ctrl Pts',(13.716872430334,32.6727747711858,9.17052232737716));
#47402=CARTESIAN_POINT('Ctrl Pts',(13.6986465683587,32.8004595027004,9.1976672148543));
#47403=CARTESIAN_POINT('Ctrl Pts',(13.6961492852466,32.8179546930028,9.20138657085338));
#47404=CARTESIAN_POINT('Ctrl Pts',(13.6936792456254,32.8354631714845,9.20506219838908));
#47405=CARTESIAN_POINT('Ctrl Pts',(13.6912366347723,32.8529849844081,9.20869400810665));
#47406=CARTESIAN_POINT('Ctrl Pts',(13.6709671751925,32.9983858280898,9.23883176835602));
#47407=CARTESIAN_POINT('Ctrl Pts',(13.6525860055183,33.1447047525089,9.2659530160941));
#47408=CARTESIAN_POINT('Ctrl Pts',(13.6361884527326,33.2919630415462,9.29002162328209));
#47409=CARTESIAN_POINT('Ctrl Pts',(13.6197908999469,33.4392213305834,9.31409023047008));
#47410=CARTESIAN_POINT('Ctrl Pts',(13.6053769480128,33.5874190011587,9.33510616152985));
#47411=CARTESIAN_POINT('Ctrl Pts',(13.5930518504658,33.7365821076625,9.35301783205155));
#47412=CARTESIAN_POINT('Ctrl Pts',(13.5924247354764,33.7441716962714,9.35392919823146));
#47413=CARTESIAN_POINT('Ctrl Pts',(13.5918030226177,33.7517637632298,9.3548325359547));
#47414=CARTESIAN_POINT('Ctrl Pts',(13.5911867246683,33.7593583129635,9.35572783994931));
#47415=CARTESIAN_POINT('Ctrl Pts',(13.5845976814368,33.8405541315953,9.36529982819296));
#47416=CARTESIAN_POINT('Ctrl Pts',(13.5786276639973,33.9220343469512,9.37395107782386));
#47417=CARTESIAN_POINT('Ctrl Pts',(13.5732924325667,34.0038056340085,9.38167002937256));
#47418=CARTESIAN_POINT('Ctrl Pts',(13.5706230872623,34.0447177863659,9.38553200749673));
#47419=CARTESIAN_POINT('Ctrl Pts',(13.5681126448878,34.0857028095819,9.3891605744006));
#47420=CARTESIAN_POINT('Ctrl Pts',(13.5657630841551,34.1267615927872,9.39255406929206));
#47421=CARTESIAN_POINT('Ctrl Pts',(13.5646152616427,34.1468198934904,9.39421188123031));
#47422=CARTESIAN_POINT('Ctrl Pts',(13.5635054330467,34.1669044611196,9.39581417050262));
#47423=CARTESIAN_POINT('Ctrl Pts',(13.562434633342,34.1869983310107,9.39735956752719));
#47424=CARTESIAN_POINT('Ctrl Pts',(13.5614279561067,34.2058889239908,9.39881242187242));
#47425=CARTESIAN_POINT('Ctrl Pts',(13.5604553138571,34.2247967000574,9.40021565665452));
#47426=CARTESIAN_POINT('Ctrl Pts',(13.5595183430496,34.2436929639982,9.40156701329765));
#47427=CARTESIAN_POINT('Ctrl Pts',(13.5594112076896,34.2458536055287,9.40172153047071));
#47428=CARTESIAN_POINT('Ctrl Pts',(13.5593045331735,34.2480141986753,9.40187537735987));
#47429=CARTESIAN_POINT('Ctrl Pts',(13.5591983208464,34.2501747229023,9.4020285521773));
#47430=CARTESIAN_POINT('Ctrl Pts',(13.5583756349098,34.2669094367188,9.40321499419979));
#47431=CARTESIAN_POINT('Ctrl Pts',(13.5575806104702,34.2836402092014,9.40436124872476));
#47432=CARTESIAN_POINT('Ctrl Pts',(13.5568132309541,34.3003672974803,9.40546738423807));
#47433=CARTESIAN_POINT('Ctrl Pts',(13.555080327866,34.3381405535122,9.40796526906137));
#47434=CARTESIAN_POINT('Ctrl Pts',(13.5534883604341,34.375894555659,9.41025862411392));
#47435=CARTESIAN_POINT('Ctrl Pts',(13.5520369777938,34.4136293845627,9.4123484688034));
#47436=CARTESIAN_POINT('Ctrl Pts',(13.5491342125133,34.4890990423703,9.41652815818236));
#47437=CARTESIAN_POINT('Ctrl Pts',(13.5467937861962,34.564492007726,9.41989380592011));
#47438=CARTESIAN_POINT('Ctrl Pts',(13.5450131527534,34.639808895649,9.42245319556493));
#47439=CARTESIAN_POINT('Ctrl Pts',(13.5442006828786,34.6741745887956,9.42362099739002));
#47440=CARTESIAN_POINT('Ctrl Pts',(13.5435048599725,34.7085244273738,9.42462079538545));
#47441=CARTESIAN_POINT('Ctrl Pts',(13.5429254222363,34.7428584709684,9.42545335820768));
#47442=CARTESIAN_POINT('Ctrl Pts',(13.5409650335913,34.8590194749976,9.42827013488828));
#47443=CARTESIAN_POINT('Ctrl Pts',(13.5403378655916,34.9749998595297,9.4291761058855));
#47444=CARTESIAN_POINT('Ctrl Pts',(13.5410293473817,35.0908012044776,9.42818546292229));
#47445=CARTESIAN_POINT('Ctrl Pts',(13.5419252124423,35.2408302875462,9.4269020127561));
#47446=CARTESIAN_POINT('Ctrl Pts',(13.545033190514,35.3905590014421,9.4224368778565));
#47447=CARTESIAN_POINT('Ctrl Pts',(13.5503249881556,35.5399902323981,9.41481602126595));
#47448=CARTESIAN_POINT('Ctrl Pts',(13.5524631372416,35.6003678718186,9.4117368166823));
#47449=CARTESIAN_POINT('Ctrl Pts',(13.5549580993085,35.6606969039799,9.40814200182775));
#47450=CARTESIAN_POINT('Ctrl Pts',(13.5578078379326,35.7209775476613,9.40403352980553));
#47451=CARTESIAN_POINT('Ctrl Pts',(13.562011040672,35.8098880759867,9.3979737667407));
#47452=CARTESIAN_POINT('Ctrl Pts',(13.566985985049,35.8986933353278,9.39079652578675));
#47453=CARTESIAN_POINT('Ctrl Pts',(13.5727235618244,35.9873935429952,9.38249904885336));
#47454=CARTESIAN_POINT('Ctrl Pts',(13.5823511708345,36.1362317985809,9.36857594737473));
#47455=CARTESIAN_POINT('Ctrl Pts',(13.5941242809196,36.2847745196704,9.35150127372894));
#47456=CARTESIAN_POINT('Ctrl Pts',(13.6080006813988,36.4330226315577,9.33126069412123));
#47457=CARTESIAN_POINT('Ctrl Pts',(13.6160160175688,36.5186542371842,9.31956925799733));
#47458=CARTESIAN_POINT('Ctrl Pts',(13.6247337631313,36.6041874492391,9.30682057126));
#47459=CARTESIAN_POINT('Ctrl Pts',(13.6341456855963,36.6896224774574,9.29301196727616));
#47460=CARTESIAN_POINT('Ctrl Pts',(13.6410279774516,36.7520952401738,9.28291468448575));
#47461=CARTESIAN_POINT('Ctrl Pts',(13.6482810994821,36.8145154277135,9.27224936331575));
#47462=CARTESIAN_POINT('Ctrl Pts',(13.6559013066663,36.8768830050661,9.26101289493422));
#47463=CARTESIAN_POINT('Ctrl Pts',(13.658078080858,36.8946988110537,9.25780310630416));
#47464=CARTESIAN_POINT('Ctrl Pts',(13.6602848252828,36.9125104930323,9.25454668824333));
#47465=CARTESIAN_POINT('Ctrl Pts',(13.6625214262135,36.9303178286985,9.25124360711876));
#47466=CARTESIAN_POINT('Ctrl Pts',(13.6675536560891,36.9703833608706,9.24381185508443));
#47467=CARTESIAN_POINT('Ctrl Pts',(13.6727370256631,37.0104268883538,9.23614384654524));
#47468=CARTESIAN_POINT('Ctrl Pts',(13.6780701456487,37.0504458776819,9.22823911105019));
#47469=CARTESIAN_POINT('Ctrl Pts',(13.6801894433611,37.0663487924424,9.22509789392069));
#47470=CARTESIAN_POINT('Ctrl Pts',(13.6823330914514,37.082252742982,9.22191824754957));
#47471=CARTESIAN_POINT('Ctrl Pts',(13.6844999020291,37.0981498912587,9.21870177221577));
#47472=CARTESIAN_POINT('Ctrl Pts',(13.6870106441776,37.1165703478635,9.21497475506304));
#47473=CARTESIAN_POINT('Ctrl Pts',(13.6895539090126,37.1349919943203,9.21119617473931));
#47474=CARTESIAN_POINT('Ctrl Pts',(13.692126041947,37.153389257747,9.20737120104998));
#47475=CARTESIAN_POINT('Ctrl Pts',(13.6929190136733,37.159061013488,9.20619198672997));
#47476=CARTESIAN_POINT('Ctrl Pts',(13.6937147748413,37.1647308023172,9.20500829519152));
#47477=CARTESIAN_POINT('Ctrl Pts',(13.6945132874207,37.1703983687995,9.20382017537598));
#47478=CARTESIAN_POINT('Ctrl Pts',(13.6963048804354,37.1831144772008,9.20115443507714));
#47479=CARTESIAN_POINT('Ctrl Pts',(13.6981102581906,37.1958192091792,9.19846651393387));
#47480=CARTESIAN_POINT('Ctrl Pts',(13.6999295033177,37.2085136766366,9.19575620104296));
#47481=CARTESIAN_POINT('Ctrl Pts',(13.7051896678105,37.2452184537887,9.18791960364278));
#47482=CARTESIAN_POINT('Ctrl Pts',(13.7105651593549,37.2818337180102,9.17989671027503));
#47483=CARTESIAN_POINT('Ctrl Pts',(13.7160536764026,37.3183604197314,9.17168881921092));
#47484=CARTESIAN_POINT('Ctrl Pts',(13.7324696154778,37.4276103509729,9.14713933918296));
#47485=CARTESIAN_POINT('Ctrl Pts',(13.749897166982,37.536067723453,9.1209341917559));
#47486=CARTESIAN_POINT('Ctrl Pts',(13.7682796425987,37.6437540820578,9.09310044392041));
#47487=CARTESIAN_POINT('Ctrl Pts',(13.7744812082209,37.6800834662732,9.08371036951942));
#47488=CARTESIAN_POINT('Ctrl Pts',(13.7807913364897,37.7163252869045,9.07413535277473));
#47489=CARTESIAN_POINT('Ctrl Pts',(13.7872080111268,37.7524800859917,9.06437582107082));
#47490=CARTESIAN_POINT('Ctrl Pts',(13.8126447804049,37.8958037442233,9.0256874084189));
#47491=CARTESIAN_POINT('Ctrl Pts',(13.8397556926634,38.0377606814329,8.98409980770552));
#47492=CARTESIAN_POINT('Ctrl Pts',(13.868407440965,38.178392692106,8.9396504174699));
#47493=CARTESIAN_POINT('Ctrl Pts',(13.8944482538081,38.3062093904499,8.8992515475674));
#47494=CARTESIAN_POINT('Ctrl Pts',(13.9217625847717,38.4329310416233,8.8564876540994));
#47495=CARTESIAN_POINT('Ctrl Pts',(13.9502567594613,38.5585839638948,8.81137539463128));
#47496=CARTESIAN_POINT('Ctrl Pts',(13.9531136768512,38.5711823290918,8.80685229473544));
#47497=CARTESIAN_POINT('Ctrl Pts',(13.9559824579279,38.5837699469257,8.80230558332653));
#47498=CARTESIAN_POINT('Ctrl Pts',(13.9588630164218,38.5963468272929,8.79773524200746));
#47499=CARTESIAN_POINT('Ctrl Pts',(13.990473540025,38.7343623456489,8.74758146716013));
#47500=CARTESIAN_POINT('Ctrl Pts',(14.0235015619679,38.8710858072657,8.69458344629727));
#47501=CARTESIAN_POINT('Ctrl Pts',(14.0578212325299,39.0065423683161,8.6387349163809));
#47502=CARTESIAN_POINT('Ctrl Pts',(14.0921409030919,39.1419989293664,8.58288638646454));
#47503=CARTESIAN_POINT('Ctrl Pts',(14.1277522803669,39.2761886042384,8.52418741505491));
#47504=CARTESIAN_POINT('Ctrl Pts',(14.164539316697,39.4091280855466,8.46261347849984));
#47505=CARTESIAN_POINT('Ctrl Pts',(14.1667788306083,39.4172211489582,8.45886499258629));
#47506=CARTESIAN_POINT('Ctrl Pts',(14.1690226941704,39.4253095865658,8.45510586318291));
#47507=CARTESIAN_POINT('Ctrl Pts',(14.1712708793468,39.4333934036186,8.45133608751763));
#47508=CARTESIAN_POINT('Ctrl Pts',(14.1874874309478,39.4917033852633,8.4241440384631));
#47509=CARTESIAN_POINT('Ctrl Pts',(14.2039291632183,39.5497722972026,8.39639657437115));
#47510=CARTESIAN_POINT('Ctrl Pts',(14.220586013407,39.6076010566071,8.36809019771358));
#47511=CARTESIAN_POINT('Ctrl Pts',(14.2242846970821,39.620442037101,8.36180471564109));
#47512=CARTESIAN_POINT('Ctrl Pts',(14.2279940116495,39.6332712521396,8.35549163407334));
#47513=CARTESIAN_POINT('Ctrl Pts',(14.2317138707491,39.6460887874945,8.34915087306062));
#47514=CARTESIAN_POINT('Ctrl Pts',(14.2375313413513,39.6661340723086,8.33923458596492));
#47515=CARTESIAN_POINT('Ctrl Pts',(14.2433757952081,39.6861546944092,8.32924851654006));
#47516=CARTESIAN_POINT('Ctrl Pts',(14.2492418576234,39.7061341133082,8.31920104913758));
#47517=CARTESIAN_POINT('Ctrl Pts',(14.2536890975557,39.7212811170836,8.31158375919293));
#47518=CARTESIAN_POINT('Ctrl Pts',(14.2581484788514,39.736403444488,8.30393165731456));
#47519=CARTESIAN_POINT('Ctrl Pts',(14.2626178939433,39.7514947403366,8.29624799601414));
#47520=CARTESIAN_POINT('Ctrl Pts',(14.2678134243439,39.7690378158295,8.28731602280211));
#47521=CARTESIAN_POINT('Ctrl Pts',(14.2730238234764,39.7865435386285,8.27833918385668));
#47522=CARTESIAN_POINT('Ctrl Pts',(14.2782491820152,39.8040136477705,8.26931679747083));
#47523=CARTESIAN_POINT('Ctrl Pts',(14.2834414501267,39.8213731246233,8.26035154680477));
#47524=CARTESIAN_POINT('Ctrl Pts',(14.2886481552757,39.8386962121138,8.25134189848024));
#47525=CARTESIAN_POINT('Ctrl Pts',(14.2938689492472,39.8559830980089,8.2422879385366));
#47526=CARTESIAN_POINT('Ctrl Pts',(14.32774350029,39.9681471676544,8.18354230905482));
#47527=CARTESIAN_POINT('Ctrl Pts',(14.3622105379506,40.07878847771,8.12293253524994));
#47528=CARTESIAN_POINT('Ctrl Pts',(14.3971792690442,40.1879497097792,8.06047326532415));
#47529=CARTESIAN_POINT('Ctrl Pts',(14.4053895058454,40.2135794520311,8.04580858117672));
#47530=CARTESIAN_POINT('Ctrl Pts',(14.4136274917622,40.2391274299263,8.03104176990634));
#47531=CARTESIAN_POINT('Ctrl Pts',(14.4218920252206,40.2645942448818,8.01617305282824));
#47532=CARTESIAN_POINT('Ctrl Pts',(14.454252553542,40.3643118624307,7.95795324616492));
#47533=CARTESIAN_POINT('Ctrl Pts',(14.4870188730222,40.4627881460053,7.89817432298111));
#47534=CARTESIAN_POINT('Ctrl Pts',(14.5201258358726,40.5600444217448,7.8368339102019));
#47535=CARTESIAN_POINT('Ctrl Pts',(14.5616879635914,40.6821389120185,7.75982781085761));
#47536=CARTESIAN_POINT('Ctrl Pts',(14.6037856063819,40.8023132277205,7.68036347799239));
#47537=CARTESIAN_POINT('Ctrl Pts',(14.6462939201702,40.9206016188664,7.59842619851696));
#47538=CARTESIAN_POINT('Ctrl Pts',(14.6605297485143,40.9602158279793,7.5709858005891));
#47539=CARTESIAN_POINT('Ctrl Pts',(14.6748118124644,40.9996181534556,7.54326767465988));
#47540=CARTESIAN_POINT('Ctrl Pts',(14.6891352187837,41.0388102533568,7.51527155359934));
#47541=CARTESIAN_POINT('Ctrl Pts',(14.7175816348888,41.1166461226299,7.45967100082168));
#47542=CARTESIAN_POINT('Ctrl Pts',(14.7461916611224,41.1936525631517,7.40297395014157));
#47543=CARTESIAN_POINT('Ctrl Pts',(14.7749303180739,41.2698321114896,7.34516658947509));
#47544=CARTESIAN_POINT('Ctrl Pts',(14.8181395311428,41.384369765117,7.25825193065136));
#47545=CARTESIAN_POINT('Ctrl Pts',(14.8616378266614,41.4970416057414,7.16883096877626));
#47546=CARTESIAN_POINT('Ctrl Pts',(14.9053081022752,41.6078521323305,7.07685057936598));
#47547=CARTESIAN_POINT('Ctrl Pts',(14.9252103018943,41.6583526888091,7.03493163002678));
#47548=CARTESIAN_POINT('Ctrl Pts',(14.9451486273982,41.7084657999447,6.99248017876618));
#47549=CARTESIAN_POINT('Ctrl Pts',(14.9651116680086,41.7581924532683,6.9494915471597));
#47550=CARTESIAN_POINT('Ctrl Pts',(14.9889524029723,41.8175781944316,6.89815264580769));
#47551=CARTESIAN_POINT('Ctrl Pts',(15.0128287365156,41.8764113900424,6.84604605414212));
#47552=CARTESIAN_POINT('Ctrl Pts',(15.0367217535436,41.9346894966983,6.7931586175325));
#47553=CARTESIAN_POINT('Ctrl Pts',(15.0586716715574,41.988228137783,6.74457225038686));
#47554=CARTESIAN_POINT('Ctrl Pts',(15.080635583353,42.0412985081664,6.69532707559198));
#47555=CARTESIAN_POINT('Ctrl Pts',(15.1025992182023,42.0938977223522,6.64541171525283));
#47556=CARTESIAN_POINT('Ctrl Pts',(15.1031379467204,42.0951878866127,6.64418738110714));
#47557=CARTESIAN_POINT('Ctrl Pts',(15.1036766779631,42.0964777746802,6.64296263716632));
#47558=CARTESIAN_POINT('Ctrl Pts',(15.1042154112924,42.0977673854986,6.64173748421894));
#47559=CARTESIAN_POINT('Ctrl Pts',(15.1146585934605,42.1227661000223,6.61798826597259));
#47560=CARTESIAN_POINT('Ctrl Pts',(15.125102165282,42.1476594144795,6.59408588091983));
#47561=CARTESIAN_POINT('Ctrl Pts',(15.1355215378525,42.1723927739372,6.57008277606289));
#47562=CARTESIAN_POINT('Ctrl Pts',(15.1366606880725,42.1750968726416,6.56745851610917));
#47563=CARTESIAN_POINT('Ctrl Pts',(15.1377995943815,42.1777991668441,6.56483294813743));
#47564=CARTESIAN_POINT('Ctrl Pts',(15.1389382253939,42.1804995871324,6.56220613876985));
#47565=CARTESIAN_POINT('Ctrl Pts',(15.1487514780318,42.203773067505,6.53956707161244));
#47566=CARTESIAN_POINT('Ctrl Pts',(15.1585492995077,42.2269193893911,6.5168244186884));
#47567=CARTESIAN_POINT('Ctrl Pts',(15.1683284209863,42.249934449691,6.49398282359018));
#47568=CARTESIAN_POINT('Ctrl Pts',(15.1700553459567,42.2539987495787,6.489949156453));
#47569=CARTESIAN_POINT('Ctrl Pts',(15.1717817099298,42.258059005505,6.48591235260955));
#47570=CARTESIAN_POINT('Ctrl Pts',(15.1735075060744,42.2621152203853,6.48187241181925));
#47571=CARTESIAN_POINT('Ctrl Pts',(15.1964839485354,42.3161177676152,6.42808653021052));
#47572=CARTESIAN_POINT('Ctrl Pts',(15.2193597296865,42.3694041467529,6.37374468565707));
#47573=CARTESIAN_POINT('Ctrl Pts',(15.2421189807697,42.4219798813043,6.31884554139977));
#47574=CARTESIAN_POINT('Ctrl Pts',(15.2608644872042,42.4652835368918,6.27362822479454));
#47575=CARTESIAN_POINT('Ctrl Pts',(15.2795307517416,42.508106509307,6.22803369293663));
#47576=CARTESIAN_POINT('Ctrl Pts',(15.2981092430933,42.5504495124992,6.18205979987793));
#47577=CARTESIAN_POINT('Ctrl Pts',(15.3409384613079,42.6480633439594,6.07607563460213));
#47578=CARTESIAN_POINT('Ctrl Pts',(15.3833002938721,42.7431310467078,5.968077837435));
#47579=CARTESIAN_POINT('Ctrl Pts',(15.4250886320099,42.8356685001976,5.85804219315313));
#47580=CARTESIAN_POINT('Ctrl Pts',(15.4529471198793,42.897359240734,5.78468616135029));
#47581=CARTESIAN_POINT('Ctrl Pts',(15.4805511466514,42.9579234845588,5.71042330098948));
#47582=CARTESIAN_POINT('Ctrl Pts',(15.5078694486391,43.017364224858,5.63524490719013));
#47583=CARTESIAN_POINT('Ctrl Pts',(15.5215291942096,43.0470858887221,5.59765407404954));
#47584=CARTESIAN_POINT('Ctrl Pts',(15.5351176224385,43.0765266266366,5.55983436456525));
#47585=CARTESIAN_POINT('Ctrl Pts',(15.5486308477265,43.1056851559705,5.521783643378));
#47586=CARTESIAN_POINT('Ctrl Pts',(15.5891693471925,43.1931582055674,5.40763479233376));
#47587=CARTESIAN_POINT('Ctrl Pts',(15.6290303150042,43.2780960580346,5.29140933264386));
#47588=CARTESIAN_POINT('Ctrl Pts',(15.6681066473624,43.3604744479936,5.1730534869981));
#47589=CARTESIAN_POINT('Ctrl Pts',(15.6976993071593,43.4228599258919,5.08342214076338));
#47590=CARTESIAN_POINT('Ctrl Pts',(15.7268423285855,43.4837755221708,4.99256790568704));
#47591=CARTESIAN_POINT('Ctrl Pts',(15.7554897945147,43.5432056956577,4.90046337961948));
#47592=CARTESIAN_POINT('Ctrl Pts',(15.7646705571918,43.5622515100411,4.87094629083393));
#47593=CARTESIAN_POINT('Ctrl Pts',(15.7738004920941,43.5811448088722,4.84130084737862));
#47594=CARTESIAN_POINT('Ctrl Pts',(15.7828779731803,43.5998843939893,4.81152567589992));
#47595=CARTESIAN_POINT('Ctrl Pts',(15.820280642411,43.6770986009926,4.68884066234464));
#47596=CARTESIAN_POINT('Ctrl Pts',(15.8567922974239,43.7517065136738,4.56395518348118));
#47597=CARTESIAN_POINT('Ctrl Pts',(15.8922960486642,43.8236398234513,4.43678015380184));
#47598=CARTESIAN_POINT('Ctrl Pts',(15.9220503656959,43.883924340706,4.33019969344502));
#47599=CARTESIAN_POINT('Ctrl Pts',(15.951097141453,43.9423283107648,4.22200998600328));
#47600=CARTESIAN_POINT('Ctrl Pts',(15.9793684755964,43.9988013639996,4.11215066858206));
#47601=CARTESIAN_POINT('Ctrl Pts',(15.9848313526463,44.0097136663654,4.09092252487934));
#47602=CARTESIAN_POINT('Ctrl Pts',(15.9902652197226,44.0205536468183,4.0696318793639));
#47603=CARTESIAN_POINT('Ctrl Pts',(15.9956695421084,44.0313207899642,4.04827818753736));
#47604=CARTESIAN_POINT('Ctrl Pts',(16.0040126986106,44.0479430330382,4.01531250190834));
#47605=CARTESIAN_POINT('Ctrl Pts',(16.0122853930047,44.0643920223782,3.98219675102727));
#47606=CARTESIAN_POINT('Ctrl Pts',(16.0204856406259,44.0806659925568,3.94892897658108));
#47607=CARTESIAN_POINT('Ctrl Pts',(16.0239840231979,44.0876087796871,3.93473630732213));
#47608=CARTESIAN_POINT('Ctrl Pts',(16.0274694356842,44.094520134833,3.92051509179209));
#47609=CARTESIAN_POINT('Ctrl Pts',(16.0309415561632,44.1013995895602,3.90626584129641));
#47610=CARTESIAN_POINT('Ctrl Pts',(16.0356081246678,44.1106456531553,3.88711469029829));
#47611=CARTESIAN_POINT('Ctrl Pts',(16.0402460460161,44.1198248975802,3.8679318106028));
#47612=CARTESIAN_POINT('Ctrl Pts',(16.0448535023226,44.1289342001359,3.84872390390704));
#47613=CARTESIAN_POINT('Ctrl Pts',(16.0485719715433,44.1362859054851,3.83322207272546));
#47614=CARTESIAN_POINT('Ctrl Pts',(16.0522710666275,44.1435929733322,3.81770199088401));
#47615=CARTESIAN_POINT('Ctrl Pts',(16.0559499973327,44.1508540876384,3.8021664460082));
#47616=CARTESIAN_POINT('Ctrl Pts',(16.0641803427192,44.167098339955,3.76741099385671));
#47617=CARTESIAN_POINT('Ctrl Pts',(16.0723121239858,44.1831172675052,3.73256848436886));
#47618=CARTESIAN_POINT('Ctrl Pts',(16.0803438330845,44.198910582354,3.69764008656643));
#47619=CARTESIAN_POINT('Ctrl Pts',(16.0842385396404,44.2065690179529,3.6807027375868));
#47620=CARTESIAN_POINT('Ctrl Pts',(16.0881097169479,44.2141744366289,3.66374520113459));
#47621=CARTESIAN_POINT('Ctrl Pts',(16.0919571938468,44.2217267787567,3.64676760402783));
#47622=CARTESIAN_POINT('Ctrl Pts',(16.119779354582,44.2763398361267,3.52399794276193));
#47623=CARTESIAN_POINT('Ctrl Pts',(16.146363769354,44.3281808208329,3.40017266404339));
#47624=CARTESIAN_POINT('Ctrl Pts',(16.1716578797485,44.3772491775588,3.27528341069522));
#47625=CARTESIAN_POINT('Ctrl Pts',(16.1742349382788,44.3822484451867,3.26255922665919));
#47626=CARTESIAN_POINT('Ctrl Pts',(16.1767986099626,44.3872189871422,3.24982401275424));
#47627=CARTESIAN_POINT('Ctrl Pts',(16.1793488358425,44.392160772613,3.23707775248512));
#47628=CARTESIAN_POINT('Ctrl Pts',(16.2069298067276,44.4456067211725,3.09922555823363));
#47629=CARTESIAN_POINT('Ctrl Pts',(16.2329384035846,44.4956855666432,2.96008015930213));
#47630=CARTESIAN_POINT('Ctrl Pts',(16.2572990629811,44.5423720081378,2.81962161298135));
#47631=CARTESIAN_POINT('Ctrl Pts',(16.2807607446571,44.58733558696,2.6843463871008));
#47632=CARTESIAN_POINT('Ctrl Pts',(16.3026939376851,44.6291520070692,2.54785305659329));
#47633=CARTESIAN_POINT('Ctrl Pts',(16.3230308540642,44.6677770232203,2.41011695510189));
#47634=CARTESIAN_POINT('Ctrl Pts',(16.3238101006238,44.6692570121423,2.40483934166183));
#47635=CARTESIAN_POINT('Ctrl Pts',(16.3245870042843,44.6707323159118,2.39955990406438));
#47636=CARTESIAN_POINT('Ctrl Pts',(16.3253615607141,44.6722029293553,2.39427864025978));
#47637=CARTESIAN_POINT('Ctrl Pts',(16.3463506296786,44.7120538760335,2.25116600709553));
#47638=CARTESIAN_POINT('Ctrl Pts',(16.3656162765854,44.7484612211025,2.10671223998137));
#47639=CARTESIAN_POINT('Ctrl Pts',(16.3830708867426,44.7813476320185,1.96087946147297));
#47640=CARTESIAN_POINT('Ctrl Pts',(16.4005254968998,44.8142340429344,1.81504668296456));
#47641=CARTESIAN_POINT('Ctrl Pts',(16.416169147287,44.8435995213574,1.66783495942057));
#47642=CARTESIAN_POINT('Ctrl Pts',(16.4299130047968,44.8693369120098,1.51919671520907));
#47643=CARTESIAN_POINT('Ctrl Pts',(16.4299744557924,44.8694519880194,1.51853212973313));
#47644=CARTESIAN_POINT('Ctrl Pts',(16.4300358688024,44.8695669915828,1.51786751575435));
#47645=CARTESIAN_POINT('Ctrl Pts',(16.4300972438189,44.8696819226926,1.51720287326893));
#47646=CARTESIAN_POINT('Ctrl Pts',(16.4334675848922,44.8759932373363,1.48070476707978));
#47647=CARTESIAN_POINT('Ctrl Pts',(16.4367232683546,44.8820856492454,1.4441205857469));
#47648=CARTESIAN_POINT('Ctrl Pts',(16.4398627890822,44.8879572706997,1.40744951143586));
#47649=CARTESIAN_POINT('Ctrl Pts',(16.4414611352971,44.8909465435032,1.38878007813454));
#47650=CARTESIAN_POINT('Ctrl Pts',(16.4430293733771,44.893878591633,1.37008812314347));
#47651=CARTESIAN_POINT('Ctrl Pts',(16.4445673042119,44.8967531505756,1.35137353294673));
#47652=CARTESIAN_POINT('Ctrl Pts',(16.4461052350467,44.8996277095182,1.33265894274999));
#47653=CARTESIAN_POINT('Ctrl Pts',(16.4476131566932,44.902445337259,1.31391780126205));
#47654=CARTESIAN_POINT('Ctrl Pts',(16.4490892691905,44.9052027752656,1.29517070927396));
#47655=CARTESIAN_POINT('Ctrl Pts',(16.4549937191796,44.916232527292,1.22018234132153));
#47656=CARTESIAN_POINT('Ctrl Pts',(16.4603932334168,44.9263069163642,1.14505238033023));
#47657=CARTESIAN_POINT('Ctrl Pts',(16.4652837831854,44.9354238512759,1.0697803390153));
#47658=CARTESIAN_POINT('Ctrl Pts',(16.4654957634851,44.9358190237382,1.06651768131284));
#47659=CARTESIAN_POINT('Ctrl Pts',(16.4657067875804,44.9362123981677,1.06325475685442));
#47660=CARTESIAN_POINT('Ctrl Pts',(16.4659168551513,44.9366039744898,1.05999156564776));
#47661=CARTESIAN_POINT('Ctrl Pts',(16.4705532092148,44.9452463673385,0.987970407184138));
#47662=CARTESIAN_POINT('Ctrl Pts',(16.4747234822227,44.9530123827719,0.915819173905195));
#47663=CARTESIAN_POINT('Ctrl Pts',(16.4784236180288,44.9598986924698,0.843537246033712));
#47664=CARTESIAN_POINT('Ctrl Pts',(16.4786783669902,44.9603728048634,0.838560740570758));
#47665=CARTESIAN_POINT('Ctrl Pts',(16.4789308802764,44.9608427339334,0.83358375782864));
#47666=CARTESIAN_POINT('Ctrl Pts',(16.4791811594326,44.9613084838401,0.828606248227442));
#47667=CARTESIAN_POINT('Ctrl Pts',(16.4808308405885,44.9643784112603,0.795797667937533));
#47668=CARTESIAN_POINT('Ctrl Pts',(16.4823838000093,44.9672673955566,0.762958679875174));
#47669=CARTESIAN_POINT('Ctrl Pts',(16.4838394108821,44.9699745720358,0.730094620377697));
#47670=CARTESIAN_POINT('Ctrl Pts',(16.4841034886147,44.9704657094954,0.724132404460733));
#47671=CARTESIAN_POINT('Ctrl Pts',(16.4843643638248,44.9709508668914,0.718169308811079));
#47672=CARTESIAN_POINT('Ctrl Pts',(16.484622032976,44.9714300393822,0.712205328484882));
#47673=CARTESIAN_POINT('Ctrl Pts',(16.4860001270905,44.9739928016937,0.680308121744984));
#47674=CARTESIAN_POINT('Ctrl Pts',(16.4872841965825,44.9763800615371,0.648441210361427));
#47675=CARTESIAN_POINT('Ctrl Pts',(16.4884754167523,44.9785942330604,0.616586113928043));
#47676=CARTESIAN_POINT('Ctrl Pts',(16.4887361289235,44.979078829846,0.6096142613972));
#47677=CARTESIAN_POINT('Ctrl Pts',(16.4889923805622,44.9795551113289,0.602643277310825));
#47678=CARTESIAN_POINT('Ctrl Pts',(16.4892441756933,44.9800230876665,0.595673160690036));
#47679=CARTESIAN_POINT('Ctrl Pts',(16.4944547318202,44.9897072184245,0.451436122767426));
#47680=CARTESIAN_POINT('Ctrl Pts',(16.4977573423716,44.9958371005211,0.307570384139903));
#47681=CARTESIAN_POINT('Ctrl Pts',(16.4991842745932,44.9984857834022,0.164068590449055));
#47682=CARTESIAN_POINT('Ctrl Pts',(16.4992938671831,44.9986892100349,0.153047230779077));
#47683=CARTESIAN_POINT('Ctrl Pts',(16.4993923956434,44.9988720974294,0.142028018465499));
#47684=CARTESIAN_POINT('Ctrl Pts',(16.4994798745568,44.9990344787445,0.13101095028804));
#47685=CARTESIAN_POINT('Ctrl Pts',(16.5005864417034,45.0010885260745,-0.00834978501705821));
#47686=CARTESIAN_POINT('Ctrl Pts',(16.4999249385232,44.99986126589,-0.147367414719779));
#47687=CARTESIAN_POINT('Ctrl Pts',(16.4975203492931,44.9953967706039,-0.286046671625515));
#47688=CARTESIAN_POINT('Ctrl Pts',(16.4972585106042,44.9949106262023,-0.301147627060495));
#47689=CARTESIAN_POINT('Ctrl Pts',(16.4969760035298,44.9943860851946,-0.316244569169732));
#47690=CARTESIAN_POINT('Ctrl Pts',(16.496672860267,44.9938232046973,-0.331337503657238));
#47691=CARTESIAN_POINT('Ctrl Pts',(16.4939720147342,44.9888082382989,-0.465807537110266));
#47692=CARTESIAN_POINT('Ctrl Pts',(16.4896330752602,44.9807498770209,-0.599959432563676));
#47693=CARTESIAN_POINT('Ctrl Pts',(16.4836750864447,44.9696687937092,-0.733795728849868));
#47694=CARTESIAN_POINT('Ctrl Pts',(16.4828199556229,44.9680783617411,-0.753004818622123));
#47695=CARTESIAN_POINT('Ctrl Pts',(16.4819314724365,44.9664256375575,-0.772207405753413));
#47696=CARTESIAN_POINT('Ctrl Pts',(16.4810096931329,44.964710682917,-0.791403496870234));
#47697=CARTESIAN_POINT('Ctrl Pts',(16.4747882752629,44.9531358412971,-0.920964774557578));
#47698=CARTESIAN_POINT('Ctrl Pts',(16.4670500736832,44.9387261544842,-1.05023011813212));
#47699=CARTESIAN_POINT('Ctrl Pts',(16.4578093131587,44.9214832065221,-1.1792002767713));
#47700=CARTESIAN_POINT('Ctrl Pts',(16.4561366865308,44.9183621415591,-1.20254455898384));
#47701=CARTESIAN_POINT('Ctrl Pts',(16.4544148316611,44.9151482076373,-1.22587916896365));
#47702=CARTESIAN_POINT('Ctrl Pts',(16.4526438329193,44.9118414151564,-1.2492041094649));
#47703=CARTESIAN_POINT('Ctrl Pts',(16.443180940093,44.8941723891387,-1.37383514783657));
#47704=CARTESIAN_POINT('Ctrl Pts',(16.4323149566667,44.8738522519087,-1.49819010731742));
#47705=CARTESIAN_POINT('Ctrl Pts',(16.4200562281029,44.8508667452653,-1.6222682560188));
#47706=CARTESIAN_POINT('Ctrl Pts',(16.4173388192111,44.8457715170114,-1.64977282656279));
#47707=CARTESIAN_POINT('Ctrl Pts',(16.4145529103487,44.8405451493894,-1.67726442598618));
#47708=CARTESIAN_POINT('Ctrl Pts',(16.4116986443443,44.8351875376271,-1.70474268064929));
#47709=CARTESIAN_POINT('Ctrl Pts',(16.4038308879674,44.820419333107,-1.78048622137831));
#47710=CARTESIAN_POINT('Ctrl Pts',(16.3954436387708,44.8046533890257,-1.85612832314843));
#47711=CARTESIAN_POINT('Ctrl Pts',(16.3865397744708,44.7878852560871,-1.9316610001985));
#47712=CARTESIAN_POINT('Ctrl Pts',(16.3820866822432,44.7794990049107,-1.96943717981755));
#47713=CARTESIAN_POINT('Ctrl Pts',(16.377504371403,44.7708620589204,-2.00718598805293));
#47714=CARTESIAN_POINT('Ctrl Pts',(16.3727932172076,44.7619737563975,-2.04490642000078));
#47715=CARTESIAN_POINT('Ctrl Pts',(16.3720401557642,44.7605529924721,-2.05093589850025));
#47716=CARTESIAN_POINT('Ctrl Pts',(16.3712837309502,44.7591256713598,-2.05696519021422));
#47717=CARTESIAN_POINT('Ctrl Pts',(16.3705239817059,44.7576918606981,-2.06299400873138));
#47718=CARTESIAN_POINT('Ctrl Pts',(16.3682159895784,44.7533361818419,-2.08130855893217));
#47719=CARTESIAN_POINT('Ctrl Pts',(16.3658775520689,44.7489210288428,-2.09961695772403));
#47720=CARTESIAN_POINT('Ctrl Pts',(16.3635087125001,44.7444463373124,-2.11791921235832));
#47721=CARTESIAN_POINT('Ctrl Pts',(16.3617786253703,44.7411782366236,-2.13128630382624));
#47722=CARTESIAN_POINT('Ctrl Pts',(16.3600322470299,44.7378782361758,-2.14465061537265));
#47723=CARTESIAN_POINT('Ctrl Pts',(16.3582707990857,44.7345485708757,-2.15800288780629));
#47724=CARTESIAN_POINT('Ctrl Pts',(16.3576204681566,44.7333192502277,-2.16293257974857));
#47725=CARTESIAN_POINT('Ctrl Pts',(16.3569681873215,44.7320860844049,-2.16785987516607));
#47726=CARTESIAN_POINT('Ctrl Pts',(16.3563140031161,44.7308491577237,-2.17278446775161));
#47727=CARTESIAN_POINT('Ctrl Pts',(16.3514618653041,44.7216747712565,-2.20931057415699));
#47728=CARTESIAN_POINT('Ctrl Pts',(16.3465010296124,44.7122858451787,-2.24571805287309));
#47729=CARTESIAN_POINT('Ctrl Pts',(16.341433306043,44.7026846488829,-2.28200831008602));
#47730=CARTESIAN_POINT('Ctrl Pts',(16.3312978589041,44.6834822562912,-2.35458882451186));
#47731=CARTESIAN_POINT('Ctrl Pts',(16.3207348679184,44.663430782441,-2.42670045515599));
#47732=CARTESIAN_POINT('Ctrl Pts',(16.3097587820106,44.6425471384181,-2.49835388334598));
#47733=CARTESIAN_POINT('Ctrl Pts',(16.3043316767858,44.6322212595444,-2.53378278739943));
#47734=CARTESIAN_POINT('Ctrl Pts',(16.298803590232,44.6216917192259,-2.56909957998654));
#47735=CARTESIAN_POINT('Ctrl Pts',(16.2931762640366,44.610960536853,-2.60430551760671));
#47736=CARTESIAN_POINT('Ctrl Pts',(16.2760415418866,44.578285013538,-2.71150455640482));
#47737=CARTESIAN_POINT('Ctrl Pts',(16.2579866657359,44.5437398675915,-2.81767574143081));
#47738=CARTESIAN_POINT('Ctrl Pts',(16.2390566392221,44.507368577513,-2.92284842704556));
#47739=CARTESIAN_POINT('Ctrl Pts',(16.2320092324275,44.4938280113313,-2.96200287295586));
#47740=CARTESIAN_POINT('Ctrl Pts',(16.2248405515908,44.4800339777492,-3.0010187855979));
#47741=CARTESIAN_POINT('Ctrl Pts',(16.2175529061345,44.4659887626675,-3.03989765234625));
#47742=CARTESIAN_POINT('Ctrl Pts',(16.1988363578857,44.4299170372631,-3.13974858358623));
#47743=CARTESIAN_POINT('Ctrl Pts',(16.1793357237602,44.3921918998984,-3.23869700091219));
#47744=CARTESIAN_POINT('Ctrl Pts',(16.1590864494294,44.3528367566819,-3.33676146628663));
#47745=CARTESIAN_POINT('Ctrl Pts',(16.1309527334746,44.298157936961,-3.4730092038118));
#47746=CARTESIAN_POINT('Ctrl Pts',(16.1013735545187,44.2403372266431,-3.60755228756136));
#47747=CARTESIAN_POINT('Ctrl Pts',(16.0704438737352,44.1794272699162,-3.74043491721408));
#47748=CARTESIAN_POINT('Ctrl Pts',(16.0595449233439,44.1579639188604,-3.78725988118906));
#47749=CARTESIAN_POINT('Ctrl Pts',(16.0484783200874,44.1361163383025,-3.83387845461765));
#47750=CARTESIAN_POINT('Ctrl Pts',(16.0372481693921,44.113887257799,-3.88029266336609));
#47751=CARTESIAN_POINT('Ctrl Pts',(16.0166087396519,44.073033349629,-3.96559541899249));
#47752=CARTESIAN_POINT('Ctrl Pts',(15.9954165095932,44.0308907581977,-4.05020776137457));
#47753=CARTESIAN_POINT('Ctrl Pts',(15.9736952183765,43.9874629851133,-4.13413673701598));
#47754=CARTESIAN_POINT('Ctrl Pts',(15.9401551232136,43.9204056620733,-4.26373243194281));
#47755=CARTESIAN_POINT('Ctrl Pts',(15.905353150331,43.8502891232181,-4.39170062734481));
#47756=CARTESIAN_POINT('Ctrl Pts',(15.869376700399,43.777119676058,-4.51806349542216));
#47757=CARTESIAN_POINT('Ctrl Pts',(15.8538182611451,43.745476687352,-4.57271060514651));
#47758=CARTESIAN_POINT('Ctrl Pts',(15.8380402437097,43.7132618093626,-4.62705717641083));
#47759=CARTESIAN_POINT('Ctrl Pts',(15.822049652599,43.6804760856509,-4.68110508221071));
#47760=CARTESIAN_POINT('Ctrl Pts',(15.8027755650205,43.6409581650331,-4.74625114608124));
#47761=CARTESIAN_POINT('Ctrl Pts',(15.783192557801,43.6006087489436,-4.81096243631331));
#47762=CARTESIAN_POINT('Ctrl Pts',(15.7633127763008,43.5594253043274,-4.87524053934891));
#47763=CARTESIAN_POINT('Ctrl Pts',(15.7615479512871,43.555769249395,-4.88094681957486));
#47764=CARTESIAN_POINT('Ctrl Pts',(15.7597807873781,43.552106620627,-4.88664968554212));
#47765=CARTESIAN_POINT('Ctrl Pts',(15.7580112930854,43.548437415296,-4.89234913800578));
#47766=CARTESIAN_POINT('Ctrl Pts',(15.7498073372243,43.5314257760349,-4.91877366881019));
#47767=CARTESIAN_POINT('Ctrl Pts',(15.7415544292727,43.514275118157,-4.94512121020454));
#47768=CARTESIAN_POINT('Ctrl Pts',(15.7332502456038,43.4969785891754,-4.97140188570682));
#47769=CARTESIAN_POINT('Ctrl Pts',(15.7318779865615,43.494120352985,-4.9757447442022));
#47770=CARTESIAN_POINT('Ctrl Pts',(15.7305044376723,43.4912583615479,-4.98008541804862));
#47771=CARTESIAN_POINT('Ctrl Pts',(15.7291296393024,43.4883926909596,-4.98442379964834));
#47772=CARTESIAN_POINT('Ctrl Pts',(15.7203852640188,43.4701656551905,-5.01201798193912));
#47773=CARTESIAN_POINT('Ctrl Pts',(15.711597089659,43.4518037974615,-5.03949821938434));
#47774=CARTESIAN_POINT('Ctrl Pts',(15.7027746567282,43.4333249627762,-5.06684004878928));
#47775=CARTESIAN_POINT('Ctrl Pts',(15.701816203265,43.4313174549562,-5.06981041663333));
#47776=CARTESIAN_POINT('Ctrl Pts',(15.7008572951018,43.4293084622317,-5.07277931161621));
#47777=CARTESIAN_POINT('Ctrl Pts',(15.6998979279679,43.4272979728774,-5.07574675362532));
#47778=CARTESIAN_POINT('Ctrl Pts',(15.6803175074106,43.3862644355702,-5.13631143263322));
#47779=CARTESIAN_POINT('Ctrl Pts',(15.6605550261926,43.3446258030676,-5.19624268367425));
#47780=CARTESIAN_POINT('Ctrl Pts',(15.6406249503671,43.3023913589472,-5.25555493854259));
#47781=CARTESIAN_POINT('Ctrl Pts',(15.619858525843,43.2583845822638,-5.31735618179178));
#47782=CARTESIAN_POINT('Ctrl Pts',(15.598910322171,43.213730246343,-5.37848484512116));
#47783=CARTESIAN_POINT('Ctrl Pts',(15.5777971164023,43.1684369147297,-5.43895550636533));
#47784=CARTESIAN_POINT('Ctrl Pts',(15.5583845406235,43.1267918778816,-5.49455536678717));
#47785=CARTESIAN_POINT('Ctrl Pts',(15.5388325010489,43.0846079034054,-5.54960000848349));
#47786=CARTESIAN_POINT('Ctrl Pts',(15.5191535351483,43.0418879348754,-5.60409744798316));
#47787=CARTESIAN_POINT('Ctrl Pts',(15.4780716363702,42.9527055341427,-5.71786655071465));
#47788=CARTESIAN_POINT('Ctrl Pts',(15.4364351847114,42.8611928677454,-5.82925514163746));
#47789=CARTESIAN_POINT('Ctrl Pts',(15.3943559547313,42.7673817983009,-5.93833747396013));
#47790=CARTESIAN_POINT('Ctrl Pts',(15.3682783871389,42.7092446958513,-6.00593856589142));
#47791=CARTESIAN_POINT('Ctrl Pts',(15.3420312154126,42.6502231410027,-6.07265263288714));
#47792=CARTESIAN_POINT('Ctrl Pts',(15.3156411568502,42.5903237758893,-6.13849622909734));
#47793=CARTESIAN_POINT('Ctrl Pts',(15.2994477444082,42.553568452971,-6.17889903864669));
#47794=CARTESIAN_POINT('Ctrl Pts',(15.2832003544436,42.5164826160552,-6.21897402344193));
#47795=CARTESIAN_POINT('Ctrl Pts',(15.2669052552736,42.4790655001611,-6.25872313049107));
#47796=CARTESIAN_POINT('Ctrl Pts',(15.2240543808514,42.3806705092686,-6.363250508741));
#47797=CARTESIAN_POINT('Ctrl Pts',(15.1808723838033,42.2799892221281,-6.4655276503284));
#47798=CARTESIAN_POINT('Ctrl Pts',(15.1374702843923,42.1770158208016,-6.56559359303154));
#47799=CARTESIAN_POINT('Ctrl Pts',(15.1058399630617,42.1019714838535,-6.63851904974661));
#47800=CARTESIAN_POINT('Ctrl Pts',(15.0740932923155,42.0257078582054,-6.71026872409978));
#47801=CARTESIAN_POINT('Ctrl Pts',(15.0422738349374,41.948220165619,-6.78085524655767));
#47802=CARTESIAN_POINT('Ctrl Pts',(15.0304316665642,41.9193817636449,-6.80712525719604));
#47803=CARTESIAN_POINT('Ctrl Pts',(15.0185794677439,41.8903734206547,-6.83323385195918));
#47804=CARTESIAN_POINT('Ctrl Pts',(15.0067196161185,41.8611942483808,-6.85918119667358));
#47805=CARTESIAN_POINT('Ctrl Pts',(14.9722967908615,41.7765026704379,-6.93449250251397));
#47806=CARTESIAN_POINT('Ctrl Pts',(14.9378087380572,41.6903744753995,-7.00844713018512));
#47807=CARTESIAN_POINT('Ctrl Pts',(14.9033129588711,41.6027897699871,-7.0810495585008));
#47808=CARTESIAN_POINT('Ctrl Pts',(14.8939892424914,41.5791168751655,-7.10067295782853));
#47809=CARTESIAN_POINT('Ctrl Pts',(14.8846649774315,41.5553375106934,-7.12019752487661));
#47810=CARTESIAN_POINT('Ctrl Pts',(14.8753413457217,41.5314511178781,-7.13962322834019));
#47811=CARTESIAN_POINT('Ctrl Pts',(14.8643865713129,41.5033858689625,-7.16244740306092));
#47812=CARTESIAN_POINT('Ctrl Pts',(14.8534326525802,41.4751729344196,-7.18513513563339));
#47813=CARTESIAN_POINT('Ctrl Pts',(14.8424815052911,41.4468114212109,-7.20768636692352));
#47814=CARTESIAN_POINT('Ctrl Pts',(14.839526559386,41.4391586397165,-7.21377136119811));
#47815=CARTESIAN_POINT('Ctrl Pts',(14.8365718795728,41.4314952045087,-7.21984628480176));
#47816=CARTESIAN_POINT('Ctrl Pts',(14.8336174020316,41.4238208387543,-7.2259113453007));
#47817=CARTESIAN_POINT('Ctrl Pts',(14.8310971738157,41.4172744518406,-7.23108496276333));
#47818=CARTESIAN_POINT('Ctrl Pts',(14.8285769848935,41.4107198134149,-7.23625161312468));
#47819=CARTESIAN_POINT('Ctrl Pts',(14.8260571075248,41.4041575738866,-7.24141079712401));
#47820=CARTESIAN_POINT('Ctrl Pts',(14.8205831639148,41.3899023844958,-7.25261812119303));
#47821=CARTESIAN_POINT('Ctrl Pts',(14.8151098042831,41.3756089978122,-7.26379201309443));
#47822=CARTESIAN_POINT('Ctrl Pts',(14.8096438019145,41.3612944710306,-7.27491924106125));
#47823=CARTESIAN_POINT('Ctrl Pts',(14.806022034559,41.3518096808106,-7.28229213047671));
#47824=CARTESIAN_POINT('Ctrl Pts',(14.8024024578911,41.342312907149,-7.28964665424675));
#47825=CARTESIAN_POINT('Ctrl Pts',(14.7987860936221,41.3328066241553,-7.29698089316516));
#47826=CARTESIAN_POINT('Ctrl Pts',(14.787192400397,41.3023304551242,-7.32049371149171));
#47827=CARTESIAN_POINT('Ctrl Pts',(14.7756248165093,41.2717387024353,-7.34381230341903));
#47828=CARTESIAN_POINT('Ctrl Pts',(14.7640863609218,41.2410335710712,-7.36693653612173));
#47829=CARTESIAN_POINT('Ctrl Pts',(14.7574965735345,41.2234974037867,-7.38014313694009));
#47830=CARTESIAN_POINT('Ctrl Pts',(14.7509162585555,41.2059243753268,-7.39328652526075));
#47831=CARTESIAN_POINT('Ctrl Pts',(14.7443459874502,41.1883148488364,-7.40636660041844));
#47832=CARTESIAN_POINT('Ctrl Pts',(14.7010199283645,41.0721930978521,-7.49261998327614));
#47833=CARTESIAN_POINT('Ctrl Pts',(14.6581251019111,40.954469129494,-7.57613167115738));
#47834=CARTESIAN_POINT('Ctrl Pts',(14.6157752637112,40.8351450172988,-7.65696941752765));
#47835=CARTESIAN_POINT('Ctrl Pts',(14.5743516489294,40.7184306148866,-7.73603918043128));
#47836=CARTESIAN_POINT('Ctrl Pts',(14.5334494998714,40.6001850804501,-7.81255034269787));
#47837=CARTESIAN_POINT('Ctrl Pts',(14.4931826853823,40.4803989550325,-7.88654903288741));
#47838=CARTESIAN_POINT('Ctrl Pts',(14.4922823277783,40.4777205621614,-7.88820362822203));
#47839=CARTESIAN_POINT('Ctrl Pts',(14.4913822873103,40.4750413992675,-7.88985696731292));
#47840=CARTESIAN_POINT('Ctrl Pts',(14.4904825653626,40.47236146595,-7.89150905022655));
#47841=CARTESIAN_POINT('Ctrl Pts',(14.4493444574659,40.3498265136191,-7.96704745998726));
#47842=CARTESIAN_POINT('Ctrl Pts',(14.408872387569,40.2256806345653,-8.03995982187575));
#47843=CARTESIAN_POINT('Ctrl Pts',(14.3691870118136,40.0999011485163,-8.1102716271545));
#47844=CARTESIAN_POINT('Ctrl Pts',(14.3295016360582,39.9741216624673,-8.18058343243325));
#47845=CARTESIAN_POINT('Ctrl Pts',(14.2906028707937,39.846708554917,-8.24829461494413));
#47846=CARTESIAN_POINT('Ctrl Pts',(14.2526202581606,39.7176264034462,-8.31341191098604));
#47847=CARTESIAN_POINT('Ctrl Pts',(14.248137967391,39.7023935456742,-8.32109633906382));
#47848=CARTESIAN_POINT('Ctrl Pts',(14.2436684144369,39.6871374675747,-8.32874467778675));
#47849=CARTESIAN_POINT('Ctrl Pts',(14.2392118009553,39.6718581285822,-8.33635695538212));
#47850=CARTESIAN_POINT('Ctrl Pts',(14.2059033893122,39.557661437553,-8.39325057578117));
#47851=CARTESIAN_POINT('Ctrl Pts',(14.1733193051381,39.4421622806704,-8.44812547388581));
#47852=CARTESIAN_POINT('Ctrl Pts',(14.1415516469276,39.325327603003,-8.5009715729199));
#47853=CARTESIAN_POINT('Ctrl Pts',(14.1346399853956,39.2999079846639,-8.51246925233306));
#47854=CARTESIAN_POINT('Ctrl Pts',(14.1277670070846,39.2744250860744,-8.52387082842112));
#47855=CARTESIAN_POINT('Ctrl Pts',(14.1209336546232,39.2488785816658,-8.53517619746252));
#47856=CARTESIAN_POINT('Ctrl Pts',(14.0921569708267,39.1412968809374,-8.5827854832335));
#47857=CARTESIAN_POINT('Ctrl Pts',(14.0640830121568,39.032587235213,-8.62868866018023));
#47858=CARTESIAN_POINT('Ctrl Pts',(14.0367872922916,38.9227161423072,-8.67286593317823));
#47859=CARTESIAN_POINT('Ctrl Pts',(14.0277166460954,38.8862048571731,-8.68754649171477));
#47860=CARTESIAN_POINT('Ctrl Pts',(14.0187320348612,38.8495651717845,-8.70203629691729));
#47861=CARTESIAN_POINT('Ctrl Pts',(14.0098362084193,38.8127959120846,-8.71633463178559));
#47862=CARTESIAN_POINT('Ctrl Pts',(13.9856056306185,38.7126432827975,-8.75528063840029));
#47863=CARTESIAN_POINT('Ctrl Pts',(13.9620337294482,38.6115293995748,-8.79280618368359));
#47864=CARTESIAN_POINT('Ctrl Pts',(13.9391806731364,38.5094228580167,-8.82888688050722));
#47865=CARTESIAN_POINT('Ctrl Pts',(13.9313698855874,38.4745245716522,-8.84121865152567));
#47866=CARTESIAN_POINT('Ctrl Pts',(13.9236430764078,38.4395103239397,-8.85338162525871));
#47867=CARTESIAN_POINT('Ctrl Pts',(13.9160027405551,38.4043787548999,-8.8653746637582));
#47868=CARTESIAN_POINT('Ctrl Pts',(13.9130052106185,38.390595600344,-8.87007988779891));
#47869=CARTESIAN_POINT('Ctrl Pts',(13.910020831446,38.3767936600104,-8.87475920513983));
#47870=CARTESIAN_POINT('Ctrl Pts',(13.9070497732776,38.3629729696956,-8.87941251455177));
#47871=CARTESIAN_POINT('Ctrl Pts',(13.9024479688811,38.3415664169289,-8.88661991962326));
#47872=CARTESIAN_POINT('Ctrl Pts',(13.8978835001752,38.3201396295624,-8.89375650346339));
#47873=CARTESIAN_POINT('Ctrl Pts',(13.8933570138086,38.2986941565034,-8.90082193318904));
#47874=CARTESIAN_POINT('Ctrl Pts',(13.8817723344466,38.243808554508,-8.91890455429896));
#47875=CARTESIAN_POINT('Ctrl Pts',(13.8704362542691,38.1887995487795,-8.93652141653211));
#47876=CARTESIAN_POINT('Ctrl Pts',(13.8593562640666,38.1336760029268,-8.95367209281636));
#47877=CARTESIAN_POINT('Ctrl Pts',(13.85618744769,38.1179109714023,-8.95857709208856));
#47878=CARTESIAN_POINT('Ctrl Pts',(13.8530394321209,38.1021358845332,-8.96344418765362));
#47879=CARTESIAN_POINT('Ctrl Pts',(13.8499123051586,38.0863505151219,-8.96827348830095));
#47880=CARTESIAN_POINT('Ctrl Pts',(13.8378223340655,38.0253217618366,-8.98694433407386));
#47881=CARTESIAN_POINT('Ctrl Pts',(13.8260460707125,37.9641458211664,-9.00504796639664));
#47882=CARTESIAN_POINT('Ctrl Pts',(13.8145911106071,37.9028221956007,-9.02258679352785));
#47883=CARTESIAN_POINT('Ctrl Pts',(13.7994004865694,37.8214998573276,-9.04584534061672));
#47884=CARTESIAN_POINT('Ctrl Pts',(13.7847749381894,37.7399183242153,-9.06811310342971));
#47885=CARTESIAN_POINT('Ctrl Pts',(13.7707320465202,37.6580753553695,-9.08939044769318));
#47886=CARTESIAN_POINT('Ctrl Pts',(13.7460996778528,37.5145161633648,-9.12671263179219));
#47887=CARTESIAN_POINT('Ctrl Pts',(13.7232576460597,37.3701536907579,-9.16099116468723));
#47888=CARTESIAN_POINT('Ctrl Pts',(13.702299523627,37.2249766791102,-9.19222897002465));
#47889=CARTESIAN_POINT('Ctrl Pts',(13.689764940887,37.1381495661241,-9.21091160044037));
#47890=CARTESIAN_POINT('Ctrl Pts',(13.677905036562,37.0510307339763,-9.22850534417129));
#47891=CARTESIAN_POINT('Ctrl Pts',(13.666739988455,36.9636177322509,-9.24501044282744));
#47892=CARTESIAN_POINT('Ctrl Pts',(13.6592368088238,36.9048741023298,-9.25610226427426));
#47893=CARTESIAN_POINT('Ctrl Pts',(13.6520474529696,36.845997636278,-9.26670251302155));
#47894=CARTESIAN_POINT('Ctrl Pts',(13.6451779510603,36.7869869886694,-9.27680829891729));
#47895=CARTESIAN_POINT('Ctrl Pts',(13.6280863402507,36.6401660057417,-9.30195192093463));
#47896=CARTESIAN_POINT('Ctrl Pts',(13.6129724662781,36.492515433864,-9.32403804535087));
#47897=CARTESIAN_POINT('Ctrl Pts',(13.5999250865708,36.3440166675744,-9.34302753896882));
#47898=CARTESIAN_POINT('Ctrl Pts',(13.5898455510966,36.229296423642,-9.35769755539006));
#47899=CARTESIAN_POINT('Ctrl Pts',(13.5810002995574,36.114069533427,-9.37051802455725));
#47900=CARTESIAN_POINT('Ctrl Pts',(13.5734319623329,35.9983267443972,-9.38146815610025));
#47901=CARTESIAN_POINT('Ctrl Pts',(13.5712035217423,35.9642471412434,-9.38469234086887));
#47902=CARTESIAN_POINT('Ctrl Pts',(13.5690857701538,35.9301227262426,-9.38775395342427));
#47903=CARTESIAN_POINT('Ctrl Pts',(13.5670797784949,35.8959531945743,-9.39065210232899));
#47904=CARTESIAN_POINT('Ctrl Pts',(13.5642827085755,35.8483086449258,-9.39469315857526));
#47905=CARTESIAN_POINT('Ctrl Pts',(13.5617027314333,35.8005764620705,-9.39841668469839));
#47906=CARTESIAN_POINT('Ctrl Pts',(13.5593426708374,35.7527558543533,-9.40182037346003));
#47907=CARTESIAN_POINT('Ctrl Pts',(13.5579822327385,35.7251900466087,-9.40378240268769));
#47908=CARTESIAN_POINT('Ctrl Pts',(13.5566948689149,35.697594853584,-9.4056381399649));
#47909=CARTESIAN_POINT('Ctrl Pts',(13.5554811164538,35.669970111593,-9.40738708330099));
#47910=CARTESIAN_POINT('Ctrl Pts',(13.5548859234267,35.6564236477657,-9.40824472018485));
#47911=CARTESIAN_POINT('Ctrl Pts',(13.5543085108019,35.6428719569098,-9.40907656239463));
#47912=CARTESIAN_POINT('Ctrl Pts',(13.5537488650355,35.6293134090097,-9.40988266151869));
#47913=CARTESIAN_POINT('Ctrl Pts',(13.5527479600881,35.6050644671116,-9.41132433882568));
#47914=CARTESIAN_POINT('Ctrl Pts',(13.5518034882189,35.5807810331349,-9.41268424408725));
#47915=CARTESIAN_POINT('Ctrl Pts',(13.5509164078193,35.5564825681396,-9.41396115050902));
#47916=CARTESIAN_POINT('Ctrl Pts',(13.550295559802,35.5394766081131,-9.4148548291661));
#47917=CARTESIAN_POINT('Ctrl Pts',(13.5497028741862,35.5224643640414,-9.41570777996314));
#47918=CARTESIAN_POINT('Ctrl Pts',(13.5491389538032,35.5054603497194,-9.41651918760508));
#47919=CARTESIAN_POINT('Ctrl Pts',(13.5490747427451,35.5035241796801,-9.41661157891552));
#47920=CARTESIAN_POINT('Ctrl Pts',(13.5490109040932,35.5015881247004,-9.41670343285821));
#47921=CARTESIAN_POINT('Ctrl Pts',(13.5489474379496,35.499652191645,-9.41679474932162));
#47922=CARTESIAN_POINT('Ctrl Pts',(13.5483265934797,35.4807143255304,-9.41768803380448));
#47923=CARTESIAN_POINT('Ctrl Pts',(13.5477412466006,35.4617829285047,-9.41853009944171));
#47924=CARTESIAN_POINT('Ctrl Pts',(13.5471913035612,35.442857980976,-9.4193211140302));
#47925=CARTESIAN_POINT('Ctrl Pts',(13.5430022229461,35.2987009953143,-9.42534650873831));
#47926=CARTESIAN_POINT('Ctrl Pts',(13.5408674811866,35.1549181959707,-9.42840961630309));
#47927=CARTESIAN_POINT('Ctrl Pts',(13.5407592808403,35.0115034033078,-9.42856500737733));
#47928=CARTESIAN_POINT('Ctrl Pts',(13.5407538447441,35.0042980972761,-9.42857281438402));
#47929=CARTESIAN_POINT('Ctrl Pts',(13.5407535274295,34.9970937191213,-9.42857329535632));
#47930=CARTESIAN_POINT('Ctrl Pts',(13.5407583244004,34.9898902683715,-9.42856645346899));
#47931=CARTESIAN_POINT('Ctrl Pts',(13.5408586005346,34.8393089525897,-9.42842343029414));
#47932=CARTESIAN_POINT('Ctrl Pts',(13.5431955597245,34.6891331210029,-9.42507782600044));
#47933=CARTESIAN_POINT('Ctrl Pts',(13.5477229961778,34.5393569862264,-9.41856595336358));
#47934=CARTESIAN_POINT('Ctrl Pts',(13.5522504326312,34.3895808514499,-9.41205408072671));
#47935=CARTESIAN_POINT('Ctrl Pts',(13.5589683476105,34.2402044010644,-9.40237594907378));
#47936=CARTESIAN_POINT('Ctrl Pts',(13.5678384517885,34.0912233027804,-9.38955637262442));
#47937=CARTESIAN_POINT('Ctrl Pts',(13.5689885488583,34.0719064242919,-9.387894187264));
#47938=CARTESIAN_POINT('Ctrl Pts',(13.5701748380717,34.0525961922414,-9.38617917383737));
#47939=CARTESIAN_POINT('Ctrl Pts',(13.5713972196396,34.0332925947168,-9.38441140971383));
#47940=CARTESIAN_POINT('Ctrl Pts',(13.5796024352172,33.9037175231669,-9.37254532296499));
#47941=CARTESIAN_POINT('Ctrl Pts',(13.5894337323259,33.7744414510532,-9.35830230953036));
#47942=CARTESIAN_POINT('Ctrl Pts',(13.6008538043109,33.6454626048097,-9.34167733991798));
#47943=CARTESIAN_POINT('Ctrl Pts',(13.6139751948495,33.4972689844025,-9.32257564605289));
#47944=CARTESIAN_POINT('Ctrl Pts',(13.6291932512565,33.3494676061594,-9.30033053952966));
#47945=CARTESIAN_POINT('Ctrl Pts',(13.6464570722265,33.2020569656426,-9.27492584007278));
#47946=CARTESIAN_POINT('Ctrl Pts',(13.6517062465988,33.1572358244975,-9.26720137991093));
#47947=CARTESIAN_POINT('Ctrl Pts',(13.6571445977731,33.1124507933225,-9.25918474429875));
#47948=CARTESIAN_POINT('Ctrl Pts',(13.6627705971131,33.0677018138577,-9.25087561318739));
#47949=CARTESIAN_POINT('Ctrl Pts',(13.6728200500002,32.9877688572938,-9.23603341065783));
#47950=CARTESIAN_POINT('Ctrl Pts',(13.6834677371398,32.907951109785,-9.22025577061754));
#47951=CARTESIAN_POINT('Ctrl Pts',(13.6947039744194,32.8282485786631,-9.20353644274965));
#47952=CARTESIAN_POINT('Ctrl Pts',(13.6978656042632,32.8058220407795,-9.19883199190547));
#47953=CARTESIAN_POINT('Ctrl Pts',(13.7010738298154,32.7834046255516,-9.19405297520816));
#47954=CARTESIAN_POINT('Ctrl Pts',(13.704328429154,32.7609963352982,-9.18919922232318));
#47955=CARTESIAN_POINT('Ctrl Pts',(13.7068555947766,32.7435965097287,-9.18543032908765));
#47956=CARTESIAN_POINT('Ctrl Pts',(13.7094107324537,32.7262021023487,-9.18161635742941));
#47957=CARTESIAN_POINT('Ctrl Pts',(13.7119938175221,32.7088126084929,-9.17775710880594));
#47958=CARTESIAN_POINT('Ctrl Pts',(13.7148526957193,32.689566457659,-9.17348581248596));
#47959=CARTESIAN_POINT('Ctrl Pts',(13.717746213636,32.670324099751,-9.16915843765454));
#47960=CARTESIAN_POINT('Ctrl Pts',(13.7206719802958,32.6510994569933,-9.16477824576685));
#47961=CARTESIAN_POINT('Ctrl Pts',(13.7237925263614,32.6305949567047,-9.16010644785847));
#47962=CARTESIAN_POINT('Ctrl Pts',(13.7269492160484,32.6101141402426,-9.15537537818358));
#47963=CARTESIAN_POINT('Ctrl Pts',(13.7301396445541,32.5896707038453,-9.15058825109336));
#47964=CARTESIAN_POINT('Ctrl Pts',(13.7326432238633,32.5736284185275,-9.14683171735109));
#47965=CARTESIAN_POINT('Ctrl Pts',(13.735168271931,32.557604298108,-9.14303964568289));
#47966=CARTESIAN_POINT('Ctrl Pts',(13.7377149247936,32.5415963237026,-9.13921163623647));
#47967=CARTESIAN_POINT('Ctrl Pts',(13.7492988688276,32.4687809501066,-9.12179919348068));
#47968=CARTESIAN_POINT('Ctrl Pts',(13.761323702081,32.3963376875117,-9.10365238666682));
#47969=CARTESIAN_POINT('Ctrl Pts',(13.7737713161574,32.3242591214252,-9.08478005398837));
#47970=CARTESIAN_POINT('Ctrl Pts',(13.7855758014131,32.2559046267088,-9.0668827950056));
#47971=CARTESIAN_POINT('Ctrl Pts',(13.7977609475819,32.187878518565,-9.04833238126448));
#47972=CARTESIAN_POINT('Ctrl Pts',(13.8103118541531,32.1201748608641,-9.02913542323162));
#47973=CARTESIAN_POINT('Ctrl Pts',(13.8242303510202,32.0450939778811,-9.00784669809264));
#47974=CARTESIAN_POINT('Ctrl Pts',(13.8385981219998,31.9704087713137,-8.98576461959821));
#47975=CARTESIAN_POINT('Ctrl Pts',(13.8533964756602,31.8961139063031,-8.96289268199796));
#47976=CARTESIAN_POINT('Ctrl Pts',(13.8815391405615,31.7548241697653,-8.91939613567287));
#47977=CARTESIAN_POINT('Ctrl Pts',(13.9112357191329,31.6149430430769,-8.87304823794877));
#47978=CARTESIAN_POINT('Ctrl Pts',(13.9423542403051,31.4764299357821,-8.82387705704306));
#47979=CARTESIAN_POINT('Ctrl Pts',(13.9621098348215,31.3884948836058,-8.79266073071149));
#47980=CARTESIAN_POINT('Ctrl Pts',(13.9824396027645,31.3011122143628,-8.76030478122907));
#47981=CARTESIAN_POINT('Ctrl Pts',(14.0033100035835,31.2142716336085,-8.7268155098858));
#47982=CARTESIAN_POINT('Ctrl Pts',(14.0153141390999,31.1643230912332,-8.70755331386777));
#47983=CARTESIAN_POINT('Ctrl Pts',(14.0274972073736,31.1145539360271,-8.68791611827075));
#47984=CARTESIAN_POINT('Ctrl Pts',(14.039853406829,31.0649633164737,-8.66790286279505));
#47985=CARTESIAN_POINT('Ctrl Pts',(14.0736921057848,30.9291544011065,-8.61309454332662));
#47986=CARTESIAN_POINT('Ctrl Pts',(14.10882687604,30.7946821312524,-8.55546981872774));
#47987=CARTESIAN_POINT('Ctrl Pts',(14.1451333866133,30.6615234073939,-8.49501412466315));
#47988=CARTESIAN_POINT('Ctrl Pts',(14.1736757128249,30.5568408126122,-8.44748694251072));
#47989=CARTESIAN_POINT('Ctrl Pts',(14.2029432110629,30.4529709991461,-8.39820846486423));
#47990=CARTESIAN_POINT('Ctrl Pts',(14.2328774579981,30.3499044844853,-8.34716714015086));
#47991=CARTESIAN_POINT('Ctrl Pts',(14.2410202775501,30.3218679672295,-8.33328269877051));
#47992=CARTESIAN_POINT('Ctrl Pts',(14.2492125117705,30.2938910607097,-8.31926745952062));
#47993=CARTESIAN_POINT('Ctrl Pts',(14.2574530348856,30.2659737110311,-8.30512090606144));
#47994=CARTESIAN_POINT('Ctrl Pts',(14.2670865206991,30.2333372644947,-8.28858304552095));
#47995=CARTESIAN_POINT('Ctrl Pts',(14.2767858699329,30.2007820737878,-8.27186594876041));
#47996=CARTESIAN_POINT('Ctrl Pts',(14.2865492521489,30.1683080065208,-8.25496883936316));
#47997=CARTESIAN_POINT('Ctrl Pts',(14.2893829928678,30.1588826778092,-8.25006459349105));
#47998=CARTESIAN_POINT('Ctrl Pts',(14.292222325135,30.1494635276478,-8.24514484143581));
#47999=CARTESIAN_POINT('Ctrl Pts',(14.2950670737642,30.1400509907427,-8.24020978838424));
#48000=CARTESIAN_POINT('Ctrl Pts',(14.3020236340514,30.1170335333246,-8.2281415888526));
#48001=CARTESIAN_POINT('Ctrl Pts',(14.3090108870272,30.0940614536975,-8.2159847713543));
#48002=CARTESIAN_POINT('Ctrl Pts',(14.3160202505588,30.0711599081366,-8.20375303932115));
#48003=CARTESIAN_POINT('Ctrl Pts',(14.3195972339208,30.0594729058764,-8.19751100296879));
#48004=CARTESIAN_POINT('Ctrl Pts',(14.3231806312391,30.0478021255475,-8.19124831435603));
#48005=CARTESIAN_POINT('Ctrl Pts',(14.3267695230049,30.0361502051769,-8.18496640400546));
#48006=CARTESIAN_POINT('Ctrl Pts',(14.3373838140425,30.00168918433,-8.1663874027196));
#48007=CARTESIAN_POINT('Ctrl Pts',(14.3480518032559,29.9673744337054,-8.14763050023152));
#48008=CARTESIAN_POINT('Ctrl Pts',(14.3587697894377,29.9332076692579,-8.12869793595085));
#48009=CARTESIAN_POINT('Ctrl Pts',(14.3644386177442,29.9151365952559,-8.11868435182325));
#48010=CARTESIAN_POINT('Ctrl Pts',(14.3701214124312,29.8971068793201,-8.10862166579222));
#48011=CARTESIAN_POINT('Ctrl Pts',(14.3758176419001,29.879118802236,-8.09851018473152));
#48012=CARTESIAN_POINT('Ctrl Pts',(14.4131276182726,29.7612979288577,-8.03228056362499));
#48013=CARTESIAN_POINT('Ctrl Pts',(14.4510196947368,29.6452440596771,-7.96394759139418));
#48014=CARTESIAN_POINT('Ctrl Pts',(14.4893852619753,29.5309085105395,-7.89352359406489));
#48015=CARTESIAN_POINT('Ctrl Pts',(14.4923724608226,29.5220061784439,-7.88804027923891));
#48016=CARTESIAN_POINT('Ctrl Pts',(14.4953625194179,29.5131142368237,-7.88254431476432));
#48017=CARTESIAN_POINT('Ctrl Pts',(14.4983553912906,29.5042326741083,-7.8770356952244));
#48018=CARTESIAN_POINT('Ctrl Pts',(14.5397866909133,29.3812823101657,-7.80077808167639));
#48019=CARTESIAN_POINT('Ctrl Pts',(14.5817591054257,29.2603242335815,-7.72209176784764));
#48020=CARTESIAN_POINT('Ctrl Pts',(14.6241433376865,29.1413144445618,-7.64097208577998));
#48021=CARTESIAN_POINT('Ctrl Pts',(14.6665275699472,29.022304655542,-7.55985240371234));
#48022=CARTESIAN_POINT('Ctrl Pts',(14.7093237189971,28.9052431377277,-7.47629941382632));
#48023=CARTESIAN_POINT('Ctrl Pts',(14.7524104879707,28.7901025279864,-7.39028991647064));
#48024=CARTESIAN_POINT('Ctrl Pts',(14.7549211635545,28.783393259121,-7.38527812398457));
#48025=CARTESIAN_POINT('Ctrl Pts',(14.7574328257359,28.7766905125821,-7.38025798958));
#48026=CARTESIAN_POINT('Ctrl Pts',(14.7599454485781,28.7699942792284,-7.37522951202236));
#48027=CARTESIAN_POINT('Ctrl Pts',(14.8005530124361,28.6617736107886,-7.29396215263163));
#48028=CARTESIAN_POINT('Ctrl Pts',(14.8414126162536,28.5552547310724,-7.2105156873878));
#48029=CARTESIAN_POINT('Ctrl Pts',(14.8824237170485,28.4504289161673,-7.12485201694789));
#48030=CARTESIAN_POINT('Ctrl Pts',(14.9259724098299,28.3391169269646,-7.03388784397486));
#48031=CARTESIAN_POINT('Ctrl Pts',(14.969691679003,28.2297133004615,-6.94042438590296));
#48032=CARTESIAN_POINT('Ctrl Pts',(15.0134672850339,28.1222220970918,-6.84439955098032));
#48033=CARTESIAN_POINT('Ctrl Pts',(15.0212656977202,28.1030730586198,-6.82729319064052));
#48034=CARTESIAN_POINT('Ctrl Pts',(15.0290658824068,28.0839846740001,-6.81010556361074));
#48035=CARTESIAN_POINT('Ctrl Pts',(15.0368671643906,28.0649569085011,-6.79283636491335));
#48036=CARTESIAN_POINT('Ctrl Pts',(15.0728575949509,27.9771742242786,-6.71316665192975));
#48037=CARTESIAN_POINT('Ctrl Pts',(15.108872128155,27.8906849392576,-6.63175735053518));
#48038=CARTESIAN_POINT('Ctrl Pts',(15.1448458274244,27.8055007475085,-6.54856071175149));
#48039=CARTESIAN_POINT('Ctrl Pts',(15.1550957132048,27.7812294533839,-6.52485572554879));
#48040=CARTESIAN_POINT('Ctrl Pts',(15.1653425249988,27.7570636708736,-6.50100506088306));
#48041=CARTESIAN_POINT('Ctrl Pts',(15.1755841559372,27.7330051752369,-6.47700899536732));
#48042=CARTESIAN_POINT('Ctrl Pts',(15.1762765507258,27.7313786787247,-6.47538671950028));
#48043=CARTESIAN_POINT('Ctrl Pts',(15.176968933695,27.7297526458408,-6.47376374952505));
#48044=CARTESIAN_POINT('Ctrl Pts',(15.1776612975255,27.7281270926064,-6.47214010149995));
#48045=CARTESIAN_POINT('Ctrl Pts',(15.1884972135519,27.7026861935163,-6.44672902009784));
#48046=CARTESIAN_POINT('Ctrl Pts',(15.1993295170106,27.6773601866701,-6.42114932420259));
#48047=CARTESIAN_POINT('Ctrl Pts',(15.2101297653433,27.6522113320498,-6.39546343288883));
#48048=CARTESIAN_POINT('Ctrl Pts',(15.2102270648348,27.6519847658921,-6.3952320285649));
#48049=CARTESIAN_POINT('Ctrl Pts',(15.2103243621927,27.6517582130066,-6.39500061453552));
#48050=CARTESIAN_POINT('Ctrl Pts',(15.2104216574152,27.6515316733944,-6.39476919080245));
#48051=CARTESIAN_POINT('Ctrl Pts',(15.2218073439199,27.6250215432897,-6.36768751085094));
#48052=CARTESIAN_POINT('Ctrl Pts',(15.233164174659,27.5986923805235,-6.34047202426355));
#48053=CARTESIAN_POINT('Ctrl Pts',(15.2444901971976,27.5725432631787,-6.31312273186159));
#48054=CARTESIAN_POINT('Ctrl Pts',(15.2548441070592,27.5486385249507,-6.28812082961882));
#48055=CARTESIAN_POINT('Ctrl Pts',(15.2651722657739,27.5248842285587,-6.26300711771079));
#48056=CARTESIAN_POINT('Ctrl Pts',(15.2754732056469,27.5012797929199,-6.23778152604866));
#48057=CARTESIAN_POINT('Ctrl Pts',(15.287880939932,27.4728476722624,-6.2073966832686));
#48058=CARTESIAN_POINT('Ctrl Pts',(15.3002492612591,27.4446333351571,-6.17684932533396));
#48059=CARTESIAN_POINT('Ctrl Pts',(15.3125756070521,27.4166357721296,-6.14613929864308));
#48060=CARTESIAN_POINT('Ctrl Pts',(15.3431043357434,27.3472940531772,-6.0700796059574));
#48061=CARTESIAN_POINT('Ctrl Pts',(15.3733751765106,27.2792782283333,-5.99302430475968));
#48062=CARTESIAN_POINT('Ctrl Pts',(15.4033505610025,27.2125834223929,-5.91496498170904));
#48063=CARTESIAN_POINT('Ctrl Pts',(15.4454288718318,27.1189597767709,-5.80538825686893));
#48064=CARTESIAN_POINT('Ctrl Pts',(15.4869241736851,27.0279350941902,-5.69383535682826));
#48065=CARTESIAN_POINT('Ctrl Pts',(15.5277334515159,26.9395021548202,-5.58027802205931));
#48066=CARTESIAN_POINT('Ctrl Pts',(15.5435349373662,26.9052606314599,-5.53630825062664));
#48067=CARTESIAN_POINT('Ctrl Pts',(15.5592336972788,26.871408433392,-5.49203755996307));
#48068=CARTESIAN_POINT('Ctrl Pts',(15.574823623311,26.8379446654303,-5.44746446549149));
#48069=CARTESIAN_POINT('Ctrl Pts',(15.5994965958972,26.7849841428569,-5.37692206935047));
#48070=CARTESIAN_POINT('Ctrl Pts',(15.6238973986934,26.7329965873824,-5.30562234479574));
#48071=CARTESIAN_POINT('Ctrl Pts',(15.6480018369203,26.6819887826648,-5.23355301636256));
#48072=CARTESIAN_POINT('Ctrl Pts',(15.6873369656403,26.5987510591629,-5.11594578220904));
#48073=CARTESIAN_POINT('Ctrl Pts',(15.7258820530778,26.5181175702425,-4.99629189854525));
#48074=CARTESIAN_POINT('Ctrl Pts',(15.7635321084066,26.4401221421386,-4.87453424819488));
#48075=CARTESIAN_POINT('Ctrl Pts',(15.7814963336588,26.4029076566122,-4.81643919792282));
#48076=CARTESIAN_POINT('Ctrl Pts',(15.799257015528,26.3662951462581,-4.7578644141531));
#48077=CARTESIAN_POINT('Ctrl Pts',(15.8168026043343,26.3302880236965,-4.69880361108633));
#48078=CARTESIAN_POINT('Ctrl Pts',(15.8360296778645,26.290830151935,-4.63408270511698));
#48079=CARTESIAN_POINT('Ctrl Pts',(15.8549987958215,26.252099025531,-4.56877841580672));
#48080=CARTESIAN_POINT('Ctrl Pts',(15.8736935430838,26.2141060677325,-4.5028778267482));
#48081=CARTESIAN_POINT('Ctrl Pts',(15.9094481069526,26.1414427887319,-4.37683991955305));
#48082=CARTESIAN_POINT('Ctrl Pts',(15.9441982142166,26.071473598024,-4.2486243383595));
#48083=CARTESIAN_POINT('Ctrl Pts',(15.9778282576488,26.0042788083171,-4.11813863898061));
#48084=CARTESIAN_POINT('Ctrl Pts',(15.99657064445,25.9668304255266,-4.04541754795051));
#48085=CARTESIAN_POINT('Ctrl Pts',(16.0149654186617,25.9302457759999,-3.97199016296204));
#48086=CARTESIAN_POINT('Ctrl Pts',(16.0329923372658,25.8945387960944,-3.89784000610498));
#48087=CARTESIAN_POINT('Ctrl Pts',(16.0473116754131,25.8661756392668,-3.83894024663796));
#48088=CARTESIAN_POINT('Ctrl Pts',(16.0613984893021,25.8383679468724,-3.77958327653742));
#48089=CARTESIAN_POINT('Ctrl Pts',(16.0752417085548,25.8111258267813,-3.71975861341477));
#48090=CARTESIAN_POINT('Ctrl Pts',(16.0776115084942,25.8064622891054,-3.70951731907025));
#48091=CARTESIAN_POINT('Ctrl Pts',(16.0799740221123,25.8018156156547,-3.69926296026429));
#48092=CARTESIAN_POINT('Ctrl Pts',(16.082329545527,25.7971851587797,-3.68899395351471));
#48093=CARTESIAN_POINT('Ctrl Pts',(16.0838593165519,25.7941779550665,-3.68232485021419));
#48094=CARTESIAN_POINT('Ctrl Pts',(16.0853860612706,25.7911777468393,-3.67564986683594));
#48095=CARTESIAN_POINT('Ctrl Pts',(16.0869097019712,25.7881846675679,-3.66896929579596));
#48096=CARTESIAN_POINT('Ctrl Pts',(16.0907794266855,25.7805828800706,-3.65200206011619));
#48097=CARTESIAN_POINT('Ctrl Pts',(16.0946280676787,25.7730291844909,-3.63500339665168));
#48098=CARTESIAN_POINT('Ctrl Pts',(16.0984513321492,25.7655317108836,-3.61799165083566));
#48099=CARTESIAN_POINT('Ctrl Pts',(16.1010438385578,25.760447770569,-3.60645620504334));
#48100=CARTESIAN_POINT('Ctrl Pts',(16.1036256032075,25.7553878660265,-3.5949106355367));
#48101=CARTESIAN_POINT('Ctrl Pts',(16.1061956520486,25.7503538215281,-3.58335898535595));
#48102=CARTESIAN_POINT('Ctrl Pts',(16.1112058941486,25.7405400851994,-3.56083934949041));
#48103=CARTESIAN_POINT('Ctrl Pts',(16.1161742261471,25.7308194838903,-3.53828527581221));
#48104=CARTESIAN_POINT('Ctrl Pts',(16.1210997272461,25.7211931674899,-3.51569958736613));
#48105=CARTESIAN_POINT('Ctrl Pts',(16.1238878355848,25.7157441355057,-3.50291482800349));
#48106=CARTESIAN_POINT('Ctrl Pts',(16.1266622680174,25.7103252359564,-3.4901197249234));
#48107=CARTESIAN_POINT('Ctrl Pts',(16.1294229723656,25.7049364454398,-3.4773142766403));
#48108=CARTESIAN_POINT('Ctrl Pts',(16.1414199393083,25.6815188195244,-3.42166668806785));
#48109=CARTESIAN_POINT('Ctrl Pts',(16.1531576830853,25.6586694316974,-3.36582381852307));
#48110=CARTESIAN_POINT('Ctrl Pts',(16.1646318524645,25.6363874743175,-3.30978527491759));
#48111=CARTESIAN_POINT('Ctrl Pts',(16.1823179306242,25.6020424662609,-3.22340847243103));
#48112=CARTESIAN_POINT('Ctrl Pts',(16.1993778298018,25.569046127284,-3.13656665175364));
#48113=CARTESIAN_POINT('Ctrl Pts',(16.2157956548538,25.5373983162666,-3.04925749651258));
#48114=CARTESIAN_POINT('Ctrl Pts',(16.2255826815076,25.5185323599673,-2.99721058854791));
#48115=CARTESIAN_POINT('Ctrl Pts',(16.2351416656231,25.500144713963,-2.94499782115509));
#48116=CARTESIAN_POINT('Ctrl Pts',(16.2444690004062,25.4822373725231,-2.89261825720388));
#48117=CARTESIAN_POINT('Ctrl Pts',(16.2694430230024,25.4342903050961,-2.7523715046085));
#48118=CARTESIAN_POINT('Ctrl Pts',(16.2927563240971,25.3897821894178,-2.61092958676889));
#48119=CARTESIAN_POINT('Ctrl Pts',(16.3143388732363,25.3487423680397,-2.46827426826731));
#48120=CARTESIAN_POINT('Ctrl Pts',(16.3290674062958,25.320735650111,-2.37092230297782));
#48121=CARTESIAN_POINT('Ctrl Pts',(16.3429899648793,25.2943464232017,-2.27300479163498));
#48122=CARTESIAN_POINT('Ctrl Pts',(16.3560840754507,25.2695873114563,-2.1745145933834));
#48123=CARTESIAN_POINT('Ctrl Pts',(16.3621775026809,25.2580655020991,-2.12868155625828));
#48124=CARTESIAN_POINT('Ctrl Pts',(16.36809158417,25.2468966669633,-2.08272451927544));
#48125=CARTESIAN_POINT('Ctrl Pts',(16.3738237295954,25.2360837950792,-2.03664236952968));
#48126=CARTESIAN_POINT('Ctrl Pts',(16.3918736303947,25.2020352407632,-1.89153470567869));
#48127=CARTESIAN_POINT('Ctrl Pts',(16.4081195618896,25.1715109887614,-1.74518744974002));
#48128=CARTESIAN_POINT('Ctrl Pts',(16.422479453318,25.1445929873555,-1.59756606226281));
#48129=CARTESIAN_POINT('Ctrl Pts',(16.4328873816435,25.1250830467201,-1.49057132432628));
#48130=CARTESIAN_POINT('Ctrl Pts',(16.4423045573777,25.1074701737894,-1.38290671322239));
#48131=CARTESIAN_POINT('Ctrl Pts',(16.4506992102471,25.0917907162153,-1.27455697949911));
#48132=CARTESIAN_POINT('Ctrl Pts',(16.4538867185929,25.0858371166259,-1.23341582859115));
#48133=CARTESIAN_POINT('Ctrl Pts',(16.4569266867854,25.0801628066784,-1.19217577139639));
#48134=CARTESIAN_POINT('Ctrl Pts',(16.4598171317225,25.0747707396732,-1.15083574514861));
#48135=CARTESIAN_POINT('Ctrl Pts',(16.4611299753143,25.0723216563077,-1.13205905514945));
#48136=CARTESIAN_POINT('Ctrl Pts',(16.462411971524,25.0699307471454,-1.11326175181383));
#48137=CARTESIAN_POINT('Ctrl Pts',(16.4636629333543,25.0675982499494,-1.09444373942888));
#48138=CARTESIAN_POINT('Ctrl Pts',(16.4649138951847,25.0652657527534,-1.0756257270439));
#48139=CARTESIAN_POINT('Ctrl Pts',(16.4661340498209,25.0629912442797,-1.05678322505441));
#48140=CARTESIAN_POINT('Ctrl Pts',(16.4673219194188,25.0607773949756,-1.03793713672155));
#48141=CARTESIAN_POINT('Ctrl Pts',(16.4696976586148,25.0563496963676,-1.00024496005579));
#48142=CARTESIAN_POINT('Ctrl Pts',(16.4719451548503,25.0521629702833,-0.962525713485337));
#48143=CARTESIAN_POINT('Ctrl Pts',(16.4740640279585,25.0482172985549,-0.924779372504798));
#48144=CARTESIAN_POINT('Ctrl Pts',(16.4761199328798,25.0443888833974,-0.888154768660442));
#48145=CARTESIAN_POINT('Ctrl Pts',(16.4780547473837,25.0407875238464,-0.851504629468));
#48146=CARTESIAN_POINT('Ctrl Pts',(16.4798681346825,25.0374132198755,-0.814828978053869));
#48147=CARTESIAN_POINT('Ctrl Pts',(16.4817926027118,25.0338322197672,-0.77590672540095));
#48148=CARTESIAN_POINT('Ctrl Pts',(16.4835802779039,25.0305070766299,-0.736955706434156));
#48149=CARTESIAN_POINT('Ctrl Pts',(16.4852306641202,25.0274381872021,-0.697975849237231));
#48150=CARTESIAN_POINT('Ctrl Pts',(16.4868334200033,25.0244578662707,-0.660120955133343));
#48151=CARTESIAN_POINT('Ctrl Pts',(16.4883066964389,25.0217191663817,-0.622238876861686));
#48152=CARTESIAN_POINT('Ctrl Pts',(16.4896500561993,25.0192225741471,-0.584329551221999));
#48153=CARTESIAN_POINT('Ctrl Pts',(16.489672264156,25.0191813013518,-0.58370284742364));
#48154=CARTESIAN_POINT('Ctrl Pts',(16.4896944360742,25.0191400957001,-0.583076151230041));
#48155=CARTESIAN_POINT('Ctrl Pts',(16.4897165719879,25.0190989571266,-0.582449461762879));
#48156=CARTESIAN_POINT('Ctrl Pts',(16.4904036405537,25.0178220719222,-0.562997875556125));
#48157=CARTESIAN_POINT('Ctrl Pts',(16.4910560498663,25.0166097642747,-0.543552782867375));
#48158=CARTESIAN_POINT('Ctrl Pts',(16.4916746257547,25.0154604569063,-0.524087815387606));
#48159=CARTESIAN_POINT('Ctrl Pts',(16.4922416397358,25.0144069510089,-0.506245366450441));
#48160=CARTESIAN_POINT('Ctrl Pts',(16.4927805500429,25.0134057777586,-0.488373007878846));
#48161=CARTESIAN_POINT('Ctrl Pts',(16.4932898396429,25.0124597261385,-0.470521203664524));
#48162=CARTESIAN_POINT('Ctrl Pts',(16.4933360446607,25.0123738961275,-0.468901608581097));
#48163=CARTESIAN_POINT('Ctrl Pts',(16.4933820019059,25.012288527186,-0.467282315369493));
#48164=CARTESIAN_POINT('Ctrl Pts',(16.493427709802,25.0122036222164,-0.465663377919828));
#48165=CARTESIAN_POINT('Ctrl Pts',(16.4945251650366,25.0101650378337,-0.426792383474895));
#48166=CARTESIAN_POINT('Ctrl Pts',(16.4954849227943,25.0083826845251,-0.387926620808362));
#48167=CARTESIAN_POINT('Ctrl Pts',(16.4963070000775,25.0068562319132,-0.349077869818753));
#48168=CARTESIAN_POINT('Ctrl Pts',(16.4970554181005,25.0054665515637,-0.313710020579238));
#48169=CARTESIAN_POINT('Ctrl Pts',(16.4976897549768,25.0042888272114,-0.278356255691909));
#48170=CARTESIAN_POINT('Ctrl Pts',(16.498210217178,25.0033226005218,-0.243025431918962));
#48171=CARTESIAN_POINT('Ctrl Pts',(16.4999726614186,25.0000506613489,-0.123384453707664));
#48172=CARTESIAN_POINT('Ctrl Pts',(16.5004305548395,24.9992010730262,-0.00393429210566608));
#48173=CARTESIAN_POINT('Ctrl Pts',(16.499596954495,25.0007483441252,0.115327096639625));
#48174=CARTESIAN_POINT('Ctrl Pts',(16.4993749034989,25.0011604997717,0.14709544984387));
#48175=CARTESIAN_POINT('Ctrl Pts',(16.4990612127222,25.0017427308057,0.178850407212994));
#48176=CARTESIAN_POINT('Ctrl Pts',(16.4986560772927,25.0024948211525,0.210591977021957));
#48177=CARTESIAN_POINT('Ctrl Pts',(16.4970960245892,25.0053908911909,0.332819060104328));
#48178=CARTESIAN_POINT('Ctrl Pts',(16.494180020726,25.0108042715314,0.454847837492651));
#48179=CARTESIAN_POINT('Ctrl Pts',(16.4899193671244,25.0187223059899,0.576679517355416));
#48180=CARTESIAN_POINT('Ctrl Pts',(16.4889197880066,25.0205799322226,0.605262081080578));
#48181=CARTESIAN_POINT('Ctrl Pts',(16.4878461984108,25.0225754170087,0.633833795606361));
#48182=CARTESIAN_POINT('Ctrl Pts',(16.4866987100243,25.0247087838443,0.662394655330664));
#48183=CARTESIAN_POINT('Ctrl Pts',(16.4817000544053,25.0340020945612,0.786810643869416));
#48184=CARTESIAN_POINT('Ctrl Pts',(16.4752990557455,25.0459105789055,0.911020810466703));
#48185=CARTESIAN_POINT('Ctrl Pts',(16.4675050432796,25.0604360570855,1.03502543425808));
#48186=CARTESIAN_POINT('Ctrl Pts',(16.4658835433093,25.0634580002168,1.06082389104392));
#48187=CARTESIAN_POINT('Ctrl Pts',(16.4642017499146,25.0665932131767,1.08661345083528));
#48188=CARTESIAN_POINT('Ctrl Pts',(16.462459724081,25.0698418499384,1.11239410072457));
#48189=CARTESIAN_POINT('Ctrl Pts',(16.4539313788003,25.085746031989,1.23860708767925));
#48190=CARTESIAN_POINT('Ctrl Pts',(16.4439594021546,25.1043674102929,1.36460664508112));
#48191=CARTESIAN_POINT('Ctrl Pts',(16.4325509764523,25.1257240376614,1.49039203107667));
#48192=CARTESIAN_POINT('Ctrl Pts',(16.4304280078101,25.1296982450929,1.5137991546437));
#48193=CARTESIAN_POINT('Ctrl Pts',(16.4282552963827,25.1337671697023,1.53719886137606));
#48194=CARTESIAN_POINT('Ctrl Pts',(16.4260328727072,25.1379310344828,1.560591134797));
#48195=CARTESIAN_POINT('',(16.4999920017365,20.5440045013611,0.0163625070472239));
#48196=CARTESIAN_POINT('Ctrl Pts',(16.4260328550488,25.1379310203705,1.56059112033272));
#48197=CARTESIAN_POINT('Ctrl Pts',(16.4325781611128,25.0612095504425,1.49169837182591));
#48198=CARTESIAN_POINT('Ctrl Pts',(16.4443923286176,24.904358406813,1.35815502612164));
#48199=CARTESIAN_POINT('Ctrl Pts',(16.4587719843597,24.6590142485308,1.17040662826285));
#48200=CARTESIAN_POINT('Ctrl Pts',(16.470251474698,24.4036762388895,0.995167615974384));
#48201=CARTESIAN_POINT('Ctrl Pts',(16.4762395063454,24.2267833177273,0.886709887603812));
#48202=CARTESIAN_POINT('Ctrl Pts',(16.4795386598462,24.1141229826323,0.821569064101446));
#48203=CARTESIAN_POINT('Ctrl Pts',(16.4801762990835,24.091485733423,0.808673248628822));
#48204=CARTESIAN_POINT('Ctrl Pts',(16.4814090233489,24.046000126645,0.783147417153865));
#48205=CARTESIAN_POINT('Ctrl Pts',(16.4820042698769,24.0231445615983,0.770513634247026));
#48206=CARTESIAN_POINT('Ctrl Pts',(16.4837257714998,23.9543880665996,0.7330816742982));
#48207=CARTESIAN_POINT('Ctrl Pts',(16.4869148522506,23.8160056559258,0.660032469923707));
#48208=CARTESIAN_POINT('Ctrl Pts',(16.4894179646491,23.6750358803599,0.592386407658213));
#48209=CARTESIAN_POINT('Ctrl Pts',(16.4915535542388,23.5323553154947,0.528316178904632));
#48210=CARTESIAN_POINT('Ctrl Pts',(16.4922040416757,23.4845098446298,0.507555720552931));
#48211=CARTESIAN_POINT('Ctrl Pts',(16.4933958339036,23.3882488812412,0.467226741424712));
#48212=CARTESIAN_POINT('Ctrl Pts',(16.4939373899151,23.3398009033332,0.447646619206234));
#48213=CARTESIAN_POINT('Ctrl Pts',(16.4954125301957,23.194122538035,0.390893759436398));
#48214=CARTESIAN_POINT('Ctrl Pts',(16.496986028094,22.998707615173,0.320392791852394));
#48215=CARTESIAN_POINT('Ctrl Pts',(16.4984694808079,22.7021396582226,0.2297772781522));
#48216=CARTESIAN_POINT('Ctrl Pts',(16.4993275684369,22.402181338922,0.154058563252679));
#48217=CARTESIAN_POINT('Ctrl Pts',(16.4997658338623,22.098859610186,0.0931210861774427));
#48218=CARTESIAN_POINT('Ctrl Pts',(16.4999479248813,21.792174258382,0.0469681249854355));
#48219=CARTESIAN_POINT('Ctrl Pts',(16.4999811846693,21.5854566915983,0.0261372463727013));
#48220=CARTESIAN_POINT('Ctrl Pts',(16.4999920914489,21.455540117511,0.0162749117889595));
#48221=CARTESIAN_POINT('Ctrl Pts',(16.4999937468063,21.4295168568963,0.0144601446280865));
#48222=CARTESIAN_POINT('Ctrl Pts',(16.4999963161695,21.3774149533551,0.0111492969632006));
#48223=CARTESIAN_POINT('Ctrl Pts',(16.4999990408472,21.2992639192183,0.00666633889523769));
#48224=CARTESIAN_POINT('Ctrl Pts',(16.5000002603666,21.1169242222562,-0.000419245858196618));
#48225=CARTESIAN_POINT('Ctrl Pts',(16.5000000702348,20.8564753422434,-0.000939509443136404));
#48226=CARTESIAN_POINT('Ctrl Pts',(16.4999993099702,20.6481548381454,0.0088764751499754));
#48227=CARTESIAN_POINT('Ctrl Pts',(16.4999918882417,20.5440044054399,0.0163611721806806));
#48228=CARTESIAN_POINT('',(8.52036860632481,20.5440036583397,-14.1298732767534));
#48229=CARTESIAN_POINT('Origin',(6.61363325216158E-15,20.5440037453176,
8.67361737988404E-16));
#48230=CARTESIAN_POINT('',(6.24602095305321E-15,27.1622780870028,-16.5000001006436));
#48231=CARTESIAN_POINT('Ctrl Pts',(8.52036867104336,20.5440037453176,-14.1298732375596));
#48232=CARTESIAN_POINT('Ctrl Pts',(8.58356973556036,20.6246183822895,-14.0917627491615));
#48233=CARTESIAN_POINT('Ctrl Pts',(8.64460810914305,20.7071305594912,-14.0543784285267));
#48234=CARTESIAN_POINT('Ctrl Pts',(8.71820078920157,20.812702180057,-14.0086857037865));
#48235=CARTESIAN_POINT('Ctrl Pts',(8.73278393179618,20.8339381962245,-13.9995991057947));
#48236=CARTESIAN_POINT('Ctrl Pts',(8.76167886001795,20.8766555969633,-13.9815333163542));
#48237=CARTESIAN_POINT('Ctrl Pts',(8.77598021132686,20.8981217579526,-13.9725606313828));
#48238=CARTESIAN_POINT('Ctrl Pts',(8.8184076223346,20.9627832131134,-13.9458525761399));
#48239=CARTESIAN_POINT('Ctrl Pts',(8.90140518031076,21.0932318928779,-13.8932455450086));
#48240=CARTESIAN_POINT('Ctrl Pts',(9.03052355651088,21.3162917133111,-13.8097792924337));
#48241=CARTESIAN_POINT('Ctrl Pts',(9.17080434164138,21.5931460660356,-13.7169551928144));
#48242=CARTESIAN_POINT('Ctrl Pts',(9.29632299716888,21.8794396203386,-13.6321374667544));
#48243=CARTESIAN_POINT('Ctrl Pts',(9.36997146821566,22.0768411939832,-13.5814347795442));
#48244=CARTESIAN_POINT('Ctrl Pts',(9.42132449791413,22.2274690286921,-13.5458140656644));
#48245=CARTESIAN_POINT('Ctrl Pts',(9.44191187979202,22.2907678651923,-13.5314737738112));
#48246=CARTESIAN_POINT('Ctrl Pts',(9.46146566890013,22.3547580121912,-13.5177915988317));
#48247=CARTESIAN_POINT('Ctrl Pts',(9.46920397396335,22.3804098312845,-13.5123720498178));
#48248=CARTESIAN_POINT('Ctrl Pts',(9.47303319764194,22.3932693111686,-13.5096877608054));
#48249=CARTESIAN_POINT('Ctrl Pts',(9.48438274145507,22.4318890364132,-13.5017246841252));
#48250=CARTESIAN_POINT('Ctrl Pts',(9.52126642056339,22.5608025012239,-13.4757985800892));
#48251=CARTESIAN_POINT('Ctrl Pts',(9.57917707246071,22.7944720582964,-13.4347193862869));
#48252=CARTESIAN_POINT('Ctrl Pts',(9.63851629653991,23.1094990108463,-13.3921717551923));
#48253=CARTESIAN_POINT('Ctrl Pts',(9.68000107488758,23.4280224786546,-13.3621887684031));
#48254=CARTESIAN_POINT('Ctrl Pts',(9.70346143786766,23.750099543279,-13.3451456898397));
#48255=CARTESIAN_POINT('Ctrl Pts',(9.7068399497473,23.9672442799538,-13.342685693239));
#48256=CARTESIAN_POINT('Ctrl Pts',(9.70499841460441,24.1037427373277,-13.3440251041407));
#48257=CARTESIAN_POINT('Ctrl Pts',(9.70443222180082,24.1310828669418,-13.3444368989173));
#48258=CARTESIAN_POINT('Ctrl Pts',(9.70290046268754,24.1858371549446,-13.3455507008099));
#48259=CARTESIAN_POINT('Ctrl Pts',(9.7000109928316,24.2678204701582,-13.3476514275137));
#48260=CARTESIAN_POINT('Ctrl Pts',(9.68916397490106,24.4580880152858,-13.3555317041429));
#48261=CARTESIAN_POINT('Ctrl Pts',(9.66213830977216,24.7270183053258,-13.3751235730946));
#48262=CARTESIAN_POINT('Ctrl Pts',(9.61169454034366,25.0452581559799,-13.4114533409026));
#48263=CARTESIAN_POINT('Ctrl Pts',(9.56620835788032,25.2544954002469,-13.4439075432828));
#48264=CARTESIAN_POINT('Ctrl Pts',(9.52765523426529,25.4103411250022,-13.4712298559432));
#48265=CARTESIAN_POINT('Ctrl Pts',(9.51406393953746,25.462109235537,-13.4808343470393));
#48266=CARTESIAN_POINT('Ctrl Pts',(9.4853960356642,25.5652856616541,-13.5010210497032));
#48267=CARTESIAN_POINT('Ctrl Pts',(9.47031765250651,25.6166997302657,-13.5116045036733));
#48268=CARTESIAN_POINT('Ctrl Pts',(9.42285181695582,25.7703679435337,-13.5447906756782));
#48269=CARTESIAN_POINT('Ctrl Pts',(9.35423263799206,25.9717569689352,-13.5924367699028));
#48270=CARTESIAN_POINT('Ctrl Pts',(9.23589274235606,26.2638847079763,-13.6731842177505));
#48271=CARTESIAN_POINT('Ctrl Pts',(9.10250881132217,26.5464727923424,-13.7624061878736));
#48272=CARTESIAN_POINT('Ctrl Pts',(9.00367297582431,26.7287040698433,-13.8270636691253));
#48273=CARTESIAN_POINT('Ctrl Pts',(8.92582693941875,26.86311490726,-13.8773400779457));
#48274=CARTESIAN_POINT('Ctrl Pts',(8.89925793564753,26.9075411417532,-13.8943962929227));
#48275=CARTESIAN_POINT('Ctrl Pts',(8.85846953453316,26.9736179421189,-13.9204086701232));
#48276=CARTESIAN_POINT('Ctrl Pts',(8.84471258649409,26.9955575542314,-13.9291539631109));
#48277=CARTESIAN_POINT('Ctrl Pts',(8.81690762026432,27.0392155833153,-13.9467706255413));
#48278=CARTESIAN_POINT('Ctrl Pts',(8.74675476164461,27.1476705617355,-13.9910722905394));
#48279=CARTESIAN_POINT('Ctrl Pts',(8.61476617389104,27.3367718819407,-14.0730584659179));
#48280=CARTESIAN_POINT('Ctrl Pts',(8.42682897940193,27.5764190798257,-14.1864547250946));
#48281=CARTESIAN_POINT('Ctrl Pts',(8.22702390985309,27.8039646543995,-14.3033160861774));
#48282=CARTESIAN_POINT('Ctrl Pts',(8.01529570680411,28.0196373988293,-14.4230965455344));
#48283=CARTESIAN_POINT('Ctrl Pts',(7.86606700155189,28.1555579746117,-14.5045702358948));
#48284=CARTESIAN_POINT('Ctrl Pts',(7.77020561634108,28.2380379248674,-14.5559052506994));
#48285=CARTESIAN_POINT('Ctrl Pts',(7.75089034450941,28.2544211982413,-14.5661999638286));
#48286=CARTESIAN_POINT('Ctrl Pts',(7.71207921912852,28.2868721608515,-14.5867856855695));
#48287=CARTESIAN_POINT('Ctrl Pts',(7.65358922171243,28.3350784667842,-14.6176602712913));
#48288=CARTESIAN_POINT('Ctrl Pts',(7.51520251850315,28.4442939198586,-14.6896485772748));
#48289=CARTESIAN_POINT('Ctrl Pts',(7.31206110143769,28.5911128669389,-14.7922039875687));
#48290=CARTESIAN_POINT('Ctrl Pts',(7.0595338938036,28.7528122439669,-14.9144197286055));
#48291=CARTESIAN_POINT('Ctrl Pts',(6.79811902487365,28.9000931027409,-15.0354236930373));
#48292=CARTESIAN_POINT('Ctrl Pts',(6.52759964013339,29.0328506210847,-15.1548791157694));
#48293=CARTESIAN_POINT('Ctrl Pts',(6.34097767462334,29.1114881121681,-15.2332703436679));
#48294=CARTESIAN_POINT('Ctrl Pts',(6.22229167082311,29.157455801492,-15.2818108895932));
#48295=CARTESIAN_POINT('Ctrl Pts',(6.19845201502356,29.1664901400402,-15.2914963053156));
#48296=CARTESIAN_POINT('Ctrl Pts',(6.1505652609305,29.1842373202765,-15.3108201481523));
#48297=CARTESIAN_POINT('Ctrl Pts',(6.12650550559815,29.192954592622,-15.3204635969749));
#48298=CARTESIAN_POINT('Ctrl Pts',(6.05411458449316,29.21858273349,-15.3492799421749));
#48299=CARTESIAN_POINT('Ctrl Pts',(5.90854023930549,29.2677275125996,-15.406436019442));
#48300=CARTESIAN_POINT('Ctrl Pts',(5.76056712447322,29.3105198925897,-15.4621195869495));
#48301=CARTESIAN_POINT('Ctrl Pts',(5.61095373220127,29.3490081544351,-15.5167656792345));
#48302=CARTESIAN_POINT('Ctrl Pts',(5.56080907911311,29.3611197173853,-15.5348081407752));
#48303=CARTESIAN_POINT('Ctrl Pts',(5.48517531992791,29.3781968950826,-15.5616055439635));
#48304=CARTESIAN_POINT('Ctrl Pts',(5.45992174054239,29.383701314867,-15.5704839711456));
#48305=CARTESIAN_POINT('Ctrl Pts',(5.40937365701591,29.3943253639894,-15.5881170494493));
#48306=CARTESIAN_POINT('Ctrl Pts',(5.28286658753632,29.4199307135622,-15.6319025319486));
#48307=CARTESIAN_POINT('Ctrl Pts',(5.05392249571448,29.4574578294063,-15.7080373618841));
#48308=CARTESIAN_POINT('Ctrl Pts',(4.74602717236481,29.4892626374968,-15.8037960831374));
#48309=CARTESIAN_POINT('Ctrl Pts',(4.43547463092405,29.5026830764944,-15.8937570526983));
#48310=CARTESIAN_POINT('Ctrl Pts',(4.12223271289369,29.4973754911404,-15.9778716462655));
#48311=CARTESIAN_POINT('Ctrl Pts',(3.91158214250878,29.4809872600072,-16.0300139016686));
#48312=CARTESIAN_POINT('Ctrl Pts',(3.77934373830044,29.466567150816,-16.0613604558222));
#48313=CARTESIAN_POINT('Ctrl Pts',(3.75284652996683,29.4634712408978,-16.0675722891403));
#48314=CARTESIAN_POINT('Ctrl Pts',(3.69997737442021,29.4568803671405,-16.0798290965113));
#48315=CARTESIAN_POINT('Ctrl Pts',(3.62081101329016,29.4463908628385,-16.0979763101384));
#48316=CARTESIAN_POINT('Ctrl Pts',(3.43704882469573,29.4177128600773,-16.1386741697335));
#48317=CARTESIAN_POINT('Ctrl Pts',(3.17726317966928,29.3648358288221,-16.19222548041));
#48318=CARTESIAN_POINT('Ctrl Pts',(2.86990903950336,29.2824713373728,-16.2494807144156));
#48319=CARTESIAN_POINT('Ctrl Pts',(2.56701318537708,29.1811477696582,-16.3000402857368));
#48320=CARTESIAN_POINT('Ctrl Pts',(2.36813622523175,29.1008034970775,-16.3294779261791));
#48321=CARTESIAN_POINT('Ctrl Pts',(2.22016840429561,29.0356389912742,-16.350025439958));
#48322=CARTESIAN_POINT('Ctrl Pts',(2.14648219853387,29.0018293678555,-16.3599164766422));
#48323=CARTESIAN_POINT('Ctrl Pts',(2.07325316811817,28.9661508133544,-16.3692462842728));
#48324=CARTESIAN_POINT('Ctrl Pts',(2.02453675387829,28.941946133812,-16.375342852792));
#48325=CARTESIAN_POINT('Ctrl Pts',(2.00027966959624,28.9296588123334,-16.3783232300789));
#48326=CARTESIAN_POINT('Ctrl Pts',(1.87964446253043,28.8673778523924,-16.3928760766113));
#48327=CARTESIAN_POINT('Ctrl Pts',(1.6904817909171,28.7621787042267,-16.413966852621));
#48328=CARTESIAN_POINT('Ctrl Pts',(1.41806400209131,28.5881274996996,-16.439677345571));
#48329=CARTESIAN_POINT('Ctrl Pts',(1.15686246306753,28.3980418347844,-16.4600591391421));
#48330=CARTESIAN_POINT('Ctrl Pts',(0.906884940340453,28.1919726464131,-16.4756642554084));
#48331=CARTESIAN_POINT('Ctrl Pts',(0.747798975294972,28.0438617742335,-16.4832287491238));
#48332=CARTESIAN_POINT('Ctrl Pts',(0.660487452314263,27.9574775763779,-16.4867780538133));
#48333=CARTESIAN_POINT('Ctrl Pts',(0.65081639862174,27.9478366294134,-16.4871626151795));
#48334=CARTESIAN_POINT('Ctrl Pts',(0.631534954029398,27.9284690767797,-16.487912441723));
#48335=CARTESIAN_POINT('Ctrl Pts',(0.602691356915125,27.899276349876,-16.4890086703192));
#48336=CARTESIAN_POINT('Ctrl Pts',(0.536287826182138,27.8305242123613,-16.4913578844274));
#48337=CARTESIAN_POINT('Ctrl Pts',(0.407044276552453,27.6904990051635,-16.4952601873013));
#48338=CARTESIAN_POINT('Ctrl Pts',(0.232437371388159,27.4833706236392,-16.498773144052));
#48339=CARTESIAN_POINT('Ctrl Pts',(0.0887795656506141,27.2908969996746,
-16.499907810755));
#48340=CARTESIAN_POINT('Ctrl Pts',(0.0136105057645173,27.1822328811265,
-16.500000075685));
#48341=CARTESIAN_POINT('Ctrl Pts',(6.24602095305321E-15,27.1622780870028,
-16.5000001006436));
#48342=CARTESIAN_POINT('',(-0.948483647701403,24.5,-16.4727162159814));
#48343=CARTESIAN_POINT('Ctrl Pts',(6.24602095305321E-15,27.1622780870028,
-16.5000001006436));
#48344=CARTESIAN_POINT('Ctrl Pts',(-0.0472377228897633,27.0930213634507,
-16.500000187267));
#48345=CARTESIAN_POINT('Ctrl Pts',(-0.151744971279771,26.932023013624,-16.4995362318231));
#48346=CARTESIAN_POINT('Ctrl Pts',(-0.24805737644771,26.7652319559107,-16.4982159706337));
#48347=CARTESIAN_POINT('Ctrl Pts',(-0.325446292899342,26.6216010796214,
-16.4968103092495));
#48348=CARTESIAN_POINT('Ctrl Pts',(-0.356870012161321,26.5611741884442,
-16.4961639215616));
#48349=CARTESIAN_POINT('Ctrl Pts',(-0.387256442555717,26.5000142859108,
-16.4954560075668));
#48350=CARTESIAN_POINT('Ctrl Pts',(-0.399327758053236,26.475491492047,-16.4951681953086));
#48351=CARTESIAN_POINT('Ctrl Pts',(-0.40532387922394,26.4631963125769,-16.495021913523));
#48352=CARTESIAN_POINT('Ctrl Pts',(-0.42316131880117,26.4262757584871,-16.4945771693899));
#48353=CARTESIAN_POINT('Ctrl Pts',(-0.481641589570278,26.3029164586969,
-16.4930545121647));
#48354=CARTESIAN_POINT('Ctrl Pts',(-0.578188697338098,26.0782767729238,
-16.4900107723047));
#48355=CARTESIAN_POINT('Ctrl Pts',(-0.688771519624153,25.7733547477354,
-16.4857218407985));
#48356=CARTESIAN_POINT('Ctrl Pts',(-0.781453084810564,25.463099138679,-16.4815550888826));
#48357=CARTESIAN_POINT('Ctrl Pts',(-0.856288053441708,25.1475226392437,
-16.4778094315988));
#48358=CARTESIAN_POINT('Ctrl Pts',(-0.894191822217506,24.9335626849954,
-16.4757602126714));
#48359=CARTESIAN_POINT('Ctrl Pts',(-0.914067562624034,24.7986994366961,
-16.4746622527135));
#48360=CARTESIAN_POINT('Ctrl Pts',(-0.917851839507087,24.7716698243462,
-16.4744517646284));
#48361=CARTESIAN_POINT('Ctrl Pts',(-0.925036263082085,24.7174959519111,
-16.474049922722));
#48362=CARTESIAN_POINT('Ctrl Pts',(-0.928436494465732,24.6903491769012,
-16.4738585631455));
#48363=CARTESIAN_POINT('Ctrl Pts',(-0.938041179156906,24.6088805414888,
-16.4733153881458));
#48364=CARTESIAN_POINT('Ctrl Pts',(-0.94365634381575,24.5544828879381,-16.4729941445046));
#48365=CARTESIAN_POINT('Ctrl Pts',(-0.948483646373672,24.5,-16.4727161929222));
#48366=CARTESIAN_POINT('',(-12.6567683575148,24.5,-10.5856608081032));
#48367=CARTESIAN_POINT('Origin',(6.61363325216158E-15,24.5,8.67361737988404E-16));
#48368=CARTESIAN_POINT('',(-12.6567683575148,23.5,-10.5856608081032));
#48369=CARTESIAN_POINT('',(-12.6567683575148,52.,-10.5856608081032));
#48370=CARTESIAN_POINT('',(-0.948483680554045,23.5000000000023,-16.4727167864039));
#48371=CARTESIAN_POINT('Origin',(6.61363325216158E-15,23.5,8.67361737988404E-16));
#48372=CARTESIAN_POINT('',(-1.70949320542661E-11,20.8377220411253,-16.5000002469429));
#48373=CARTESIAN_POINT('Ctrl Pts',(-0.948483646373667,23.5,-16.4727161929222));
#48374=CARTESIAN_POINT('Ctrl Pts',(-0.936570751042234,23.3655462479154,
-16.473402126333));
#48375=CARTESIAN_POINT('Ctrl Pts',(-0.919881054270985,23.2317908343366,
-16.4743522007642));
#48376=CARTESIAN_POINT('Ctrl Pts',(-0.887701935566159,23.0322016836209,
-16.4761069634426));
#48377=CARTESIAN_POINT('Ctrl Pts',(-0.875783591794726,22.9658461353017,
-16.4767465113257));
#48378=CARTESIAN_POINT('Ctrl Pts',(-0.859388727144383,22.8831203518824,
-16.4776048561917));
#48379=CARTESIAN_POINT('Ctrl Pts',(-0.856033751776329,22.8665807883718,
-16.4777795223152));
#48380=CARTESIAN_POINT('Ctrl Pts',(-0.849181370413379,22.8335596647343,
-16.478134080361));
#48381=CARTESIAN_POINT('Ctrl Pts',(-0.838688352910079,22.7841101256929,
-16.4786737977762));
#48382=CARTESIAN_POINT('Ctrl Pts',(-0.797863035066176,22.6036956423096,
-16.4807342001022));
#48383=CARTESIAN_POINT('Ctrl Pts',(-0.718348342681733,22.3133396372222,
-16.4844985774509));
#48384=CARTESIAN_POINT('Ctrl Pts',(-0.585692611919195,21.9363933078712,
-16.4898158669865));
#48385=CARTESIAN_POINT('Ctrl Pts',(-0.426443232786663,21.5696178472444,
-16.4947882638331));
#48386=CARTESIAN_POINT('Ctrl Pts',(-0.302290706141837,21.3319736271105,
-16.4973656109522));
#48387=CARTESIAN_POINT('Ctrl Pts',(-0.227236552358115,21.2002907335068,
-16.498437292914));
#48388=CARTESIAN_POINT('Ctrl Pts',(-0.218824617931184,21.1856870077043,
-16.4985510815842));
#48389=CARTESIAN_POINT('Ctrl Pts',(-0.201854838211685,21.1565352459083,
-16.4987674275792));
#48390=CARTESIAN_POINT('Ctrl Pts',(-0.193295857165294,21.1419854169811,
-16.4988699923641));
#48391=CARTESIAN_POINT('Ctrl Pts',(-0.167435923262676,21.0984815372009,
-16.4991594472239));
#48392=CARTESIAN_POINT('Ctrl Pts',(-0.114949217821082,21.0119958671242,
-16.4996658454698));
#48393=CARTESIAN_POINT('Ctrl Pts',(-0.0601661390105475,20.9270736538768,
-16.499933015325));
#48394=CARTESIAN_POINT('Ctrl Pts',(-0.0151228573542697,20.8599822262627,
-16.4999947743784));
#48395=CARTESIAN_POINT('Ctrl Pts',(-0.00758180657007838,20.8488382595036,
-16.5000000179473));
#48396=CARTESIAN_POINT('Ctrl Pts',(6.67038445962762E-15,20.8377220411027,
-16.5000000441008));
#48397=CARTESIAN_POINT('',(0.214930999317485,20.5439968211114,-16.4986004257358));
#48398=CARTESIAN_POINT('Origin',(4.47125871799245,23.8871484228103,-15.8444072749798));
#48399=CARTESIAN_POINT('',(-16.499654466181,20.5440037453176,0.106782473437621));
#48400=CARTESIAN_POINT('Origin',(6.61363325216158E-15,20.5440037453176,
8.67361737988404E-16));
#48401=CARTESIAN_POINT('',(-16.4714285499925,22.,0.970588235294111));
#48402=CARTESIAN_POINT('Ctrl Pts',(-16.499654466181,20.5440037453176,0.106782473437621));
#48403=CARTESIAN_POINT('Ctrl Pts',(-16.4996850755552,20.5535144807161,0.102052819949738));
#48404=CARTESIAN_POINT('Ctrl Pts',(-16.4997126952277,20.5631072668192,0.0974703596247774));
#48405=CARTESIAN_POINT('Ctrl Pts',(-16.4997376258724,20.5727456617118,0.0930496248789231));
#48406=CARTESIAN_POINT('Ctrl Pts',(-16.4997625565171,20.5823840566043,0.0886288901330683));
#48407=CARTESIAN_POINT('Ctrl Pts',(-16.4997848039146,20.5920679507547,0.084369593340066));
#48408=CARTESIAN_POINT('Ctrl Pts',(-16.4998047468791,20.6017971921991,0.0802702612752421));
#48409=CARTESIAN_POINT('Ctrl Pts',(-16.4998049929255,20.6019172267505,0.0802196857511204));
#48410=CARTESIAN_POINT('Ctrl Pts',(-16.4998052386174,20.6020372667433,0.080169135257586));
#48411=CARTESIAN_POINT('Ctrl Pts',(-16.4998054839553,20.6021573121326,0.0801186098125461));
#48412=CARTESIAN_POINT('Ctrl Pts',(-16.4998450097016,20.6214975065332,0.0719785893151182));
#48413=CARTESIAN_POINT('Ctrl Pts',(-16.4998754990255,20.641016717206,0.0644676880107839));
#48414=CARTESIAN_POINT('Ctrl Pts',(-16.4998995537066,20.6607098412591,0.0575735908839684));
#48415=CARTESIAN_POINT('Ctrl Pts',(-16.4998998914639,20.660986356993,0.0574767892631659));
#48416=CARTESIAN_POINT('Ctrl Pts',(-16.4999002279526,20.6612629071222,0.0573801092205637));
#48417=CARTESIAN_POINT('Ctrl Pts',(-16.4999005631797,20.6615394916358,0.0572835507204533));
#48418=CARTESIAN_POINT('Ctrl Pts',(-16.4999482732881,20.7009034849249,0.0435411755571679));
#48419=CARTESIAN_POINT('Ctrl Pts',(-16.4999708656352,20.7409617256664,0.0322534156903742));
#48420=CARTESIAN_POINT('Ctrl Pts',(-16.4999833980792,20.781710378534,0.0234067813658331));
#48421=CARTESIAN_POINT('Ctrl Pts',(-16.4999836034944,20.7823782764952,0.0232617790501028));
#48422=CARTESIAN_POINT('Ctrl Pts',(-16.4999838062025,20.7830463600297,0.0231174328684831));
#48423=CARTESIAN_POINT('Ctrl Pts',(-16.4999840062693,20.7837146291111,0.02297374275987));
#48424=CARTESIAN_POINT('Ctrl Pts',(-16.4999899521532,20.803575243884,0.0187033463386016));
#48425=CARTESIAN_POINT('Ctrl Pts',(-16.499993462673,20.8236002580073,0.0150141556328887));
#48426=CARTESIAN_POINT('Ctrl Pts',(-16.4999956982758,20.8437920839178,0.0119148065284029));
#48427=CARTESIAN_POINT('Ctrl Pts',(-16.499995798485,20.84469716762,0.0117758804909841));
#48428=CARTESIAN_POINT('Ctrl Pts',(-16.4999958961317,20.8456025864146,0.0116381392857442));
#48429=CARTESIAN_POINT('Ctrl Pts',(-16.4999959913199,20.8465083405368,0.0115015837651071));
#48430=CARTESIAN_POINT('Ctrl Pts',(-16.499996993652,20.856045936145,0.0100636534239759));
#48431=CARTESIAN_POINT('Ctrl Pts',(-16.4999977180954,20.8656207442355,0.00875729385934541));
#48432=CARTESIAN_POINT('Ctrl Pts',(-16.4999982570698,20.8752332106515,0.00758408663351017));
#48433=CARTESIAN_POINT('Ctrl Pts',(-16.4999983150879,20.8762679485595,0.00745779625827971));
#48434=CARTESIAN_POINT('Ctrl Pts',(-16.4999983709589,20.8773031577963,0.00733304411345781));
#48435=CARTESIAN_POINT('Ctrl Pts',(-16.4999984247971,20.8783388333972,0.00720983309849447));
#48436=CARTESIAN_POINT('Ctrl Pts',(-16.4999989186003,20.8878380267597,0.00607974443509351));
#48437=CARTESIAN_POINT('Ctrl Pts',(-16.4999992405276,20.8973642148206,0.00508130425039852));
#48438=CARTESIAN_POINT('Ctrl Pts',(-16.4999994608597,20.9068704272133,0.00421826344624561));
#48439=CARTESIAN_POINT('Ctrl Pts',(-16.4999994877968,20.9080326271967,0.00411275075971433));
#48440=CARTESIAN_POINT('Ctrl Pts',(-16.4999995132179,20.9091946134966,0.00400925275482219));
#48441=CARTESIAN_POINT('Ctrl Pts',(-16.4999995372511,20.9103563075049,0.00390777595391313));
#48442=CARTESIAN_POINT('Ctrl Pts',(-16.5000003852682,20.9513468671561,0.00032715073647429));
#48443=CARTESIAN_POINT('Ctrl Pts',(-16.5000000779434,20.9922292246122,-0.000777075137903916));
#48444=CARTESIAN_POINT('Ctrl Pts',(-16.4999999941945,21.0329747879212,0.000528103560881647));
#48445=CARTESIAN_POINT('Ctrl Pts',(-16.499999990816,21.0346184768029,0.000580754881455815));
#48446=CARTESIAN_POINT('Ctrl Pts',(-16.4999999878023,21.0362619608369,0.00063732859592822));
#48447=CARTESIAN_POINT('Ctrl Pts',(-16.499999985244,21.0379052402467,0.000697819978592266));
#48448=CARTESIAN_POINT('Ctrl Pts',(-16.4999999225867,21.0781518367236,0.00217935273184643));
#48449=CARTESIAN_POINT('Ctrl Pts',(-16.5000001351939,21.1182755725363,0.0060110870606543));
#48450=CARTESIAN_POINT('Ctrl Pts',(-16.4999954686141,21.1582742498412,0.0122343404349139));
#48451=CARTESIAN_POINT('Ctrl Pts',(-16.4999952233127,21.1603768029377,0.0125614692685093));
#48452=CARTESIAN_POINT('Ctrl Pts',(-16.4999949645496,21.1624787881589,0.0128951791688783));
#48453=CARTESIAN_POINT('Ctrl Pts',(-16.4999946915747,21.1645802697767,0.0132354829271487));
#48454=CARTESIAN_POINT('Ctrl Pts',(-16.499993325008,21.1751007045472,0.0149391111962692));
#48455=CARTESIAN_POINT('Ctrl Pts',(-16.4999915645246,21.1856084870641,0.0168085463933244));
#48456=CARTESIAN_POINT('Ctrl Pts',(-16.4999892357063,21.1961115765617,0.0188473228317351));
#48457=CARTESIAN_POINT('Ctrl Pts',(-16.4999874242188,21.2042814771213,0.0204331991368735));
#48458=CARTESIAN_POINT('Ctrl Pts',(-16.4999852651097,21.2124588137965,0.0221239408880127));
#48459=CARTESIAN_POINT('Ctrl Pts',(-16.4999826683071,21.2206193345647,0.0239154460820305));
#48460=CARTESIAN_POINT('Ctrl Pts',(-16.4999819294058,21.2229413514076,0.0244252058575302));
#48461=CARTESIAN_POINT('Ctrl Pts',(-16.4999811553101,21.2252612088109,0.0249429486522115));
#48462=CARTESIAN_POINT('Ctrl Pts',(-16.499980343994,21.2275783324658,0.025468565185762));
#48463=CARTESIAN_POINT('Ctrl Pts',(-16.4999739062223,21.2459646482072,0.029639318664803));
#48464=CARTESIAN_POINT('Ctrl Pts',(-16.499965168879,21.2641329203393,0.0342923029695724));
#48465=CARTESIAN_POINT('Ctrl Pts',(-16.4999528955845,21.2821222293978,0.0394268528483906));
#48466=CARTESIAN_POINT('Ctrl Pts',(-16.4999512094238,21.2845936821723,0.0401322605715414));
#48467=CARTESIAN_POINT('Ctrl Pts',(-16.4999494565824,21.2870615167562,0.0408467089387852));
#48468=CARTESIAN_POINT('Ctrl Pts',(-16.499947633876,21.2895257430366,0.0415701738064822));
#48469=CARTESIAN_POINT('Ctrl Pts',(-16.4999195782284,21.3274558582823,0.0527059635781082));
#48470=CARTESIAN_POINT('Ctrl Pts',(-16.4998753415841,21.3645335982835,0.0659717015008427));
#48471=CARTESIAN_POINT('Ctrl Pts',(-16.4997994440263,21.4007641483025,0.0813542360780683));
#48472=CARTESIAN_POINT('Ctrl Pts',(-16.4997938623563,21.4034286210488,0.0824855008291571));
#48473=CARTESIAN_POINT('Ctrl Pts',(-16.4997881092592,21.4060885042182,0.0836282355142637));
#48474=CARTESIAN_POINT('Ctrl Pts',(-16.499782178525,21.40874380041,0.0847824347605743));
#48475=CARTESIAN_POINT('Ctrl Pts',(-16.4997022260076,21.4445399778131,0.100342251065656));
#48476=CARTESIAN_POINT('Ctrl Pts',(-16.4995901346931,21.4795026091028,0.117985016276668));
#48477=CARTESIAN_POINT('Ctrl Pts',(-16.4994246315052,21.5135982764372,0.137793818801735));
#48478=CARTESIAN_POINT('Ctrl Pts',(-16.4994113971708,21.516324710114,0.139377814380164));
#48479=CARTESIAN_POINT('Ctrl Pts',(-16.4993978180569,21.5190461487608,0.140976029923642));
#48480=CARTESIAN_POINT('Ctrl Pts',(-16.4993838850203,21.5217621567528,0.142588269970934));
#48481=CARTESIAN_POINT('Ctrl Pts',(-16.4993510266202,21.5281673417792,0.146390429552292));
#48482=CARTESIAN_POINT('Ctrl Pts',(-16.4993161672843,21.5345419408095,0.150271257276818));
#48483=CARTESIAN_POINT('Ctrl Pts',(-16.4992793247798,21.5408581501453,0.154213193100599));
#48484=CARTESIAN_POINT('Ctrl Pts',(-16.4992635095367,21.5435694855291,0.155905333039508));
#48485=CARTESIAN_POINT('Ctrl Pts',(-16.4992473206821,21.5462714940611,0.157609622888016));
#48486=CARTESIAN_POINT('Ctrl Pts',(-16.4992307576353,21.5489622035107,0.159324845208098));
#48487=CARTESIAN_POINT('Ctrl Pts',(-16.4991923750128,21.5551975590362,0.16329964113873));
#48488=CARTESIAN_POINT('Ctrl Pts',(-16.4991519431483,21.5613804148635,0.167337906081907));
#48489=CARTESIAN_POINT('Ctrl Pts',(-16.499109342362,21.5675089764998,0.171437780545278));
#48490=CARTESIAN_POINT('Ctrl Pts',(-16.4990907943137,21.5701773041687,0.173222833730487));
#48491=CARTESIAN_POINT('Ctrl Pts',(-16.4990718342908,21.5728354457023,0.175019650671196));
#48492=CARTESIAN_POINT('Ctrl Pts',(-16.4990524512606,21.575483432979,0.176828195013071));
#48493=CARTESIAN_POINT('Ctrl Pts',(-16.4989443754721,21.5902480652543,0.186912266185078));
#48494=CARTESIAN_POINT('Ctrl Pts',(-16.4988231621382,21.6046972465362,0.197360668681009));
#48495=CARTESIAN_POINT('Ctrl Pts',(-16.4986867741193,21.6188338672979,0.208170018128185));
#48496=CARTESIAN_POINT('Ctrl Pts',(-16.4986621113215,21.6213901667587,0.210124653159401));
#48497=CARTESIAN_POINT('Ctrl Pts',(-16.4986369521581,21.6239362359053,0.212091100647114));
#48498=CARTESIAN_POINT('Ctrl Pts',(-16.4986112845102,21.6264720928427,0.214069340712306));
#48499=CARTESIAN_POINT('Ctrl Pts',(-16.4983021475512,21.6570135395292,0.237894940884204));
#48500=CARTESIAN_POINT('Ctrl Pts',(-16.4979196123918,21.6860781938654,0.263425997552144));
#48501=CARTESIAN_POINT('Ctrl Pts',(-16.4974392639963,21.7136459342938,0.290685235672527));
#48502=CARTESIAN_POINT('Ctrl Pts',(-16.497400197548,21.7158880021684,0.292902213238513));
#48503=CARTESIAN_POINT('Ctrl Pts',(-16.4973604834622,21.7181201515103,0.295130644757958));
#48504=CARTESIAN_POINT('Ctrl Pts',(-16.4973201084484,21.7203423726231,0.297370542231756));
#48505=CARTESIAN_POINT('Ctrl Pts',(-16.4970916547833,21.7329163511894,0.310044538830837));
#48506=CARTESIAN_POINT('Ctrl Pts',(-16.4968419806759,21.7451714933841,0.323086675437377));
#48507=CARTESIAN_POINT('Ctrl Pts',(-16.4965682638719,21.7571008003871,0.336504926313332));
#48508=CARTESIAN_POINT('Ctrl Pts',(-16.4965213022176,21.7591475143029,0.338807098668096));
#48509=CARTESIAN_POINT('Ctrl Pts',(-16.4964736410885,21.76118427836,0.341119936936436));
#48510=CARTESIAN_POINT('Ctrl Pts',(-16.4964252607106,21.7632113073105,0.343443762192151));
#48511=CARTESIAN_POINT('Ctrl Pts',(-16.4963077302334,21.7681355697923,0.349089032092526));
#48512=CARTESIAN_POINT('Ctrl Pts',(-16.4961858538074,21.7730059618872,0.354803597494513));
#48513=CARTESIAN_POINT('Ctrl Pts',(-16.4960595381071,21.7778168568144,0.360582400563539));
#48514=CARTESIAN_POINT('Ctrl Pts',(-16.496008584632,21.7797574850508,0.362913465485598));
#48515=CARTESIAN_POINT('Ctrl Pts',(-16.4959569121632,21.7816883298161,0.365254813842329));
#48516=CARTESIAN_POINT('Ctrl Pts',(-16.4959045350397,21.7836082214615,0.367605183393828));
#48517=CARTESIAN_POINT('Ctrl Pts',(-16.4958652649051,21.785047674378,0.369367390294314));
#48518=CARTESIAN_POINT('Ctrl Pts',(-16.4958256260704,21.786480009922,0.371133463281377));
#48519=CARTESIAN_POINT('Ctrl Pts',(-16.4957856214331,21.7879050133131,0.372903113111902));
#48520=CARTESIAN_POINT('Ctrl Pts',(-16.4956922600184,21.791230636081,0.377033059612092));
#48521=CARTESIAN_POINT('Ctrl Pts',(-16.495596855473,21.7945180371583,0.38118474027107));
#48522=CARTESIAN_POINT('Ctrl Pts',(-16.495499365647,21.7977677372998,0.385357857057256));
#48523=CARTESIAN_POINT('Ctrl Pts',(-16.4954449712311,21.7995809064064,0.387686246171819));
#48524=CARTESIAN_POINT('Ctrl Pts',(-16.4953899269477,21.8013822834842,0.390021339107209));
#48525=CARTESIAN_POINT('Ctrl Pts',(-16.4953342248032,21.8031719099425,0.392363112479807));
#48526=CARTESIAN_POINT('Ctrl Pts',(-16.4945912578509,21.8270423251592,0.42359817971177));
#48527=CARTESIAN_POINT('Ctrl Pts',(-16.4937314527037,21.8488302173248,0.456017327146848));
#48528=CARTESIAN_POINT('Ctrl Pts',(-16.4927345257884,21.8685708106081,0.489599721324281));
#48529=CARTESIAN_POINT('Ctrl Pts',(-16.4926692122777,21.8698641124863,0.491799866620864));
#48530=CARTESIAN_POINT('Ctrl Pts',(-16.4926033098955,21.8711486154602,0.494005011689312));
#48531=CARTESIAN_POINT('Ctrl Pts',(-16.4925368128699,21.8724243299332,0.49621515106008));
#48532=CARTESIAN_POINT('Ctrl Pts',(-16.491512221602,21.8920806363306,0.530269147916579));
#48533=CARTESIAN_POINT('Ctrl Pts',(-16.490346617639,21.9096504663962,0.565508710461108));
#48534=CARTESIAN_POINT('Ctrl Pts',(-16.4890155715004,21.9250723817395,0.601968047138723));
#48535=CARTESIAN_POINT('Ctrl Pts',(-16.488946257453,21.9258754758924,0.603866662158586));
#48536=CARTESIAN_POINT('Ctrl Pts',(-16.4888764943784,21.9266727342239,0.605768592818671));
#48537=CARTESIAN_POINT('Ctrl Pts',(-16.4888062788131,21.9274641490614,0.607673843251827));
#48538=CARTESIAN_POINT('Ctrl Pts',(-16.488517527398,21.9307187287754,0.615508911683253));
#48539=CARTESIAN_POINT('Ctrl Pts',(-16.4882211081858,21.9338741041944,0.62340032606399));
#48540=CARTESIAN_POINT('Ctrl Pts',(-16.4879167508124,21.9369290908268,0.631348731739397));
#48541=CARTESIAN_POINT('Ctrl Pts',(-16.487848077967,21.9376183943997,0.633142148565797));
#48542=CARTESIAN_POINT('Ctrl Pts',(-16.4877789945818,21.9383026502421,0.63493863384876));
#48543=CARTESIAN_POINT('Ctrl Pts',(-16.4877095008555,21.9389818061129,0.636738105814736));
#48544=CARTESIAN_POINT('Ctrl Pts',(-16.487396103929,21.9420446057924,0.644853212224946));
#48545=CARTESIAN_POINT('Ctrl Pts',(-16.4870740546098,21.9450055504829,0.653036041884953));
#48546=CARTESIAN_POINT('Ctrl Pts',(-16.4867453299528,21.9478453209401,0.661232434512168));
#48547=CARTESIAN_POINT('Ctrl Pts',(-16.4866783910109,21.9484235897912,0.66290148439462));
#48548=CARTESIAN_POINT('Ctrl Pts',(-16.4866111636593,21.9489969449142,0.664571390435223));
#48549=CARTESIAN_POINT('Ctrl Pts',(-16.4865436620896,21.9495652434028,0.666241756430982));
#48550=CARTESIAN_POINT('Ctrl Pts',(-16.4858011779881,21.9558162475649,0.684614961712526));
#48551=CARTESIAN_POINT('Ctrl Pts',(-16.4850234343973,21.9614778442179,0.703099012587878));
#48552=CARTESIAN_POINT('Ctrl Pts',(-16.4842100219045,21.9665568108032,0.721678566231952));
#48553=CARTESIAN_POINT('Ctrl Pts',(-16.4841497338362,21.9669332509083,0.723055635564778));
#48554=CARTESIAN_POINT('Ctrl Pts',(-16.4840892488147,21.9673064991026,0.724433254441731));
#48555=CARTESIAN_POINT('Ctrl Pts',(-16.4840285664534,21.9676765602153,0.725811422028464));
#48556=CARTESIAN_POINT('Ctrl Pts',(-16.4823029170785,21.9782001409525,0.765002943035284));
#48557=CARTESIAN_POINT('Ctrl Pts',(-16.4804177593127,21.9861539386864,0.804636913831577));
#48558=CARTESIAN_POINT('Ctrl Pts',(-16.4783635401719,21.9915540521472,0.844710032025303));
#48559=CARTESIAN_POINT('Ctrl Pts',(-16.4783260674647,21.9916525600749,0.845441038856458));
#48560=CARTESIAN_POINT('Ctrl Pts',(-16.478288538507,21.9917502179696,0.846172191647967));
#48561=CARTESIAN_POINT('Ctrl Pts',(-16.4782509532398,21.9918470259295,0.846903490398947));
#48562=CARTESIAN_POINT('Ctrl Pts',(-16.476155695451,21.9972437584032,0.88767104425426));
#48563=CARTESIAN_POINT('Ctrl Pts',(-16.473885478833,21.9999999929008,0.928892770239698));
#48564=CARTESIAN_POINT('Ctrl Pts',(-16.4714285499925,22.,0.970588235294111));
#48565=CARTESIAN_POINT('',(-16.20259362019,22.0000000000005,3.11864719131614));
#48566=CARTESIAN_POINT('Origin',(6.61363325216158E-15,22.,8.67361737988404E-16));
#48567=CARTESIAN_POINT('',(-12.9440892692056,20.5440037453176,10.2323288156136));
#48568=CARTESIAN_POINT('Ctrl Pts',(-16.2025936491961,22.0000000000008,3.11864719690075));
#48569=CARTESIAN_POINT('Ctrl Pts',(-16.2007285738033,22.0380649929751,3.12833708065861));
#48570=CARTESIAN_POINT('Ctrl Pts',(-16.1987464412966,22.076002889804,3.13858807784552));
#48571=CARTESIAN_POINT('Ctrl Pts',(-16.1966434424578,22.113812826353,3.14940330822996));
#48572=CARTESIAN_POINT('Ctrl Pts',(-16.1954407636136,22.1354358581637,3.15558840378915));
#48573=CARTESIAN_POINT('Ctrl Pts',(-16.1941985162796,22.1570170203631,3.16195812198267));
#48574=CARTESIAN_POINT('Ctrl Pts',(-16.1929158191893,22.1785560753722,3.16851342763732));
#48575=CARTESIAN_POINT('Ctrl Pts',(-16.1923820249429,22.1875195506344,3.17124141733076));
#48576=CARTESIAN_POINT('Ctrl Pts',(-16.1918415464089,22.1964703807905,3.17399990822218));
#48577=CARTESIAN_POINT('Ctrl Pts',(-16.1912942180195,22.2054106120283,3.17678950286713));
#48578=CARTESIAN_POINT('Ctrl Pts',(-16.1903609681165,22.2206546046626,3.18154604205381));
#48579=CARTESIAN_POINT('Ctrl Pts',(-16.1894050293091,22.2359116524264,3.18640708997119));
#48580=CARTESIAN_POINT('Ctrl Pts',(-16.188431284714,22.2510992279796,3.19134650893528));
#48581=CARTESIAN_POINT('Ctrl Pts',(-16.1880901743651,22.2564195545014,3.19307682603722));
#48582=CARTESIAN_POINT('Ctrl Pts',(-16.1877467681858,22.2617332382891,3.19481732744566));
#48583=CARTESIAN_POINT('Ctrl Pts',(-16.1874010331489,22.2670407278125,3.19656812763937));
#48584=CARTESIAN_POINT('Ctrl Pts',(-16.1867593824459,22.2768909137073,3.19981744302596));
#48585=CARTESIAN_POINT('Ctrl Pts',(-16.1861095468107,22.2867219813628,3.20310305888488));
#48586=CARTESIAN_POINT('Ctrl Pts',(-16.1854514865211,22.2965339989238,3.20642482797795));
#48587=CARTESIAN_POINT('Ctrl Pts',(-16.1841491605544,22.3159523492761,3.21299873346044));
#48588=CARTESIAN_POINT('Ctrl Pts',(-16.1828147481359,22.3352962992668,3.21971388856837));
#48589=CARTESIAN_POINT('Ctrl Pts',(-16.1814477998186,22.354566151568,3.22656954932038));
#48590=CARTESIAN_POINT('Ctrl Pts',(-16.1743353285268,22.4548305650421,3.26224075185642));
#48591=CARTESIAN_POINT('Ctrl Pts',(-16.1663424831819,22.5530897779929,3.301714432485));
#48592=CARTESIAN_POINT('Ctrl Pts',(-16.1573962736503,22.6493676325255,3.34492834844848));
#48593=CARTESIAN_POINT('Ctrl Pts',(-16.1559898083244,22.6645038154616,3.35172216142433));
#48594=CARTESIAN_POINT('Ctrl Pts',(-16.154559779912,22.6795910150878,3.3586084292314));
#48595=CARTESIAN_POINT('Ctrl Pts',(-16.1531057632547,22.6946291085995,3.36558724834429));
#48596=CARTESIAN_POINT('Ctrl Pts',(-16.1435883678908,22.793062287306,3.41126772960764));
#48597=CARTESIAN_POINT('Ctrl Pts',(-16.1330447934926,22.8893959143685,3.46090714479232));
#48598=CARTESIAN_POINT('Ctrl Pts',(-16.1213537652987,22.983602889284,3.51453450318926));
#48599=CARTESIAN_POINT('Ctrl Pts',(-16.1198977674386,22.9953354034488,3.52121324160092));
#48600=CARTESIAN_POINT('Ctrl Pts',(-16.1184239776341,23.0070349326023,3.52795382961854));
#48601=CARTESIAN_POINT('Ctrl Pts',(-16.1169320732323,23.0187013074004,3.53475650588613));
#48602=CARTESIAN_POINT('Ctrl Pts',(-16.104683326423,23.1144838997095,3.59060744320198));
#48603=CARTESIAN_POINT('Ctrl Pts',(-16.0912152664552,23.2080355812782,3.65063731207971));
#48604=CARTESIAN_POINT('Ctrl Pts',(-16.0763458930289,23.2992682237434,3.71498354339455));
#48605=CARTESIAN_POINT('Ctrl Pts',(-16.0748618388374,23.3083737981056,3.72140568987996));
#48606=CARTESIAN_POINT('Ctrl Pts',(-16.0733637723816,23.3174562066199,3.72787093347258));
#48607=CARTESIAN_POINT('Ctrl Pts',(-16.071851478507,23.3265153204774,3.73437947411941));
#48608=CARTESIAN_POINT('Ctrl Pts',(-16.0712451133794,23.3301476374644,3.73698912039648));
#48609=CARTESIAN_POINT('Ctrl Pts',(-16.0706364514506,23.3337762715684,3.73960576817669));
#48610=CARTESIAN_POINT('Ctrl Pts',(-16.0700255132432,23.3374010109535,3.74222928262171));
#48611=CARTESIAN_POINT('Ctrl Pts',(-16.0685376647248,23.3462285209347,3.74861845919112));
#48612=CARTESIAN_POINT('Ctrl Pts',(-16.0670366490278,23.3550307520345,3.7550468950703));
#48613=CARTESIAN_POINT('Ctrl Pts',(-16.0655247928919,23.363793655777,3.76150409636277));
#48614=CARTESIAN_POINT('Ctrl Pts',(-16.0648683173262,23.367598668737,3.7643079311789));
#48615=CARTESIAN_POINT('Ctrl Pts',(-16.0642096111748,23.3713973521618,3.76711798752819));
#48616=CARTESIAN_POINT('Ctrl Pts',(-16.063548842397,23.3751886669207,3.76993349913855));
#48617=CARTESIAN_POINT('Ctrl Pts',(-16.0620630117603,23.3837139662545,3.77626456917164));
#48618=CARTESIAN_POINT('Ctrl Pts',(-16.0605660425622,23.392206247396,3.78262627293113));
#48619=CARTESIAN_POINT('Ctrl Pts',(-16.0590580817749,23.4006642630481,3.78901748951433));
#48620=CARTESIAN_POINT('Ctrl Pts',(-16.0561407034788,23.4170275740167,3.80138226497942));
#48621=CARTESIAN_POINT('Ctrl Pts',(-16.053181928325,23.4332641387232,3.81385859904748));
#48622=CARTESIAN_POINT('Ctrl Pts',(-16.0501811226695,23.4493747077355,3.82644559996654));
#48623=CARTESIAN_POINT('Ctrl Pts',(-16.048700186204,23.4573254822511,3.83265744798126));
#48624=CARTESIAN_POINT('Ctrl Pts',(-16.0472090166894,23.4652455849803,3.83889623746635));
#48625=CARTESIAN_POINT('Ctrl Pts',(-16.0457075303997,23.4731350759295,3.84516188518223));
#48626=CARTESIAN_POINT('Ctrl Pts',(-16.0379996871877,23.5136355851095,3.87732643476738));
#48627=CARTESIAN_POINT('Ctrl Pts',(-16.0300200108983,23.5533296060536,3.91019866626501));
#48628=CARTESIAN_POINT('Ctrl Pts',(-16.0217569622216,23.592225091995,3.94376772179914));
#48629=CARTESIAN_POINT('Ctrl Pts',(-16.0202775371902,23.5991889812037,3.94977796123755));
#48630=CARTESIAN_POINT('Ctrl Pts',(-16.0187890414494,23.6061273175812,3.95581050241583));
#48631=CARTESIAN_POINT('Ctrl Pts',(-16.0172913967662,23.6130401043791,3.96186531572998));
#48632=CARTESIAN_POINT('Ctrl Pts',(-15.9988886073062,23.6979831896424,4.03626577659036));
#48633=CARTESIAN_POINT('Ctrl Pts',(-15.9791056210773,23.7790726584468,4.11402593979942));
#48634=CARTESIAN_POINT('Ctrl Pts',(-15.9577944161881,23.856323891952,4.19509205747428));
#48635=CARTESIAN_POINT('Ctrl Pts',(-15.9562633431416,23.8618738963764,4.20091613679774));
#48636=CARTESIAN_POINT('Ctrl Pts',(-15.9547243824016,23.8674040880027,4.20675728039115));
#48637=CARTESIAN_POINT('Ctrl Pts',(-15.9531774663352,23.8729144364266,4.21261549553058));
#48638=CARTESIAN_POINT('Ctrl Pts',(-15.9315756165195,23.9498634847105,4.294422315163));
#48639=CARTESIAN_POINT('Ctrl Pts',(-15.9084236027008,24.0229466751676,4.37955564841957));
#48640=CARTESIAN_POINT('Ctrl Pts',(-15.8835326793682,24.092086587039,4.46804091559637));
#48641=CARTESIAN_POINT('Ctrl Pts',(-15.8818310324434,24.0968132786463,4.4740901360599));
#48642=CARTESIAN_POINT('Ctrl Pts',(-15.8801212452089,24.1015215089774,4.48015504546405));
#48643=CARTESIAN_POINT('Ctrl Pts',(-15.8784032469458,24.1062112288154,4.48623566993863));
#48644=CARTESIAN_POINT('Ctrl Pts',(-15.8667154020255,24.1381162192709,4.52760322973444));
#48645=CARTESIAN_POINT('Ctrl Pts',(-15.854647612731,24.1691649603628,4.5696979166866));
#48646=CARTESIAN_POINT('Ctrl Pts',(-15.8421772586022,24.1993421971384,4.61252855893889));
#48647=CARTESIAN_POINT('Ctrl Pts',(-15.8403248125551,24.2038249650214,4.61889096477889));
#48648=CARTESIAN_POINT('Ctrl Pts',(-15.8384634783031,24.2082884910049,4.62526961845721));
#48649=CARTESIAN_POINT('Ctrl Pts',(-15.8365931763335,24.2127327135982,4.63166455724276));
#48650=CARTESIAN_POINT('Ctrl Pts',(-15.8348597372067,24.2168517218954,4.6375915344283));
#48651=CARTESIAN_POINT('Ctrl Pts',(-15.8331187534389,24.2209537913896,4.64353195877213));
#48652=CARTESIAN_POINT('Ctrl Pts',(-15.8313700238803,24.225039196167,4.64948633366989));
#48653=CARTESIAN_POINT('Ctrl Pts',(-15.8294716493301,24.2294742035238,4.6559502455501));
#48654=CARTESIAN_POINT('Ctrl Pts',(-15.8275633970074,24.2338912489374,4.66243312324216));
#48655=CARTESIAN_POINT('Ctrl Pts',(-15.8256464412423,24.2382874378699,4.6689307713959));
#48656=CARTESIAN_POINT('Ctrl Pts',(-15.8238950452432,24.2423039456306,4.67486724378985));
#48657=CARTESIAN_POINT('Ctrl Pts',(-15.8221363144475,24.2463032099063,4.68081628009433));
#48658=CARTESIAN_POINT('Ctrl Pts',(-15.8203715407341,24.2502821258543,4.68677333707624));
#48659=CARTESIAN_POINT('Ctrl Pts',(-15.8184253822281,24.2546699978282,4.6933426649334));
#48660=CARTESIAN_POINT('Ctrl Pts',(-15.8164722187656,24.2590324257771,4.69992061175821));
#48661=CARTESIAN_POINT('Ctrl Pts',(-15.8145123720079,24.263368748324,4.70650596817048));
#48662=CARTESIAN_POINT('Ctrl Pts',(-15.8090339354155,24.2754902409986,4.72491427351423));
#48663=CARTESIAN_POINT('Ctrl Pts',(-15.8035010071365,24.2874125709219,4.74338811479279));
#48664=CARTESIAN_POINT('Ctrl Pts',(-15.7979130801256,24.2991380625097,4.76192632374751));
#48665=CARTESIAN_POINT('Ctrl Pts',(-15.7958775667432,24.303409305673,4.76867923450323));
#48666=CARTESIAN_POINT('Ctrl Pts',(-15.7938347604507,24.3076544889671,4.77544066605381));
#48667=CARTESIAN_POINT('Ctrl Pts',(-15.791784633935,24.3118736919458,4.78221057381387));
#48668=CARTESIAN_POINT('Ctrl Pts',(-15.7633442780802,24.3704045353914,4.87612603918684));
#48669=CARTESIAN_POINT('Ctrl Pts',(-15.7334953011493,24.4239355410877,4.97167279196691));
#48670=CARTESIAN_POINT('Ctrl Pts',(-15.7021601295571,24.4726571112215,5.06874415074919));
#48671=CARTESIAN_POINT('Ctrl Pts',(-15.699656516845,24.4765498597256,5.0764999432175));
#48672=CARTESIAN_POINT('Ctrl Pts',(-15.6971434172225,24.4804118997891,5.08426546999268));
#48673=CARTESIAN_POINT('Ctrl Pts',(-15.6946207847607,24.4842432686933,5.09204069647819));
#48674=CARTESIAN_POINT('Ctrl Pts',(-15.6634240457132,24.5316248106776,5.18819489863686));
#48675=CARTESIAN_POINT('Ctrl Pts',(-15.6307698276384,24.5743194217589,5.2858316951789));
#48676=CARTESIAN_POINT('Ctrl Pts',(-15.5965690625268,24.6124021579424,5.3848893654224));
#48677=CARTESIAN_POINT('Ctrl Pts',(-15.5933907822553,24.6159411901455,5.39409480389885));
#48678=CARTESIAN_POINT('Ctrl Pts',(-15.5901991470769,24.6194403916291,5.40331251334931));
#48679=CARTESIAN_POINT('Ctrl Pts',(-15.5869940737593,24.6228997410832,5.41254247021877));
#48680=CARTESIAN_POINT('Ctrl Pts',(-15.5530605223862,24.6595254281681,5.51026417096084));
#48681=CARTESIAN_POINT('Ctrl Pts',(-15.5176212035088,24.6916877662491,5.60935762993737));
#48682=CARTESIAN_POINT('Ctrl Pts',(-15.4805748894808,24.7193633611184,5.70979869095014));
#48683=CARTESIAN_POINT('Ctrl Pts',(-15.476469324288,24.7224304397729,5.72092982058731));
#48684=CARTESIAN_POINT('Ctrl Pts',(-15.4723440086735,24.7254423332042,5.73207752534907));
#48685=CARTESIAN_POINT('Ctrl Pts',(-15.4681987867402,24.7283989099965,5.74324180268951));
#48686=CARTESIAN_POINT('Ctrl Pts',(-15.4519326446998,24.740000725009,5.78705121118856));
#48687=CARTESIAN_POINT('Ctrl Pts',(-15.4353600150741,24.7507511884474,5.83111573139675));
#48688=CARTESIAN_POINT('Ctrl Pts',(-15.4184713230428,24.7606424131365,5.87543547837171));
#48689=CARTESIAN_POINT('Ctrl Pts',(-15.4137902225723,24.7633840000196,5.88771974455598));
#48690=CARTESIAN_POINT('Ctrl Pts',(-15.4090848343034,24.7660595443407,5.90002362803513));
#48691=CARTESIAN_POINT('Ctrl Pts',(-15.4043549426926,24.768668821489,5.9123471481084));
#48692=CARTESIAN_POINT('Ctrl Pts',(-15.4037377466213,24.769009301935,5.9139552247411));
#48693=CARTESIAN_POINT('Ctrl Pts',(-15.4031201219804,24.7693486604333,5.91556366528412));
#48694=CARTESIAN_POINT('Ctrl Pts',(-15.4025020739784,24.7696868932433,5.91717245490538));
#48695=CARTESIAN_POINT('Ctrl Pts',(-15.3976639474252,24.7723346052877,5.9297661818648));
#48696=CARTESIAN_POINT('Ctrl Pts',(-15.3928004416522,24.7749128458777,5.94237973041235));
#48697=CARTESIAN_POINT('Ctrl Pts',(-15.3879251262603,24.7774148313734,5.95497777334009));
#48698=CARTESIAN_POINT('Ctrl Pts',(-15.3874066974078,24.7776808862571,5.95631741773523));
#48699=CARTESIAN_POINT('Ctrl Pts',(-15.3868881094435,24.7779460925336,5.95765695307419));
#48700=CARTESIAN_POINT('Ctrl Pts',(-15.3863693767468,24.7782104429972,5.95899634186062));
#48701=CARTESIAN_POINT('Ctrl Pts',(-15.3813867729795,24.7807496190012,5.97186162615066));
#48702=CARTESIAN_POINT('Ctrl Pts',(-15.3763875592422,24.7832116475652,5.98472187761016));
#48703=CARTESIAN_POINT('Ctrl Pts',(-15.3713729754319,24.7855965717697,5.99757391400886));
#48704=CARTESIAN_POINT('Ctrl Pts',(-15.3655247331818,24.7883779819573,6.01256256014777));
#48705=CARTESIAN_POINT('Ctrl Pts',(-15.3596550017188,24.7910548193452,6.02754153987971));
#48706=CARTESIAN_POINT('Ctrl Pts',(-15.353763791016,24.7936280765825,6.04251085639781));
#48707=CARTESIAN_POINT('Ctrl Pts',(-15.3485003517419,24.7959271257744,6.05588503234282));
#48708=CARTESIAN_POINT('Ctrl Pts',(-15.3432197688761,24.7981436780431,6.06925149589424));
#48709=CARTESIAN_POINT('Ctrl Pts',(-15.3379220487496,24.8002782541417,6.08261024575491));
#48710=CARTESIAN_POINT('Ctrl Pts',(-15.2991635046816,24.8158949835662,6.18034392794347));
#48711=CARTESIAN_POINT('Ctrl Pts',(-15.2594875723158,24.8271341266431,6.27766502745761));
#48712=CARTESIAN_POINT('Ctrl Pts',(-15.2188960426122,24.8342169899472,6.37457475006575));
#48713=CARTESIAN_POINT('Ctrl Pts',(-15.2124545056988,24.8353409812271,6.38995351405937));
#48714=CARTESIAN_POINT('Ctrl Pts',(-15.2059899125782,24.8363602703669,6.40532191504176));
#48715=CARTESIAN_POINT('Ctrl Pts',(-15.1995022675384,24.8372753461937,6.42067995159775));
#48716=CARTESIAN_POINT('Ctrl Pts',(-15.1595189390471,24.8429149545807,6.51533146487176));
#48717=CARTESIAN_POINT('Ctrl Pts',(-15.1186599228528,24.8446016656592,6.60958959202436));
#48718=CARTESIAN_POINT('Ctrl Pts',(-15.076925813321,24.8424503931545,6.70345493157287));
#48719=CARTESIAN_POINT('Ctrl Pts',(-15.069215981448,24.8420529736454,6.72079532758813));
#48720=CARTESIAN_POINT('Ctrl Pts',(-15.0614762860052,24.8415245576396,6.73812231536534));
#48721=CARTESIAN_POINT('Ctrl Pts',(-15.0537067262432,24.8408653570098,6.75543589059264));
#48722=CARTESIAN_POINT('Ctrl Pts',(-15.0125937514738,24.8373771672421,6.84705145225807));
#48723=CARTESIAN_POINT('Ctrl Pts',(-14.970644518116,24.8302323129595,6.93829155693857));
#48724=CARTESIAN_POINT('Ctrl Pts',(-14.9278586228369,24.8194623041218,7.02915620374142));
#48725=CARTESIAN_POINT('Ctrl Pts',(-14.9187900350446,24.8171795712252,7.04841521471614));
#48726=CARTESIAN_POINT('Ctrl Pts',(-14.9096838594696,24.8147337373671,7.06765735337678));
#48727=CARTESIAN_POINT('Ctrl Pts',(-14.9005400880507,24.8121245721257,7.08688261044366));
#48728=CARTESIAN_POINT('Ctrl Pts',(-14.8840368164733,24.8074153815087,7.12158160104474));
#48729=CARTESIAN_POINT('Ctrl Pts',(-14.8674110679554,24.8021745077348,7.15622561418776));
#48730=CARTESIAN_POINT('Ctrl Pts',(-14.8506627812048,24.7964006907752,7.19081462415348));
#48731=CARTESIAN_POINT('Ctrl Pts',(-14.8408807561578,24.79302842811,7.2110167240382));
#48732=CARTESIAN_POINT('Ctrl Pts',(-14.831056929161,24.7894742940814,7.23120006011304));
#48733=CARTESIAN_POINT('Ctrl Pts',(-14.8211912848237,24.7857377155243,7.25136462334682));
#48734=CARTESIAN_POINT('Ctrl Pts',(-14.8179315553191,24.7845031042863,7.25802724156755));
#48735=CARTESIAN_POINT('Ctrl Pts',(-14.8146674293716,24.7832486492219,7.26468746547449));
#48736=CARTESIAN_POINT('Ctrl Pts',(-14.8113987894915,24.7819742863765,7.27134553563859));
#48737=CARTESIAN_POINT('Ctrl Pts',(-14.8048178735146,24.7794085479907,7.28475056094716));
#48738=CARTESIAN_POINT('Ctrl Pts',(-14.7982186612007,24.7767621098732,7.29814685649007));
#48739=CARTESIAN_POINT('Ctrl Pts',(-14.7916001771697,24.7740343302663,7.31153637744859));
#48740=CARTESIAN_POINT('Ctrl Pts',(-14.7880142587479,24.7725564094771,7.31879086799941));
#48741=CARTESIAN_POINT('Ctrl Pts',(-14.7844216216961,24.7710541341929,7.32604549272862));
#48742=CARTESIAN_POINT('Ctrl Pts',(-14.7808248885348,24.7695286159718,7.33329498920607));
#48743=CARTESIAN_POINT('Ctrl Pts',(-14.7777839200856,24.7682388197677,7.33942429851873));
#48744=CARTESIAN_POINT('Ctrl Pts',(-14.7747407828823,24.7669327178474,7.3455484114189));
#48745=CARTESIAN_POINT('Ctrl Pts',(-14.7716970861947,24.7656110144841,7.35166411050637));
#48746=CARTESIAN_POINT('Ctrl Pts',(-14.761196250836,24.7610511023656,7.37276343669141));
#48747=CARTESIAN_POINT('Ctrl Pts',(-14.7506837912226,24.7563041603517,7.39377288964028));
#48748=CARTESIAN_POINT('Ctrl Pts',(-14.7401572275992,24.7513709251904,7.41469939794161));
#48749=CARTESIAN_POINT('Ctrl Pts',(-14.6973102122001,24.7312908296831,7.49987804270287));
#48750=CARTESIAN_POINT('Ctrl Pts',(-14.6542479183378,24.7081389531941,7.58364572268321));
#48751=CARTESIAN_POINT('Ctrl Pts',(-14.6110004483275,24.6820430612744,7.66607239067015));
#48752=CARTESIAN_POINT('Ctrl Pts',(-14.5994294499354,24.6750610222471,7.68812590830979));
#48753=CARTESIAN_POINT('Ctrl Pts',(-14.5878451889963,24.6678681797709,7.71008339601883));
#48754=CARTESIAN_POINT('Ctrl Pts',(-14.5762483668385,24.6604656595606,7.73194574887356));
#48755=CARTESIAN_POINT('Ctrl Pts',(-14.5336920324701,24.6333009655649,7.81217303747932));
#48756=CARTESIAN_POINT('Ctrl Pts',(-14.4909656746514,24.6033180861438,7.89112095375525));
#48757=CARTESIAN_POINT('Ctrl Pts',(-14.4481043018837,24.5705726924211,7.9688319145224));
#48758=CARTESIAN_POINT('Ctrl Pts',(-14.435631055481,24.5610433344449,7.99144686824979));
#48759=CARTESIAN_POINT('Ctrl Pts',(-14.4231463598431,24.551280024261,8.01395704999258));
#48760=CARTESIAN_POINT('Ctrl Pts',(-14.4106512663725,24.5412826396292,8.03636303047209));
#48761=CARTESIAN_POINT('Ctrl Pts',(-14.368350330057,24.5074374561882,8.1122163208515));
#48762=CARTESIAN_POINT('Ctrl Pts',(-14.3259294292655,24.4709147430595,8.18687686290484));
#48763=CARTESIAN_POINT('Ctrl Pts',(-14.2834297196491,24.4317100865886,8.26036533355924));
#48764=CARTESIAN_POINT('Ctrl Pts',(-14.2702374163509,24.4195405982901,8.28317683515631));
#48765=CARTESIAN_POINT('Ctrl Pts',(-14.2570374921994,24.4071127715725,8.30587540847742));
#48766=CARTESIAN_POINT('Ctrl Pts',(-14.2438314706936,24.3944246468114,8.32846112690485));
#48767=CARTESIAN_POINT('Ctrl Pts',(-14.2159565081634,24.3676428486639,8.37613453517622));
#48768=CARTESIAN_POINT('Ctrl Pts',(-14.1880541401679,24.3397031404335,8.4233055533928));
#48769=CARTESIAN_POINT('Ctrl Pts',(-14.1601384898672,24.3105891204553,8.46997506646264));
#48770=CARTESIAN_POINT('Ctrl Pts',(-14.1461806647169,24.2960321104662,8.49330982299757));
#48771=CARTESIAN_POINT('Ctrl Pts',(-14.1322195167082,24.2811815214874,8.51651920302677));
#48772=CARTESIAN_POINT('Ctrl Pts',(-14.1182570229551,24.2660341768511,8.53960295526646));
#48773=CARTESIAN_POINT('Ctrl Pts',(-14.1180026993283,24.2657582714368,8.54002342052814));
#48774=CARTESIAN_POINT('Ctrl Pts',(-14.1177483689363,24.2654822610159,8.54044385455583));
#48775=CARTESIAN_POINT('Ctrl Pts',(-14.1174940323106,24.2652061461278,8.54086425648329));
#48776=CARTESIAN_POINT('Ctrl Pts',(-14.1107667652363,24.2579028385899,8.55198399213569));
#48777=CARTESIAN_POINT('Ctrl Pts',(-14.1040377514951,24.2505288686595,8.56307686259749));
#48778=CARTESIAN_POINT('Ctrl Pts',(-14.0973217926706,24.243100392135,8.57411904861985));
#48779=CARTESIAN_POINT('Ctrl Pts',(-14.0903519247494,24.2353910684802,8.58557870466419));
#48780=CARTESIAN_POINT('Ctrl Pts',(-14.0833932795755,24.2276198183536,8.59698848455036));
#48781=CARTESIAN_POINT('Ctrl Pts',(-14.0764459696852,24.2197869328603,8.60834878828686));
#48782=CARTESIAN_POINT('Ctrl Pts',(-14.0762845790342,24.2196049696963,8.60861269573363));
#48783=CARTESIAN_POINT('Ctrl Pts',(-14.0761231961318,24.2194229749766,8.60887657380321));
#48784=CARTESIAN_POINT('Ctrl Pts',(-14.07596182105,24.2192409487787,8.60914042238491));
#48785=CARTESIAN_POINT('Ctrl Pts',(-14.0621446620437,24.2036556124843,8.63173150501409));
#48786=CARTESIAN_POINT('Ctrl Pts',(-14.0483724087833,24.1878261032494,8.65412699149244));
#48787=CARTESIAN_POINT('Ctrl Pts',(-14.0346469182352,24.171753729845,8.67632905556684));
#48788=CARTESIAN_POINT('Ctrl Pts',(-14.0071500385025,24.1395552363216,8.72080742838211));
#48789=CARTESIAN_POINT('Ctrl Pts',(-13.9798407035581,24.10638250377,8.76450982437772));
#48790=CARTESIAN_POINT('Ctrl Pts',(-13.9527353713041,24.0722403709581,8.80745000884873));
#48791=CARTESIAN_POINT('Ctrl Pts',(-13.939110440033,24.0550782786933,8.82903458330466));
#48792=CARTESIAN_POINT('Ctrl Pts',(-13.9255368723932,24.037671755944,8.85042686711888));
#48793=CARTESIAN_POINT('Ctrl Pts',(-13.9120172216432,24.0200199465187,8.87162769785873));
#48794=CARTESIAN_POINT('Ctrl Pts',(-13.8715627914303,23.9672009864928,8.93506628391983));
#48795=CARTESIAN_POINT('Ctrl Pts',(-13.8315892997756,23.9121884637842,8.99679365402703));
#48796=CARTESIAN_POINT('Ctrl Pts',(-13.792165484045,23.8549566280595,9.05683008898569));
#48797=CARTESIAN_POINT('Ctrl Pts',(-13.7789671094322,23.8357964530822,9.0769291926446));
#48798=CARTESIAN_POINT('Ctrl Pts',(-13.7658302672435,23.816387664989,9.09683881806451));
#48799=CARTESIAN_POINT('Ctrl Pts',(-13.7527583233579,23.7967271682685,9.11655844889056));
#48800=CARTESIAN_POINT('Ctrl Pts',(-13.7134944654266,23.7376734455135,9.17578979122058));
#48801=CARTESIAN_POINT('Ctrl Pts',(-13.6748140062712,23.6763543421238,9.23331031479049));
#48802=CARTESIAN_POINT('Ctrl Pts',(-13.6368080138338,23.6126902613882,9.28910475739456));
#48803=CARTESIAN_POINT('Ctrl Pts',(-13.6243655648898,23.5918478356728,9.30737081121752));
#48804=CARTESIAN_POINT('Ctrl Pts',(-13.6119956065496,23.5707535567129,9.32545155666013));
#48805=CARTESIAN_POINT('Ctrl Pts',(-13.5997020461054,23.5494028742049,9.34334544254682));
#48806=CARTESIAN_POINT('Ctrl Pts',(-13.5872408544575,23.5277610603664,9.36148332394995));
#48807=CARTESIAN_POINT('Ctrl Pts',(-13.5748580142948,23.5058562285921,9.37942942446946));
#48808=CARTESIAN_POINT('Ctrl Pts',(-13.5625576774649,23.4836835500919,9.39718198423395));
#48809=CARTESIAN_POINT('Ctrl Pts',(-13.5622002858085,23.4830393132384,9.39769779260794));
#48810=CARTESIAN_POINT('Ctrl Pts',(-13.5618429499553,23.4823948255231,9.39821345757555));
#48811=CARTESIAN_POINT('Ctrl Pts',(-13.5614856716924,23.4817500898084,9.39872897664797));
#48812=CARTESIAN_POINT('Ctrl Pts',(-13.5556947328696,23.4712999016273,9.40708475901662));
#48813=CARTESIAN_POINT('Ctrl Pts',(-13.5499210866683,23.4607881047525,9.41539904702796));
#48814=CARTESIAN_POINT('Ctrl Pts',(-13.5441763047212,23.4502351047131,9.4236557490121));
#48815=CARTESIAN_POINT('Ctrl Pts',(-13.5380770922097,23.4390310258696,9.43242185719667));
#48816=CARTESIAN_POINT('Ctrl Pts',(-13.5320084142969,23.4277769507785,9.44112595533259));
#48817=CARTESIAN_POINT('Ctrl Pts',(-13.5259706946607,23.4164726630393,9.44976807943773));
#48818=CARTESIAN_POINT('Ctrl Pts',(-13.5255027633295,23.4155965656501,9.45043785559172));
#48819=CARTESIAN_POINT('Ctrl Pts',(-13.5250350313337,23.4147201914592,9.45110724028288));
#48820=CARTESIAN_POINT('Ctrl Pts',(-13.5245675011861,23.4138435446244,9.45177623020461));
#48821=CARTESIAN_POINT('Ctrl Pts',(-13.5123698737289,23.3909722676434,9.46922984229624));
#48822=CARTESIAN_POINT('Ctrl Pts',(-13.500298009852,23.3678945493989,9.48643154991876));
#48823=CARTESIAN_POINT('Ctrl Pts',(-13.4883559012739,23.3446105257168,9.50338124461869));
#48824=CARTESIAN_POINT('Ctrl Pts',(-13.4771310581609,23.3227249842178,9.51931290882832));
#48825=CARTESIAN_POINT('Ctrl Pts',(-13.4660205123182,23.3006577021536,9.5350224652864));
#48826=CARTESIAN_POINT('Ctrl Pts',(-13.4550281249885,23.2784079358377,9.5505089073953));
#48827=CARTESIAN_POINT('Ctrl Pts',(-13.4190914907655,23.2056683489166,9.60113763696881));
#48828=CARTESIAN_POINT('Ctrl Pts',(-13.3844104675413,23.1309760363863,9.64939219710768));
#48829=CARTESIAN_POINT('Ctrl Pts',(-13.351102074414,23.0542737878051,9.69526035744458));
#48830=CARTESIAN_POINT('Ctrl Pts',(-13.3415236222338,23.0322166198911,9.7084506058815));
#48831=CARTESIAN_POINT('Ctrl Pts',(-13.3320585708577,23.0099933738321,9.72144360699642));
#48832=CARTESIAN_POINT('Ctrl Pts',(-13.3227106391527,22.9876013095394,9.7342376265637));
#48833=CARTESIAN_POINT('Ctrl Pts',(-13.2893807312244,22.9077627458071,9.77985450820822));
#48834=CARTESIAN_POINT('Ctrl Pts',(-13.2575356335838,22.8257836447286,9.82294763255116));
#48835=CARTESIAN_POINT('Ctrl Pts',(-13.2273415092598,22.7415472155431,9.86343938985887));
#48836=CARTESIAN_POINT('Ctrl Pts',(-13.2196187511697,22.7200020447678,9.87379597589437));
#48837=CARTESIAN_POINT('Ctrl Pts',(-13.2120043126901,22.6983087533948,9.88398192053575));
#48838=CARTESIAN_POINT('Ctrl Pts',(-13.2045015037799,22.6764646402634,9.89399515055105));
#48839=CARTESIAN_POINT('Ctrl Pts',(-13.2025807266856,22.6708723783987,9.89655861485929));
#48840=CARTESIAN_POINT('Ctrl Pts',(-13.2006673073772,22.6652703809769,9.89911070390188));
#48841=CARTESIAN_POINT('Ctrl Pts',(-13.198761277514,22.6596585418442,9.90165141474883));
#48842=CARTESIAN_POINT('Ctrl Pts',(-13.1940803008402,22.6458765499752,9.90789109044276));
#48843=CARTESIAN_POINT('Ctrl Pts',(-13.1894438989135,22.632035190591,9.91406213189617));
#48844=CARTESIAN_POINT('Ctrl Pts',(-13.1848526053688,22.6181327976104,9.92016440260441));
#48845=CARTESIAN_POINT('Ctrl Pts',(-13.1823499568869,22.6105548019219,9.92349066313972));
#48846=CARTESIAN_POINT('Ctrl Pts',(-13.179859834685,22.6029559187992,9.92679765089893));
#48847=CARTESIAN_POINT('Ctrl Pts',(-13.1773841523027,22.5953415704692,9.93008292268043));
#48848=CARTESIAN_POINT('Ctrl Pts',(-13.1753150145708,22.5889776137895,9.93282870293533));
#48849=CARTESIAN_POINT('Ctrl Pts',(-13.173255856113,22.5826025218678,9.93555945631742));
#48850=CARTESIAN_POINT('Ctrl Pts',(-13.1712079133685,22.5762198102661,9.93827359770395));
#48851=CARTESIAN_POINT('Ctrl Pts',(-13.1688678331854,22.5689266098223,9.94137490924681));
#48852=CARTESIAN_POINT('Ctrl Pts',(-13.1665425556495,22.5616240730917,9.94445432949206));
#48853=CARTESIAN_POINT('Ctrl Pts',(-13.1642322713302,22.5543125982023,9.947511695335));
#48854=CARTESIAN_POINT('Ctrl Pts',(-13.1599001203913,22.5406024186617,9.95324474308009));
#48855=CARTESIAN_POINT('Ctrl Pts',(-13.1556201306553,22.5268590117228,9.95890098193524));
#48856=CARTESIAN_POINT('Ctrl Pts',(-13.1513926252604,22.5130823508635,9.96448056704778));
#48857=CARTESIAN_POINT('Ctrl Pts',(-13.140516049515,22.4776375953031,9.97883578943898));
#48858=CARTESIAN_POINT('Ctrl Pts',(-13.1299870882692,22.4419725804668,9.99268335057632));
#48859=CARTESIAN_POINT('Ctrl Pts',(-13.119812808503,22.4060859326332,10.0060237791964));
#48860=CARTESIAN_POINT('Ctrl Pts',(-13.1141689397606,22.3861789186108,10.0134239716256));
#48861=CARTESIAN_POINT('Ctrl Pts',(-13.1086340371467,22.3662038533071,10.0206684376741));
#48862=CARTESIAN_POINT('Ctrl Pts',(-13.1032096331651,22.3461602255949,10.0277566190844));
#48863=CARTESIAN_POINT('Ctrl Pts',(-13.0773232529071,22.2505078791861,10.0615828901267));
#48864=CARTESIAN_POINT('Ctrl Pts',(-13.053948109445,22.1532971922261,10.0918570257584));
#48865=CARTESIAN_POINT('Ctrl Pts',(-13.0332474114134,22.0544759208489,10.1185207373871));
#48866=CARTESIAN_POINT('Ctrl Pts',(-13.0296331007545,22.0372218758926,10.1231761812276));
#48867=CARTESIAN_POINT('Ctrl Pts',(-13.0261002717855,22.0199187719173,10.1277216224077));
#48868=CARTESIAN_POINT('Ctrl Pts',(-13.022650085095,22.0025660932098,10.1321561991668));
#48869=CARTESIAN_POINT('Ctrl Pts',(-13.0020944629492,21.8991818016561,10.1585766489604));
#48870=CARTESIAN_POINT('Ctrl Pts',(-12.9844670907416,21.7940409596459,10.1810687787178));
#48871=CARTESIAN_POINT('Ctrl Pts',(-12.9700083867339,21.6870408589478,10.1994550074039));
#48872=CARTESIAN_POINT('Ctrl Pts',(-12.9681406962007,21.6732192138671,10.2018300325264));
#48873=CARTESIAN_POINT('Ctrl Pts',(-12.9663259866237,21.65936645822,10.2041363436325));
#48874=CARTESIAN_POINT('Ctrl Pts',(-12.9645648615698,21.6454823027918,10.206373398571));
#48875=CARTESIAN_POINT('Ctrl Pts',(-12.9643305992097,21.6436354521025,10.2066709684504));
#48876=CARTESIAN_POINT('Ctrl Pts',(-12.9640972861417,21.6417880600603,10.2069673114271));
#48877=CARTESIAN_POINT('Ctrl Pts',(-12.9638649230306,21.6399401205276,10.2072624271848));
#48878=CARTESIAN_POINT('Ctrl Pts',(-12.9618845878823,21.6241908925574,10.2097775773093));
#48879=CARTESIAN_POINT('Ctrl Pts',(-12.9599718992166,21.6083902294373,10.2122053056697));
#48880=CARTESIAN_POINT('Ctrl Pts',(-12.9581319554774,21.5925740951444,10.2145394523902));
#48881=CARTESIAN_POINT('Ctrl Pts',(-12.9566409127781,21.5797571100018,10.2164309843715));
#48882=CARTESIAN_POINT('Ctrl Pts',(-12.9551986494885,21.5669393234458,10.2182597889915));
#48883=CARTESIAN_POINT('Ctrl Pts',(-12.9538049100276,21.5541189441617,10.2200263443705));
#48884=CARTESIAN_POINT('Ctrl Pts',(-12.9517580067449,21.5352904061316,10.2226207804944));
#48885=CARTESIAN_POINT('Ctrl Pts',(-12.949815968165,21.5164579315467,10.2250806929422));
#48886=CARTESIAN_POINT('Ctrl Pts',(-12.9479786258968,21.4976215359301,10.2274067829201));
#48887=CARTESIAN_POINT('Ctrl Pts',(-12.946839985827,21.4859482210606,10.2288483103375));
#48888=CARTESIAN_POINT('Ctrl Pts',(-12.9457415466821,21.4742734009023,10.2302384667876));
#48889=CARTESIAN_POINT('Ctrl Pts',(-12.9446832872844,21.4625970774996,10.2315773638437));
#48890=CARTESIAN_POINT('Ctrl Pts',(-12.9400000881751,21.410924918974,10.2375024910041));
#48891=CARTESIAN_POINT('Ctrl Pts',(-12.9361036268393,21.359223297895,10.2424239343794));
#48892=CARTESIAN_POINT('Ctrl Pts',(-12.9329927241096,21.3074924518508,10.2463505307075));
#48893=CARTESIAN_POINT('Ctrl Pts',(-12.9324290289144,21.2981188288556,10.2470620294834));
#48894=CARTESIAN_POINT('Ctrl Pts',(-12.9318911062848,21.2887442482392,10.2477409236525));
#48895=CARTESIAN_POINT('Ctrl Pts',(-12.9313789674242,21.2793687105475,10.2483872117065));
#48896=CARTESIAN_POINT('Ctrl Pts',(-12.9249592111551,21.1618445945224,10.2564885531696));
#48897=CARTESIAN_POINT('Ctrl Pts',(-12.9225871454633,21.0441697906819,10.2594711806111));
#48898=CARTESIAN_POINT('Ctrl Pts',(-12.924282557788,20.9263441761685,10.2573349543856));
#48899=CARTESIAN_POINT('Ctrl Pts',(-12.9243505015238,20.9216223086244,10.2572493450101));
#48900=CARTESIAN_POINT('Ctrl Pts',(-12.9244249772314,20.9169001978544,10.2571555157621));
#48901=CARTESIAN_POINT('Ctrl Pts',(-12.9245059893016,20.9121778438395,10.2570534574116));
#48902=CARTESIAN_POINT('Ctrl Pts',(-12.9266085102063,20.7896177363176,10.2544047185896));
#48903=CARTESIAN_POINT('Ctrl Pts',(-12.9331112218386,20.6668943505176,10.246216252939));
#48904=CARTESIAN_POINT('Ctrl Pts',(-12.9440892692056,20.5440037453176,10.2323288156136));
#48905=CARTESIAN_POINT('Origin',(6.61363325216158E-15,20.5440037453176,
8.67361737988404E-16));
#48906=CARTESIAN_POINT('',(-10.3714285714286,51.,-12.8329057265981));
#48907=CARTESIAN_POINT('Origin',(6.61363325216158E-15,51.,8.67361737988404E-16));
#48908=CARTESIAN_POINT('',(-10.3714285714286,38.7323075626015,-12.8329057265981));
#48909=CARTESIAN_POINT('',(-10.3714285714286,52.,-12.8329057265981));
#48910=CARTESIAN_POINT('',(-6.12857142857143,38.7323075626015,-15.3196152773136));
#48911=CARTESIAN_POINT('Origin',(6.61363325216158E-15,38.7323075626015,
8.67361737988404E-16));
#48912=CARTESIAN_POINT('',(-4.71428571428571,40.2323075626015,-15.8121949837485));
#48913=CARTESIAN_POINT('Ctrl Pts',(-6.1285714285714,38.7323075626015,-15.3196152773135));
#48914=CARTESIAN_POINT('Ctrl Pts',(-6.08389803240923,38.732307564115,-15.3374867508708));
#48915=CARTESIAN_POINT('Ctrl Pts',(-6.03943307100923,38.7345475002831,-15.3550481877686));
#48916=CARTESIAN_POINT('Ctrl Pts',(-5.99517535721625,38.7389948597807,-15.3723086241536));
#48917=CARTESIAN_POINT('Ctrl Pts',(-5.95085559139461,38.743448454749,-15.3895932607289));
#48918=CARTESIAN_POINT('Ctrl Pts',(-5.90674351021535,38.7501152623945,-15.4065760832571));
#48919=CARTESIAN_POINT('Ctrl Pts',(-5.86284535065981,38.7590216606717,-15.4232630916498));
#48920=CARTESIAN_POINT('Ctrl Pts',(-5.84087298176195,38.7634795848872,-15.4316154487399));
#48921=CARTESIAN_POINT('Ctrl Pts',(-5.8189543016697,38.7684994073214,-15.4398936577168));
#48922=CARTESIAN_POINT('Ctrl Pts',(-5.79709081670919,38.7740900839308,-15.4480982021357));
#48923=CARTESIAN_POINT('Ctrl Pts',(-5.79402296690483,38.7748745588749,-15.4492494508975));
#48924=CARTESIAN_POINT('Ctrl Pts',(-5.79095620446294,38.7756702787681,-15.4503992490416));
#48925=CARTESIAN_POINT('Ctrl Pts',(-5.78789053458143,38.7764772771096,-15.4515475975481));
#48926=CARTESIAN_POINT('Ctrl Pts',(-5.78002619336392,38.7785474642351,-15.4544934478322));
#48927=CARTESIAN_POINT('Ctrl Pts',(-5.77216887004003,38.780691882803,-15.4574298223162));
#48928=CARTESIAN_POINT('Ctrl Pts',(-5.76431958430387,38.7829108473491,-15.4603563907826));
#48929=CARTESIAN_POINT('Ctrl Pts',(-5.76097517290875,38.7838563002938,-15.4616033384994));
#48930=CARTESIAN_POINT('Ctrl Pts',(-5.75763116042156,38.7848156307194,-15.4628488974097));
#48931=CARTESIAN_POINT('Ctrl Pts',(-5.75428915114725,38.7857883786975,-15.4640924786037));
#48932=CARTESIAN_POINT('Ctrl Pts',(-5.74672518435317,38.7879899983825,-15.4669070748795));
#48933=CARTESIAN_POINT('Ctrl Pts',(-5.73916807189642,38.7902613571697,-15.4697128057579));
#48934=CARTESIAN_POINT('Ctrl Pts',(-5.73163991938189,38.7925961353347,-15.4725015377136));
#48935=CARTESIAN_POINT('Ctrl Pts',(-5.72803537708487,38.7937140466196,-15.4738368058646));
#48936=CARTESIAN_POINT('Ctrl Pts',(-5.72443685547801,38.7948465963981,-15.4751684118958));
#48937=CARTESIAN_POINT('Ctrl Pts',(-5.72084482266767,38.7959936038935,-15.4764961982283));
#48938=CARTESIAN_POINT('Ctrl Pts',(-5.68106174251764,38.8086971323785,-15.4912019186035));
#48939=CARTESIAN_POINT('Ctrl Pts',(-5.64200959372428,38.8231914289868,-15.5054631835893));
#48940=CARTESIAN_POINT('Ctrl Pts',(-5.60367895309638,38.8394402713874,-15.5193035343287));
#48941=CARTESIAN_POINT('Ctrl Pts',(-5.59925348853597,38.8413162816762,-15.5209014721846));
#48942=CARTESIAN_POINT('Ctrl Pts',(-5.59483764214321,38.8432156804498,-15.5224937978581));
#48943=CARTESIAN_POINT('Ctrl Pts',(-5.59043142565676,38.8451384787602,-15.5240805366705));
#48944=CARTESIAN_POINT('Ctrl Pts',(-5.55305205649131,38.8614502029107,-15.5375413586752));
#48945=CARTESIAN_POINT('Ctrl Pts',(-5.51636486426997,38.87944394213,-15.5506004482821));
#48946=CARTESIAN_POINT('Ctrl Pts',(-5.48037827656239,38.8991259320294,-15.5632725975544));
#48947=CARTESIAN_POINT('Ctrl Pts',(-5.47538091537747,38.9018591173251,-15.5650323450308));
#48948=CARTESIAN_POINT('Ctrl Pts',(-5.47039706155543,38.9046248491444,-15.5667846303121));
#48949=CARTESIAN_POINT('Ctrl Pts',(-5.46542678317876,38.9074232578379,-15.5685294762621));
#48950=CARTESIAN_POINT('Ctrl Pts',(-5.43021578892617,38.927248053344,-15.580890506382));
#48951=CARTESIAN_POINT('Ctrl Pts',(-5.39568522742716,38.9487106524382,-15.592878507899));
#48952=CARTESIAN_POINT('Ctrl Pts',(-5.36185996218247,38.9718552620562,-15.6045012014465));
#48953=CARTESIAN_POINT('Ctrl Pts',(-5.35652757041948,38.9755038993926,-15.606333463659));
#48954=CARTESIAN_POINT('Ctrl Pts',(-5.35121274451998,38.9791944311442,-15.6081566340073));
#48955=CARTESIAN_POINT('Ctrl Pts',(-5.34591562608015,38.9829271390391,-15.6099707276299));
#48956=CARTESIAN_POINT('Ctrl Pts',(-5.34160108750772,38.985967454708,-15.6114483190785));
#48957=CARTESIAN_POINT('Ctrl Pts',(-5.33729719551838,38.9890365160764,-15.612920265461));
#48958=CARTESIAN_POINT('Ctrl Pts',(-5.33300532281936,38.9921335685879,-15.6143861303216));
#48959=CARTESIAN_POINT('Ctrl Pts',(-5.32762362465907,38.9960170485912,-15.6162242189084));
#48960=CARTESIAN_POINT('Ctrl Pts',(-5.32226600824693,38.9999409310175,-15.6180509684498));
#48961=CARTESIAN_POINT('Ctrl Pts',(-5.31694034680845,39.0038991173282,-15.6198638033924));
#48962=CARTESIAN_POINT('Ctrl Pts',(-5.31279156023976,39.0069826160432,-15.6212760345955));
#48963=CARTESIAN_POINT('Ctrl Pts',(-5.30866045530928,39.0100882064183,-15.6226804043607));
#48964=CARTESIAN_POINT('Ctrl Pts',(-5.30454965428839,39.0132138538924,-15.6240760675692));
#48965=CARTESIAN_POINT('Ctrl Pts',(-5.29917525738694,39.017300276469,-15.6259007357993));
#48966=CARTESIAN_POINT('Ctrl Pts',(-5.29383249930033,39.0214231565641,-15.6277115711503));
#48967=CARTESIAN_POINT('Ctrl Pts',(-5.28852147331464,39.0255821615688,-15.6295086519552));
#48968=CARTESIAN_POINT('Ctrl Pts',(-5.27523819943273,39.0359841446702,-15.634003285682));
#48969=CARTESIAN_POINT('Ctrl Pts',(-5.26215435627483,39.0466112362339,-15.6384115654574));
#48970=CARTESIAN_POINT('Ctrl Pts',(-5.24926792632382,39.0574606587315,-15.6427358936241));
#48971=CARTESIAN_POINT('Ctrl Pts',(-5.24396771194819,39.0619230478733,-15.6445144984356));
#48972=CARTESIAN_POINT('Ctrl Pts',(-5.23870084062666,39.0664229819347,-15.6462789219801));
#48973=CARTESIAN_POINT('Ctrl Pts',(-5.23346726793452,39.0709603894454,-15.6480292907943));
#48974=CARTESIAN_POINT('Ctrl Pts',(-5.20292155523454,39.0974429386287,-15.6582453069006));
#48975=CARTESIAN_POINT('Ctrl Pts',(-5.17350952617169,39.1252011529477,-15.6679828099636));
#48976=CARTESIAN_POINT('Ctrl Pts',(-5.14522556958604,39.1542216236436,-15.677265508949));
#48977=CARTESIAN_POINT('Ctrl Pts',(-5.14025296855357,39.159323711186,-15.6788974998064));
#48978=CARTESIAN_POINT('Ctrl Pts',(-5.13531522996645,39.164464805851,-15.6805154313045));
#48979=CARTESIAN_POINT('Ctrl Pts',(-5.13041246516379,39.1696450090146,-15.6821193766617));
#48980=CARTESIAN_POINT('Ctrl Pts',(-5.10245967567077,39.1991795949864,-15.6912641651092));
#48981=CARTESIAN_POINT('Ctrl Pts',(-5.0756420302649,39.2299833688396,-15.6999549216315));
#48982=CARTESIAN_POINT('Ctrl Pts',(-5.04998073674471,39.262072774733,-15.7082046892224));
#48983=CARTESIAN_POINT('Ctrl Pts',(-5.04554053096291,39.2676252448558,-15.709632156849));
#48984=CARTESIAN_POINT('Ctrl Pts',(-5.04113500250986,39.2732162744901,-15.7110463994174));
#48985=CARTESIAN_POINT('Ctrl Pts',(-5.03676437235535,39.2788460836699,-15.7124474439407));
#48986=CARTESIAN_POINT('Ctrl Pts',(-5.02935691609034,39.2883876288946,-15.7148219701908));
#48987=CARTESIAN_POINT('Ctrl Pts',(-5.02204963581774,39.2980404584332,-15.717158607631));
#48988=CARTESIAN_POINT('Ctrl Pts',(-5.01484358250578,39.3078055673202,-15.7194574924501));
#48989=CARTESIAN_POINT('Ctrl Pts',(-5.01179639128175,39.3119348948194,-15.7204296114926));
#48990=CARTESIAN_POINT('Ctrl Pts',(-5.00876656817256,39.3160853177002,-15.7213952133697));
#48991=CARTESIAN_POINT('Ctrl Pts',(-5.00575492521623,39.3202559331036,-15.7223540740142));
#48992=CARTESIAN_POINT('Ctrl Pts',(-5.00164458005159,39.3259480649749,-15.7236627444879));
#48993=CARTESIAN_POINT('Ctrl Pts',(-4.99757075494386,39.3316744395192,-15.7249580073045));
#48994=CARTESIAN_POINT('Ctrl Pts',(-4.99354092680169,39.3374239844029,-15.726237596301));
#48995=CARTESIAN_POINT('Ctrl Pts',(-4.99052725240488,39.3417237350618,-15.7271945265871));
#48996=CARTESIAN_POINT('Ctrl Pts',(-4.98753678343045,39.3460384288584,-15.7281431360081));
#48997=CARTESIAN_POINT('Ctrl Pts',(-4.98457197773345,39.3503644677928,-15.7290826877728));
#48998=CARTESIAN_POINT('Ctrl Pts',(-4.97763382745679,39.360488135681,-15.7312813989203));
#48999=CARTESIAN_POINT('Ctrl Pts',(-4.97082708885116,39.3706864848032,-15.733433415924));
#49000=CARTESIAN_POINT('Ctrl Pts',(-4.96415136662745,39.3809575748776,-15.7355394317834));
#49001=CARTESIAN_POINT('Ctrl Pts',(-4.9604608960052,39.3866356356039,-15.7367036787965));
#49002=CARTESIAN_POINT('Ctrl Pts',(-4.95681037613533,39.3923358701638,-15.7378539039165));
#49003=CARTESIAN_POINT('Ctrl Pts',(-4.95319982488722,39.3980580037776,-15.7389901876635));
#49004=CARTESIAN_POINT('Ctrl Pts',(-4.93060481845661,39.4338673960053,-15.7461011069683));
#49005=CARTESIAN_POINT('Ctrl Pts',(-4.90956865712636,39.4705390286067,-15.7526681103024));
#49006=CARTESIAN_POINT('Ctrl Pts',(-4.890065673627,39.5080554757784,-15.7587200529617));
#49007=CARTESIAN_POINT('Ctrl Pts',(-4.8872429986393,39.5134852469241,-15.7595959531629));
#49008=CARTESIAN_POINT('Ctrl Pts',(-4.88445243845779,39.5189327124889,-15.7604610623351));
#49009=CARTESIAN_POINT('Ctrl Pts',(-4.88169403147935,39.5243978910723,-15.7613154212793));
#49010=CARTESIAN_POINT('Ctrl Pts',(-4.86223767862383,39.5629463880009,-15.7673416201742));
#49011=CARTESIAN_POINT('Ctrl Pts',(-4.84437854675939,39.6023747382796,-15.7728337732031));
#49012=CARTESIAN_POINT('Ctrl Pts',(-4.82812990008951,39.6426872307578,-15.777805983972));
#49013=CARTESIAN_POINT('Ctrl Pts',(-4.82615816357802,39.6475790605146,-15.7784093504994));
#49014=CARTESIAN_POINT('Ctrl Pts',(-4.82421018319831,39.6524839344262,-15.7790050442279));
#49015=CARTESIAN_POINT('Ctrl Pts',(-4.82228603965509,39.6574018950085,-15.7795930685527));
#49016=CARTESIAN_POINT('Ctrl Pts',(-4.81512379702973,39.6757080276441,-15.7817818724487));
#49017=CARTESIAN_POINT('Ctrl Pts',(-4.80829157794962,39.6941953038606,-15.7838644898425));
#49018=CARTESIAN_POINT('Ctrl Pts',(-4.80179347933714,39.7128657246913,-15.785841104667));
#49019=CARTESIAN_POINT('Ctrl Pts',(-4.8002256680114,39.7173703804345,-15.7863180071109));
#49020=CARTESIAN_POINT('Ctrl Pts',(-4.7986773156128,39.721885702968,-15.7867887354881));
#49021=CARTESIAN_POINT('Ctrl Pts',(-4.79714850220147,39.7264117342425,-15.7872532840548));
#49022=CARTESIAN_POINT('Ctrl Pts',(-4.79465045226035,39.7338071770577,-15.7880123469405));
#49023=CARTESIAN_POINT('Ctrl Pts',(-4.7922042856598,39.7412320052383,-15.7887549965822));
#49024=CARTESIAN_POINT('Ctrl Pts',(-4.78981048689747,39.7486860660883,-15.7894811662577));
#49025=CARTESIAN_POINT('Ctrl Pts',(-4.78843576777426,39.7529668102166,-15.789898193518));
#49026=CARTESIAN_POINT('Ctrl Pts',(-4.78707968180564,39.7572530601147,-15.7903093722902));
#49027=CARTESIAN_POINT('Ctrl Pts',(-4.78574260519565,39.7615433383508,-15.7907146044043));
#49028=CARTESIAN_POINT('Ctrl Pts',(-4.78332253508594,39.7693086182488,-15.7914480628461));
#49029=CARTESIAN_POINT('Ctrl Pts',(-4.78096487665038,39.777086869378,-15.7921619986678));
#49030=CARTESIAN_POINT('Ctrl Pts',(-4.77867094065993,39.7848722502327,-15.7928561077752));
#49031=CARTESIAN_POINT('Ctrl Pts',(-4.77749058521369,39.7888782542063,-15.7932132648488));
#49032=CARTESIAN_POINT('Ctrl Pts',(-4.77632672235366,39.7928871971688,-15.7935652914508));
#49033=CARTESIAN_POINT('Ctrl Pts',(-4.77517921318359,39.7968994113442,-15.7939122395095));
#49034=CARTESIAN_POINT('Ctrl Pts',(-4.76246087899298,39.8413684945181,-15.7977576130129));
#49035=CARTESIAN_POINT('Ctrl Pts',(-4.7517677361539,39.8861804968818,-15.8009742178634));
#49036=CARTESIAN_POINT('Ctrl Pts',(-4.74304960963775,39.9313262331944,-15.8035907438948));
#49037=CARTESIAN_POINT('Ctrl Pts',(-4.73352637830731,39.9806411048806,-15.8064489018526));
#49038=CARTESIAN_POINT('Ctrl Pts',(-4.7263581061177,40.0303539996461,-15.8085914687166));
#49039=CARTESIAN_POINT('Ctrl Pts',(-4.72155073199278,40.0804653705169,-15.810027156372));
#49040=CARTESIAN_POINT('Ctrl Pts',(-4.71673391401152,40.130675182777,-15.811465664367));
#49041=CARTESIAN_POINT('Ctrl Pts',(-4.71428571809898,40.1812848466719,-15.8121949826116));
#49042=CARTESIAN_POINT('Ctrl Pts',(-4.71428571428571,40.2323075626015,-15.8121949837485));
#49043=CARTESIAN_POINT('',(-4.71428571428571,52.,-15.8121949837485));
#49044=CARTESIAN_POINT('',(3.94534942910196E-9,28.7540327056294,-16.5000000412986));
#49045=CARTESIAN_POINT('',(0.731312635855993,28.7467958750258,-16.4837854216996));
#49046=CARTESIAN_POINT('Origin',(0.470077120411344,40.0190250852893,-14.4549067130411));
#49047=CARTESIAN_POINT('',(0.3210340492655,44.2777094964746,-16.496876587379));
#49048=CARTESIAN_POINT('Ctrl Pts',(0.731312635812438,28.7467958754239,-16.4837854217016));
#49049=CARTESIAN_POINT('Ctrl Pts',(0.734616685498146,28.7471690084713,-16.483638835634));
#49050=CARTESIAN_POINT('Ctrl Pts',(0.737920010933865,28.7475475691393,-16.4834912865799));
#49051=CARTESIAN_POINT('Ctrl Pts',(0.741222612912324,28.7479315514833,-16.483342775688));
#49052=CARTESIAN_POINT('Ctrl Pts',(0.845120434181737,28.760011399194,-16.4786707146258));
#49053=CARTESIAN_POINT('Ctrl Pts',(0.948323680373575,28.7774576338618,-16.4730453966297));
#49054=CARTESIAN_POINT('Ctrl Pts',(1.05079165216144,28.8001000249142,-16.466506517891));
#49055=CARTESIAN_POINT('Ctrl Pts',(1.05587756435429,28.801223861082,-16.4661819661065));
#49056=CARTESIAN_POINT('Ctrl Pts',(1.06096252503882,28.8023607191809,-16.4658551046886));
#49057=CARTESIAN_POINT('Ctrl Pts',(1.06604599104648,28.8035104462793,-16.4655259757118));
#49058=CARTESIAN_POINT('Ctrl Pts',(1.07948376023311,28.8065496654563,-16.4646559474247));
#49059=CARTESIAN_POINT('Ctrl Pts',(1.09291006996102,28.8096785418744,-16.4637701472321));
#49060=CARTESIAN_POINT('Ctrl Pts',(1.10632404935655,28.8128965822484,-16.4628687224595));
#49061=CARTESIAN_POINT('Ctrl Pts',(1.11422078750616,28.8147910254588,-16.4623380585021));
#49062=CARTESIAN_POINT('Ctrl Pts',(1.12211200562617,28.8167160726008,-16.4618020600035));
#49063=CARTESIAN_POINT('Ctrl Pts',(1.12999383075715,28.818670716019,-16.4612610070569));
#49064=CARTESIAN_POINT('Ctrl Pts',(1.13550065267297,28.8200363734694,-16.4608829877308));
#49065=CARTESIAN_POINT('Ctrl Pts',(1.1410004192206,28.8214158328344,-16.4605026765839));
#49066=CARTESIAN_POINT('Ctrl Pts',(1.14649254658236,28.8228088410152,-16.4601201352088));
#49067=CARTESIAN_POINT('Ctrl Pts',(1.16726650596732,28.8280778913238,-16.4586731733185));
#49068=CARTESIAN_POINT('Ctrl Pts',(1.18794518936591,28.833544327345,-16.4571933294199));
#49069=CARTESIAN_POINT('Ctrl Pts',(1.20853084392565,28.8392035794322,-16.4556814869297));
#49070=CARTESIAN_POINT('Ctrl Pts',(1.21440895604015,28.8408195454514,-16.455249789233));
#49071=CARTESIAN_POINT('Ctrl Pts',(1.22027948624603,28.8424512259965,-16.4548154834927));
#49072=CARTESIAN_POINT('Ctrl Pts',(1.22614248193765,28.8440985249416,-16.4543785888375));
#49073=CARTESIAN_POINT('Ctrl Pts',(1.27220783047617,28.8570412941407,-16.4509459230761));
#49074=CARTESIAN_POINT('Ctrl Pts',(1.3178082038286,28.8709478913296,-16.447353427901));
#49075=CARTESIAN_POINT('Ctrl Pts',(1.36296608480579,28.8857718606986,-16.4436104141296));
#49076=CARTESIAN_POINT('Ctrl Pts',(1.36955965797723,28.8879363317634,-16.4430638908064));
#49077=CARTESIAN_POINT('Ctrl Pts',(1.37614381062977,28.8901203327012,-16.4425141624419));
#49078=CARTESIAN_POINT('Ctrl Pts',(1.38271860044915,28.892323744337,-16.4419612544658));
#49079=CARTESIAN_POINT('Ctrl Pts',(1.47768180782263,28.9241487975866,-16.4339753087194));
#49080=CARTESIAN_POINT('Ctrl Pts',(1.57069371812965,28.9600199707892,-16.4253258894182));
#49081=CARTESIAN_POINT('Ctrl Pts',(1.6619297639424,28.9995770867733,-16.4160893473363));
#49082=CARTESIAN_POINT('Ctrl Pts',(1.66985101459179,29.0030114950478,-16.4152874168678));
#49083=CARTESIAN_POINT('Ctrl Pts',(1.6777588721055,29.0064737005077,-16.414481058856));
#49084=CARTESIAN_POINT('Ctrl Pts',(1.68565342634818,29.0099635189963,-16.4136703161511));
#49085=CARTESIAN_POINT('Ctrl Pts',(1.77500332989141,29.0494609922869,-16.4044943981371));
#49086=CARTESIAN_POINT('Ctrl Pts',(1.86265046663758,29.0924930099575,-16.3947566911446));
#49087=CARTESIAN_POINT('Ctrl Pts',(1.94872552747264,29.1387927117366,-16.3845191817942));
#49088=CARTESIAN_POINT('Ctrl Pts',(1.9578515268182,29.1437015789977,-16.383433762827));
#49089=CARTESIAN_POINT('Ctrl Pts',(1.96695984784121,29.1486471906051,-16.3823427237235));
#49090=CARTESIAN_POINT('Ctrl Pts',(1.9760506137378,29.1536292958558,-16.3812461293587));
#49091=CARTESIAN_POINT('Ctrl Pts',(2.06029660563837,29.1997994869451,-16.3710837644901));
#49092=CARTESIAN_POINT('Ctrl Pts',(2.1430359410388,29.2491015209459,-16.3604441914389));
#49093=CARTESIAN_POINT('Ctrl Pts',(2.22436702801141,29.301335893347,-16.3493789277972));
#49094=CARTESIAN_POINT('Ctrl Pts',(2.23458821889496,29.3079003880669,-16.347988313506));
#49095=CARTESIAN_POINT('Ctrl Pts',(2.24478716184637,29.3145112072703,-16.3465909740617));
#49096=CARTESIAN_POINT('Ctrl Pts',(2.25496401208747,29.3211680380968,-16.3451870012336));
#49097=CARTESIAN_POINT('Ctrl Pts',(2.27775279060625,29.336074520923,-16.3420431182963));
#49098=CARTESIAN_POINT('Ctrl Pts',(2.30043071534413,29.3512118385305,-16.338865983534));
#49099=CARTESIAN_POINT('Ctrl Pts',(2.32299970540114,29.3665761205162,-16.3356566023839));
#49100=CARTESIAN_POINT('Ctrl Pts',(2.34556869545816,29.3819404025018,-16.3324472212339));
#49101=CARTESIAN_POINT('Ctrl Pts',(2.36804092323506,29.3975404318301,-16.329203784601));
#49102=CARTESIAN_POINT('Ctrl Pts',(2.39036258748978,29.4133328398107,-16.3259355337187));
#49103=CARTESIAN_POINT('Ctrl Pts',(2.41268425174452,29.4291252477914,-16.3226672828364));
#49104=CARTESIAN_POINT('Ctrl Pts',(2.43486066092521,29.4451132785474,-16.3193735215193));
#49105=CARTESIAN_POINT('Ctrl Pts',(2.45689550418518,29.4612920769389,-16.3160554493108));
#49106=CARTESIAN_POINT('Ctrl Pts',(2.4678508029967,29.4693358632594,-16.3144057678453));
#49107=CARTESIAN_POINT('Ctrl Pts',(2.47877011604896,29.477426086673,-16.3127502284335));
#49108=CARTESIAN_POINT('Ctrl Pts',(2.4896578027103,29.4855650408066,-16.311088376482));
#49109=CARTESIAN_POINT('Ctrl Pts',(2.50066896820931,29.4937963000026,-16.3094076772258));
#49110=CARTESIAN_POINT('Ctrl Pts',(2.51163612628462,29.5020688330178,-16.3077222797715));
#49111=CARTESIAN_POINT('Ctrl Pts',(2.52256015072484,29.5103819452868,-16.3060323219646));
#49112=CARTESIAN_POINT('Ctrl Pts',(2.53317374658008,29.5184588234012,-16.3043903877787));
#49113=CARTESIAN_POINT('Ctrl Pts',(2.54374758129008,29.5265747525576,-16.3027439980989));
#49114=CARTESIAN_POINT('Ctrl Pts',(2.55427857869813,29.5347263140629,-16.3010938572356));
#49115=CARTESIAN_POINT('Ctrl Pts',(2.57566004008263,29.5512767214742,-16.2977435171128));
#49116=CARTESIAN_POINT('Ctrl Pts',(2.59687480044613,29.5679813972322,-16.2943762062056));
#49117=CARTESIAN_POINT('Ctrl Pts',(2.61792789046617,29.5848353002105,-16.2909930194669));
#49118=CARTESIAN_POINT('Ctrl Pts',(2.66006203009866,29.6185654890218,-16.2842221529425));
#49119=CARTESIAN_POINT('Ctrl Pts',(2.70154891715646,29.6528931031441,-16.2773877442513));
#49120=CARTESIAN_POINT('Ctrl Pts',(2.74242506837524,29.687781395081,-16.2704979869811));
#49121=CARTESIAN_POINT('Ctrl Pts',(2.75343149573759,29.6971755146239,-16.2686428315744));
#49122=CARTESIAN_POINT('Ctrl Pts',(2.76439370647325,29.7066102235636,-16.2667836725572));
#49123=CARTESIAN_POINT('Ctrl Pts',(2.77531229191419,29.7160849216131,-16.2649206515303));
#49124=CARTESIAN_POINT('Ctrl Pts',(2.8456018154237,29.7770792706431,-16.2529272609048));
#49125=CARTESIAN_POINT('Ctrl Pts',(2.91408883144597,29.8397324669013,-16.2407729461803));
#49126=CARTESIAN_POINT('Ctrl Pts',(2.98093811843778,29.9038965360028,-16.2284937050254));
#49127=CARTESIAN_POINT('Ctrl Pts',(2.99179906065064,29.9143212133332,-16.2264987080015));
#49128=CARTESIAN_POINT('Ctrl Pts',(3.00261674765443,29.9247857948943,-16.2245004096329));
#49129=CARTESIAN_POINT('Ctrl Pts',(3.01339173931629,29.9352897861473,-16.22249894315));
#49130=CARTESIAN_POINT('Ctrl Pts',(3.07936347969847,29.9996022798977,-16.2102446202386));
#49131=CARTESIAN_POINT('Ctrl Pts',(3.14373670241214,30.0653901737341,-16.1978712029431));
#49132=CARTESIAN_POINT('Ctrl Pts',(3.20663867175698,30.1325397322854,-16.1854091214524));
#49133=CARTESIAN_POINT('Ctrl Pts',(3.21724458806279,30.1438618356374,-16.1833078868701));
#49134=CARTESIAN_POINT('Ctrl Pts',(3.22780865912799,30.1552226669215,-16.1812041287764));
#49135=CARTESIAN_POINT('Ctrl Pts',(3.23833137423545,30.1666217964529,-16.179097976329));
#49136=CARTESIAN_POINT('Ctrl Pts',(3.30051780922609,30.2339876065426,-16.1666511780536));
#49137=CARTESIAN_POINT('Ctrl Pts',(3.36126109250365,30.3026896174408,-16.1541205481176));
#49138=CARTESIAN_POINT('Ctrl Pts',(3.42066110077687,30.3726394183252,-16.1415326915899));
#49139=CARTESIAN_POINT('Ctrl Pts',(3.43092444856263,30.3847255973492,-16.1393577163133));
#49140=CARTESIAN_POINT('Ctrl Pts',(3.44114781103686,30.3968489132885,-16.1371810457367));
#49141=CARTESIAN_POINT('Ctrl Pts',(3.45133156533654,30.4090090427529,-16.1350027997543));
#49142=CARTESIAN_POINT('Ctrl Pts',(3.52045467376127,30.491546967637,-16.1202177677526));
#49143=CARTESIAN_POINT('Ctrl Pts',(3.58775143477868,30.5757822736924,-16.105360573047));
#49144=CARTESIAN_POINT('Ctrl Pts',(3.65334819678238,30.6616030099696,-16.0904663944269));
#49145=CARTESIAN_POINT('Ctrl Pts',(3.70914483972207,30.7346021768891,-16.0777973976509));
#49146=CARTESIAN_POINT('Ctrl Pts',(3.76371063983931,30.8087513309492,-16.0651017701954));
#49147=CARTESIAN_POINT('Ctrl Pts',(3.81710946620164,30.8839857712926,-16.0524040356279));
#49148=CARTESIAN_POINT('Ctrl Pts',(3.82648843290392,30.8971999439423,-16.0501738062799));
#49149=CARTESIAN_POINT('Ctrl Pts',(3.83583337260282,30.9104510140065,-16.0479429610118));
#49150=CARTESIAN_POINT('Ctrl Pts',(3.84514079754373,30.9237330962212,-16.0457125481931));
#49151=CARTESIAN_POINT('Ctrl Pts',(3.86071553022625,30.9459588870576,-16.0419802502007));
#49152=CARTESIAN_POINT('Ctrl Pts',(3.87619388529158,30.9682835953682,-16.0382470688338));
#49153=CARTESIAN_POINT('Ctrl Pts',(3.89154316500324,30.9906557222109,-16.0345218565835));
#49154=CARTESIAN_POINT('Ctrl Pts',(3.89773456957979,30.9996799169043,-16.0330192260622));
#49155=CARTESIAN_POINT('Ctrl Pts',(3.90390673158024,31.0087143633717,-16.0315174679896));
#49156=CARTESIAN_POINT('Ctrl Pts',(3.91005845705946,31.0177570719153,-16.0300169326915));
#49157=CARTESIAN_POINT('Ctrl Pts',(3.91915764176106,31.0311323884047,-16.0277974500644));
#49158=CARTESIAN_POINT('Ctrl Pts',(3.92821432019911,31.044528753913,-16.0255801318543));
#49159=CARTESIAN_POINT('Ctrl Pts',(3.93722860915545,31.0579453074097,-16.0233651619476));
#49160=CARTESIAN_POINT('Ctrl Pts',(3.95846129759498,31.0895473008347,-16.0181479156225));
#49161=CARTESIAN_POINT('Ctrl Pts',(3.97945901013079,31.1212615902012,-16.012943649059));
#49162=CARTESIAN_POINT('Ctrl Pts',(4.00022876823323,31.1530850595607,-16.0077534276925));
#49163=CARTESIAN_POINT('Ctrl Pts',(4.00901742940061,31.166551065664,-16.005557201008));
#49164=CARTESIAN_POINT('Ctrl Pts',(4.01776531294456,31.1800366018781,-16.0033634911397));
#49165=CARTESIAN_POINT('Ctrl Pts',(4.02647287172629,31.1935414708459,-16.0011723745607));
#49166=CARTESIAN_POINT('Ctrl Pts',(4.07643282159421,31.2710261704631,-15.9886007598075));
#49167=CARTESIAN_POINT('Ctrl Pts',(4.12506630677904,31.3491467663653,-15.9761142740004));
#49168=CARTESIAN_POINT('Ctrl Pts',(4.1724572629542,31.4278654560049,-15.963727647039));
#49169=CARTESIAN_POINT('Ctrl Pts',(4.18062581228057,31.4414338148464,-15.96159262421));
#49170=CARTESIAN_POINT('Ctrl Pts',(4.18875754981286,31.4550198912338,-15.9594605716859));
#49171=CARTESIAN_POINT('Ctrl Pts',(4.19685278850281,31.4686235486063,-15.9573315597597));
#49172=CARTESIAN_POINT('Ctrl Pts',(4.2519136616836,31.5611506848738,-15.9428507939464));
#49173=CARTESIAN_POINT('Ctrl Pts',(4.30528494322195,31.6544921398643,-15.9285110242643));
#49174=CARTESIAN_POINT('Ctrl Pts',(4.3570738298972,31.7486000042021,-15.9143317969289));
#49175=CARTESIAN_POINT('Ctrl Pts',(4.40154566221242,31.8294117271614,-15.9021558985673));
#49176=CARTESIAN_POINT('Ctrl Pts',(4.44484660746696,31.9107908818802,-15.890099467165));
#49177=CARTESIAN_POINT('Ctrl Pts',(4.48703986256301,31.9927091048758,-15.8781760058382));
#49178=CARTESIAN_POINT('Ctrl Pts',(4.54311742712378,32.101583720695,-15.8623289546729));
#49179=CARTESIAN_POINT('Ctrl Pts',(4.59723619017192,32.2114115949789,-15.8467165556072));
#49180=CARTESIAN_POINT('Ctrl Pts',(4.64949281461725,32.3221519839062,-15.8313691559524));
#49181=CARTESIAN_POINT('Ctrl Pts',(4.68921103260749,32.4063214256646,-15.8197041972693));
#49182=CARTESIAN_POINT('Ctrl Pts',(4.72785240054499,32.4910185880583,-15.8081926424038));
#49183=CARTESIAN_POINT('Ctrl Pts',(4.76545874007257,32.5762252746749,-15.7968478816819));
#49184=CARTESIAN_POINT('Ctrl Pts',(4.8145581895929,32.6874725127972,-15.7820359772696));
#49185=CARTESIAN_POINT('Ctrl Pts',(4.86189217437588,32.7995888343388,-15.767508226408));
#49186=CARTESIAN_POINT('Ctrl Pts',(4.90751726593677,32.9125521688301,-15.7532948069065));
#49187=CARTESIAN_POINT('Ctrl Pts',(4.94292643975522,33.000221874452,-15.7422639152531));
#49188=CARTESIAN_POINT('Ctrl Pts',(4.97730545013789,33.0884022086102,-15.7314226152448));
#49189=CARTESIAN_POINT('Ctrl Pts',(5.01068036844344,33.1770825485621,-15.7207850390979));
#49190=CARTESIAN_POINT('Ctrl Pts',(5.05324703184162,33.2901862315797,-15.7072177812226));
#49191=CARTESIAN_POINT('Ctrl Pts',(5.09417985157194,33.4041034930525,-15.6939817639376));
#49192=CARTESIAN_POINT('Ctrl Pts',(5.1335045001183,33.5188268327618,-15.6811080106665));
#49193=CARTESIAN_POINT('Ctrl Pts',(5.16483497343243,33.6102284514955,-15.6708513192981));
#49194=CARTESIAN_POINT('Ctrl Pts',(5.19514785591287,33.7021488152071,-15.66082350329));
#49195=CARTESIAN_POINT('Ctrl Pts',(5.2244462630085,33.7945633654866,-15.6510434554676));
#49196=CARTESIAN_POINT('Ctrl Pts',(5.22795148832419,33.8056197283844,-15.6498733825997));
#49197=CARTESIAN_POINT('Ctrl Pts',(5.23144245196559,33.8166841411844,-15.6487067609901));
#49198=CARTESIAN_POINT('Ctrl Pts',(5.2349189486445,33.8277559098327,-15.6475436910747));
#49199=CARTESIAN_POINT('Ctrl Pts',(5.2446746186188,33.8588252681381,-15.6442799093716));
#49200=CARTESIAN_POINT('Ctrl Pts',(5.25431701128392,33.8899539217391,-15.6410438820536));
#49201=CARTESIAN_POINT('Ctrl Pts',(5.2638444202153,33.9211357782144,-15.6378368672982));
#49202=CARTESIAN_POINT('Ctrl Pts',(5.26693462334182,33.9312495742175,-15.6367966760883));
#49203=CARTESIAN_POINT('Ctrl Pts',(5.27001255653563,33.9413684091124,-15.6357595952178));
#49204=CARTESIAN_POINT('Ctrl Pts',(5.27307794881816,33.9514913720823,-15.6347257393818));
#49205=CARTESIAN_POINT('Ctrl Pts',(5.27632085614409,33.9622005498154,-15.6336320135694));
#49206=CARTESIAN_POINT('Ctrl Pts',(5.27954900617633,33.9729119185877,-15.6325421418139));
#49207=CARTESIAN_POINT('Ctrl Pts',(5.28276229076912,33.9836249799428,-15.631456189949));
#49208=CARTESIAN_POINT('Ctrl Pts',(5.2952909009369,34.0253952513105,-15.6272220590513));
#49209=CARTESIAN_POINT('Ctrl Pts',(5.30759740664544,34.0672041752914,-15.6230462074124));
#49210=CARTESIAN_POINT('Ctrl Pts',(5.31968392036379,34.1090516118263,-15.6189296364195));
#49211=CARTESIAN_POINT('Ctrl Pts',(5.32266165147491,34.1193614841844,-15.6179154447508));
#49212=CARTESIAN_POINT('Ctrl Pts',(5.3256260357014,34.1296736930948,-15.6169048508008));
#49213=CARTESIAN_POINT('Ctrl Pts',(5.32857709711616,34.1399882377568,-15.6158978700675));
#49214=CARTESIAN_POINT('Ctrl Pts',(5.35573331102589,34.2349045888094,-15.6066314467867));
#49215=CARTESIAN_POINT('Ctrl Pts',(5.38176097528874,34.330018513957,-15.5976711212928));
#49216=CARTESIAN_POINT('Ctrl Pts',(5.40667913038459,34.4253275758219,-15.5890288594613));
#49217=CARTESIAN_POINT('Ctrl Pts',(5.43655671445108,34.5396058800228,-15.5786665391611));
#49218=CARTESIAN_POINT('Ctrl Pts',(5.4648418408843,34.6541642591764,-15.5687612237176));
#49219=CARTESIAN_POINT('Ctrl Pts',(5.49154896429295,34.7690018144804,-15.5593350786686));
#49220=CARTESIAN_POINT('Ctrl Pts',(5.51425047771342,34.8666157080854,-15.5513226935436));
#49221=CARTESIAN_POINT('Ctrl Pts',(5.53581096326103,34.9644314725277,-15.5436568302854));
#49222=CARTESIAN_POINT('Ctrl Pts',(5.55623902970539,35.0624484180682,-15.5363511753867));
#49223=CARTESIAN_POINT('Ctrl Pts',(5.57988683156696,35.1759141400214,-15.527894051949));
#49224=CARTESIAN_POINT('Ctrl Pts',(5.60201700179433,35.2896494727898,-15.5199195687207));
#49225=CARTESIAN_POINT('Ctrl Pts',(5.62262129551896,35.403657194424,-15.5124513197386));
#49226=CARTESIAN_POINT('Ctrl Pts',(5.64077602836221,35.5041110006062,-15.5058709405764));
#49227=CARTESIAN_POINT('Ctrl Pts',(5.65774561136324,35.6047763774753,-15.4996837693532));
#49228=CARTESIAN_POINT('Ctrl Pts',(5.67352437393353,35.7056550526876,-15.4939059368047));
#49229=CARTESIAN_POINT('Ctrl Pts',(5.69112288890293,35.8181679869503,-15.4874617513281));
#49230=CARTESIAN_POINT('Ctrl Pts',(5.70724024386807,35.9309462212848,-15.4815266881963));
#49231=CARTESIAN_POINT('Ctrl Pts',(5.72184788894286,36.0439958608173,-15.476125906358));
#49232=CARTESIAN_POINT('Ctrl Pts',(5.73521687343338,36.1474594149925,-15.4711830857827));
#49233=CARTESIAN_POINT('Ctrl Pts',(5.74732086117479,36.2511503898043,-15.4666879504269));
#49234=CARTESIAN_POINT('Ctrl Pts',(5.75813800618103,36.3550732611076,-15.4626597551001));
#49235=CARTESIAN_POINT('Ctrl Pts',(5.76973743980501,36.4665117642431,-15.4583402434091));
#49236=CARTESIAN_POINT('Ctrl Pts',(5.77985764006083,36.5782168324163,-15.4545575498512));
#49237=CARTESIAN_POINT('Ctrl Pts',(5.78844979037594,36.6901979213228,-15.4513387051517));
#49238=CARTESIAN_POINT('Ctrl Pts',(5.79663487698932,36.7968737682468,-15.4482723571836));
#49239=CARTESIAN_POINT('Ctrl Pts',(5.80343362974005,36.9038002277388,-15.4457175623473));
#49240=CARTESIAN_POINT('Ctrl Pts',(5.8088031368251,37.0109851036483,-15.4436979418038));
#49241=CARTESIAN_POINT('Ctrl Pts',(5.81430863978894,37.1208846982762,-15.4416271694383));
#49242=CARTESIAN_POINT('Ctrl Pts',(5.81830887505587,37.2310564494967,-15.4401194484732));
#49243=CARTESIAN_POINT('Ctrl Pts',(5.82073968029914,37.3415118986157,-15.4392030096826));
#49244=CARTESIAN_POINT('Ctrl Pts',(5.82074760164734,37.3418718435659,-15.4392000232522));
#49245=CARTESIAN_POINT('Ctrl Pts',(5.82075550629764,37.3422317922858,-15.4391970431108));
#49246=CARTESIAN_POINT('Ctrl Pts',(5.82076339424765,37.3425917447223,-15.4391940692593));
#49247=CARTESIAN_POINT('Ctrl Pts',(5.8213620453315,37.3699101121222,-15.4389683706475));
#49248=CARTESIAN_POINT('Ctrl Pts',(5.82186461765603,37.3972541851766,-15.4387788590838));
#49249=CARTESIAN_POINT('Ctrl Pts',(5.82226993685469,37.4245958984253,-15.4386260036546));
#49250=CARTESIAN_POINT('Ctrl Pts',(5.82267525605335,37.4519376116741,-15.4384731482255));
#49251=CARTESIAN_POINT('Ctrl Pts',(5.82298322987151,37.4792662650347,-15.4383569837344));
#49252=CARTESIAN_POINT('Ctrl Pts',(5.82319306158449,37.5065817823569,-15.4382778368426));
#49253=CARTESIAN_POINT('Ctrl Pts',(5.82319492313034,37.5068241150683,-15.4382771346819));
#49254=CARTESIAN_POINT('Ctrl Pts',(5.82319677694153,37.5070664459699,-15.4382764354387));
#49255=CARTESIAN_POINT('Ctrl Pts',(5.82319862301729,37.5073087750453,-15.4382757391131));
#49256=CARTESIAN_POINT('Ctrl Pts',(5.82361295281936,37.5616966609361,-15.4381194571051));
#49257=CARTESIAN_POINT('Ctrl Pts',(5.82363882494282,37.6160331651307,-15.4381096966784));
#49258=CARTESIAN_POINT('Ctrl Pts',(5.82327195590684,37.6703166990449,-15.4382480783256));
#49259=CARTESIAN_POINT('Ctrl Pts',(5.82326629494549,37.6711543194408,-15.4382502136194));
#49260=CARTESIAN_POINT('Ctrl Pts',(5.8232605403331,37.6719919272872,-15.4382523842383));
#49261=CARTESIAN_POINT('Ctrl Pts',(5.8232546920561,37.6728295225823,-15.4382545901876));
#49262=CARTESIAN_POINT('Ctrl Pts',(5.82249914619176,37.781039455463,-15.4385395793989));
#49263=CARTESIAN_POINT('Ctrl Pts',(5.82018359012415,37.8890402606468,-15.4394141505793));
#49264=CARTESIAN_POINT('Ctrl Pts',(5.8162661747651,37.9968265190168,-15.4408897890572));
#49265=CARTESIAN_POINT('Ctrl Pts',(5.81220429168145,38.1085877542688,-15.4424198466134));
#49266=CARTESIAN_POINT('Ctrl Pts',(5.8064178675135,38.220117964245,-15.4445970100905));
#49267=CARTESIAN_POINT('Ctrl Pts',(5.79885506465812,38.3314104977014,-15.4474360312433));
#49268=CARTESIAN_POINT('Ctrl Pts',(5.79171731437334,38.4364480515768,-15.4501154907544));
#49269=CARTESIAN_POINT('Ctrl Pts',(5.78299784892559,38.541273967809,-15.4533845335069));
#49270=CARTESIAN_POINT('Ctrl Pts',(5.77263170026572,38.6458799562132,-15.4572559204152));
#49271=CARTESIAN_POINT('Ctrl Pts',(5.76143267394023,38.7588906081323,-15.4614383574343));
#49272=CARTESIAN_POINT('Ctrl Pts',(5.74831194401947,38.8716445920318,-15.4663237377932));
#49273=CARTESIAN_POINT('Ctrl Pts',(5.73318723260849,38.9841316418235,-15.4719282623814));
#49274=CARTESIAN_POINT('Ctrl Pts',(5.71947849532972,39.0860876640547,-15.4770080918779));
#49275=CARTESIAN_POINT('Ctrl Pts',(5.70412446117446,39.1878245192004,-15.4826787537311));
#49276=CARTESIAN_POINT('Ctrl Pts',(5.68703815784452,39.2893313225491,-15.4889524181855));
#49277=CARTESIAN_POINT('Ctrl Pts',(5.669069433215,39.3960804397909,-15.4955500857337));
#49278=CARTESIAN_POINT('Ctrl Pts',(5.64918879223543,39.5025757189157,-15.5028132260879));
#49279=CARTESIAN_POINT('Ctrl Pts',(5.62728826714314,39.6088036853509,-15.5107584481952));
#49280=CARTESIAN_POINT('Ctrl Pts',(5.62579498641333,39.6160468073572,-15.5113001907798));
#49281=CARTESIAN_POINT('Ctrl Pts',(5.62429232542101,39.6232886887372,-15.5118451005988));
#49282=CARTESIAN_POINT('Ctrl Pts',(5.62278025233869,39.6305293255435,-15.5123931820307));
#49283=CARTESIAN_POINT('Ctrl Pts',(5.60211619080702,39.7294802071136,-15.5198832885376));
#49284=CARTESIAN_POINT('Ctrl Pts',(5.57969076442153,39.8281981964826,-15.5279657157206));
#49285=CARTESIAN_POINT('Ctrl Pts',(5.5553990454623,39.9266703282958,-15.5366515625495));
#49286=CARTESIAN_POINT('Ctrl Pts',(5.55338471517728,39.9348358845363,-15.5373718147617));
#49287=CARTESIAN_POINT('Ctrl Pts',(5.55135754681633,39.9429997503324,-15.5380962180081));
#49288=CARTESIAN_POINT('Ctrl Pts',(5.54931748055969,39.9511619183062,-15.5388247785975));
#49289=CARTESIAN_POINT('Ctrl Pts',(5.53815638953542,39.9958166933237,-15.5428106937748));
#49290=CARTESIAN_POINT('Ctrl Pts',(5.52660900541491,40.0404206196005,-15.5469210408861));
#49291=CARTESIAN_POINT('Ctrl Pts',(5.51466417079211,40.0849723231114,-15.551156843479));
#49292=CARTESIAN_POINT('Ctrl Pts',(5.51235605772304,40.0935810960555,-15.5519753321087));
#49293=CARTESIAN_POINT('Ctrl Pts',(5.51003293440113,40.1021885423761,-15.5527985653375));
#49294=CARTESIAN_POINT('Ctrl Pts',(5.50769484480291,40.110794174102,-15.5536265062696));
#49295=CARTESIAN_POINT('Ctrl Pts',(5.50287711171511,40.1285264443873,-15.5553325137837));
#49296=CARTESIAN_POINT('Ctrl Pts',(5.49799592481585,40.1462502263921,-15.5570584685343));
#49297=CARTESIAN_POINT('Ctrl Pts',(5.49305708097302,40.1639430592698,-15.5588021349732));
#49298=CARTESIAN_POINT('Ctrl Pts',(5.49059650190236,40.1727577972257,-15.5596708462106));
#49299=CARTESIAN_POINT('Ctrl Pts',(5.48812116123534,40.1815664747305,-15.5605441128286));
#49300=CARTESIAN_POINT('Ctrl Pts',(5.48563167606625,40.1903666381514,-15.5614216932303));
#49301=CARTESIAN_POINT('Ctrl Pts',(5.48069927406808,40.2078023490285,-15.563160438004));
#49302=CARTESIAN_POINT('Ctrl Pts',(5.47570951682564,40.225211449671,-15.56491676568));
#49303=CARTESIAN_POINT('Ctrl Pts',(5.47066250971218,40.2425923596256,-15.5666904547911));
#49304=CARTESIAN_POINT('Ctrl Pts',(5.46805116268897,40.2515853304003,-15.5676081705138));
#49305=CARTESIAN_POINT('Ctrl Pts',(5.46542444821896,40.2605708241239,-15.5685305485455));
#49306=CARTESIAN_POINT('Ctrl Pts',(5.46278232737112,40.2695488251422,-15.5694575770565));
#49307=CARTESIAN_POINT('Ctrl Pts',(5.43468911829116,40.3650103404363,-15.5793145091508));
#49308=CARTESIAN_POINT('Ctrl Pts',(5.40485794134804,40.4596263778678,-15.5896979385596));
#49309=CARTESIAN_POINT('Ctrl Pts',(5.37323020349376,40.5533733304178,-15.6005915390615));
#49310=CARTESIAN_POINT('Ctrl Pts',(5.3351536160963,40.6662351496368,-15.6137063287912));
#49311=CARTESIAN_POINT('Ctrl Pts',(5.29447121827874,40.7778361260763,-15.6275612366279));
#49312=CARTESIAN_POINT('Ctrl Pts',(5.25107269225853,40.8881316463221,-15.6421301484521));
#49313=CARTESIAN_POINT('Ctrl Pts',(5.21559399463491,40.9782992573194,-15.6540403690221));
#49314=CARTESIAN_POINT('Ctrl Pts',(5.17830112171146,41.0675948734014,-15.6664279778806));
#49315=CARTESIAN_POINT('Ctrl Pts',(5.13910957611281,41.155983365789,-15.679273903052));
#49316=CARTESIAN_POINT('Ctrl Pts',(5.09554371104179,41.254237238515,-15.6935536114479));
#49317=CARTESIAN_POINT('Ctrl Pts',(5.04963603199427,41.3513725988285,-15.7083982580537));
#49318=CARTESIAN_POINT('Ctrl Pts',(5.00126317578049,41.4473382083884,-15.7237835817552));
#49319=CARTESIAN_POINT('Ctrl Pts',(4.99592362906449,41.4579311916331,-15.7254818617634));
#49320=CARTESIAN_POINT('Ctrl Pts',(4.9905540005862,41.4685099032567,-15.7271867431753));
#49321=CARTESIAN_POINT('Ctrl Pts',(4.98515414659887,41.4790742849983,-15.7288981856539));
#49322=CARTESIAN_POINT('Ctrl Pts',(4.94163479931358,41.5642164016083,-15.7426913103871));
#49323=CARTESIAN_POINT('Ctrl Pts',(4.89615436809763,41.6484285807815,-15.7569108569489));
#49324=CARTESIAN_POINT('Ctrl Pts',(4.84860359708565,41.7316662063295,-15.771529762144));
#49325=CARTESIAN_POINT('Ctrl Pts',(4.79515275549666,41.8252319055333,-15.7879625721524));
#49326=CARTESIAN_POINT('Ctrl Pts',(4.7390875857014,41.9175670258641,-15.8048995653748));
#49327=CARTESIAN_POINT('Ctrl Pts',(4.68023107128565,42.0085977892414,-15.8223083797611));
#49328=CARTESIAN_POINT('Ctrl Pts',(4.6734321579909,42.0191133672279,-15.8243193894302));
#49329=CARTESIAN_POINT('Ctrl Pts',(4.66659499601975,42.0296129979074,-15.8263369893176));
#49330=CARTESIAN_POINT('Ctrl Pts',(4.65972037206363,42.0400950170412,-15.8283608138738));
#49331=CARTESIAN_POINT('Ctrl Pts',(4.65171701528829,42.0522980610753,-15.8307169267429));
#49332=CARTESIAN_POINT('Ctrl Pts',(4.64366667531103,42.064470958696,-15.8330802653263));
#49333=CARTESIAN_POINT('Ctrl Pts',(4.63557576166612,42.076603952368,-15.8354487521939));
#49334=CARTESIAN_POINT('Ctrl Pts',(4.62860930468073,42.08705073035,-15.8374880721778));
#49335=CARTESIAN_POINT('Ctrl Pts',(4.62161112726301,42.0974703956641,-15.8395316899087));
#49336=CARTESIAN_POINT('Ctrl Pts',(4.61458421977622,42.1078582381447,-15.8415785980626));
#49337=CARTESIAN_POINT('Ctrl Pts',(4.60643986708164,42.1198979943329,-15.8439510132352));
#49338=CARTESIAN_POINT('Ctrl Pts',(4.59825427875283,42.1318990443132,-15.8463286271726));
#49339=CARTESIAN_POINT('Ctrl Pts',(4.59002734719915,42.143861320884,-15.8487112713859));
#49340=CARTESIAN_POINT('Ctrl Pts',(4.58291897753297,42.1541971652215,-15.8507699631035));
#49341=CARTESIAN_POINT('Ctrl Pts',(4.57577995255875,42.1645037551717,-15.8528323494342));
#49342=CARTESIAN_POINT('Ctrl Pts',(4.56861020602952,42.1747810570319,-15.8548983215082));
#49343=CARTESIAN_POINT('Ctrl Pts',(4.54486512980106,42.2088178692257,-15.8617404970554));
#49344=CARTESIAN_POINT('Ctrl Pts',(4.52078312516702,42.2425334732247,-15.8686220086643));
#49345=CARTESIAN_POINT('Ctrl Pts',(4.49636147268642,42.2759263536235,-15.8755388446782));
#49346=CARTESIAN_POINT('Ctrl Pts',(4.48898761919182,42.286008972235,-15.8776273084074));
#49347=CARTESIAN_POINT('Ctrl Pts',(4.48158279691073,42.2960621611675,-15.8797189935682));
#49348=CARTESIAN_POINT('Ctrl Pts',(4.47414693197282,42.3060858788081,-15.8818137890834));
#49349=CARTESIAN_POINT('Ctrl Pts',(4.41745663849877,42.3825057034674,-15.8977843013931));
#49350=CARTESIAN_POINT('Ctrl Pts',(4.35896286596554,42.4572133051137,-15.9139357728764));
#49351=CARTESIAN_POINT('Ctrl Pts',(4.2986246258115,42.5301826611137,-15.9302174160106));
#49352=CARTESIAN_POINT('Ctrl Pts',(4.29080043326918,42.5396447582775,-15.9323286925487));
#49353=CARTESIAN_POINT('Ctrl Pts',(4.28294516445785,42.5490775657595,-15.9344421737816));
#49354=CARTESIAN_POINT('Ctrl Pts',(4.27505873967226,42.5584810363298,-15.9365577453965));
#49355=CARTESIAN_POINT('Ctrl Pts',(4.21414970207225,42.6311066376772,-15.9528968895007));
#49356=CARTESIAN_POINT('Ctrl Pts',(4.15138652022233,42.7019861374178,-15.9693615490908));
#49357=CARTESIAN_POINT('Ctrl Pts',(4.08671233631728,42.7710801369558,-15.9858954857721));
#49358=CARTESIAN_POINT('Ctrl Pts',(4.01366422126778,42.8491203397498,-16.0045702155636));
#49359=CARTESIAN_POINT('Ctrl Pts',(3.93817953530957,42.9248840324747,-16.0233330708574));
#49360=CARTESIAN_POINT('Ctrl Pts',(3.86016029203208,42.9982987128954,-16.0421060217848));
#49361=CARTESIAN_POINT('Ctrl Pts',(3.8518401275407,43.0061278354493,-16.0441080155641));
#49362=CARTESIAN_POINT('Ctrl Pts',(3.84349115471137,43.0139302653613,-16.0461101186922));
#49363=CARTESIAN_POINT('Ctrl Pts',(3.83511326420841,43.0217059258672,-16.0481122332415));
#49364=CARTESIAN_POINT('Ctrl Pts',(3.76493060726311,43.0868436253411,-16.0648842020959));
#49365=CARTESIAN_POINT('Ctrl Pts',(3.69271486095244,43.1500991909802,-16.0816562485315));
#49366=CARTESIAN_POINT('Ctrl Pts',(3.61837518308114,43.2114031096698,-16.0983651920145));
#49367=CARTESIAN_POINT('Ctrl Pts',(3.61006299158089,43.218257725219,-16.1002334801477));
#49368=CARTESIAN_POINT('Ctrl Pts',(3.60172445231722,43.2250877486212,-16.102100932142));
#49369=CARTESIAN_POINT('Ctrl Pts',(3.59335932873714,43.231893174722,-16.1039674842747));
#49370=CARTESIAN_POINT('Ctrl Pts',(3.55985259783473,43.2591524947852,-16.1114440098067));
#49371=CARTESIAN_POINT('Ctrl Pts',(3.52591396943127,43.2860208906304,-16.118907152479));
#49372=CARTESIAN_POINT('Ctrl Pts',(3.49153886080801,43.3124866299023,-16.1263497545402));
#49373=CARTESIAN_POINT('Ctrl Pts',(3.48330870851789,43.3188231063064,-16.1281316761355));
#49374=CARTESIAN_POINT('Ctrl Pts',(3.47505293205268,43.3251369536414,-16.1299125489504));
#49375=CARTESIAN_POINT('Ctrl Pts',(3.46677335588102,43.3314265638105,-16.1316918672206));
#49376=CARTESIAN_POINT('Ctrl Pts',(3.46424918367963,43.333344060409,-16.1322343232138));
#49377=CARTESIAN_POINT('Ctrl Pts',(3.46172361412074,43.3352586871739,-16.132776459702));
#49378=CARTESIAN_POINT('Ctrl Pts',(3.45919669857441,43.337170407617,-16.1333182638196));
#49379=CARTESIAN_POINT('Ctrl Pts',(3.44838120836836,43.3453527917724,-16.1356372479805));
#49380=CARTESIAN_POINT('Ctrl Pts',(3.43753889753725,43.353483581322,-16.1379506072427));
#49381=CARTESIAN_POINT('Ctrl Pts',(3.42666980412844,43.3615628623861,-16.1402581785502));
#49382=CARTESIAN_POINT('Ctrl Pts',(3.4049316173108,43.3777214245144,-16.1448733211651));
#49383=CARTESIAN_POINT('Ctrl Pts',(3.38308629026371,43.3936739435806,-16.1494653142701));
#49384=CARTESIAN_POINT('Ctrl Pts',(3.36113403095232,43.4094213680059,-16.1540328721413));
#49385=CARTESIAN_POINT('Ctrl Pts',(3.35312024544098,43.4151700465319,-16.1557002827059));
#49386=CARTESIAN_POINT('Ctrl Pts',(3.34509218035729,43.4208913270488,-16.157364442952));
#49387=CARTESIAN_POINT('Ctrl Pts',(3.33704985191415,43.4265852616513,-16.1590252888546));
#49388=CARTESIAN_POINT('Ctrl Pts',(3.25697039112238,43.4832811819894,-16.1755627438067));
#49389=CARTESIAN_POINT('Ctrl Pts',(3.17548097013196,43.5372743319747,-16.1917713019819));
#49390=CARTESIAN_POINT('Ctrl Pts',(3.09258174654553,43.5885854537716,-16.2075894156856));
#49391=CARTESIAN_POINT('Ctrl Pts',(3.00135700756265,43.6450497183369,-16.2249961323156));
#49392=CARTESIAN_POINT('Ctrl Pts',(2.90842605358659,43.698268165434,-16.2419299379221));
#49393=CARTESIAN_POINT('Ctrl Pts',(2.81377567269317,43.7482407963283,-16.2583106986815));
#49394=CARTESIAN_POINT('Ctrl Pts',(2.80721705605344,43.7517035539572,-16.2594457720861));
#49395=CARTESIAN_POINT('Ctrl Pts',(2.80065019446355,43.7551507511571,-16.2605781876481));
#49396=CARTESIAN_POINT('Ctrl Pts',(2.7940750859381,43.7585823937821,-16.2617079181173));
#49397=CARTESIAN_POINT('Ctrl Pts',(2.70576181166361,43.8046743472732,-16.2768818420762));
#49398=CARTESIAN_POINT('Ctrl Pts',(2.61595748637249,43.8479530702011,-16.2915716528802));
#49399=CARTESIAN_POINT('Ctrl Pts',(2.52463667353454,43.888389861414,-16.3057109554111));
#49400=CARTESIAN_POINT('Ctrl Pts',(2.51914011705615,43.8908237327277,-16.3065619933346));
#49401=CARTESIAN_POINT('Ctrl Pts',(2.51363806443321,43.8932473037575,-16.307411037061));
#49402=CARTESIAN_POINT('Ctrl Pts',(2.50813050985484,43.8956605680324,-16.3082580720792));
#49403=CARTESIAN_POINT('Ctrl Pts',(2.41532189681294,43.936326839617,-16.3225315838741));
#49404=CARTESIAN_POINT('Ctrl Pts',(2.32095115683523,43.9740667478834,-16.3362348517856));
#49405=CARTESIAN_POINT('Ctrl Pts',(2.22497391796444,44.0088152926355,-16.3492963499814));
#49406=CARTESIAN_POINT('Ctrl Pts',(2.22078398009584,44.0103322590043,-16.3498665566945));
#49407=CARTESIAN_POINT('Ctrl Pts',(2.21659097944139,44.011843522778,-16.3504355403514));
#49408=CARTESIAN_POINT('Ctrl Pts',(2.21239491225654,44.0133490785428,-16.3510032949731));
#49409=CARTESIAN_POINT('Ctrl Pts',(2.16568019776689,44.0301103944604,-16.3573240934465));
#49410=CARTESIAN_POINT('Ctrl Pts',(2.11858514986288,44.0461637036814,-16.3634925290769));
#49411=CARTESIAN_POINT('Ctrl Pts',(2.07110297782734,44.0614982206348,-16.3695000678039));
#49412=CARTESIAN_POINT('Ctrl Pts',(2.06766461695933,44.0626086501026,-16.369935096051));
#49413=CARTESIAN_POINT('Ctrl Pts',(2.06422431548232,44.0637152812176,-16.3703692692713));
#49414=CARTESIAN_POINT('Ctrl Pts',(2.06078205357121,44.0648181159706,-16.3708025865466));
#49415=CARTESIAN_POINT('Ctrl Pts',(2.0353054952823,44.0729803170441,-16.3740096152693));
#49416=CARTESIAN_POINT('Ctrl Pts',(2.00972154956067,44.0809345613566,-16.3771697632539));
#49417=CARTESIAN_POINT('Ctrl Pts',(1.98402190675294,44.0886811098014,-16.3802825700146));
#49418=CARTESIAN_POINT('Ctrl Pts',(1.96093443196556,44.0956402820843,-16.3830789842739));
#49419=CARTESIAN_POINT('Ctrl Pts',(1.93774050146882,44.102435507638,-16.3858387078791));
#49420=CARTESIAN_POINT('Ctrl Pts',(1.91447177282552,44.1090558359448,-16.3885569152829));
#49421=CARTESIAN_POINT('Ctrl Pts',(1.91185576698155,44.109800131768,-16.3888625119728));
#49422=CARTESIAN_POINT('Ctrl Pts',(1.90923900132739,44.1105421640974,-16.3891675621339));
#49423=CARTESIAN_POINT('Ctrl Pts',(1.90662152694395,44.1112819164273,-16.3894720583976));
#49424=CARTESIAN_POINT('Ctrl Pts',(1.80384027180714,44.140330022281,-16.4014288165477));
#49425=CARTESIAN_POINT('Ctrl Pts',(1.70067567536909,44.1656739884806,-16.412450946857));
#49426=CARTESIAN_POINT('Ctrl Pts',(1.59703092198111,44.1874452736728,-16.4225300192871));
#49427=CARTESIAN_POINT('Ctrl Pts',(1.59623408355844,44.1876126550016,-16.4226075089035));
#49428=CARTESIAN_POINT('Ctrl Pts',(1.59543721887446,44.1877798245714,-16.4226849425315));
#49429=CARTESIAN_POINT('Ctrl Pts',(1.59464032793329,44.1879467824285,-16.4227623201619));
#49430=CARTESIAN_POINT('Ctrl Pts',(1.4902358885778,44.2098207184566,-16.4328999283282));
#49431=CARTESIAN_POINT('Ctrl Pts',(1.38538072211209,44.2280603589026,-16.4420763846834));
#49432=CARTESIAN_POINT('Ctrl Pts',(1.28007904888983,44.2427191450539,-16.450270442415));
#49433=CARTESIAN_POINT('Ctrl Pts',(1.27897978977937,44.2428721702028,-16.4503559813465));
#49434=CARTESIAN_POINT('Ctrl Pts',(1.27788048201033,44.2430248051197,-16.4504414132241));
#49435=CARTESIAN_POINT('Ctrl Pts',(1.27678112558196,44.2431770498101,-16.450526738023));
#49436=CARTESIAN_POINT('Ctrl Pts',(1.17261275427984,44.2576028365959,-16.4586116003123));
#49437=CARTESIAN_POINT('Ctrl Pts',(1.06800752483145,44.268525295453,-16.4657350787401));
#49438=CARTESIAN_POINT('Ctrl Pts',(0.962964461020188,44.2759488312969,-16.471876014796));
#49439=CARTESIAN_POINT('Ctrl Pts',(0.959893094589279,44.2761658889299,-16.4720555703437));
#49440=CARTESIAN_POINT('Ctrl Pts',(0.956821353860735,44.2763799553317,-16.4722342859168));
#49441=CARTESIAN_POINT('Ctrl Pts',(0.953749238691236,44.2765910294275,-16.4724121609579));
#49442=CARTESIAN_POINT('Ctrl Pts',(0.850687348730451,44.2836720449596,-16.4783794300541));
#49443=CARTESIAN_POINT('Ctrl Pts',(0.747204104196679,44.2873859651881,-16.4834007362283));
#49444=CARTESIAN_POINT('Ctrl Pts',(0.643293723744948,44.2876920068837,-16.4874550245025));
#49445=CARTESIAN_POINT('Ctrl Pts',(0.638173013631758,44.2877070886378,-16.4876548200848));
#49446=CARTESIAN_POINT('Ctrl Pts',(0.633051265512239,44.2877138871714,-16.4878522670302));
#49447=CARTESIAN_POINT('Ctrl Pts',(0.627928478272138,44.2877123933833,-16.4880473626812));
#49448=CARTESIAN_POINT('Ctrl Pts',(0.57954225879359,44.2876982841195,-16.4898900980021));
#49449=CARTESIAN_POINT('Ctrl Pts',(0.531063351358693,44.2869444885894,-16.4915230658722));
#49450=CARTESIAN_POINT('Ctrl Pts',(0.482490764213168,44.2854433093263,-16.492944026536));
#49451=CARTESIAN_POINT('Ctrl Pts',(0.47631563182451,44.285252461335,-16.4931246761726));
#49452=CARTESIAN_POINT('Ctrl Pts',(0.470138985065216,44.2850495309885,-16.4933018991296));
#49453=CARTESIAN_POINT('Ctrl Pts',(0.463960821511663,44.2848344986047,-16.4934756906589));
#49454=CARTESIAN_POINT('Ctrl Pts',(0.443272462987042,44.2841144355938,-16.4940576534764));
#49455=CARTESIAN_POINT('Ctrl Pts',(0.422567101634483,44.2832586764287,-16.4946011385449));
#49456=CARTESIAN_POINT('Ctrl Pts',(0.401844644788766,44.282266486453,-16.4951059675728));
#49457=CARTESIAN_POINT('Ctrl Pts',(0.395134665523894,44.2819452130532,-16.495269432375));
#49458=CARTESIAN_POINT('Ctrl Pts',(0.38842289375111,44.2816096343698,-16.4954288441383));
#49459=CARTESIAN_POINT('Ctrl Pts',(0.381709326061794,44.2812597228911,-16.4955841967083));
#49460=CARTESIAN_POINT('Ctrl Pts',(0.374961908381315,44.2809080471491,-16.4957403325702));
#49461=CARTESIAN_POINT('Ctrl Pts',(0.368212082100221,44.2805418556977,-16.4958923819046));
#49462=CARTESIAN_POINT('Ctrl Pts',(0.361459979158117,44.2801611282481,-16.4960403334699));
#49463=CARTESIAN_POINT('Ctrl Pts',(0.354478999419505,44.2797674952372,-16.4961933001662));
#49464=CARTESIAN_POINT('Ctrl Pts',(0.347499905430398,44.2793586053598,-16.4963418025197));
#49465=CARTESIAN_POINT('Ctrl Pts',(0.340516126202715,44.2789339995285,-16.4964859594806));
#49466=CARTESIAN_POINT('Ctrl Pts',(0.334023738302003,44.2785392697308,-16.4966199732973));
#49467=CARTESIAN_POINT('Ctrl Pts',(0.327529005644791,44.2781310584524,-16.4967501936259));
#49468=CARTESIAN_POINT('Ctrl Pts',(0.3210340492655,44.2777094964746,-16.496876587379));
#49469=CARTESIAN_POINT('',(1.20079349241742E-9,44.2459666925969,-16.5000000000016));
#49470=CARTESIAN_POINT('Origin',(0.582847305389121,39.8653351592355,-15.2258139418661));
#49471=CARTESIAN_POINT('Ctrl Pts',(1.19175561086315E-9,44.2459666925957,
-16.5000000000016));
#49472=CARTESIAN_POINT('Ctrl Pts',(-0.000287594851848401,44.2459284389849,
-16.5000000000006));
#49473=CARTESIAN_POINT('Ctrl Pts',(-0.000575187647762856,44.2458901592331,
-16.4999999924808));
#49474=CARTESIAN_POINT('Ctrl Pts',(-0.000862777466105232,44.2458518533049,
-16.4999999774429));
#49475=CARTESIAN_POINT('Ctrl Pts',(-0.0103516191796766,44.2445879737586,
-16.4999994812757));
#49476=CARTESIAN_POINT('Ctrl Pts',(-0.0198372289636732,44.2432956404934,
-16.4999908074579));
#49477=CARTESIAN_POINT('Ctrl Pts',(-0.0293292763690019,44.2419734378186,
-16.4999739378784));
#49478=CARTESIAN_POINT('Ctrl Pts',(-0.126346576415198,44.2284593319417,
-16.4998015155357));
#49479=CARTESIAN_POINT('Ctrl Pts',(-0.22254089868835,44.2120370516237,-16.4987750615445));
#49480=CARTESIAN_POINT('Ctrl Pts',(-0.31793273935584,44.1927764300431,-16.4969366481553));
#49481=CARTESIAN_POINT('Ctrl Pts',(-0.329950839341052,44.1903498485418,
-16.4967050325814));
#49482=CARTESIAN_POINT('Ctrl Pts',(-0.341956199703173,44.1878782093579,
-16.4964605269095));
#49483=CARTESIAN_POINT('Ctrl Pts',(-0.353948844961121,44.1853615808569,
-16.4962032109953));
#49484=CARTESIAN_POINT('Ctrl Pts',(-0.446812032272869,44.1658744586372,
-16.4942107251494));
#49485=CARTESIAN_POINT('Ctrl Pts',(-0.53891338367438,44.1436920944281,-16.4914501879687));
#49486=CARTESIAN_POINT('Ctrl Pts',(-0.630262954075812,44.1188466417855,
-16.48795829109));
#49487=CARTESIAN_POINT('Ctrl Pts',(-0.644348813976517,44.1150155393123,
-16.4874198499128));
#49488=CARTESIAN_POINT('Ctrl Pts',(-0.658416797366746,44.1111211141125,
-16.4868640168006));
#49489=CARTESIAN_POINT('Ctrl Pts',(-0.672466915608358,44.1071633726003,
-16.486290922113));
#49490=CARTESIAN_POINT('Ctrl Pts',(-0.761656457698557,44.08203980089,-16.4826529418566));
#49491=CARTESIAN_POINT('Ctrl Pts',(-0.850126501765724,44.0543665861713,
-16.4783194037139));
#49492=CARTESIAN_POINT('Ctrl Pts',(-0.937878878218134,44.0241463006682,
-16.4733233808419));
#49493=CARTESIAN_POINT('Ctrl Pts',(-0.953599764081856,44.0187323201201,
-16.4724283406331));
#49494=CARTESIAN_POINT('Ctrl Pts',(-0.969297601751398,44.013236528157,-16.4715120357243));
#49495=CARTESIAN_POINT('Ctrl Pts',(-0.984972374783481,44.0076588214043,
-16.4705746539486));
#49496=CARTESIAN_POINT('Ctrl Pts',(-1.02006761572815,43.9951705409039,-16.468475890591));
#49497=CARTESIAN_POINT('Ctrl Pts',(-1.05504725157008,43.9822717635392,-16.4662714695351));
#49498=CARTESIAN_POINT('Ctrl Pts',(-1.08991105395408,43.9689613980953,-16.4639634928673));
#49499=CARTESIAN_POINT('Ctrl Pts',(-1.10629194689102,43.9627074712033,-16.4628790810674));
#49500=CARTESIAN_POINT('Ctrl Pts',(-1.122647264236,43.9563626635983,-16.4617718079304));
#49501=CARTESIAN_POINT('Ctrl Pts',(-1.13897696696911,43.9499267937656,-16.460641891158));
#49502=CARTESIAN_POINT('Ctrl Pts',(-1.14781951505116,43.9464417647129,-16.4600300402535));
#49503=CARTESIAN_POINT('Ctrl Pts',(-1.15665336778823,43.9429305052519,-16.4594116322874));
#49504=CARTESIAN_POINT('Ctrl Pts',(-1.16547967269564,43.9393925413287,-16.4587866239445));
#49505=CARTESIAN_POINT('Ctrl Pts',(-1.18214872627634,43.9327108652683,-16.4576062548471));
#49506=CARTESIAN_POINT('Ctrl Pts',(-1.19880065193612,43.92592977154,-16.4564015924395));
#49507=CARTESIAN_POINT('Ctrl Pts',(-1.21541537661102,43.919057552372,-16.4551744063969));
#49508=CARTESIAN_POINT('Ctrl Pts',(-1.22386355918631,43.9155631964098,-16.4545504122024));
#49509=CARTESIAN_POINT('Ctrl Pts',(-1.23229930086346,43.9120464177848,-16.4539208013987));
#49510=CARTESIAN_POINT('Ctrl Pts',(-1.24071965867521,43.9085084561819,-16.4532858337956));
#49511=CARTESIAN_POINT('Ctrl Pts',(-1.25762786584244,43.9014041752157,-16.4520108091447));
#49512=CARTESIAN_POINT('Ctrl Pts',(-1.27447653768259,43.8942138491217,-16.4507140885787));
#49513=CARTESIAN_POINT('Ctrl Pts',(-1.29127166034123,43.8869356668845,-16.4493956999265));
#49514=CARTESIAN_POINT('Ctrl Pts',(-1.37385183559153,43.8511494700897,-16.4429132961857));
#49515=CARTESIAN_POINT('Ctrl Pts',(-1.45507840509518,43.8132674301109,-16.4359115711727));
#49516=CARTESIAN_POINT('Ctrl Pts',(-1.53499451539265,43.7733496234825,-16.4284445958157));
#49517=CARTESIAN_POINT('Ctrl Pts',(-1.55246848750381,43.7646214379243,-16.4268119122597));
#49518=CARTESIAN_POINT('Ctrl Pts',(-1.56987994576714,43.7557961626709,-16.4251570101115));
#49519=CARTESIAN_POINT('Ctrl Pts',(-1.58722914805154,43.7468741126144,-16.4234804086485));
#49520=CARTESIAN_POINT('Ctrl Pts',(-1.68392383369332,43.6971476288631,-16.4141359760485));
#49521=CARTESIAN_POINT('Ctrl Pts',(-1.77868541818864,43.6444153556874,-16.4041175368783));
#49522=CARTESIAN_POINT('Ctrl Pts',(-1.87156724575009,43.5887474390751,-16.3935133157434));
#49523=CARTESIAN_POINT('Ctrl Pts',(-1.94591646107952,43.5441868826368,-16.3850249435693));
#49524=CARTESIAN_POINT('Ctrl Pts',(-2.01905972959809,43.497742839128,-16.3761613437901));
#49525=CARTESIAN_POINT('Ctrl Pts',(-2.09101827632614,43.4494412260899,-16.3669680322317));
#49526=CARTESIAN_POINT('Ctrl Pts',(-2.10895497999385,43.4374013537032,-16.3646764669813));
#49527=CARTESIAN_POINT('Ctrl Pts',(-2.1268178795326,43.4252457496787,-16.3623643762301));
#49528=CARTESIAN_POINT('Ctrl Pts',(-2.14460708840311,43.4129744720201,-16.3600324324806));
#49529=CARTESIAN_POINT('Ctrl Pts',(-2.2152949005473,43.3642129011028,-16.3507661406011));
#49530=CARTESIAN_POINT('Ctrl Pts',(-2.28482159990252,43.3136289353957,-16.3411860785326));
#49531=CARTESIAN_POINT('Ctrl Pts',(-2.35319652713571,43.261229959548,-16.3313338740189));
#49532=CARTESIAN_POINT('Ctrl Pts',(-2.37106047535531,43.2475399619249,-16.3287598417178));
#49533=CARTESIAN_POINT('Ctrl Pts',(-2.38884576178364,43.2337260025664,-16.3261672273417));
#49534=CARTESIAN_POINT('Ctrl Pts',(-2.40655245014132,43.2197880421058,-16.3235567627833));
#49535=CARTESIAN_POINT('Ctrl Pts',(-2.43131192910212,43.2002984214716,-16.319906518254));
#49536=CARTESIAN_POINT('Ctrl Pts',(-2.4559177628072,43.1805664117049,-16.3162213666243));
#49537=CARTESIAN_POINT('Ctrl Pts',(-2.48037013200753,43.1605919335146,-16.3125033029344));
#49538=CARTESIAN_POINT('Ctrl Pts',(-2.49812747829513,43.1460864382296,-16.3098032396432));
#49539=CARTESIAN_POINT('Ctrl Pts',(-2.51580388217014,43.1314530555792,-16.3070858189739));
#49540=CARTESIAN_POINT('Ctrl Pts',(-2.53339936203802,43.1166916692541,-16.3043518017035));
#49541=CARTESIAN_POINT('Ctrl Pts',(-2.53659528477317,43.114010511905,-16.3038552134878));
#49542=CARTESIAN_POINT('Ctrl Pts',(-2.53978839688599,43.1113252501751,-16.303358099636));
#49543=CARTESIAN_POINT('Ctrl Pts',(-2.54297873799425,43.108635851673,-16.3028604587695));
#49544=CARTESIAN_POINT('Ctrl Pts',(-2.5564235447244,43.0973021284585,-16.3007632895188));
#49545=CARTESIAN_POINT('Ctrl Pts',(-2.56982581198324,43.0858891047701,-16.2986556897146));
#49546=CARTESIAN_POINT('Ctrl Pts',(-2.5831748059359,43.0744062107563,-16.2965397397059));
#49547=CARTESIAN_POINT('Ctrl Pts',(-2.58738539041937,43.0707842377798,-16.2958723196512));
#49548=CARTESIAN_POINT('Ctrl Pts',(-2.59159015953406,43.0671557509872,-16.2952041496852));
#49549=CARTESIAN_POINT('Ctrl Pts',(-2.59578791111343,43.0635217980843,-16.2945354333241));
#49550=CARTESIAN_POINT('Ctrl Pts',(-2.59883434722028,43.0608845278398,-16.2940501255041));
#49551=CARTESIAN_POINT('Ctrl Pts',(-2.60187735140753,43.0582441402771,-16.293564487923));
#49552=CARTESIAN_POINT('Ctrl Pts',(-2.60491671719938,43.0556008159899,-16.2930785579784));
#49553=CARTESIAN_POINT('Ctrl Pts',(-2.62249340560043,43.0403144403046,-16.290268419349));
#49554=CARTESIAN_POINT('Ctrl Pts',(-2.63995009420414,43.0249295007639,-16.287448475097));
#49555=CARTESIAN_POINT('Ctrl Pts',(-2.65728973642841,43.0094452202597,-16.2846192743798));
#49556=CARTESIAN_POINT('Ctrl Pts',(-2.73864180813259,42.9367979140711,-16.2713455668467));
#49557=CARTESIAN_POINT('Ctrl Pts',(-2.81740647187134,42.8619806646524,-16.257869986989));
#49558=CARTESIAN_POINT('Ctrl Pts',(-2.89370698839488,42.7850844218323,-16.2442772420212));
#49559=CARTESIAN_POINT('Ctrl Pts',(-2.9532230042938,42.7251037268282,-16.2336746135925));
#49560=CARTESIAN_POINT('Ctrl Pts',(-3.01123780484442,42.6638563555137,-16.2230009895172));
#49561=CARTESIAN_POINT('Ctrl Pts',(-3.0678032857904,42.601379891981,-16.2122972770594));
#49562=CARTESIAN_POINT('Ctrl Pts',(-3.08375568676903,42.5837604961705,-16.2092786531525));
#49563=CARTESIAN_POINT('Ctrl Pts',(-3.09959271192341,42.5660432617362,-16.2062576035456));
#49564=CARTESIAN_POINT('Ctrl Pts',(-3.1153150843048,42.5482286686331,-16.2032349211562));
#49565=CARTESIAN_POINT('Ctrl Pts',(-3.18678728121458,42.4672454636026,-16.189494135371));
#49566=CARTESIAN_POINT('Ctrl Pts',(-3.25589359579216,42.3842532040227,-16.1757190417709));
#49567=CARTESIAN_POINT('Ctrl Pts',(-3.32271183889098,42.2993064142606,-16.1619814398496));
#49568=CARTESIAN_POINT('Ctrl Pts',(-3.37482391194637,42.2330557451528,-16.1512673761191));
#49569=CARTESIAN_POINT('Ctrl Pts',(-3.42554300779128,42.1656150910847,-16.1405763359259));
#49570=CARTESIAN_POINT('Ctrl Pts',(-3.47490173611287,42.0970065664878,-16.1299428989804));
#49571=CARTESIAN_POINT('Ctrl Pts',(-3.48883090471556,42.0776450525431,-16.1269421138898));
#49572=CARTESIAN_POINT('Ctrl Pts',(-3.50265152984663,42.0581903586756,-16.1239458580045));
#49573=CARTESIAN_POINT('Ctrl Pts',(-3.51636409988177,42.0386427804829,-16.1209548424507));
#49574=CARTESIAN_POINT('Ctrl Pts',(-3.56510545985841,41.9691608713351,-16.1103232711678));
#49575=CARTESIAN_POINT('Ctrl Pts',(-3.61247340068011,41.8985222806704,-16.099759789884));
#49576=CARTESIAN_POINT('Ctrl Pts',(-3.65851424794237,41.8267064889586,-16.0892906461908));
#49577=CARTESIAN_POINT('Ctrl Pts',(-3.67132523342633,41.8067235581516,-16.0863775797323));
#49578=CARTESIAN_POINT('Ctrl Pts',(-3.68403837676501,41.7866413785747,-16.0834706554539));
#49579=CARTESIAN_POINT('Ctrl Pts',(-3.69664022626714,41.7664823851024,-16.0805737153154));
#49580=CARTESIAN_POINT('Ctrl Pts',(-3.69855743306794,41.7634154575554,-16.0801329837121));
#49581=CARTESIAN_POINT('Ctrl Pts',(-3.70047201025498,41.7603468390133,-16.0796924955201));
#49582=CARTESIAN_POINT('Ctrl Pts',(-3.70238391075417,41.757276608805,-16.07925226425));
#49583=CARTESIAN_POINT('Ctrl Pts',(-3.71686830527126,41.7340168075681,-16.0759171098327));
#49584=CARTESIAN_POINT('Ctrl Pts',(-3.73118649436856,41.7106850658504,-16.0725996217207));
#49585=CARTESIAN_POINT('Ctrl Pts',(-3.74534174109064,41.6872813480322,-16.0693003967952));
#49586=CARTESIAN_POINT('Ctrl Pts',(-3.77366972281652,41.6404449979715,-16.0626978708744));
#49587=CARTESIAN_POINT('Ctrl Pts',(-3.80134529335873,41.5933204608883,-16.056168507382));
#49588=CARTESIAN_POINT('Ctrl Pts',(-3.82839252587146,41.5459065217004,-16.0497168407379));
#49589=CARTESIAN_POINT('Ctrl Pts',(-3.83991423543571,41.5257089049438,-16.0469685289007));
#49590=CARTESIAN_POINT('Ctrl Pts',(-3.85132220043387,41.5054588928288,-16.0442343936167));
#49591=CARTESIAN_POINT('Ctrl Pts',(-3.8626179551858,41.4851562470067,-16.0415147212928));
#49592=CARTESIAN_POINT('Ctrl Pts',(-3.91542972205789,41.3902339844763,-16.0287992627958));
#49593=CARTESIAN_POINT('Ctrl Pts',(-3.96577569488318,41.2941842813233,-16.0164031290562));
#49594=CARTESIAN_POINT('Ctrl Pts',(-4.01378102990947,41.1970584880573,-16.0043630454092));
#49595=CARTESIAN_POINT('Ctrl Pts',(-4.05205445786877,41.1196225728717,-15.994763794121));
#49596=CARTESIAN_POINT('Ctrl Pts',(-4.08883676825536,41.0415008769695,-15.9853916721705));
#49597=CARTESIAN_POINT('Ctrl Pts',(-4.12418854585123,40.9627184322293,-15.9762657976971));
#49598=CARTESIAN_POINT('Ctrl Pts',(-4.1775183427968,40.8438714585666,-15.9624989925826));
#49599=CARTESIAN_POINT('Ctrl Pts',(-4.22759059698956,40.7235199332857,-15.9492920561166));
#49600=CARTESIAN_POINT('Ctrl Pts',(-4.27455440445767,40.6017235175999,-15.9366948019296));
#49601=CARTESIAN_POINT('Ctrl Pts',(-4.30628985941116,40.5194204661253,-15.9281822980604));
#49602=CARTESIAN_POINT('Ctrl Pts',(-4.33660590845058,40.4364577805763,-15.9199481700165));
#49603=CARTESIAN_POINT('Ctrl Pts',(-4.36554553024948,40.3528526743455,-15.9120084283324));
#49604=CARTESIAN_POINT('Ctrl Pts',(-4.37221368788543,40.333588703607,-15.9101789832378));
#49605=CARTESIAN_POINT('Ctrl Pts',(-4.37880864040679,40.3142905709198,-15.9083651338701));
#49606=CARTESIAN_POINT('Ctrl Pts',(-4.38533078328216,40.2949584322355,-15.9065670430312));
#49607=CARTESIAN_POINT('Ctrl Pts',(-4.40274481558523,40.2433418862676,-15.9017661650757));
#49608=CARTESIAN_POINT('Ctrl Pts',(-4.41964036451411,40.191483202052,-15.8970774727432));
#49609=CARTESIAN_POINT('Ctrl Pts',(-4.43602545975743,40.1393855975829,-15.8925039099366));
#49610=CARTESIAN_POINT('Ctrl Pts',(-4.44421800737909,40.1133367953484,-15.8902171285334));
#49611=CARTESIAN_POINT('Ctrl Pts',(-4.45228294155174,40.0872282629743,-15.8879591292164));
#49612=CARTESIAN_POINT('Ctrl Pts',(-4.4602211938315,40.0610603695998,-15.8857302987635));
#49613=CARTESIAN_POINT('Ctrl Pts',(-4.46250714010584,40.0535249076041,-15.8850884715086));
#49614=CARTESIAN_POINT('Ctrl Pts',(-4.46478259945335,40.0459844688889,-15.8844490579797));
#49615=CARTESIAN_POINT('Ctrl Pts',(-4.4670475891545,40.0384390820634,-15.8838120687771));
#49616=CARTESIAN_POINT('Ctrl Pts',(-4.4726480772472,40.019782110224,-15.8822370283067));
#49617=CARTESIAN_POINT('Ctrl Pts',(-4.47818614257714,40.0010890903067,-15.8806763429741));
#49618=CARTESIAN_POINT('Ctrl Pts',(-4.48365551823457,39.9823832990067,-15.8791320027934));
#49619=CARTESIAN_POINT('Ctrl Pts',(-4.48594316046568,39.9745593423389,-15.8784860610922));
#49620=CARTESIAN_POINT('Ctrl Pts',(-4.48821884891952,39.9667329479437,-15.8778429610696));
#49621=CARTESIAN_POINT('Ctrl Pts',(-4.49048212941797,39.9589057970096,-15.8772028470187));
#49622=CARTESIAN_POINT('Ctrl Pts',(-4.49815744596312,39.9323620870686,-15.8750320697025));
#49623=CARTESIAN_POINT('Ctrl Pts',(-4.50569321252847,39.9057996224596,-15.8728947529067));
#49624=CARTESIAN_POINT('Ctrl Pts',(-4.51309160005012,39.8792187000441,-15.8707909131699));
#49625=CARTESIAN_POINT('Ctrl Pts',(-4.52789012262557,39.8260505766805,-15.86658273676));
#49626=CARTESIAN_POINT('Ctrl Pts',(-4.54213908424658,39.7728086148232,-15.8625085085832));
#49627=CARTESIAN_POINT('Ctrl Pts',(-4.55585476778786,39.7194950587087,-15.8585682624515));
#49628=CARTESIAN_POINT('Ctrl Pts',(-4.56041739946515,39.7017598784514,-15.857257508105));
#49629=CARTESIAN_POINT('Ctrl Pts',(-4.56492117524414,39.6840167959074,-15.8559615946077));
#49630=CARTESIAN_POINT('Ctrl Pts',(-4.56936658116792,39.6662658793576,-15.8546805129273));
#49631=CARTESIAN_POINT('Ctrl Pts',(-4.59582617304182,39.5606102844924,-15.8470553603542));
#49632=CARTESIAN_POINT('Ctrl Pts',(-4.62021701530607,39.4546766082389,-15.8399559209133));
#49633=CARTESIAN_POINT('Ctrl Pts',(-4.64264870943165,39.3484787986427,-15.8333781662229));
#49634=CARTESIAN_POINT('Ctrl Pts',(-4.66178195243537,39.2578967638623,-15.8277676323861));
#49635=CARTESIAN_POINT('Ctrl Pts',(-4.67948651884887,39.1671220345694,-15.8225376116097));
#49636=CARTESIAN_POINT('Ctrl Pts',(-4.69582718945552,39.0761629007493,-15.817686525125));
#49637=CARTESIAN_POINT('Ctrl Pts',(-4.71780191836416,38.9538421982777,-15.8111628448563));
#49638=CARTESIAN_POINT('Ctrl Pts',(-4.73730857665041,38.8311878214691,-15.8053242615517));
#49639=CARTESIAN_POINT('Ctrl Pts',(-4.75445938729691,38.7082138782734,-15.8001631138445));
#49640=CARTESIAN_POINT('Ctrl Pts',(-4.76754387615524,38.6143960860551,-15.7962256335083));
#49641=CARTESIAN_POINT('Ctrl Pts',(-4.77925615587046,38.5203921558907,-15.7926827509398));
#49642=CARTESIAN_POINT('Ctrl Pts',(-4.78964569348943,38.4262084972978,-15.7895311561511));
#49643=CARTESIAN_POINT('Ctrl Pts',(-4.80300125257063,38.3051371404239,-15.7854798391489));
#49644=CARTESIAN_POINT('Ctrl Pts',(-4.81417020258914,38.1837686885202,-15.7820749892995));
#49645=CARTESIAN_POINT('Ctrl Pts',(-4.82322444707439,38.0621123276519,-15.7793072293277));
#49646=CARTESIAN_POINT('Ctrl Pts',(-4.83045479780361,37.964962514771,-15.777097008987));
#49647=CARTESIAN_POINT('Ctrl Pts',(-4.83633583316492,37.8676289962459,-15.7752932949556));
#49648=CARTESIAN_POINT('Ctrl Pts',(-4.84090392814595,37.7701165801615,-15.773891376532));
#49649=CARTESIAN_POINT('Ctrl Pts',(-4.84650627563929,37.6505265886908,-15.7721720527879));
#49650=CARTESIAN_POINT('Ctrl Pts',(-4.85013347106028,37.530667475693,-15.7710569786778));
#49651=CARTESIAN_POINT('Ctrl Pts',(-4.85182630775392,37.4105445950497,-15.7705360637344));
#49652=CARTESIAN_POINT('Ctrl Pts',(-4.85324388282397,37.3099541473224,-15.7700998515232));
#49653=CARTESIAN_POINT('Ctrl Pts',(-4.85330572152953,37.209171080088,-15.770080067804));
#49654=CARTESIAN_POINT('Ctrl Pts',(-4.8520335653668,37.1082211610075,-15.7704714666542));
#49655=CARTESIAN_POINT('Ctrl Pts',(-4.85192676926515,37.099746527047,-15.7705043241544));
#49656=CARTESIAN_POINT('Ctrl Pts',(-4.8518105219929,37.0912699173234,-15.770540088642));
#49657=CARTESIAN_POINT('Ctrl Pts',(-4.85168485778478,37.0827921015805,-15.7705787486076));
#49658=CARTESIAN_POINT('Ctrl Pts',(-4.85127921342682,37.0554256925192,-15.7707035430673));
#49659=CARTESIAN_POINT('Ctrl Pts',(-4.85077526171592,37.0280351670598,-15.770858564662));
#49660=CARTESIAN_POINT('Ctrl Pts',(-4.85017447792787,37.0006622449712,-15.7710433266669));
#49661=CARTESIAN_POINT('Ctrl Pts',(-4.84974491910744,36.981090678032,-15.771175431012));
#49662=CARTESIAN_POINT('Ctrl Pts',(-4.84926584985124,36.9615265823381,-15.7713227417006));
#49663=CARTESIAN_POINT('Ctrl Pts',(-4.84873760633707,36.9419757558118,-15.771485143286));
#49664=CARTESIAN_POINT('Ctrl Pts',(-4.84852704500225,36.9341826679273,-15.7715498776248));
#49665=CARTESIAN_POINT('Ctrl Pts',(-4.84830867043275,36.9263909650895,-15.7716170097219));
#49666=CARTESIAN_POINT('Ctrl Pts',(-4.84808249521163,36.9186004218509,-15.7716865344286));
#49667=CARTESIAN_POINT('Ctrl Pts',(-4.84670202473089,36.8710504961042,-15.7721108815558));
#49668=CARTESIAN_POINT('Ctrl Pts',(-4.84503135746484,36.8235578278631,-15.7726242373588));
#49669=CARTESIAN_POINT('Ctrl Pts',(-4.84307509951819,36.7761213163914,-15.7732248947521));
#49670=CARTESIAN_POINT('Ctrl Pts',(-4.84278217273655,36.7690182527789,-15.7733148361821));
#49671=CARTESIAN_POINT('Ctrl Pts',(-4.84248284554652,36.7619164477046,-15.7734067348033));
#49672=CARTESIAN_POINT('Ctrl Pts',(-4.84217713097072,36.7548158979564,-15.7735005850902));
#49673=CARTESIAN_POINT('Ctrl Pts',(-4.83773173738744,36.6515668519931,-15.7748652614787));
#49674=CARTESIAN_POINT('Ctrl Pts',(-4.83193543756466,36.5485837374455,-15.7766427083583));
#49675=CARTESIAN_POINT('Ctrl Pts',(-4.82482921851815,36.4458582091488,-15.7788156403514));
#49676=CARTESIAN_POINT('Ctrl Pts',(-4.81692578793011,36.331608412288,-15.7812323428295));
#49677=CARTESIAN_POINT('Ctrl Pts',(-4.80740475334953,36.2176767076784,-15.7841380325327));
#49678=CARTESIAN_POINT('Ctrl Pts',(-4.79630431060394,36.1040551082918,-15.7875103516748));
#49679=CARTESIAN_POINT('Ctrl Pts',(-4.78608080239418,35.9994096107421,-15.7906162577387));
#49680=CARTESIAN_POINT('Ctrl Pts',(-4.77451712190974,35.8950272726645,-15.7941181161817));
#49681=CARTESIAN_POINT('Ctrl Pts',(-4.76164247051096,35.79090180384,-15.7979986385364));
#49682=CARTESIAN_POINT('Ctrl Pts',(-4.74796918719025,35.6803172923034,-15.8021198749058));
#49683=CARTESIAN_POINT('Ctrl Pts',(-4.73281698420083,35.570022559524,-15.8066682685036));
#49684=CARTESIAN_POINT('Ctrl Pts',(-4.71620044368527,35.4600140912944,-15.811624538894));
#49685=CARTESIAN_POINT('Ctrl Pts',(-4.70020316056091,35.35410536675,-15.8163961013383));
#49686=CARTESIAN_POINT('Ctrl Pts',(-4.68284862312618,35.2484619634817,-15.8215457136102));
#49687=CARTESIAN_POINT('Ctrl Pts',(-4.66415019672067,35.1430804795454,-15.8270560415562));
#49688=CARTESIAN_POINT('Ctrl Pts',(-4.64513855063192,35.0359337371696,-15.8326586736959));
#49689=CARTESIAN_POINT('Ctrl Pts',(-4.62473763649585,34.9290577615093,-15.8386342613376));
#49690=CARTESIAN_POINT('Ctrl Pts',(-4.60294317012863,34.8224525312729,-15.8449655287671));
#49691=CARTESIAN_POINT('Ctrl Pts',(-4.5810634426253,34.715430255586,-15.8513215644586));
#49692=CARTESIAN_POINT('Ctrl Pts',(-4.55777905932879,34.608680891025,-15.8580361206368));
#49693=CARTESIAN_POINT('Ctrl Pts',(-4.53308543856788,34.5022042629151,-15.8650917553867));
#49694=CARTESIAN_POINT('Ctrl Pts',(-4.50898951620644,34.3983048554899,-15.8719766115523));
#49695=CARTESIAN_POINT('Ctrl Pts',(-4.48355205009227,34.2946650869156,-15.8791862918112));
#49696=CARTESIAN_POINT('Ctrl Pts',(-4.45675032829542,34.1912883713624,-15.8867050896647));
#49697=CARTESIAN_POINT('Ctrl Pts',(-4.42875904625923,34.0833234121347,-15.8945575997715));
#49698=CARTESIAN_POINT('Ctrl Pts',(-4.39927978459254,33.9756453684566,-15.9027472583645));
#49699=CARTESIAN_POINT('Ctrl Pts',(-4.36828648579626,33.8682579088737,-15.9112561785133));
#49700=CARTESIAN_POINT('Ctrl Pts',(-4.33919134807026,33.7674473127784,-15.9192439763033));
#49701=CARTESIAN_POINT('Ctrl Pts',(-4.30876259816216,33.666892675998,-15.9275131965253));
#49702=CARTESIAN_POINT('Ctrl Pts',(-4.27695790139735,33.566601036888,-15.9360490739371));
#49703=CARTESIAN_POINT('Ctrl Pts',(-4.24411573854768,33.4630378943601,-15.9448633908317));
#49704=CARTESIAN_POINT('Ctrl Pts',(-4.20980950791299,33.3597545148029,-15.9539612235864));
#49705=CARTESIAN_POINT('Ctrl Pts',(-4.17398692835289,33.2567596124214,-15.9633277669116));
#49706=CARTESIAN_POINT('Ctrl Pts',(-4.17220721605076,33.2516426918345,-15.9637931089554));
#49707=CARTESIAN_POINT('Ctrl Pts',(-4.17042372259689,33.2465263637597,-15.9642591242467));
#49708=CARTESIAN_POINT('Ctrl Pts',(-4.16863646163622,33.2414106840141,-15.9647258056854));
#49709=CARTESIAN_POINT('Ctrl Pts',(-4.16143009229477,33.22078388217,-15.9666075000131));
#49710=CARTESIAN_POINT('Ctrl Pts',(-4.15416326324634,33.2001706046279,-15.9684997646203));
#49711=CARTESIAN_POINT('Ctrl Pts',(-4.14684307676731,33.1795915530405,-15.9704005109544));
#49712=CARTESIAN_POINT('Ctrl Pts',(-4.14494846185095,33.1742652709555,-15.9708924632247));
#49713=CARTESIAN_POINT('Ctrl Pts',(-4.1430501332869,33.1689408886548,-15.97138501989));
#49714=CARTESIAN_POINT('Ctrl Pts',(-4.14114820751058,33.1636187511498,-15.9718781463994));
#49715=CARTESIAN_POINT('Ctrl Pts',(-4.13387920555399,33.1432779847438,-15.9737628348592));
#49716=CARTESIAN_POINT('Ctrl Pts',(-4.12655565032035,33.1229642452263,-15.9756563719269));
#49717=CARTESIAN_POINT('Ctrl Pts',(-4.1191783081669,33.1026802646875,-15.9775583262229));
#49718=CARTESIAN_POINT('Ctrl Pts',(-4.11716917926544,33.0971561706859,-15.9780763002122));
#49719=CARTESIAN_POINT('Ctrl Pts',(-4.11515603619164,33.0916342148207,-15.9785949049451));
#49720=CARTESIAN_POINT('Ctrl Pts',(-4.11313887522014,33.0861143985711,-15.9791141366833));
#49721=CARTESIAN_POINT('Ctrl Pts',(-4.09646638643248,33.0404913294002,-15.9834057551793));
#49722=CARTESIAN_POINT('Ctrl Pts',(-4.07951944770782,32.9950144102283,-15.9877402079902));
#49723=CARTESIAN_POINT('Ctrl Pts',(-4.06229559308002,32.9496846741593,-15.9921153863065));
#49724=CARTESIAN_POINT('Ctrl Pts',(-4.06005348916727,32.9437839056728,-15.9926849222573));
#49725=CARTESIAN_POINT('Ctrl Pts',(-4.05780669057546,32.9378856329019,-15.9932551488779));
#49726=CARTESIAN_POINT('Ctrl Pts',(-4.05555519190291,32.9319898580281,-15.9938260614973));
#49727=CARTESIAN_POINT('Ctrl Pts',(-4.01648191768603,32.8296725743555,-16.0037338733933));
#49728=CARTESIAN_POINT('Ctrl Pts',(-3.97599387963302,32.728107175804,-16.0138483082294));
#49729=CARTESIAN_POINT('Ctrl Pts',(-3.93405403406182,32.6273098280652,-16.0241448713244));
#49730=CARTESIAN_POINT('Ctrl Pts',(-3.89516634421934,32.5338479675737,-16.0336921060991));
#49731=CARTESIAN_POINT('Ctrl Pts',(-3.85503360934473,32.4410447381093,-16.0433960887567));
#49732=CARTESIAN_POINT('Ctrl Pts',(-3.81361034359909,32.3489216104306,-16.0532367038211));
#49733=CARTESIAN_POINT('Ctrl Pts',(-3.76578719610018,32.2425654880018,-16.0645976908711));
#49734=CARTESIAN_POINT('Ctrl Pts',(-3.71624379047546,32.1371160266171,-16.0761408369553));
#49735=CARTESIAN_POINT('Ctrl Pts',(-3.66490807451357,32.0326063090271,-16.08783542948));
#49736=CARTESIAN_POINT('Ctrl Pts',(-3.62105896674335,31.9433378965044,-16.0978245265119));
#49737=CARTESIAN_POINT('Ctrl Pts',(-3.57590347039246,31.8547544475763,-16.1079243360576));
#49738=CARTESIAN_POINT('Ctrl Pts',(-3.52937024609825,31.7668908548368,-16.1181138393795));
#49739=CARTESIAN_POINT('Ctrl Pts',(-3.47886458044885,31.6715265360095,-16.1291731987021));
#49740=CARTESIAN_POINT('Ctrl Pts',(-3.42674093229675,31.5770072074372,-16.1403371547359));
#49741=CARTESIAN_POINT('Ctrl Pts',(-3.37289884216362,31.4833818651279,-16.1515805667539));
#49742=CARTESIAN_POINT('Ctrl Pts',(-3.36814188911558,31.4751100585103,-16.1525739231213));
#49743=CARTESIAN_POINT('Ctrl Pts',(-3.36337150087235,31.4668452394032,-16.1535679037735));
#49744=CARTESIAN_POINT('Ctrl Pts',(-3.35858762166542,31.458587434145,-16.1545624882756));
#49745=CARTESIAN_POINT('Ctrl Pts',(-3.30922464408307,31.3733783730022,-16.1648252165673));
#49746=CARTESIAN_POINT('Ctrl Pts',(-3.25842773463224,31.2889149064325,-16.1751525710054));
#49747=CARTESIAN_POINT('Ctrl Pts',(-3.2060976538235,31.2052454585662,-16.1855186131939));
#49748=CARTESIAN_POINT('Ctrl Pts',(-3.14869614503902,31.1134674128902,-16.1968892522708));
#49749=CARTESIAN_POINT('Ctrl Pts',(-3.08945202646307,31.0226435126636,-16.2083061104488));
#49750=CARTESIAN_POINT('Ctrl Pts',(-3.02820866784305,30.9328511554004,-16.2197396641263));
#49751=CARTESIAN_POINT('Ctrl Pts',(-3.02242456920364,30.9243707607392,-16.2208195004344));
#49752=CARTESIAN_POINT('Ctrl Pts',(-3.01662265581845,30.9158995510215,-16.2218994815536));
#49753=CARTESIAN_POINT('Ctrl Pts',(-3.01080281003991,30.9074375841179,-16.2229795795674));
#49754=CARTESIAN_POINT('Ctrl Pts',(-2.98581172706806,30.8711009310451,-16.2276176438924));
#49755=CARTESIAN_POINT('Ctrl Pts',(-2.96048834229123,30.8349355875039,-16.2322576875713));
#49756=CARTESIAN_POINT('Ctrl Pts',(-2.93482032948862,30.7989477238023,-16.2368971724292));
#49757=CARTESIAN_POINT('Ctrl Pts',(-2.92878548427683,30.7904865628775,-16.2379879687131));
#49758=CARTESIAN_POINT('Ctrl Pts',(-2.92273189589887,30.7820356435058,-16.2390786786312));
#49759=CARTESIAN_POINT('Ctrl Pts',(-2.91665928180757,30.7735948754177,-16.2401692920316));
#49760=CARTESIAN_POINT('Ctrl Pts',(-2.90681011979196,30.7599048086383,-16.2419381559698));
#49761=CARTESIAN_POINT('Ctrl Pts',(-2.89690782743331,30.7462374756054,-16.2437072886243));
#49762=CARTESIAN_POINT('Ctrl Pts',(-2.88695587177166,30.7325987650693,-16.245475820514));
#49763=CARTESIAN_POINT('Ctrl Pts',(-2.87316387298446,30.7136974470201,-16.2479267548334));
#49764=CARTESIAN_POINT('Ctrl Pts',(-2.85926885064398,30.6948407452796,-16.2503778818989));
#49765=CARTESIAN_POINT('Ctrl Pts',(-2.84529346740514,30.6760627734517,-16.2528244967358));
#49766=CARTESIAN_POINT('Ctrl Pts',(-2.83670886235749,30.6645281007359,-16.2543273694456));
#49767=CARTESIAN_POINT('Ctrl Pts',(-2.8280939989724,30.6530231651964,-16.2558285338661));
#49768=CARTESIAN_POINT('Ctrl Pts',(-2.81944868233181,30.6415484901895,-16.25732785939));
#49769=CARTESIAN_POINT('Ctrl Pts',(-2.76008246856886,30.5627534572668,-16.2676235238816));
#49770=CARTESIAN_POINT('Ctrl Pts',(-2.69925511842709,30.485339208081,-16.2778382567112));
#49771=CARTESIAN_POINT('Ctrl Pts',(-2.6368786599195,30.4094009767723,-16.2879363792964));
#49772=CARTESIAN_POINT('Ctrl Pts',(-2.63023927738889,30.401318072125,-16.2890112286913));
#49773=CARTESIAN_POINT('Ctrl Pts',(-2.62358231505887,30.3932518634772,-16.2900847614957));
#49774=CARTESIAN_POINT('Ctrl Pts',(-2.61690765823121,30.3852024536947,-16.2911569358438));
#49775=CARTESIAN_POINT('Ctrl Pts',(-2.55421731869184,30.3096000301712,-16.3012271125835));
#49776=CARTESIAN_POINT('Ctrl Pts',(-2.48996657427221,30.235479034662,-16.3111775693049));
#49777=CARTESIAN_POINT('Ctrl Pts',(-2.42403719691135,30.1629475728087,-16.3209694678104));
#49778=CARTESIAN_POINT('Ctrl Pts',(-2.41710390456308,30.1553199893307,-16.3219992074758));
#49779=CARTESIAN_POINT('Ctrl Pts',(-2.4101520341043,30.1477100003574,-16.3230271951822));
#49780=CARTESIAN_POINT('Ctrl Pts',(-2.4031814467617,30.1401177313289,-16.3240533855394));
#49781=CARTESIAN_POINT('Ctrl Pts',(-2.33681073803165,30.0678276571174,-16.3338242955004));
#49782=CARTESIAN_POINT('Ctrl Pts',(-2.26874390704782,29.9971433717163,-16.3434324167189));
#49783=CARTESIAN_POINT('Ctrl Pts',(-2.19883107131641,29.9282027371753,-16.3528328671236));
#49784=CARTESIAN_POINT('Ctrl Pts',(-2.19169909020464,29.921169932709,-16.3537918302958));
#49785=CARTESIAN_POINT('Ctrl Pts',(-2.18454788062778,29.9141552916404,-16.3547486341427));
#49786=CARTESIAN_POINT('Ctrl Pts',(-2.17737728168134,29.907158960102,-16.3557032307762));
#49787=CARTESIAN_POINT('Ctrl Pts',(-2.10687412725336,29.8383692471976,-16.3650890679102));
#49788=CARTESIAN_POINT('Ctrl Pts',(-2.03449764061465,29.7713485484957,-16.3742617525935));
#49789=CARTESIAN_POINT('Ctrl Pts',(-1.96005442350431,29.7062754434188,-16.3831678162274));
#49790=CARTESIAN_POINT('Ctrl Pts',(-1.95284479178456,29.6999732826488,-16.3840303452981));
#49791=CARTESIAN_POINT('Ctrl Pts',(-1.94561575396493,29.6936894074568,-16.3848903754564));
#49792=CARTESIAN_POINT('Ctrl Pts',(-1.93836713178303,29.6874239810535,-16.3857478578924));
#49793=CARTESIAN_POINT('Ctrl Pts',(-1.9043867100566,29.6580526293483,-16.3897676031715));
#49794=CARTESIAN_POINT('Ctrl Pts',(-1.86997530945131,29.6290872976276,-16.3937312402185));
#49795=CARTESIAN_POINT('Ctrl Pts',(-1.8351109162149,29.6005483948712,-16.3976330052129));
#49796=CARTESIAN_POINT('Ctrl Pts',(-1.82791828155379,29.5946607289145,-16.3984379516793));
#49797=CARTESIAN_POINT('Ctrl Pts',(-1.82070636560761,29.5887912119688,-16.3992402648017));
#49798=CARTESIAN_POINT('Ctrl Pts',(-1.8134749722379,29.5829400248555,-16.4000398940084));
#49799=CARTESIAN_POINT('Ctrl Pts',(-1.79944159999906,29.5715851057407,-16.4015916688514));
#49800=CARTESIAN_POINT('Ctrl Pts',(-1.78533484467896,29.5602992475422,-16.4031333296018));
#49801=CARTESIAN_POINT('Ctrl Pts',(-1.77115313127047,29.5490839118721,-16.4046644777802));
#49802=CARTESIAN_POINT('Ctrl Pts',(-1.76398520072988,29.5434152916738,-16.4054383732521));
#49803=CARTESIAN_POINT('Ctrl Pts',(-1.75679804992629,29.5377646410318,-16.4062095906596));
#49804=CARTESIAN_POINT('Ctrl Pts',(-1.74959177812074,29.5321323688344,-16.406978046244));
#49805=CARTESIAN_POINT('Ctrl Pts',(-1.74599580265247,29.5293218291823,-16.4073615104685));
#49806=CARTESIAN_POINT('Ctrl Pts',(-1.74239474124608,29.5265156339911,-16.407744318411));
#49807=CARTESIAN_POINT('Ctrl Pts',(-1.73878901023859,29.5237141339682,-16.4081264187999));
#49808=CARTESIAN_POINT('Ctrl Pts',(-1.72795745749596,29.5152984770063,-16.4092742416704));
#49809=CARTESIAN_POINT('Ctrl Pts',(-1.71707771413516,29.5069205819797,-16.4104163140041));
#49810=CARTESIAN_POINT('Ctrl Pts',(-1.70617071975849,29.4985974823528,-16.4115502304429));
#49811=CARTESIAN_POINT('Ctrl Pts',(-1.69904772283669,29.4931619415451,-16.4122907537277));
#49812=CARTESIAN_POINT('Ctrl Pts',(-1.69191078376265,29.4877479656186,-16.4130280427508));
#49813=CARTESIAN_POINT('Ctrl Pts',(-1.68476277503216,29.4823580137381,-16.413761738001));
#49814=CARTESIAN_POINT('Ctrl Pts',(-1.60434843675212,29.4217216281141,-16.422015731563));
#49815=CARTESIAN_POINT('Ctrl Pts',(-1.52231566709107,29.3639460194625,-16.4298395576141));
#49816=CARTESIAN_POINT('Ctrl Pts',(-1.43855993631844,29.309244218134,-16.4371696403728));
#49817=CARTESIAN_POINT('Ctrl Pts',(-1.43185569577448,29.3048656039077,-16.4377563779914));
#49818=CARTESIAN_POINT('Ctrl Pts',(-1.42514038609923,29.3005066777212,-16.4383399545619));
#49819=CARTESIAN_POINT('Ctrl Pts',(-1.41841394664406,29.2961675441765,-16.4389203379045));
#49820=CARTESIAN_POINT('Ctrl Pts',(-1.33363764949706,29.2414795213092,-16.446235166357));
#49821=CARTESIAN_POINT('Ctrl Pts',(-1.24709418954388,29.1899341559574,-16.4530430363004));
#49822=CARTESIAN_POINT('Ctrl Pts',(-1.1586319078417,29.1417972150289,-16.4592701105399));
#49823=CARTESIAN_POINT('Ctrl Pts',(-1.15256807669246,29.1384975682617,-16.4596969582994));
#49824=CARTESIAN_POINT('Ctrl Pts',(-1.14649522370832,29.135213947848,-16.4601210769962));
#49825=CARTESIAN_POINT('Ctrl Pts',(-1.14041329917068,29.1319464398898,-16.4605424426742));
#49826=CARTESIAN_POINT('Ctrl Pts',(-1.05072914523714,29.08376371666,-16.4667559075235));
#49827=CARTESIAN_POINT('Ctrl Pts',(-0.959073575743241,29.0390825445539,
-16.4723711392616));
#49828=CARTESIAN_POINT('Ctrl Pts',(-0.865245924595666,28.9982558106099,
-16.4772980159103));
#49829=CARTESIAN_POINT('Ctrl Pts',(-0.860089178972269,28.9960119829215,
-16.4775687958913));
#49830=CARTESIAN_POINT('Ctrl Pts',(-0.854925867180395,28.993779805817,-16.4778374964889));
#49831=CARTESIAN_POINT('Ctrl Pts',(-0.849755955267688,28.9915593384622,
-16.4781041026111));
#49832=CARTESIAN_POINT('Ctrl Pts',(-0.804702679736403,28.9722090421252,
-16.4804274456939));
#49833=CARTESIAN_POINT('Ctrl Pts',(-0.75914754240204,28.9537492095873,-16.4825915232));
#49834=CARTESIAN_POINT('Ctrl Pts',(-0.713063751488599,28.9362270883398,
-16.4845849257675));
#49835=CARTESIAN_POINT('Ctrl Pts',(-0.708478823168634,28.9344837927397,
-16.4847832516367));
#49836=CARTESIAN_POINT('Ctrl Pts',(-0.70388866133402,28.9327497797321,-16.4849798880179));
#49837=CARTESIAN_POINT('Ctrl Pts',(-0.69929323933093,28.9310250960911,-16.4851748236235));
#49838=CARTESIAN_POINT('Ctrl Pts',(-0.678143895164944,28.9230876470659,
-16.4860719686978));
#49839=CARTESIAN_POINT('Ctrl Pts',(-0.656883093495827,28.9153478825059,
-16.4869330756139));
#49840=CARTESIAN_POINT('Ctrl Pts',(-0.635507985977491,28.9078108306764,
-16.4877569613718));
#49841=CARTESIAN_POINT('Ctrl Pts',(-0.63124304224397,28.9063069738213,-16.4879213500841));
#49842=CARTESIAN_POINT('Ctrl Pts',(-0.626972842998408,28.9048109407091,
-16.4880842839842));
#49843=CARTESIAN_POINT('Ctrl Pts',(-0.62269785080394,28.9033229476927,-16.4882457340556));
#49844=CARTESIAN_POINT('Ctrl Pts',(-0.613932398969694,28.9002719640835,
-16.4885767715781));
#49845=CARTESIAN_POINT('Ctrl Pts',(-0.605154698954826,28.8972576033564,
-16.4889012600577));
#49846=CARTESIAN_POINT('Ctrl Pts',(-0.596371069871043,28.8942821068495,
-16.4892189364782));
#49847=CARTESIAN_POINT('Ctrl Pts',(-0.583303583379525,28.8898554330865,
-16.4896915466365));
#49848=CARTESIAN_POINT('Ctrl Pts',(-0.570221669843387,28.8855142735489,
-16.4901491375182));
#49849=CARTESIAN_POINT('Ctrl Pts',(-0.557125252287434,28.8812589290143,
-16.4905916000266));
#49850=CARTESIAN_POINT('Ctrl Pts',(-0.553224477579142,28.8799914724549,
-16.4907233877124));
#49851=CARTESIAN_POINT('Ctrl Pts',(-0.549322575762975,28.878731683996,-16.4908538273979));
#49852=CARTESIAN_POINT('Ctrl Pts',(-0.54541973243481,28.8774796356626,-16.4909829093196));
#49853=CARTESIAN_POINT('Ctrl Pts',(-0.444495674024695,28.84510277897,-16.4943208530454));
#49854=CARTESIAN_POINT('Ctrl Pts',(-0.342684747792481,28.8178087937562,
-16.4967606885858));
#49855=CARTESIAN_POINT('Ctrl Pts',(-0.240003537932831,28.7957518568242,
-16.4982544020511));
#49856=CARTESIAN_POINT('Ctrl Pts',(-0.237697811381644,28.7952565640126,
-16.4982879436777));
#49857=CARTESIAN_POINT('Ctrl Pts',(-0.235391639040659,28.794763909971,-16.4983210084487));
#49858=CARTESIAN_POINT('Ctrl Pts',(-0.233085020630584,28.7942738963076,
-16.4983535958337));
#49859=CARTESIAN_POINT('Ctrl Pts',(-0.155894242168747,28.7778756329573,
-16.4994441297518));
#49860=CARTESIAN_POINT('Ctrl Pts',(-0.0782039614584423,28.7644340236271,
-16.5000000902602));
#49861=CARTESIAN_POINT('Ctrl Pts',(3.88757237512749E-9,28.7540327056371,
-16.5000000412986));
#49862=CARTESIAN_POINT('',(-14.1696709099308,34.2228423342584,-8.45401836163377));
#49863=CARTESIAN_POINT('',(-14.1707043820172,35.7980733340469,8.45228604811576));
#49864=CARTESIAN_POINT('Ctrl Pts',(-14.1696709108715,34.2228423340475,-8.45401836462826));
#49865=CARTESIAN_POINT('Ctrl Pts',(-14.1695741904026,34.2248260380075,-8.45418047729493));
#49866=CARTESIAN_POINT('Ctrl Pts',(-14.169477830921,34.2268099148952,-8.45434197865485));
#49867=CARTESIAN_POINT('Ctrl Pts',(-14.167608911444,34.2654359276817,-8.45747422402139));
#49868=CARTESIAN_POINT('Ctrl Pts',(-14.1626664930993,34.3753969946356,-8.46575106737457));
#49869=CARTESIAN_POINT('Ctrl Pts',(-14.1563166525676,34.5588412605337,-8.47636383845025));
#49870=CARTESIAN_POINT('Ctrl Pts',(-14.1524973100839,34.7425201713618,-8.48273692051302));
#49871=CARTESIAN_POINT('Ctrl Pts',(-14.1511586618951,34.8712188614352,-8.48496958670444));
#49872=CARTESIAN_POINT('Ctrl Pts',(-14.1507878943851,34.9424970014783,-8.48558789977024));
#49873=CARTESIAN_POINT('Ctrl Pts',(-14.1507205812306,34.9769967825266,-8.4857001495824));
#49874=CARTESIAN_POINT('Ctrl Pts',(-14.1507126030543,34.9953992459202,-8.48571345413946));
#49875=CARTESIAN_POINT('Ctrl Pts',(-14.1507121043863,34.997705283278,-8.48571428571428));
#49876=CARTESIAN_POINT('Ctrl Pts',(-14.1507121010036,35.1468618614601,-8.48571420142721));
#49877=CARTESIAN_POINT('Ctrl Pts',(-14.1547776737579,35.4396107102406,-8.47893997864034));
#49878=CARTESIAN_POINT('Ctrl Pts',(-14.1728180804027,35.8758599754905,-8.44878247473178));
#49879=CARTESIAN_POINT('Ctrl Pts',(-14.2025224731818,36.3092714765184,-8.39880582800272));
#49880=CARTESIAN_POINT('Ctrl Pts',(-14.2299007195476,36.5963355642442,-8.35229744786236));
#49881=CARTESIAN_POINT('Ctrl Pts',(-14.2531943877412,36.810931871133,-8.31244167087513));
#49882=CARTESIAN_POINT('Ctrl Pts',(-14.2614188842623,36.8823469768069,-8.29832695019776));
#49883=CARTESIAN_POINT('Ctrl Pts',(-14.2744349428304,36.9892940609228,-8.27590368202145));
#49884=CARTESIAN_POINT('Ctrl Pts',(-14.2788886842903,37.0249272832859,-8.26821750742406));
#49885=CARTESIAN_POINT('Ctrl Pts',(-14.2879999806155,37.0959766543479,-8.25246271795894));
#49886=CARTESIAN_POINT('Ctrl Pts',(-14.3112981066859,37.2731437910936,-8.21210092185544));
#49887=CARTESIAN_POINT('Ctrl Pts',(-14.3578215203792,37.5879814951676,-8.13074614008949));
#49888=CARTESIAN_POINT('Ctrl Pts',(-14.4288904455033,37.9993760199721,-8.00406949270557));
#49889=CARTESIAN_POINT('Ctrl Pts',(-14.5082755714546,38.4025980690195,-7.85939563929309));
#49890=CARTESIAN_POINT('Ctrl Pts',(-14.5952758192465,38.7978060707092,-7.69678192603311));
#49891=CARTESIAN_POINT('Ctrl Pts',(-14.657896478309,39.0560030253266,-7.57635264543442));
#49892=CARTESIAN_POINT('Ctrl Pts',(-14.7064265059084,39.24768357466,-7.48146252884525));
#49893=CARTESIAN_POINT('Ctrl Pts',(-14.7228639638505,39.3112490789017,-7.44907072917455));
#49894=CARTESIAN_POINT('Ctrl Pts',(-14.7437193986859,39.3902959250722,-7.40761934898492));
#49895=CARTESIAN_POINT('Ctrl Pts',(-14.7479070967605,39.4060891979786,-7.39927862261931));
#49896=CARTESIAN_POINT('Ctrl Pts',(-14.7563048500418,39.43760451593,-7.38251685050611));
#49897=CARTESIAN_POINT('Ctrl Pts',(-14.7689360904756,39.4847752253455,-7.35725166419566));
#49898=CARTESIAN_POINT('Ctrl Pts',(-14.8156233275035,39.6566118128767,-7.26326438367064));
#49899=CARTESIAN_POINT('Ctrl Pts',(-14.8939488036773,39.9317377406937,-7.10215132097504));
#49900=CARTESIAN_POINT('Ctrl Pts',(-15.0016811570264,40.2860018252939,-6.87185639159196));
#49901=CARTESIAN_POINT('Ctrl Pts',(-15.1119376754938,40.6279408023941,-6.62607667302398));
#49902=CARTESIAN_POINT('Ctrl Pts',(-15.2239734404578,40.9576909989467,-6.36467091771852));
#49903=CARTESIAN_POINT('Ctrl Pts',(-15.3370614584757,41.2752810389499,-6.08736076314172));
#49904=CARTESIAN_POINT('Ctrl Pts',(-15.4126756708071,41.4788475427847,-5.89160359585481));
#49905=CARTESIAN_POINT('Ctrl Pts',(-15.4551351348553,41.5910215779799,-5.77831974861222));
#49906=CARTESIAN_POINT('Ctrl Pts',(-15.4645714783246,41.6158920116934,-5.75304936459231));
#49907=CARTESIAN_POINT('Ctrl Pts',(-15.4833976826855,41.6652775253122,-5.7022525407896));
#49908=CARTESIAN_POINT('Ctrl Pts',(-15.5162167852146,41.750772105944,-5.61268646577723));
#49909=CARTESIAN_POINT('Ctrl Pts',(-15.5813109712958,41.9180543172635,-5.43086629761845));
#49910=CARTESIAN_POINT('Ctrl Pts',(-15.6725353902666,42.1465300010458,-5.16344533267769));
#49911=CARTESIAN_POINT('Ctrl Pts',(-15.7785163448955,42.4040407988642,-4.83016097008632));
#49912=CARTESIAN_POINT('Ctrl Pts',(-15.8803551407113,42.6448820262437,-4.48430381136062));
#49913=CARTESIAN_POINT('Ctrl Pts',(-15.9773923092272,42.8688955481545,-4.1255771403933));
#49914=CARTESIAN_POINT('Ctrl Pts',(-16.0689491798707,43.0757670031137,-3.75357202254097));
#49915=CARTESIAN_POINT('Ctrl Pts',(-16.1258601163662,43.20193282153,-3.49636194469719));
#49916=CARTESIAN_POINT('Ctrl Pts',(-16.15656884454,43.26947017561,-3.34896447224242));
#49917=CARTESIAN_POINT('Ctrl Pts',(-16.1599628057576,43.2769266297891,-3.33254920768214));
#49918=CARTESIAN_POINT('Ctrl Pts',(-16.1667141577056,43.2917440522527,-3.29964186034883));
#49919=CARTESIAN_POINT('Ctrl Pts',(-16.1767895284817,43.3138339314586,-3.25014873591082));
#49920=CARTESIAN_POINT('Ctrl Pts',(-16.1998163579052,43.3641659816838,-3.13431622756455));
#49921=CARTESIAN_POINT('Ctrl Pts',(-16.2439213376448,43.4599998483849,-2.90125815378974));
#49922=CARTESIAN_POINT('Ctrl Pts',(-16.3012520736682,43.583202117882,-2.56434909920735));
#49923=CARTESIAN_POINT('Ctrl Pts',(-16.3606131885796,43.7092439393456,-2.15369772581687));
#49924=CARTESIAN_POINT('Ctrl Pts',(-16.4101690918599,43.8134316244425,-1.73663080953923));
#49925=CARTESIAN_POINT('Ctrl Pts',(-16.4495298899743,43.8955368530516,-1.3130485431318));
#49926=CARTESIAN_POINT('Ctrl Pts',(-16.4782739255189,43.9551426541823,-0.882801768751853));
#49927=CARTESIAN_POINT('Ctrl Pts',(-16.4900529536379,43.979471812853,-0.591393704480866));
#49928=CARTESIAN_POINT('Ctrl Pts',(-16.4950012451008,43.9896869433472,-0.40777871706539));
#49929=CARTESIAN_POINT('Ctrl Pts',(-16.4958675714987,43.9914748615063,-0.37107635173854));
#49930=CARTESIAN_POINT('Ctrl Pts',(-16.497353950166,43.9945419809135,-0.297753965897757));
#49931=CARTESIAN_POINT('Ctrl Pts',(-16.4992147466688,43.9983812928445,-0.187873401187913));
#49932=CARTESIAN_POINT('Ctrl Pts',(-16.5009893405106,44.002039303395,0.0677974336874361));
#49933=CARTESIAN_POINT('Ctrl Pts',(-16.4962759179933,43.9923237789446,0.431019295927046));
#49934=CARTESIAN_POINT('Ctrl Pts',(-16.4792634221366,43.9571888216067,0.863709911301573));
#49935=CARTESIAN_POINT('Ctrl Pts',(-16.4511064396992,43.8988136250866,1.29326197944579));
#49936=CARTESIAN_POINT('Ctrl Pts',(-16.4119922180881,43.8172491800175,1.71969094578633));
#49937=CARTESIAN_POINT('Ctrl Pts',(-16.3787219461102,43.7473246837639,2.00189093332564));
#49938=CARTESIAN_POINT('Ctrl Pts',(-16.3580119895428,43.7035584097628,2.16003652998315));
#49939=CARTESIAN_POINT('Ctrl Pts',(-16.3556824478205,43.6986323471244,2.17760524249224));
#49940=CARTESIAN_POINT('Ctrl Pts',(-16.3509756164775,43.6886727745913,2.21267018387781));
#49941=CARTESIAN_POINT('Ctrl Pts',(-16.3438414997254,43.6735675177399,2.26517652860798));
#49942=CARTESIAN_POINT('Ctrl Pts',(-16.326683133664,43.6371667634837,2.38705769395721));
#49943=CARTESIAN_POINT('Ctrl Pts',(-16.2903559198775,43.5597844011501,2.62831145762857));
#49944=CARTESIAN_POINT('Ctrl Pts',(-16.232934747708,43.4363948317854,2.96594942969864));
#49945=CARTESIAN_POINT('Ctrl Pts',(-16.1558369125918,43.2683468686933,3.36029215003981));
#49946=CARTESIAN_POINT('Ctrl Pts',(-16.0711547872304,43.0806970112392,3.74411043194686));
#49947=CARTESIAN_POINT('Ctrl Pts',(-16.0100316917562,42.9426649113339,3.99311497871483));
#49948=CARTESIAN_POINT('Ctrl Pts',(-15.9625807951282,42.834300206208,4.17732388737971));
#49949=CARTESIAN_POINT('Ctrl Pts',(-15.9464957088409,42.7973714327389,4.23830257009782));
#49950=CARTESIAN_POINT('Ctrl Pts',(-15.9138128435039,42.7218957411724,4.35941450767284));
#49951=CARTESIAN_POINT('Ctrl Pts',(-15.8972125272316,42.6833429047006,4.41955673988955));
#49952=CARTESIAN_POINT('Ctrl Pts',(-15.8466933704575,42.5652823224171,4.59866294426839));
#49953=CARTESIAN_POINT('Ctrl Pts',(-15.7779234599878,42.402642077536,4.83217499176075));
#49954=CARTESIAN_POINT('Ctrl Pts',(-15.6712884768364,42.143462768174,5.16724219532538));
#49955=CARTESIAN_POINT('Ctrl Pts',(-15.5618951178217,41.8693647418838,5.48763911494565));
#49956=CARTESIAN_POINT('Ctrl Pts',(-15.4504486904824,41.5805039812304,5.7937581096588));
#49957=CARTESIAN_POINT('Ctrl Pts',(-15.3376532680843,41.2769000449641,6.08586586123047));
#49958=CARTESIAN_POINT('Ctrl Pts',(-15.2620320937449,41.0645933577144,6.27136226359692));
#49959=CARTESIAN_POINT('Ctrl Pts',(-15.2053415900942,40.90158680001,6.40702654875819));
#49960=CARTESIAN_POINT('Ctrl Pts',(-15.1864463821522,40.846613607407,6.45167758566546));
#49961=CARTESIAN_POINT('Ctrl Pts',(-15.1487072597771,40.7354250324889,6.53979899832712));
#49962=CARTESIAN_POINT('Ctrl Pts',(-15.0923703091726,40.5673516835224,6.66975320244555));
#49963=CARTESIAN_POINT('Ctrl Pts',(-15.0000554476411,40.2808283698595,6.87540602054584));
#49964=CARTESIAN_POINT('Ctrl Pts',(-14.8925110399882,39.9268221531973,7.10514982298711));
#49965=CARTESIAN_POINT('Ctrl Pts',(-14.7889128746132,39.5626135550613,7.318157904284));
#49966=CARTESIAN_POINT('Ctrl Pts',(-14.6899912137661,39.1880940439612,7.51458827196825));
#49967=CARTESIAN_POINT('Ctrl Pts',(-14.5965014824253,38.8030707992935,7.69445703548796));
#49968=CARTESIAN_POINT('Ctrl Pts',(-14.538322404446,38.5391996458362,7.80324419207337));
#49969=CARTESIAN_POINT('Ctrl Pts',(-14.4964515165695,38.3385070734916,7.88059344160958));
#49970=CARTESIAN_POINT('Ctrl Pts',(-14.4759570917779,38.2374631441761,7.91820724260092));
#49971=CARTESIAN_POINT('Ctrl Pts',(-14.4561651015489,38.135351554819,7.95421100845906));
#49972=CARTESIAN_POINT('Ctrl Pts',(-14.4431311948623,38.0670373384614,7.9778533139139));
#49973=CARTESIAN_POINT('Ctrl Pts',(-14.4367073731516,38.0328270049686,7.98947122579105));
#49974=CARTESIAN_POINT('Ctrl Pts',(-14.4050727916094,37.8615760883448,8.04652731310212));
#49975=CARTESIAN_POINT('Ctrl Pts',(-14.3575320825755,37.586160463065,8.13125547960728));
#49976=CARTESIAN_POINT('Ctrl Pts',(-14.2959116329745,37.1688066236194,8.23900264520774));
#49977=CARTESIAN_POINT('Ctrl Pts',(-14.2444368705164,36.7472097164333,8.32759190579159));
#49978=CARTESIAN_POINT('Ctrl Pts',(-14.2035511453535,36.3213337431343,8.39706625486179));
#49979=CARTESIAN_POINT('Ctrl Pts',(-14.1815181263396,36.0039451620904,8.43414643534559));
#49980=CARTESIAN_POINT('Ctrl Pts',(-14.1722466100885,35.8288769445023,8.44970037933995));
#49981=CARTESIAN_POINT('Ctrl Pts',(-14.170704401996,35.7980733355909,8.4522860773754));
#49982=CARTESIAN_POINT('Ctrl Pts',(-14.170704401996,35.7980733355909,8.4522860773754));
#49983=CARTESIAN_POINT('Ctrl Pts',(-14.1650142937913,35.684420795022,8.46182623066452));
#49984=CARTESIAN_POINT('Ctrl Pts',(-14.1605133003307,35.5703099692951,8.46935085018393));
#49985=CARTESIAN_POINT('Ctrl Pts',(-14.1551506650199,35.382916204612,8.47830915393529));
#49986=CARTESIAN_POINT('Ctrl Pts',(-14.1527653559365,35.2734091961459,8.4822897541675));
#49987=CARTESIAN_POINT('Ctrl Pts',(-14.1512998321667,35.1451489583981,8.48473414715993));
#49988=CARTESIAN_POINT('Ctrl Pts',(-14.1509563381337,35.0900718984593,8.4853069916253));
#49989=CARTESIAN_POINT('Ctrl Pts',(-14.1507908381907,35.0533296802779,8.48558298996998));
#49990=CARTESIAN_POINT('Ctrl Pts',(-14.1507398452452,35.0349424468843,8.48566802518057));
#49991=CARTESIAN_POINT('Ctrl Pts',(-14.1505677273441,34.8695234717906,8.48595504833412));
#49992=CARTESIAN_POINT('Ctrl Pts',(-14.154337784268,34.5758999514473,8.47967359793947));
#49993=CARTESIAN_POINT('Ctrl Pts',(-14.1661751055454,34.2831792944904,8.45988898246179));
#49994=CARTESIAN_POINT('Ctrl Pts',(-14.1760617772299,34.1005103374036,8.44329837255236));
#49995=CARTESIAN_POINT('Ctrl Pts',(-14.1781635049883,34.0639906238477,8.43976886981633));
#49996=CARTESIAN_POINT('Ctrl Pts',(-14.1826148355227,33.9909793560335,8.43228648572353));
#49997=CARTESIAN_POINT('Ctrl Pts',(-14.1849621036091,33.9545270470129,8.42833752540023));
#49998=CARTESIAN_POINT('Ctrl Pts',(-14.1923590999347,33.8454073291104,8.41588040125304));
#49999=CARTESIAN_POINT('Ctrl Pts',(-14.2085801409186,33.628016870901,8.38851135454656));
#50000=CARTESIAN_POINT('Ctrl Pts',(-14.242558876821,33.2698693265225,8.33080238485682));
#50001=CARTESIAN_POINT('Ctrl Pts',(-14.2938388156815,32.8465728575125,8.24259551333885));
#50002=CARTESIAN_POINT('Ctrl Pts',(-14.3550258803295,32.4296068752297,8.13567231318596));
#50003=CARTESIAN_POINT('Ctrl Pts',(-14.4255263377446,32.0188604564641,8.01012491229647));
#50004=CARTESIAN_POINT('Ctrl Pts',(-14.4783420074819,31.7491274305981,7.9139754325281));
#50005=CARTESIAN_POINT('Ctrl Pts',(-14.5199872681947,31.5483560263418,7.83714350637601));
#50006=CARTESIAN_POINT('Ctrl Pts',(-14.5413182793014,31.4483525564814,7.79754705060685));
#50007=CARTESIAN_POINT('Ctrl Pts',(-14.5670619058874,31.332350650325,7.74926761389229));
#50008=CARTESIAN_POINT('Ctrl Pts',(-14.5782751718068,31.2827789482509,7.72812768378482));
#50009=CARTESIAN_POINT('Ctrl Pts',(-14.5857903611018,31.2497630278683,7.71393440624095));
#50010=CARTESIAN_POINT('Ctrl Pts',(-14.5895683675641,31.2332685890218,7.70678667876997));
#50011=CARTESIAN_POINT('Ctrl Pts',(-14.6237041832346,31.0851485338514,7.64208780254395));
#50012=CARTESIAN_POINT('Ctrl Pts',(-14.6864314643324,30.8258800442836,7.52155237866732));
#50013=CARTESIAN_POINT('Ctrl Pts',(-14.7857914081875,30.4487285699288,7.3244688139282));
#50014=CARTESIAN_POINT('Ctrl Pts',(-14.8896130143424,30.083018389305,7.11122176429787));
#50015=CARTESIAN_POINT('Ctrl Pts',(-14.9971260006425,29.728539153092,6.88178661466567));
#50016=CARTESIAN_POINT('Ctrl Pts',(-15.107586973597,29.3851765976609,6.63599805956354));
#50017=CARTESIAN_POINT('Ctrl Pts',(-15.1827094430498,29.1636664722939,6.46103123524353));
#50018=CARTESIAN_POINT('Ctrl Pts',(-15.2299741428703,29.0275513750395,6.34810893285796));
#50019=CARTESIAN_POINT('Ctrl Pts',(-15.2441770407058,28.9868916238194,6.31396444350626));
#50020=CARTESIAN_POINT('Ctrl Pts',(-15.2584109480816,28.9464949026306,6.279414905448));
#50021=CARTESIAN_POINT('Ctrl Pts',(-15.2679066407198,28.9196223154397,6.25629147543193));
#50022=CARTESIAN_POINT('Ctrl Pts',(-15.2726590658456,28.9062114640805,6.24468119189695));
#50023=CARTESIAN_POINT('Ctrl Pts',(-15.2964106057722,28.8393748682971,6.18646540617525));
#50024=CARTESIAN_POINT('Ctrl Pts',(-15.3533459015535,28.6809698697406,6.04508845262122));
#50025=CARTESIAN_POINT('Ctrl Pts',(-15.4476616968562,28.4268496179288,5.80119143439749));
#50026=CARTESIAN_POINT('Ctrl Pts',(-15.5592063981134,28.137488294186,5.49524715128581));
#50027=CARTESIAN_POINT('Ctrl Pts',(-15.6684242436608,27.863613730649,5.17588769171355));
#50028=CARTESIAN_POINT('Ctrl Pts',(-15.7746293906152,27.605268899128,4.84285419679768));
#50029=CARTESIAN_POINT('Ctrl Pts',(-15.8771294623924,27.3626395384143,4.49576900414588));
#50030=CARTESIAN_POINT('Ctrl Pts',(-15.9425189610858,27.2115867611153,4.25467413754807));
#50031=CARTESIAN_POINT('Ctrl Pts',(-15.9823115556383,27.1206276984159,4.10082034672238));
#50032=CARTESIAN_POINT('Ctrl Pts',(-15.9941685918194,27.0935988642727,4.05442630335374));
#50033=CARTESIAN_POINT('Ctrl Pts',(-16.0058999460955,27.0669620086443,4.00767092629643));
#50034=CARTESIAN_POINT('Ctrl Pts',(-16.0136924049493,27.0492916411347,3.97641985931698));
#50035=CARTESIAN_POINT('Ctrl Pts',(-16.017575969199,27.0404967069963,3.96074757211319));
#50036=CARTESIAN_POINT('Ctrl Pts',(-16.0368989816428,26.9967922022051,3.88227417674093));
#50037=CARTESIAN_POINT('Ctrl Pts',(-16.0823546071933,26.8945220845182,3.69290418132499));
#50038=CARTESIAN_POINT('Ctrl Pts',(-16.1533708020943,26.7370711648309,3.37213089324311));
#50039=CARTESIAN_POINT('Ctrl Pts',(-16.2305392874646,26.5687922048503,2.97892631034643));
#50040=CARTESIAN_POINT('Ctrl Pts',(-16.2991865268191,26.4212105852304,2.5773593843556));
#50041=CARTESIAN_POINT('Ctrl Pts',(-16.358824265294,26.2945334961653,2.16728320804858));
#50042=CARTESIAN_POINT('Ctrl Pts',(-16.4089359242923,26.1891478876751,1.74848541072101));
#50043=CARTESIAN_POINT('Ctrl Pts',(-16.4356234117713,26.1334700430816,1.46328384430231));
#50044=CARTESIAN_POINT('Ctrl Pts',(-16.4500763362448,26.1033937085539,1.28308059592088));
#50045=CARTESIAN_POINT('Ctrl Pts',(-16.4542451349426,26.0947252636253,1.22887309433461));
#50046=CARTESIAN_POINT('Ctrl Pts',(-16.4581595150294,26.0865940893665,1.17444330933025));
#50047=CARTESIAN_POINT('Ctrl Pts',(-16.4607121333396,26.0812933526595,1.1381071005436));
#50048=CARTESIAN_POINT('Ctrl Pts',(-16.4619601679387,26.0787025731161,1.11991054911913));
#50049=CARTESIAN_POINT('Ctrl Pts',(-16.4680452940168,26.0660740197497,1.02898093092931));
#50050=CARTESIAN_POINT('Ctrl Pts',(-16.4811896615495,26.0388350482944,0.810850535778437));
#50051=CARTESIAN_POINT('Ctrl Pts',(-16.4958379451374,26.0085796010159,0.447797325416032));
#50052=CARTESIAN_POINT('Ctrl Pts',(-16.5019014985441,25.9960803480265,0.0129168588320056));
#50053=CARTESIAN_POINT('Ctrl Pts',(-16.4965250309543,26.0071624248857,-0.421187209207354));
#50054=CARTESIAN_POINT('Ctrl Pts',(-16.4797585463819,26.0417870836736,-0.854516554641816));
#50055=CARTESIAN_POINT('Ctrl Pts',(-16.4610052678583,26.0806622765574,-1.14288393942141));
#50056=CARTESIAN_POINT('Ctrl Pts',(-16.4441004623375,26.1158254145706,-1.35896266188989));
#50057=CARTESIAN_POINT('Ctrl Pts',(-16.4379921612025,26.1285480939795,-1.43095608567496));
#50058=CARTESIAN_POINT('Ctrl Pts',(-16.4281192689933,26.1491499157046,-1.53889658081771));
#50059=CARTESIAN_POINT('Ctrl Pts',(-16.4247074826621,26.1562752423396,-1.57489137072349));
#50060=CARTESIAN_POINT('Ctrl Pts',(-16.4176713964204,26.170983711353,-1.64662271617671));
#50061=CARTESIAN_POINT('Ctrl Pts',(-16.3995385050462,26.2089239746975,-1.82543046804099));
#50062=CARTESIAN_POINT('Ctrl Pts',(-16.3620990851254,26.2876142555016,-2.14265858582978));
#50063=CARTESIAN_POINT('Ctrl Pts',(-16.3025550756539,26.4140141772911,-2.55612272970656));
#50064=CARTESIAN_POINT('Ctrl Pts',(-16.2339549247019,26.5613987045783,-2.96035789316663));
#50065=CARTESIAN_POINT('Ctrl Pts',(-16.1568331540347,26.7294614056885,-3.35556685486244));
#50066=CARTESIAN_POINT('Ctrl Pts',(-16.1000779699745,26.8552023071255,-3.61311125493434));
#50067=CARTESIAN_POINT('Ctrl Pts',(-16.0556336481855,26.954656254176,-3.80406349187298));
#50068=CARTESIAN_POINT('Ctrl Pts',(-16.0405058631815,26.9886660670731,-3.86734639076527));
#50069=CARTESIAN_POINT('Ctrl Pts',(-16.0096449541652,27.0584100439092,-3.99317729314595));
#50070=CARTESIAN_POINT('Ctrl Pts',(-15.9939769145489,27.0939972209781,-4.05546016699478));
#50071=CARTESIAN_POINT('Ctrl Pts',(-15.946310486811,27.2028616000745,-4.24044728136714));
#50072=CARTESIAN_POINT('Ctrl Pts',(-15.8809887484904,27.3536214270733,-4.48214461280834));
#50073=CARTESIAN_POINT('Ctrl Pts',(-15.7784458744819,27.5961148460772,-4.83043553146742));
#50074=CARTESIAN_POINT('Ctrl Pts',(-15.672049918236,27.8546596157552,-5.1649326097885));
#50075=CARTESIAN_POINT('Ctrl Pts',(-15.5624916037538,28.129105638327,-5.48597264019887));
#50076=CARTESIAN_POINT('Ctrl Pts',(-15.4878021056829,28.3226667451366,-5.69117614490112));
#50077=CARTESIAN_POINT('Ctrl Pts',(-15.4313404408399,28.4718461710231,-5.84179828419061));
#50078=CARTESIAN_POINT('Ctrl Pts',(-15.4029985230074,28.5474385488685,-5.91628884328912));
#50079=CARTESIAN_POINT('Ctrl Pts',(-15.3745234531469,28.624546812136,-5.98954995183328));
#50080=CARTESIAN_POINT('Ctrl Pts',(-15.3602665579123,28.6633548051861,-6.025975545843));
#50081=CARTESIAN_POINT('Ctrl Pts',(-15.3555101033097,28.6763356770808,-6.03808558623429));
#50082=CARTESIAN_POINT('Ctrl Pts',(-15.3460025377012,28.7023511935678,-6.0622087309629));
#50083=CARTESIAN_POINT('Ctrl Pts',(-15.3032311621593,28.8196938948245,-6.17035454234009));
#50084=CARTESIAN_POINT('Ctrl Pts',(-15.2226957929703,29.0459577602373,-6.36774026416183));
#50085=CARTESIAN_POINT('Ctrl Pts',(-15.1103581436995,29.3768176414454,-6.62967969820033));
#50086=CARTESIAN_POINT('Ctrl Pts',(-15.0000982739845,29.7190541567933,-6.87530387810371));
#50087=CARTESIAN_POINT('Ctrl Pts',(-14.8926447051201,30.0727157868756,-7.10487256923306));
#50088=CARTESIAN_POINT('Ctrl Pts',(-14.7887465869561,30.4379496584912,-7.31850526348433));
#50089=CARTESIAN_POINT('Ctrl Pts',(-14.722370697791,30.6893179835201,-7.4502913611161));
#50090=CARTESIAN_POINT('Ctrl Pts',(-14.6738777071513,30.880887120718,-7.54510259159816));
#50091=CARTESIAN_POINT('Ctrl Pts',(-14.6499536034456,30.9774327980255,-7.59150060955208));
#50092=CARTESIAN_POINT('Ctrl Pts',(-14.622653427221,31.0914254884024,-7.643853266848));
#50093=CARTESIAN_POINT('Ctrl Pts',(-14.6110895157115,31.1405729393151,-7.66590707737604));
#50094=CARTESIAN_POINT('Ctrl Pts',(-14.603411082087,31.1734034467758,-7.68052426092624));
#50095=CARTESIAN_POINT('Ctrl Pts',(-14.5995879179982,31.1898488485157,-7.68778896006205));
#50096=CARTESIAN_POINT('Ctrl Pts',(-14.5653679358988,31.3379480621503,-7.75269682466588));
#50097=CARTESIAN_POINT('Ctrl Pts',(-14.5070489009751,31.6032252348347,-7.86166211779646));
#50098=CARTESIAN_POINT('Ctrl Pts',(-14.4276988699282,32.0070952985095,-8.00621338887606));
#50099=CARTESIAN_POINT('Ctrl Pts',(-14.3570548434617,32.4169446945395,-8.1320931910977));
#50100=CARTESIAN_POINT('Ctrl Pts',(-14.2956946457161,32.8328361476157,-8.23937842578888));
#50101=CARTESIAN_POINT('Ctrl Pts',(-14.244197923,33.2548692668906,-8.32800172692067));
#50102=CARTESIAN_POINT('Ctrl Pts',(-14.2031474640429,33.6831811080674,-8.39774998726108));
#50103=CARTESIAN_POINT('Ctrl Pts',(-14.1831359783168,33.9730252763557,-8.43142350436688));
#50104=CARTESIAN_POINT('Ctrl Pts',(-14.1731601462849,34.1535912512886,-8.44816816605938));
#50105=CARTESIAN_POINT('Ctrl Pts',(-14.1713604525151,34.1881904088942,-8.45118653281004));
#50106=CARTESIAN_POINT('Ctrl Pts',(-14.1696709108715,34.2228423340475,-8.45401836462826));
#50107=CARTESIAN_POINT('Origin',(3.06151588455592E-17,0.499999999999993,
3.46944695195362E-15));
#50108=CARTESIAN_POINT('',(-2.38806125833734E-15,0.,19.5));
#50109=CARTESIAN_POINT('Origin',(0.,0.,0.));
#50110=CARTESIAN_POINT('Origin',(-2.35744609949178E-15,0.5,19.5));
#50111=CARTESIAN_POINT('Origin',(33.,21.,6.));
#50112=CARTESIAN_POINT('',(17.4999100362558,20.3177785969023,1.04675962888699));
#50113=CARTESIAN_POINT('',(17.5000000502851,20.9999999999962,0.999999421609969));
#50114=CARTESIAN_POINT('Ctrl Pts',(17.4999100362569,20.3177788181702,1.04676123540741));
#50115=CARTESIAN_POINT('Ctrl Pts',(17.4999659873509,20.4233535518093,1.03222017995305));
#50116=CARTESIAN_POINT('Ctrl Pts',(17.5000024591585,20.6351868947168,1.00991574296543));
#50117=CARTESIAN_POINT('Ctrl Pts',(17.4999997636355,20.8632212238551,1.00054557418263));
#50118=CARTESIAN_POINT('Ctrl Pts',(17.5000000120934,20.9851040242355,0.999999990573371));
#50119=CARTESIAN_POINT('Ctrl Pts',(17.5000000502852,21.,0.999999889154119));
#50120=CARTESIAN_POINT('',(17.3583581903393,24.8843450507804,2.85168847095763));
#50121=CARTESIAN_POINT('Ctrl Pts',(17.500000050285,20.9999999999924,0.99999895406582));
#50122=CARTESIAN_POINT('Ctrl Pts',(17.5000002619754,21.0825658826246,0.99999828024815));
#50123=CARTESIAN_POINT('Ctrl Pts',(17.5000004475595,21.1653409669682,1.0020439175894));
#50124=CARTESIAN_POINT('Ctrl Pts',(17.4999984197852,21.2483205520721,1.00617011669214));
#50125=CARTESIAN_POINT('Ctrl Pts',(17.4999981845068,21.2579484979676,1.00664887085397));
#50126=CARTESIAN_POINT('Ctrl Pts',(17.4999979042424,21.2675796394476,1.00715570195213));
#50127=CARTESIAN_POINT('Ctrl Pts',(17.4999975660631,21.2772135619585,1.00769065856536));
#50128=CARTESIAN_POINT('Ctrl Pts',(17.499997093731,21.290669177815,1.00843782781851));
#50129=CARTESIAN_POINT('Ctrl Pts',(17.4999965176582,21.3041303303614,1.00923986594952));
#50130=CARTESIAN_POINT('Ctrl Pts',(17.4999958055237,21.3175970413969,1.01009698967317));
#50131=CARTESIAN_POINT('Ctrl Pts',(17.4999953686873,21.3258577686798,1.01062276506926));
#50132=CARTESIAN_POINT('Ctrl Pts',(17.4999948801857,21.3341206497865,1.01116927435963));
#50133=CARTESIAN_POINT('Ctrl Pts',(17.4999943324047,21.3423847863016,1.01173650875285));
#50134=CARTESIAN_POINT('Ctrl Pts',(17.4999939871881,21.3475929185825,1.01209398490886));
#50135=CARTESIAN_POINT('Ctrl Pts',(17.4999936185644,21.3527990326318,1.0124595168517));
#50136=CARTESIAN_POINT('Ctrl Pts',(17.4999932241172,21.3580029700491,1.01283307974399));
#50137=CARTESIAN_POINT('Ctrl Pts',(17.4999912418066,21.3841555660329,1.01471043502578));
#50138=CARTESIAN_POINT('Ctrl Pts',(17.4999886059075,21.4102591246994,1.01679104223432));
#50139=CARTESIAN_POINT('Ctrl Pts',(17.4999850036602,21.4363140115829,1.01907337101856));
#50140=CARTESIAN_POINT('Ctrl Pts',(17.4999774808885,21.4907258700469,1.02383968419932));
#50141=CARTESIAN_POINT('Ctrl Pts',(17.4999657632806,21.5449255028529,1.02948549995329));
#50142=CARTESIAN_POINT('Ctrl Pts',(17.4999465256887,21.5989157358221,1.0359995859063));
#50143=CARTESIAN_POINT('Ctrl Pts',(17.4999436734614,21.6069205014265,1.03696538524283));
#50144=CARTESIAN_POINT('Ctrl Pts',(17.4999406460128,21.614920660968,1.03795027054161));
#50145=CARTESIAN_POINT('Ctrl Pts',(17.4999374319906,21.6229162233955,1.03895420514678));
#50146=CARTESIAN_POINT('Ctrl Pts',(17.4998979018249,21.7212559003615,1.05130187995543));
#50147=CARTESIAN_POINT('Ctrl Pts',(17.4998312965506,21.8189008936684,1.06652816328134));
#50148=CARTESIAN_POINT('Ctrl Pts',(17.49970544906,21.9158605146828,1.0845951504899));
#50149=CARTESIAN_POINT('Ctrl Pts',(17.4996728061027,21.9410103905533,1.08928145681923));
#50150=CARTESIAN_POINT('Ctrl Pts',(17.4996360623702,21.9661141374527,1.09415888464573));
#50151=CARTESIAN_POINT('Ctrl Pts',(17.4995946625124,21.9911719148272,1.09922677169631));
#50152=CARTESIAN_POINT('Ctrl Pts',(17.4994634776476,22.070573181148,1.11528552436911));
#50153=CARTESIAN_POINT('Ctrl Pts',(17.4992855829644,22.1495128532391,1.13325673599016));
#50154=CARTESIAN_POINT('Ctrl Pts',(17.4990350181115,22.2279909063928,1.15314037837427));
#50155=CARTESIAN_POINT('Ctrl Pts',(17.4989016549127,22.2697608676562,1.16372345146011));
#50156=CARTESIAN_POINT('Ctrl Pts',(17.4987473922076,22.3114000537755,1.17484829718504));
#50157=CARTESIAN_POINT('Ctrl Pts',(17.4985682696136,22.3529084437789,1.18651490676946));
#50158=CARTESIAN_POINT('Ctrl Pts',(17.4983046477483,22.4139979967894,1.20368512138396));
#50159=CARTESIAN_POINT('Ctrl Pts',(17.4979872508062,22.4748042561263,1.22202875240462));
#50160=CARTESIAN_POINT('Ctrl Pts',(17.4975990986111,22.535324706586,1.24155587502242));
#50161=CARTESIAN_POINT('Ctrl Pts',(17.4972279975313,22.593186557663,1.26022519179538));
#50162=CARTESIAN_POINT('Ctrl Pts',(17.4967921349267,22.650787135868,1.27997629693771));
#50163=CARTESIAN_POINT('Ctrl Pts',(17.4962762711174,22.7081242847861,1.30081800440496));
#50164=CARTESIAN_POINT('Ctrl Pts',(17.495885950497,22.7515075792346,1.31658757001683));
#50165=CARTESIAN_POINT('Ctrl Pts',(17.495449538331,22.794739902557,1.3329821562078));
#50166=CARTESIAN_POINT('Ctrl Pts',(17.4949590239254,22.8378195794127,1.3500086351081));
#50167=CARTESIAN_POINT('Ctrl Pts',(17.4947863574794,22.8529840977527,1.35600214226495));
#50168=CARTESIAN_POINT('Ctrl Pts',(17.4946069918883,22.8681297006789,1.36207394804995));
#50169=CARTESIAN_POINT('Ctrl Pts',(17.4944205806443,22.8832563145523,1.36822435196836));
#50170=CARTESIAN_POINT('Ctrl Pts',(17.4942996292821,22.8930710902833,1.37221498963649));
#50171=CARTESIAN_POINT('Ctrl Pts',(17.4941757073595,22.9028778694443,1.3762387260773));
#50172=CARTESIAN_POINT('Ctrl Pts',(17.4940487108157,22.9126766271726,1.38029566268096));
#50173=CARTESIAN_POINT('Ctrl Pts',(17.4937998298968,22.9318796995827,1.38824622636712));
#50174=CARTESIAN_POINT('Ctrl Pts',(17.4935391475876,22.9510520670398,1.39632434040982));
#50175=CARTESIAN_POINT('Ctrl Pts',(17.4932658729586,22.9701936608776,1.40453082497143));
#50176=CARTESIAN_POINT('Ctrl Pts',(17.4931847915148,22.9758730321039,1.40696571480785));
#50177=CARTESIAN_POINT('Ctrl Pts',(17.493102633921,22.9815473996187,1.40941092376088));
#50178=CARTESIAN_POINT('Ctrl Pts',(17.4930193820319,22.9872167194344,1.41186642563823));
#50179=CARTESIAN_POINT('Ctrl Pts',(17.4926788650094,23.0104053812626,1.42190992371267));
#50180=CARTESIAN_POINT('Ctrl Pts',(17.4923200195917,23.0335083877323,1.4321250930782));
#50181=CARTESIAN_POINT('Ctrl Pts',(17.4919416369125,23.0565230929821,1.44251025585013));
#50182=CARTESIAN_POINT('Ctrl Pts',(17.4915114173892,23.0826907165728,1.45431814247713));
#50183=CARTESIAN_POINT('Ctrl Pts',(17.4910560346414,23.108746152075,1.46634627633265));
#50184=CARTESIAN_POINT('Ctrl Pts',(17.490573424049,23.1346902308314,1.47859492778473));
#50185=CARTESIAN_POINT('Ctrl Pts',(17.4889430025631,23.222338086273,1.51997500691212));
#50186=CARTESIAN_POINT('Ctrl Pts',(17.4870025099075,23.3087082899385,1.56386879428171));
#50187=CARTESIAN_POINT('Ctrl Pts',(17.484670372646,23.3938013031274,1.61027161191652));
#50188=CARTESIAN_POINT('Ctrl Pts',(17.4844075785837,23.4033899062411,1.61550045721163));
#50189=CARTESIAN_POINT('Ctrl Pts',(17.4841397939398,23.4129622705904,1.62076120310948));
#50190=CARTESIAN_POINT('Ctrl Pts',(17.4838668892062,23.4225183818683,1.62605387207502));
#50191=CARTESIAN_POINT('Ctrl Pts',(17.4833550818764,23.4404399757191,1.63597977821284));
#50192=CARTESIAN_POINT('Ctrl Pts',(17.4828252468312,23.4583057324984,1.64601871842096));
#50193=CARTESIAN_POINT('Ctrl Pts',(17.4822766627014,23.4761117276956,1.65616865981558));
#50194=CARTESIAN_POINT('Ctrl Pts',(17.4821031455161,23.4817437647882,1.65937908674141));
#50195=CARTESIAN_POINT('Ctrl Pts',(17.4819277230214,23.4873706571504,1.66260112059914));
#50196=CARTESIAN_POINT('Ctrl Pts',(17.4817503962822,23.4929915942163,1.66583428205444));
#50197=CARTESIAN_POINT('Ctrl Pts',(17.4810681208541,23.5146184919007,1.6782740676581));
#50198=CARTESIAN_POINT('Ctrl Pts',(17.4803571578544,23.536172216311,1.6908873144974));
#50199=CARTESIAN_POINT('Ctrl Pts',(17.479617865247,23.5575963138373,1.70364094896084));
#50200=CARTESIAN_POINT('Ctrl Pts',(17.477958282088,23.6056896818678,1.7322706373397));
#50201=CARTESIAN_POINT('Ctrl Pts',(17.476155627395,23.6531491234516,1.76161615556983));
#50202=CARTESIAN_POINT('Ctrl Pts',(17.4741950847171,23.6999895710379,1.7916682113668));
#50203=CARTESIAN_POINT('Ctrl Pts',(17.4739538183649,23.7057538035907,1.79536644755433));
#50204=CARTESIAN_POINT('Ctrl Pts',(17.4737101575725,23.7115086337641,1.7990753667281));
#50205=CARTESIAN_POINT('Ctrl Pts',(17.4734640749961,23.7172540790852,1.80279494547923));
#50206=CARTESIAN_POINT('Ctrl Pts',(17.4698561915424,23.8014896126001,1.85732869926873));
#50207=CARTESIAN_POINT('Ctrl Pts',(17.4657284690486,23.8837098705248,1.91415136870024));
#50208=CARTESIAN_POINT('Ctrl Pts',(17.4609881344011,23.963949431093,1.97321360480535));
#50209=CARTESIAN_POINT('Ctrl Pts',(17.459820095904,23.9837207980343,1.98776678947066));
#50210=CARTESIAN_POINT('Ctrl Pts',(17.4586147877116,24.003371890527,2.00245593874073));
#50211=CARTESIAN_POINT('Ctrl Pts',(17.4573708344984,24.0229032147701,2.01728030685903));
#50212=CARTESIAN_POINT('Ctrl Pts',(17.4532220254637,24.0880437149274,2.06672225670958));
#50213=CARTESIAN_POINT('Ctrl Pts',(17.448643463063,24.1518518885441,2.11766841991422));
#50214=CARTESIAN_POINT('Ctrl Pts',(17.4435781789489,24.2143325102693,2.17010759160733));
#50215=CARTESIAN_POINT('Ctrl Pts',(17.4409485699867,24.2467689144586,2.19733104299799));
#50216=CARTESIAN_POINT('Ctrl Pts',(17.4381875267547,24.2788475170732,2.22495686166756));
#50217=CARTESIAN_POINT('Ctrl Pts',(17.4352871220445,24.3105689414372,2.25298341557022));
#50218=CARTESIAN_POINT('Ctrl Pts',(17.4309254795207,24.3582717716431,2.2951298818427));
#50219=CARTESIAN_POINT('Ctrl Pts',(17.4262487958785,24.4051668825869,2.33818257262917));
#50220=CARTESIAN_POINT('Ctrl Pts',(17.4212265144655,24.4512499209496,2.382143488929));
#50221=CARTESIAN_POINT('Ctrl Pts',(17.4164593011656,24.4949925262151,2.42387174898166));
#50222=CARTESIAN_POINT('Ctrl Pts',(17.4113805934181,24.5380034276377,2.46641830448673));
#50223=CARTESIAN_POINT('Ctrl Pts',(17.4059640464874,24.5802788710682,2.50978464770685));
#50224=CARTESIAN_POINT('Ctrl Pts',(17.4018796228843,24.6121572654009,2.54248565041084));
#50225=CARTESIAN_POINT('Ctrl Pts',(17.3976028472266,24.6436170609292,2.57565326805482));
#50226=CARTESIAN_POINT('Ctrl Pts',(17.39312120798,24.6746548098942,2.60929026496544));
#50227=CARTESIAN_POINT('Ctrl Pts',(17.3914919032077,24.685938616941,2.62151903140077));
#50228=CARTESIAN_POINT('Ctrl Pts',(17.389836221474,24.6971619188012,2.63380468104589));
#50229=CARTESIAN_POINT('Ctrl Pts',(17.3881529018836,24.7083293585338,2.64615245298229));
#50230=CARTESIAN_POINT('Ctrl Pts',(17.3849944327058,24.7292832014004,2.66932099287183));
#50231=CARTESIAN_POINT('Ctrl Pts',(17.3817386979368,24.750040460829,2.69270814089779));
#50232=CARTESIAN_POINT('Ctrl Pts',(17.3783762324105,24.7706297433287,2.71635091114708));
#50233=CARTESIAN_POINT('Ctrl Pts',(17.3750221597084,24.7911676343043,2.73993466826672));
#50234=CARTESIAN_POINT('Ctrl Pts',(17.3715683734,24.8114975528878,2.76372648568205));
#50235=CARTESIAN_POINT('Ctrl Pts',(17.3680128472532,24.8316081557027,2.78771437428848));
#50236=CARTESIAN_POINT('Ctrl Pts',(17.36487758354,24.8493416895462,2.80886689956845));
#50237=CARTESIAN_POINT('Ctrl Pts',(17.3616616180351,24.8669148270245,2.83018311470772));
#50238=CARTESIAN_POINT('Ctrl Pts',(17.3583581903393,24.8843453549118,2.85168822445354));
#50239=CARTESIAN_POINT('',(33.,24.8843448987171,2.85168859421269));
#50240=CARTESIAN_POINT('',(33.,24.8843448987171,2.85168859421269));
#50241=CARTESIAN_POINT('',(33.,25.9586702584784,5.35844776698921));
#50242=CARTESIAN_POINT('Origin',(33.,21.,6.));
#50243=CARTESIAN_POINT('',(16.7001695682977,25.9586702584784,5.35844776698921));
#50244=CARTESIAN_POINT('',(33.,25.9586702584784,5.35844776698921));
#50245=CARTESIAN_POINT('',(12.737739127596,21.0000000000011,11.0000004411269));
#50246=CARTESIAN_POINT('Ctrl Pts',(16.7001695682977,25.9586702584784,5.35844776698921));
#50247=CARTESIAN_POINT('Ctrl Pts',(16.6815168127983,25.965091756189,5.40808065434213));
#50248=CARTESIAN_POINT('Ctrl Pts',(16.6625310547284,25.9707499598162,5.45766867161315));
#50249=CARTESIAN_POINT('Ctrl Pts',(16.6335513874865,25.9781098541553,5.53198088911604));
#50250=CARTESIAN_POINT('Ctrl Pts',(16.6238025350965,25.9803762903565,5.55675364744136));
#50251=CARTESIAN_POINT('Ctrl Pts',(16.6041712694858,25.9845290389781,5.60619093181352));
#50252=CARTESIAN_POINT('Ctrl Pts',(16.5547571761654,25.9939617620173,5.72952013772157));
#50253=CARTESIAN_POINT('Ctrl Pts',(16.4628091547597,26.0025509939011,5.94916276413537));
#50254=CARTESIAN_POINT('Ctrl Pts',(16.3339658850875,25.9970981926254,6.23718843853165));
#50255=CARTESIAN_POINT('Ctrl Pts',(16.1990238439482,25.975504867229,6.52053499024951));
#50256=CARTESIAN_POINT('Ctrl Pts',(16.0581197695729,25.9383420850026,6.79932915724524));
#50257=CARTESIAN_POINT('Ctrl Pts',(15.9113820390098,25.8860095180281,7.07367568619639));
#50258=CARTESIAN_POINT('Ctrl Pts',(15.8097490999726,25.8411687118891,7.25366498784544));
#50259=CARTESIAN_POINT('Ctrl Pts',(15.7450631195531,25.8100512278595,7.36526337579501));
#50260=CARTESIAN_POINT('Ctrl Pts',(15.7255699171593,25.8004838956332,7.3986757512472));
#50261=CARTESIAN_POINT('Ctrl Pts',(15.7059462832927,25.790568372936,7.43198774341748));
#50262=CARTESIAN_POINT('Ctrl Pts',(15.6928349513558,25.7838806180605,7.45417346462433));
#50263=CARTESIAN_POINT('Ctrl Pts',(15.6862625186708,25.7804968261681,7.46525906337382));
#50264=CARTESIAN_POINT('Ctrl Pts',(15.6533687738807,25.7634054144588,7.52056348185176));
#50265=CARTESIAN_POINT('Ctrl Pts',(15.5740790820797,25.7207100606511,7.65217921830482));
#50266=CARTESIAN_POINT('Ctrl Pts',(15.4402879227455,25.6413656133805,7.86612271289071));
#50267=CARTESIAN_POINT('Ctrl Pts',(15.2773765226392,25.533506502716,8.11460835176959));
#50268=CARTESIAN_POINT('Ctrl Pts',(15.1123752770098,25.4132859504897,8.35518462851695));
#50269=CARTESIAN_POINT('Ctrl Pts',(14.9455696744292,25.2808344510266,8.58811755602106));
#50270=CARTESIAN_POINT('Ctrl Pts',(14.7772652512398,25.1361316840594,8.81360820573344));
#50271=CARTESIAN_POINT('Ctrl Pts',(14.6642854201341,25.0313784073232,8.95906654165782));
#50272=CARTESIAN_POINT('Ctrl Pts',(14.5935078612877,24.963246272516,9.04847246989379));
#50273=CARTESIAN_POINT('Ctrl Pts',(14.579344128161,24.9494866302156,9.06627832687579));
#50274=CARTESIAN_POINT('Ctrl Pts',(14.551002317804,24.9216984912121,9.10173957065142));
#50275=CARTESIAN_POINT('Ctrl Pts',(14.5368336488764,24.9076791503186,9.11938314343649));
#50276=CARTESIAN_POINT('Ctrl Pts',(14.4943710470597,24.8652768326577,9.17201279261008));
#50277=CARTESIAN_POINT('Ctrl Pts',(14.4095784208147,24.7790539703943,9.27611920728886));
#50278=CARTESIAN_POINT('Ctrl Pts',(14.3252656298858,24.6885446605887,9.37680712616705));
#50279=CARTESIAN_POINT('Ctrl Pts',(14.2413978267288,24.5950949713964,9.47524663394747));
#50280=CARTESIAN_POINT('Ctrl Pts',(14.2135162363307,24.5634545580881,9.50768481340854));
#50281=CARTESIAN_POINT('Ctrl Pts',(14.1718228401221,24.5152434370381,9.55578104820933));
#50282=CARTESIAN_POINT('Ctrl Pts',(14.1579527172013,24.4990549602159,9.57171244470796));
#50283=CARTESIAN_POINT('Ctrl Pts',(14.1303016537839,24.4664766756373,9.60333940388022));
#50284=CARTESIAN_POINT('Ctrl Pts',(14.061374362152,24.3845007066736,9.68184323456448));
#50285=CARTESIAN_POINT('Ctrl Pts',(13.9391682278281,24.2321564517178,9.81811300931258));
#50286=CARTESIAN_POINT('Ctrl Pts',(13.7808174685474,24.0185079321785,9.98920461970393));
#50287=CARTESIAN_POINT('Ctrl Pts',(13.6277824334408,23.7938596003848,10.1497041947624));
#50288=CARTESIAN_POINT('Ctrl Pts',(13.4809224217402,23.5575429373767,10.2994762499161));
#50289=CARTESIAN_POINT('Ctrl Pts',(13.3878214814433,23.3916173563925,10.3919699226421));
#50290=CARTESIAN_POINT('Ctrl Pts',(13.3201119848075,23.2637316738084,10.4584557028409));
#50291=CARTESIAN_POINT('Ctrl Pts',(13.2978955899498,23.2205285879578,10.4801362425612));
#50292=CARTESIAN_POINT('Ctrl Pts',(13.2651473194537,23.1548159997265,10.5119131194855));
#50293=CARTESIAN_POINT('Ctrl Pts',(13.2543248737765,23.1327546033335,10.5223836950478));
#50294=CARTESIAN_POINT('Ctrl Pts',(13.2329531891877,23.0884738040637,10.5430027132959));
#50295=CARTESIAN_POINT('Ctrl Pts',(13.1801617752673,22.9772854867132,10.5937887952691));
#50296=CARTESIAN_POINT('Ctrl Pts',(13.0910034662183,22.7727198735396,10.6783376891869));
#50297=CARTESIAN_POINT('Ctrl Pts',(12.9859558878995,22.4899170949042,10.7760329787102));
#50298=CARTESIAN_POINT('Ctrl Pts',(12.9261760314419,22.2941648401573,10.8307048734092));
#50299=CARTESIAN_POINT('Ctrl Pts',(12.8856443769417,22.144397524114,10.8675453114143));
#50300=CARTESIAN_POINT('Ctrl Pts',(12.8728519361475,22.0939822410721,10.8791305610273));
#50301=CARTESIAN_POINT('Ctrl Pts',(12.857813812923,22.0303162836497,10.8927106869919));
#50302=CARTESIAN_POINT('Ctrl Pts',(12.8518901929655,22.0047689223521,10.898055842651));
#50303=CARTESIAN_POINT('Ctrl Pts',(12.840473575693,21.9536069121313,10.9083423930165));
#50304=CARTESIAN_POINT('Ctrl Pts',(12.8108590803388,21.8126363177099,10.9349671019215));
#50305=CARTESIAN_POINT('Ctrl Pts',(12.7721821385458,21.5804510522391,10.9694847597745));
#50306=CARTESIAN_POINT('Ctrl Pts',(12.7436588266166,21.2837440777459,10.994766558077));
#50307=CARTESIAN_POINT('Ctrl Pts',(12.7377390466039,21.0894198334434,11.0000007967532));
#50308=CARTESIAN_POINT('Ctrl Pts',(12.737739163667,21.,11.0000002000205));
#50309=CARTESIAN_POINT('',(12.7903686062596,20.3177772724646,10.9532413704546));
#50310=CARTESIAN_POINT('Ctrl Pts',(12.7377390915251,21.0000000000022,11.0000006822333));
#50311=CARTESIAN_POINT('Ctrl Pts',(12.7377390793161,20.983622178571,11.0000007571318));
#50312=CARTESIAN_POINT('Ctrl Pts',(12.7378300444133,20.9672306291789,10.9999203240877));
#50313=CARTESIAN_POINT('Ctrl Pts',(12.7380124482716,20.9508252921112,10.9997589559963));
#50314=CARTESIAN_POINT('Ctrl Pts',(12.7385858332176,20.8992552573562,10.9992516968007));
#50315=CARTESIAN_POINT('Ctrl Pts',(12.7400627630646,20.8475489236218,10.9979446845314));
#50316=CARTESIAN_POINT('Ctrl Pts',(12.7424576654204,20.7957039100975,10.9958245673412));
#50317=CARTESIAN_POINT('Ctrl Pts',(12.7430870890103,20.782078104247,10.9952673622554));
#50318=CARTESIAN_POINT('Ctrl Pts',(12.7437799852258,20.7684417515929,10.9946538807978));
#50319=CARTESIAN_POINT('Ctrl Pts',(12.7445364645497,20.7547976107433,10.993983959556));
#50320=CARTESIAN_POINT('Ctrl Pts',(12.745292797437,20.7411561110799,10.9933141679953));
#50321=CARTESIAN_POINT('Ctrl Pts',(12.7461136211149,20.7274927801926,10.9925871539787));
#50322=CARTESIAN_POINT('Ctrl Pts',(12.7469962187263,20.7138522699735,10.9918052322382));
#50323=CARTESIAN_POINT('Ctrl Pts',(12.7487625516298,20.6865536667273,10.9902403808492));
#50324=CARTESIAN_POINT('Ctrl Pts',(12.7507757360796,20.6593467323395,10.9884561487339));
#50325=CARTESIAN_POINT('Ctrl Pts',(12.7530310509817,20.632228541024,10.9864560715966));
#50326=CARTESIAN_POINT('Ctrl Pts',(12.7575489874744,20.5779043018474,10.9824494375437));
#50327=CARTESIAN_POINT('Ctrl Pts',(12.7630383131326,20.5239378683579,10.9775769882869));
#50328=CARTESIAN_POINT('Ctrl Pts',(12.7694621804001,20.470317030689,10.9718644341959));
#50329=CARTESIAN_POINT('Ctrl Pts',(12.7755909244548,20.4191596240379,10.9664143243999));
#50330=CARTESIAN_POINT('Ctrl Pts',(12.7825699912624,20.3683166034407,10.9602002537898));
#50331=CARTESIAN_POINT('Ctrl Pts',(12.7903700169684,20.317778655448,10.9532395922585));
#50332=CARTESIAN_POINT('Ctrl Pts',(12.7903679797893,20.317776478529,10.9532422454443));
#50333=CARTESIAN_POINT('Ctrl Pts',(12.8434562899674,20.2488326393836,10.9437474142331));
#50334=CARTESIAN_POINT('Ctrl Pts',(12.8972986059335,20.1807439610254,10.9329018818484));
#50335=CARTESIAN_POINT('Ctrl Pts',(12.9518162533638,20.113435242677,10.9207733379228));
#50336=CARTESIAN_POINT('Ctrl Pts',(12.9656958022631,20.0962992382508,10.9176855539405));
#50337=CARTESIAN_POINT('Ctrl Pts',(12.9796187325711,20.0792144661478,10.9145147041637));
#50338=CARTESIAN_POINT('Ctrl Pts',(12.9935840678944,20.0621793443964,10.9112617948878));
#50339=CARTESIAN_POINT('Ctrl Pts',(13.0224694241203,20.0269445613606,10.9045336039041));
#50340=CARTESIAN_POINT('Ctrl Pts',(13.0515370653648,19.9919228033594,10.8974532203922));
#50341=CARTESIAN_POINT('Ctrl Pts',(13.0807805059536,19.9571014126526,10.8900268441503));
#50342=CARTESIAN_POINT('Ctrl Pts',(13.0929332878657,19.9426305857383,10.8869406433118));
#50343=CARTESIAN_POINT('Ctrl Pts',(13.1051207143587,19.928189481138,10.8837934389284));
#50344=CARTESIAN_POINT('Ctrl Pts',(13.1173327522049,19.9137883319846,10.880588317183));
#50345=CARTESIAN_POINT('Ctrl Pts',(13.131284118433,19.8973360650924,10.8769266983903));
#50346=CARTESIAN_POINT('Ctrl Pts',(13.1452710623287,19.880932077011,10.8731886307276));
#50347=CARTESIAN_POINT('Ctrl Pts',(13.1592791699167,19.8645910234659,10.8693784137979));
#50348=CARTESIAN_POINT('Ctrl Pts',(13.1626110417999,19.8607042531433,10.8684721418709));
#50349=CARTESIAN_POINT('Ctrl Pts',(13.1659443845299,19.8568207251754,10.8675617136884));
#50350=CARTESIAN_POINT('Ctrl Pts',(13.1692789570691,19.8529406974006,10.8666471986698));
#50351=CARTESIAN_POINT('Ctrl Pts',(13.1799638464198,19.8405080191595,10.8637168405299));
#50352=CARTESIAN_POINT('Ctrl Pts',(13.1906639107593,19.8281081042167,10.8607439641051));
#50353=CARTESIAN_POINT('Ctrl Pts',(13.2013775403923,19.8157419081973,10.8577292831553));
#50354=CARTESIAN_POINT('Ctrl Pts',(13.2501987616835,19.7593900635776,10.8439916040666));
#50355=CARTESIAN_POINT('Ctrl Pts',(13.2993110129335,19.7037274173886,10.8293833334505));
#50356=CARTESIAN_POINT('Ctrl Pts',(13.3486810035835,19.6487052195288,10.8139383477846));
#50357=CARTESIAN_POINT('Ctrl Pts',(13.3846020902726,19.6086716462361,10.8027007384249));
#50358=CARTESIAN_POINT('Ctrl Pts',(13.4206589640815,19.5689762942216,10.7910211694164));
#50359=CARTESIAN_POINT('Ctrl Pts',(13.4568416858135,19.529604654064,10.7789081502023));
#50360=CARTESIAN_POINT('Ctrl Pts',(13.5422974377372,19.4366173675064,10.7502998223748));
#50361=CARTESIAN_POINT('Ctrl Pts',(13.628455197024,19.345434656823,10.7192738351645));
#50362=CARTESIAN_POINT('Ctrl Pts',(13.7151819439768,19.2558755449294,10.6859395947052));
#50363=CARTESIAN_POINT('Ctrl Pts',(13.7447086494671,19.2253845417066,10.6745907278865));
#50364=CARTESIAN_POINT('Ctrl Pts',(13.7743014848463,19.1950819542101,10.6629740955655));
#50365=CARTESIAN_POINT('Ctrl Pts',(13.8039566392106,19.1649627370347,10.6510916278707));
#50366=CARTESIAN_POINT('Ctrl Pts',(13.8986692758511,19.0687679765156,10.613141400691));
#50367=CARTESIAN_POINT('Ctrl Pts',(13.994016243042,18.9744428419228,10.572479736561));
#50368=CARTESIAN_POINT('Ctrl Pts',(14.0898699742255,18.8818316359896,10.5291680010468));
#50369=CARTESIAN_POINT('Ctrl Pts',(14.1121821389326,18.8602742437526,10.5190861965661));
#50370=CARTESIAN_POINT('Ctrl Pts',(14.1345218256674,18.838809790576,10.5088607420322));
#50371=CARTESIAN_POINT('Ctrl Pts',(14.1568878251665,18.8174369505239,10.4984916258405));
#50372=CARTESIAN_POINT('Ctrl Pts',(14.2609862095409,18.7179610420582,10.450230503283));
#50373=CARTESIAN_POINT('Ctrl Pts',(14.3656526004953,18.6204691146559,10.3988575188189));
#50374=CARTESIAN_POINT('Ctrl Pts',(14.4707618766135,18.5248348974924,10.3443708077614));
#50375=CARTESIAN_POINT('Ctrl Pts',(14.4852538760654,18.5116492770229,10.3368584224046));
#50376=CARTESIAN_POINT('Ctrl Pts',(14.4997543126103,18.4984989874017,10.3292868382026));
#50377=CARTESIAN_POINT('Ctrl Pts',(14.5142629317204,18.4853838352381,10.3216558607537));
#50378=CARTESIAN_POINT('Ctrl Pts',(14.6278157552833,18.3827370879263,10.2619314287243));
#50379=CARTESIAN_POINT('Ctrl Pts',(14.7418676902513,18.2822422550503,10.1985691542882));
#50380=CARTESIAN_POINT('Ctrl Pts',(14.8562915152025,18.1838121582644,10.1314750441048));
#50381=CARTESIAN_POINT('Ctrl Pts',(14.8625245743167,18.178450332507,10.1278201972653));
#50382=CARTESIAN_POINT('Ctrl Pts',(14.868758744578,18.1730946498962,10.1241542524972));
#50383=CARTESIAN_POINT('Ctrl Pts',(14.8749940081487,18.1677451025513,10.1204771851252));
#50384=CARTESIAN_POINT('Ctrl Pts',(14.9010586359397,18.1453829427465,10.1051063204738));
#50385=CARTESIAN_POINT('Ctrl Pts',(14.9271433201623,18.123127177324,10.0895405213415));
#50386=CARTESIAN_POINT('Ctrl Pts',(14.9532438663626,18.1009796955978,10.0737797282947));
#50387=CARTESIAN_POINT('Ctrl Pts',(14.9573597919726,18.0974871484866,10.0712943300492));
#50388=CARTESIAN_POINT('Ctrl Pts',(14.9614763622577,18.0939970892013,10.0688039201571));
#50389=CARTESIAN_POINT('Ctrl Pts',(14.9655933074002,18.0905097361136,10.0663086581148));
#50390=CARTESIAN_POINT('Ctrl Pts',(14.9807052856805,18.0777087872804,10.057149355651));
#50391=CARTESIAN_POINT('Ctrl Pts',(14.9958282965693,18.0649392443808,10.0479210261676));
#50392=CARTESIAN_POINT('Ctrl Pts',(15.0109416992674,18.0522180989575,10.038635963182));
#50393=CARTESIAN_POINT('Ctrl Pts',(15.0240720819448,18.0411660869891,10.0305691874453));
#50394=CARTESIAN_POINT('Ctrl Pts',(15.0371962079393,18.0301497486976,10.0224590067606));
#50395=CARTESIAN_POINT('Ctrl Pts',(15.0503109391063,18.0191714817655,10.0143070815373));
#50396=CARTESIAN_POINT('Ctrl Pts',(15.0522915953529,18.0175134856771,10.0130759345614));
#50397=CARTESIAN_POINT('Ctrl Pts',(15.0542721295603,18.0158562786814,10.0118437808848));
#50398=CARTESIAN_POINT('Ctrl Pts',(15.0562525592192,18.0141998452599,10.0106106089146));
#50399=CARTESIAN_POINT('Ctrl Pts',(15.1166272012074,17.9637024320632,9.97301658689186));
#50400=CARTESIAN_POINT('Ctrl Pts',(15.1768397098642,17.9139782963696,9.93451667600521));
#50401=CARTESIAN_POINT('Ctrl Pts',(15.2368747587599,17.8650116797352,9.8951056799024));
#50402=CARTESIAN_POINT('Ctrl Pts',(15.2391019521154,17.8631951054971,9.89364360216164));
#50403=CARTESIAN_POINT('Ctrl Pts',(15.241328901194,17.8613795738775,9.89218027050538));
#50404=CARTESIAN_POINT('Ctrl Pts',(15.243555605196,17.8595650840876,9.89071568466755));
#50405=CARTESIAN_POINT('Ctrl Pts',(15.3613726174717,17.7635587151838,9.8132230644168));
#50406=CARTESIAN_POINT('Ctrl Pts',(15.4785036808088,17.6704633082561,9.73222462895501));
#50407=CARTESIAN_POINT('Ctrl Pts',(15.5948327357961,17.5802272850139,9.64762340806036));
#50408=CARTESIAN_POINT('Ctrl Pts',(15.6051090011199,17.5722560235203,9.64014991321654));
#50409=CARTESIAN_POINT('Ctrl Pts',(15.6153790028259,17.5643070789325,9.63264830144001));
#50410=CARTESIAN_POINT('Ctrl Pts',(15.6256426604821,17.5563804167023,9.62511850365309));
#50411=CARTESIAN_POINT('Ctrl Pts',(15.7337612215943,17.4728800366758,9.54579873973864));
#50412=CARTESIAN_POINT('Ctrl Pts',(15.8411765311664,17.3918521632454,9.46335197543339));
#50413=CARTESIAN_POINT('Ctrl Pts',(15.9477914636026,17.3133225071355,9.37763444589511));
#50414=CARTESIAN_POINT('Ctrl Pts',(15.9655564119421,17.3002373299278,9.36335157341897));
#50415=CARTESIAN_POINT('Ctrl Pts',(15.9832991118044,17.2872215143357,9.34897786889269));
#50416=CARTESIAN_POINT('Ctrl Pts',(16.0010191155428,17.2742751867206,9.33451265040545));
#50417=CARTESIAN_POINT('Ctrl Pts',(16.0997396259617,17.20214946434,9.25392498386404));
#50418=CARTESIAN_POINT('Ctrl Pts',(16.1977563839487,17.1321797945169,9.17049816457455));
#50419=CARTESIAN_POINT('Ctrl Pts',(16.2949836148963,17.064443368653,9.08405651776282));
#50420=CARTESIAN_POINT('Ctrl Pts',(16.3195919152759,17.0472992178009,9.06217805851518));
#50421=CARTESIAN_POINT('Ctrl Pts',(16.3441495460092,17.0302980831823,9.04010636353868));
#50422=CARTESIAN_POINT('Ctrl Pts',(16.3686551330205,17.0134412463967,9.01783851524058));
#50423=CARTESIAN_POINT('Ctrl Pts',(16.4583500788431,16.9517421301287,8.93633410378674));
#50424=CARTESIAN_POINT('Ctrl Pts',(16.5473485126092,16.8919749501211,8.85220358032272));
#50425=CARTESIAN_POINT('Ctrl Pts',(16.635570684301,16.8342545430765,8.76524563934774));
#50426=CARTESIAN_POINT('Ctrl Pts',(16.6662877415817,16.8141575423401,8.73496875993396));
#50427=CARTESIAN_POINT('Ctrl Pts',(16.6969105331036,16.7943085637301,8.70434886696863));
#50428=CARTESIAN_POINT('Ctrl Pts',(16.7274356688887,16.7747124983035,8.67337717653297));
#50429=CARTESIAN_POINT('Ctrl Pts',(16.7527223169831,16.7584793580493,8.64772060804303));
#50430=CARTESIAN_POINT('Ctrl Pts',(16.7779418190892,16.7424202743778,8.62182205621368));
#50431=CARTESIAN_POINT('Ctrl Pts',(16.8030919759031,16.7265389769528,8.59567542647205));
#50432=CARTESIAN_POINT('Ctrl Pts',(16.8072638582608,16.7239046035358,8.59133825020162));
#50433=CARTESIAN_POINT('Ctrl Pts',(16.8114338076789,16.7212751382847,8.58699427440255));
#50434=CARTESIAN_POINT('Ctrl Pts',(16.8156018425759,16.7186505802289,8.58264344148119));
#50435=CARTESIAN_POINT('Ctrl Pts',(16.8302381928505,16.7094342583963,8.56736518297412));
#50436=CARTESIAN_POINT('Ctrl Pts',(16.8448559912736,16.700275319775,8.55199696169292));
#50437=CARTESIAN_POINT('Ctrl Pts',(16.8594321226321,16.6911886462506,8.53656159353562));
#50438=CARTESIAN_POINT('Ctrl Pts',(16.8683206815264,16.685647571545,8.52714907003764));
#50439=CARTESIAN_POINT('Ctrl Pts',(16.8771946790775,16.6801327697938,8.51771063244034));
#50440=CARTESIAN_POINT('Ctrl Pts',(16.8860542917329,16.6746441928681,8.50824583081303));
#50441=CARTESIAN_POINT('Ctrl Pts',(16.8917136312949,16.6711382020599,8.50219990889979));
#50442=CARTESIAN_POINT('Ctrl Pts',(16.8973670214266,16.6676429512188,8.49614329638282));
#50443=CARTESIAN_POINT('Ctrl Pts',(16.903014440287,16.6641584744563,8.49007595574342));
#50444=CARTESIAN_POINT('Ctrl Pts',(16.9248346863519,16.6506953079649,8.4666332345669));
#50445=CARTESIAN_POINT('Ctrl Pts',(16.9465658296515,16.6373928781379,8.44303043631483));
#50446=CARTESIAN_POINT('Ctrl Pts',(16.9682064917946,16.6242534690107,8.41926515768809));
#50447=CARTESIAN_POINT('Ctrl Pts',(17.0039371670362,16.6025591254048,8.38002654996788));
#50448=CARTESIAN_POINT('Ctrl Pts',(17.0394206154598,16.5813090648392,8.34034481226247));
#50449=CARTESIAN_POINT('Ctrl Pts',(17.074649411893,16.5605132459453,8.30020811244834));
#50450=CARTESIAN_POINT('Ctrl Pts',(17.1310442702686,16.5272229442584,8.23595659860588));
#50451=CARTESIAN_POINT('Ctrl Pts',(17.1867866595652,16.4950965230529,8.17053934117279));
#50452=CARTESIAN_POINT('Ctrl Pts',(17.2418413741485,16.4641860460157,8.10389918362116));
#50453=CARTESIAN_POINT('Ctrl Pts',(17.2572778129006,16.4555192553658,8.08521437672919));
#50454=CARTESIAN_POINT('Ctrl Pts',(17.2726601629871,16.4469481174321,8.06643338374958));
#50455=CARTESIAN_POINT('Ctrl Pts',(17.2879875566528,16.4384739888046,8.04755478218108));
#50456=CARTESIAN_POINT('Ctrl Pts',(17.2999282500352,16.4318722811803,8.03284754638253));
#50457=CARTESIAN_POINT('Ctrl Pts',(17.311836394645,16.4253290073801,8.01808007900446));
#50458=CARTESIAN_POINT('Ctrl Pts',(17.3237108911201,16.4188451997394,8.00325252927566));
#50459=CARTESIAN_POINT('Ctrl Pts',(17.3377275293162,16.4111917227248,7.9857501113569));
#50460=CARTESIAN_POINT('Ctrl Pts',(17.351686709864,16.4036269138078,7.96817708826843));
#50461=CARTESIAN_POINT('Ctrl Pts',(17.365583475195,16.396153869281,7.95053850355612));
#50462=CARTESIAN_POINT('Ctrl Pts',(17.3785269138484,16.3891934802204,7.9341099366402));
#50463=CARTESIAN_POINT('Ctrl Pts',(17.3914178358721,16.3823118167066,7.9176224294128));
#50464=CARTESIAN_POINT('Ctrl Pts',(17.4042530587183,16.375510948613,7.90107890777878));
#50465=CARTESIAN_POINT('Ctrl Pts',(17.4168729288614,16.3688241872509,7.8848129576482));
#50466=CARTESIAN_POINT('Ctrl Pts',(17.4294407899082,16.3622143856895,7.86849077308424));
#50467=CARTESIAN_POINT('Ctrl Pts',(17.441956129715,16.3556822722113,7.85211180631862));
#50468=CARTESIAN_POINT('Ctrl Pts',(17.4924446268172,16.3293308828358,7.78603693908791));
#50469=CARTESIAN_POINT('Ctrl Pts',(17.5420754033658,16.3042456250383,7.71904290139493));
#50470=CARTESIAN_POINT('Ctrl Pts',(17.5908169186686,16.2804753070405,7.65109511034566));
#50471=CARTESIAN_POINT('Ctrl Pts',(17.6314450423743,16.2606617371477,7.59445773985922));
#50472=CARTESIAN_POINT('Ctrl Pts',(17.6714540634022,16.2417617277864,7.53715751102069));
#50473=CARTESIAN_POINT('Ctrl Pts',(17.7108251039144,16.2238041307208,7.47917308598077));
#50474=CARTESIAN_POINT('Ctrl Pts',(17.76592085136,16.198674308908,7.39802980919113));
#50475=CARTESIAN_POINT('Ctrl Pts',(17.8197679834448,16.1753887037899,7.3155473825936));
#50476=CARTESIAN_POINT('Ctrl Pts',(17.8722954333774,16.1540653486999,7.2316474353794));
#50477=CARTESIAN_POINT('Ctrl Pts',(17.9127635566461,16.1376374397992,7.16700935737528));
#50478=CARTESIAN_POINT('Ctrl Pts',(17.9524489416381,16.122374319192,7.10153009056992));
#50479=CARTESIAN_POINT('Ctrl Pts',(17.991316201208,16.1083313302537,7.03517033642935));
#50480=CARTESIAN_POINT('Ctrl Pts',(17.9956991543682,16.1067477413044,7.0276871308384));
#50481=CARTESIAN_POINT('Ctrl Pts',(18.0000716863008,16.1051797034,7.02019271084871));
#50482=CARTESIAN_POINT('Ctrl Pts',(18.0044337337432,16.1036273207594,7.01268700758106));
#50483=CARTESIAN_POINT('Ctrl Pts',(18.0442379656541,16.089461633784,6.94419652061061));
#50484=CARTESIAN_POINT('Ctrl Pts',(18.0831706474733,16.0765994460961,6.87476732283058));
#50485=CARTESIAN_POINT('Ctrl Pts',(18.1211854166012,16.0651213575359,6.80434618427197));
#50486=CARTESIAN_POINT('Ctrl Pts',(18.1242794581716,16.0641871500169,6.79861457166108));
#50487=CARTESIAN_POINT('Ctrl Pts',(18.1273674142371,16.0632621207789,6.79287638315313));
#50488=CARTESIAN_POINT('Ctrl Pts',(18.1304492568663,16.0623463189541,6.78713158711253));
#50489=CARTESIAN_POINT('Ctrl Pts',(18.1378420857906,16.0601494623868,6.77335077496775));
#50490=CARTESIAN_POINT('Ctrl Pts',(18.1452001315689,16.058005590398,6.75953118786803));
#50491=CARTESIAN_POINT('Ctrl Pts',(18.1525217962607,16.0559157320938,6.74567469572302));
#50492=CARTESIAN_POINT('Ctrl Pts',(18.1553382746071,16.0551118110036,6.74034441746996));
#50493=CARTESIAN_POINT('Ctrl Pts',(18.1581498491877,16.0543157555517,6.7350077464228));
#50494=CARTESIAN_POINT('Ctrl Pts',(18.1609559414313,16.0535277526109,6.72966573930445));
#50495=CARTESIAN_POINT('Ctrl Pts',(18.1684739225411,16.0514165635587,6.71535362654485));
#50496=CARTESIAN_POINT('Ctrl Pts',(18.175956429109,16.0493620961228,6.70099578061985));
#50497=CARTESIAN_POINT('Ctrl Pts',(18.1833902087664,16.0473685907007,6.6866164312204));
#50498=CARTESIAN_POINT('Ctrl Pts',(18.1859440579559,16.0466837288349,6.68167645566257));
#50499=CARTESIAN_POINT('Ctrl Pts',(18.1884920381816,16.0460060826363,6.67673419643011));
#50500=CARTESIAN_POINT('Ctrl Pts',(18.1910340109504,16.0453356984825,6.67178991047233));
#50501=CARTESIAN_POINT('Ctrl Pts',(18.2087823458192,16.0406550022149,6.63726835935955));
#50502=CARTESIAN_POINT('Ctrl Pts',(18.2262468855533,16.0363259299848,6.60263043249703));
#50503=CARTESIAN_POINT('Ctrl Pts',(18.2434252739949,16.0323528947381,6.5678751954291));
#50504=CARTESIAN_POINT('Ctrl Pts',(18.2454907744798,16.0318751836736,6.56369628427789));
#50505=CARTESIAN_POINT('Ctrl Pts',(18.2475521447674,16.0314026076911,6.55951567913326));
#50506=CARTESIAN_POINT('Ctrl Pts',(18.2496093793473,16.0309351770026,6.55533337795959));
#50507=CARTESIAN_POINT('Ctrl Pts',(18.287943133361,16.022225245133,6.47740191308712));
#50508=CARTESIAN_POINT('Ctrl Pts',(18.3248397905502,16.0153016529865,6.39888133669614));
#50509=CARTESIAN_POINT('Ctrl Pts',(18.360268028959,16.0102313688368,6.31975807490028));
#50510=CARTESIAN_POINT('Ctrl Pts',(18.3948840682106,16.0052773219231,6.24244872904943));
#50511=CARTESIAN_POINT('Ctrl Pts',(18.4280981536683,16.0020925640988,6.16456420270466));
#50512=CARTESIAN_POINT('Ctrl Pts',(18.4598736351268,16.0007411940976,6.08608943957913));
#50513=CARTESIAN_POINT('Ctrl Pts',(18.4606191860281,16.000709486785,6.08424817934664));
#50514=CARTESIAN_POINT('Ctrl Pts',(18.4613639439046,16.0006787906653,6.08240659389164));
#50515=CARTESIAN_POINT('Ctrl Pts',(18.4621079081254,16.0006491068532,6.08056468297652));
#50516=CARTESIAN_POINT('Ctrl Pts',(18.4941108519774,15.9993722048916,6.00133160974362));
#50517=CARTESIAN_POINT('Ctrl Pts',(18.5246472231963,15.9999683001596,5.92149668907681));
#50518=CARTESIAN_POINT('Ctrl Pts',(18.5536700389979,16.0025274553343,5.84104036577652));
#50519=CARTESIAN_POINT('Ctrl Pts',(18.5540771166406,16.0025633503647,5.83991187532773));
#50520=CARTESIAN_POINT('Ctrl Pts',(18.5544838965089,16.0025996316004,5.83878326262644));
#50521=CARTESIAN_POINT('Ctrl Pts',(18.5548903784453,16.0026362993422,5.83765452761047));
#50522=CARTESIAN_POINT('Ctrl Pts',(18.584011904991,16.0052632810575,5.75678872820492));
#50523=CARTESIAN_POINT('Ctrl Pts',(18.6116044017851,16.0098737819706,5.67529517231536));
#50524=CARTESIAN_POINT('Ctrl Pts',(18.6376092606612,16.0165802278325,5.59314944467261));
#50525=CARTESIAN_POINT('Ctrl Pts',(18.6378461675061,16.0166413242198,5.59240108894217));
#50526=CARTESIAN_POINT('Ctrl Pts',(18.6380829425191,16.016702594683,5.5916526790656));
#50527=CARTESIAN_POINT('Ctrl Pts',(18.6383195856488,16.0167640393203,5.59090421502239));
#50528=CARTESIAN_POINT('Ctrl Pts',(18.6512091581932,16.0201108303726,5.55013657644722));
#50529=CARTESIAN_POINT('Ctrl Pts',(18.6637074866172,16.0239743412651,5.50920822384317));
#50530=CARTESIAN_POINT('Ctrl Pts',(18.6758062333863,16.0283705817719,5.46811568192982));
#50531=CARTESIAN_POINT('Ctrl Pts',(18.6760096423787,16.0284444931339,5.46742481760278));
#50532=CARTESIAN_POINT('Ctrl Pts',(18.6762129384104,16.0285185551061,5.46673390686183));
#50533=CARTESIAN_POINT('Ctrl Pts',(18.6764161214387,16.0285927677704,5.46604294968955));
#50534=CARTESIAN_POINT('Ctrl Pts',(18.6823562788628,16.0307624121175,5.44584247128597));
#50535=CARTESIAN_POINT('Ctrl Pts',(18.6881997052906,16.0330607907699,5.42560283441333));
#50536=CARTESIAN_POINT('Ctrl Pts',(18.6939457824567,16.0354901416101,5.4053220485423));
#50537=CARTESIAN_POINT('Ctrl Pts',(18.6941432017144,16.03557360736,5.40462525704836));
#50538=CARTESIAN_POINT('Ctrl Pts',(18.694340503366,16.0356572270006,5.40392842553738));
#50539=CARTESIAN_POINT('Ctrl Pts',(18.6945376867791,16.0357410002752,5.40323155627735));
#50540=CARTESIAN_POINT('Ctrl Pts',(18.6975058848257,16.037002037733,5.39274159698352));
#50541=CARTESIAN_POINT('Ctrl Pts',(18.7004488043604,16.0382985767024,5.38223761241355));
#50542=CARTESIAN_POINT('Ctrl Pts',(18.7033601450231,16.0396278667465,5.37174224549491));
#50543=CARTESIAN_POINT('Ctrl Pts',(18.7060716230313,16.0408659014319,5.3619673823358));
#50544=CARTESIAN_POINT('Ctrl Pts',(18.70875684925,16.0421328325993,5.35219584814628));
#50545=CARTESIAN_POINT('Ctrl Pts',(18.7114155016037,16.0434285560388,5.34242907537816));
#50546=CARTESIAN_POINT('Ctrl Pts',(18.7116114704868,16.0435240636274,5.3417091679602));
#50547=CARTESIAN_POINT('Ctrl Pts',(18.7118073008575,16.0436197300059,5.34098926593463));
#50548=CARTESIAN_POINT('Ctrl Pts',(18.7120029932956,16.0437155554672,5.3402693672978));
#50549=CARTESIAN_POINT('Ctrl Pts',(18.7345571381285,16.054759729455,5.2572988740171));
#50550=CARTESIAN_POINT('Ctrl Pts',(18.7552130822774,16.0678862964141,5.17460458828852));
#50551=CARTESIAN_POINT('Ctrl Pts',(18.7740029111635,16.0831019318703,5.09219308902043));
#50552=CARTESIAN_POINT('Ctrl Pts',(18.7929175112079,16.098418604567,5.00923434803509));
#50553=CARTESIAN_POINT('Ctrl Pts',(18.809941093651,16.1158521667379,4.92656215336943));
#50554=CARTESIAN_POINT('Ctrl Pts',(18.8250960540203,16.1354245241954,4.8441862432899));
#50555=CARTESIAN_POINT('Ctrl Pts',(18.8253306499371,16.1357275005826,4.84291107980051));
#50556=CARTESIAN_POINT('Ctrl Pts',(18.8255647980929,16.1360309894662,4.84163598730577));
#50557=CARTESIAN_POINT('Ctrl Pts',(18.8257984985327,16.1363349909853,4.84036096585361));
#50558=CARTESIAN_POINT('Ctrl Pts',(18.8406319390535,16.1556305834727,4.75943277040838));
#50559=CARTESIAN_POINT('Ctrl Pts',(18.8536617059308,16.1769914395526,4.67879066555096));
#50560=CARTESIAN_POINT('Ctrl Pts',(18.8648995113531,16.2004534307869,4.59844631570716));
#50561=CARTESIAN_POINT('Ctrl Pts',(18.8651500703535,16.200976541203,4.59665495171533));
#50562=CARTESIAN_POINT('Ctrl Pts',(18.8653997385574,16.2015006960943,4.59486373573569));
#50563=CARTESIAN_POINT('Ctrl Pts',(18.8656485159865,16.202025896035,4.59307266793432));
#50564=CARTESIAN_POINT('Ctrl Pts',(18.8767111630417,16.2253805130466,4.51342737610455));
#50565=CARTESIAN_POINT('Ctrl Pts',(18.8860125020265,16.2508015753402,4.43407509786736));
#50566=CARTESIAN_POINT('Ctrl Pts',(18.8935544873796,16.2783399164094,4.35503007473463));
#50567=CARTESIAN_POINT('Ctrl Pts',(18.8937890310808,16.2791963148427,4.35257190073641));
#50568=CARTESIAN_POINT('Ctrl Pts',(18.8940218733296,16.2800547608349,4.35011402387073));
#50569=CARTESIAN_POINT('Ctrl Pts',(18.8942530138872,16.2809152564325,4.34765644467619));
#50570=CARTESIAN_POINT('Ctrl Pts',(18.901606715701,16.3082917934736,4.26946893501563));
#50571=CARTESIAN_POINT('Ctrl Pts',(18.9072381443165,16.337742838823,4.19158273815674));
#50572=CARTESIAN_POINT('Ctrl Pts',(18.9111396520592,16.3693348180566,4.1140148535215));
#50573=CARTESIAN_POINT('Ctrl Pts',(18.9113041187057,16.3706665665043,4.11074500742583));
#50574=CARTESIAN_POINT('Ctrl Pts',(18.9114655101248,16.3720021214958,4.10747572742533));
#50575=CARTESIAN_POINT('Ctrl Pts',(18.9116238251696,16.3733414890653,4.10420701502236));
#50576=CARTESIAN_POINT('Ctrl Pts',(18.9126022985127,16.3816195113147,4.08400458917904));
#50577=CARTESIAN_POINT('Ctrl Pts',(18.9134632533505,16.3900431716412,4.06382384207223));
#50578=CARTESIAN_POINT('Ctrl Pts',(18.9142064386167,16.3986138967783,4.04366512975419));
#50579=CARTESIAN_POINT('Ctrl Pts',(18.9145780312498,16.4028992593469,4.03358577359519));
#50580=CARTESIAN_POINT('Ctrl Pts',(18.91492018149,16.4072213881557,4.02351192619641));
#50581=CARTESIAN_POINT('Ctrl Pts',(18.9152328520037,16.4115804628294,4.01344363010595));
#50582=CARTESIAN_POINT('Ctrl Pts',(18.9154296528748,16.4143241487711,4.00710644973905));
#50583=CARTESIAN_POINT('Ctrl Pts',(18.9156147704606,16.4170826604257,4.00077103457804));
#50584=CARTESIAN_POINT('Ctrl Pts',(18.9157881985968,16.4198557820706,3.99443799822387));
#50585=CARTESIAN_POINT('Ctrl Pts',(18.9158903071701,16.4214885015411,3.9907093223537));
#50586=CARTESIAN_POINT('Ctrl Pts',(18.9159883080047,16.4231254054345,3.98698348363271));
#50587=CARTESIAN_POINT('Ctrl Pts',(18.9160822139542,16.4247664278847,3.98326061358969));
#50588=CARTESIAN_POINT('Ctrl Pts',(18.9169896933056,16.4406247839996,3.94728389742244));
#50589=CARTESIAN_POINT('Ctrl Pts',(18.9175139091381,16.4568624855893,3.91159614557049));
#50590=CARTESIAN_POINT('Ctrl Pts',(18.9176665865239,16.4734724011024,3.87619494858443));
#50591=CARTESIAN_POINT('Ctrl Pts',(18.917684442095,16.4754149253757,3.8720547899908));
#50592=CARTESIAN_POINT('Ctrl Pts',(18.9176972199449,16.4773625657582,3.86791848680186));
#50593=CARTESIAN_POINT('Ctrl Pts',(18.9177049364349,16.4793153223438,3.86378601729374));
#50594=CARTESIAN_POINT('Ctrl Pts',(18.9178429119191,16.5142317846435,3.78989497687927));
#50595=CARTESIAN_POINT('Ctrl Pts',(18.9163622303388,16.5507758632562,3.71724670105414));
#50596=CARTESIAN_POINT('Ctrl Pts',(18.9133556878514,16.5889052577576,3.64580307217914));
#50597=CARTESIAN_POINT('Ctrl Pts',(18.9131504207254,16.591508484308,3.6409253668292));
#50598=CARTESIAN_POINT('Ctrl Pts',(18.9129380401024,16.5941191010895,3.63605327719103));
#50599=CARTESIAN_POINT('Ctrl Pts',(18.9127185708611,16.5967370991315,3.63118679449738));
#50600=CARTESIAN_POINT('Ctrl Pts',(18.909541534267,16.6346352370783,3.56073959420162));
#50601=CARTESIAN_POINT('Ctrl Pts',(18.9048793505736,16.6740801868338,3.49146721648767));
#50602=CARTESIAN_POINT('Ctrl Pts',(18.8988071542983,16.7150448322063,3.42334340472042));
#50603=CARTESIAN_POINT('Ctrl Pts',(18.8983159692325,16.7183584968378,3.41783281226775));
#50604=CARTESIAN_POINT('Ctrl Pts',(18.8978155569235,16.7216821058912,3.41232973573631));
#50605=CARTESIAN_POINT('Ctrl Pts',(18.8973059507854,16.7250156515976,3.40683416612139));
#50606=CARTESIAN_POINT('Ctrl Pts',(18.8910764557557,16.7657653695806,3.3396555726092));
#50607=CARTESIAN_POINT('Ctrl Pts',(18.8834734392306,16.8079999201565,3.27359867681901));
#50608=CARTESIAN_POINT('Ctrl Pts',(18.874557502219,16.8517052118323,3.20864721855841));
#50609=CARTESIAN_POINT('Ctrl Pts',(18.873727329819,16.8557746581322,3.20259951903838));
#50610=CARTESIAN_POINT('Ctrl Pts',(18.8728857949329,16.8598568293621,3.19656138454947));
#50611=CARTESIAN_POINT('Ctrl Pts',(18.872032934654,16.8639517278831,3.1905328120563));
#50612=CARTESIAN_POINT('Ctrl Pts',(18.8620204726742,16.912025271423,3.11975820293151));
#50613=CARTESIAN_POINT('Ctrl Pts',(18.8504454165462,16.9618529594079,3.0503014032411));
#50614=CARTESIAN_POINT('Ctrl Pts',(18.8373731568207,17.0134386315685,2.98215779784787));
#50615=CARTESIAN_POINT('Ctrl Pts',(18.8256639840523,17.0596452982343,2.92111974739844));
#50616=CARTESIAN_POINT('Ctrl Pts',(18.8127529386748,17.1072623184515,2.86113547100402));
#50617=CARTESIAN_POINT('Ctrl Pts',(18.7986799351308,17.1562927705811,2.80220158006905));
#50618=CARTESIAN_POINT('Ctrl Pts',(18.7970416701605,17.1620004982847,2.79534097431564));
#50619=CARTESIAN_POINT('Ctrl Pts',(18.7953876267584,17.1677274192279,2.78849463178943));
#50620=CARTESIAN_POINT('Ctrl Pts',(18.7937178488403,17.173473563644,2.7816625657979));
#50621=CARTESIAN_POINT('Ctrl Pts',(18.7857111070413,17.2010268653014,2.74890216828991));
#50622=CARTESIAN_POINT('Ctrl Pts',(18.777343128714,17.2290221456169,2.71647005900353));
#50623=CARTESIAN_POINT('Ctrl Pts',(18.768619532796,17.2574626897857,2.68436776726638));
#50624=CARTESIAN_POINT('Ctrl Pts',(18.764257734837,17.2716829618701,2.66831662139781));
#50625=CARTESIAN_POINT('Ctrl Pts',(18.7598051746857,17.2860204098879,2.65234150641107));
#50626=CARTESIAN_POINT('Ctrl Pts',(18.7552687457753,17.3004555867387,2.63646439120962));
#50627=CARTESIAN_POINT('Ctrl Pts',(18.7527806301356,17.3083729133391,2.62775619817379));
#50628=CARTESIAN_POINT('Ctrl Pts',(18.7502684011593,17.3163161197489,2.61908129049594));
#50629=CARTESIAN_POINT('Ctrl Pts',(18.7477317115031,17.3242869956653,2.61043750466746));
#50630=CARTESIAN_POINT('Ctrl Pts',(18.7456434102184,17.3308489297889,2.6033216050123));
#50631=CARTESIAN_POINT('Ctrl Pts',(18.743537844844,17.3374316642756,2.59622471924828));
#50632=CARTESIAN_POINT('Ctrl Pts',(18.7414166468313,17.344030582907,2.5891515796704));
#50633=CARTESIAN_POINT('Ctrl Pts',(18.738865117639,17.3519682357925,2.58064349979919));
#50634=CARTESIAN_POINT('Ctrl Pts',(18.7362901984525,17.3599316998598,2.57216721755547));
#50635=CARTESIAN_POINT('Ctrl Pts',(18.7336951875099,17.3679113629952,2.56373281991339));
#50636=CARTESIAN_POINT('Ctrl Pts',(18.7289379676969,17.3825398221459,2.54827073344745));
#50637=CARTESIAN_POINT('Ctrl Pts',(18.724110082699,17.3972328178983,2.53293818335603));
#50638=CARTESIAN_POINT('Ctrl Pts',(18.7192130608308,17.4119905493229,2.51773232191264));
#50639=CARTESIAN_POINT('Ctrl Pts',(18.7094086698816,17.4415371946729,2.48728846964402));
#50640=CARTESIAN_POINT('Ctrl Pts',(18.6993272580374,17.4713432420696,2.45735228351929));
#50641=CARTESIAN_POINT('Ctrl Pts',(18.6889796594319,17.501411375434,2.42790290780628));
#50642=CARTESIAN_POINT('Ctrl Pts',(18.6865516176034,17.5084667984646,2.42099267493209));
#50643=CARTESIAN_POINT('Ctrl Pts',(18.6841089777729,17.515536610181,2.41410916805059));
#50644=CARTESIAN_POINT('Ctrl Pts',(18.6816518430478,17.5226208725668,2.40725216818588));
#50645=CARTESIAN_POINT('Ctrl Pts',(18.6606398054745,17.5832015098058,2.3486149525189));
#50646=CARTESIAN_POINT('Ctrl Pts',(18.6385732142793,17.6448185426341,2.29193550295218));
#50647=CARTESIAN_POINT('Ctrl Pts',(18.6155445047684,17.7074495954823,2.23713374068759));
#50648=CARTESIAN_POINT('Ctrl Pts',(18.5952360125508,17.7626824885256,2.18880531994261));
#50649=CARTESIAN_POINT('Ctrl Pts',(18.5741783699363,17.8187036782295,2.14193759021419));
#50650=CARTESIAN_POINT('Ctrl Pts',(18.5524266721411,17.8754960551877,2.09647914071758));
#50651=CARTESIAN_POINT('Ctrl Pts',(18.5495131449393,17.8831030997816,2.09039021697443));
#50652=CARTESIAN_POINT('Ctrl Pts',(18.5465871498316,17.8907239868604,2.08432659257798));
#50653=CARTESIAN_POINT('Ctrl Pts',(18.5436487795668,17.8983587060738,2.07828820069466));
#50654=CARTESIAN_POINT('Ctrl Pts',(18.5187732391351,17.9629924143411,2.02716861810383));
#50655=CARTESIAN_POINT('Ctrl Pts',(18.493012338885,18.0286179750865,1.97785685211132));
#50656=CARTESIAN_POINT('Ctrl Pts',(18.4664312545691,18.0952307061165,1.93031234669157));
#50657=CARTESIAN_POINT('Ctrl Pts',(18.4428122010353,18.1544205285307,1.88806590537245));
#50658=CARTESIAN_POINT('Ctrl Pts',(18.41854323848,18.2143895483544,1.8472150191826));
#50659=CARTESIAN_POINT('Ctrl Pts',(18.3936671179681,18.2751336625744,1.8077328993508));
#50660=CARTESIAN_POINT('Ctrl Pts',(18.3625516420487,18.3511134369268,1.75834799030573));
#50661=CARTESIAN_POINT('Ctrl Pts',(18.3304856337078,18.4283059298595,1.7111048659539));
#50662=CARTESIAN_POINT('Ctrl Pts',(18.2975275019964,18.5067263915645,1.66599177173665));
#50663=CARTESIAN_POINT('Ctrl Pts',(18.2707759860673,18.5703788536896,1.629374293867));
#50664=CARTESIAN_POINT('Ctrl Pts',(18.2434352523388,18.6348454890174,1.59415750987106));
#50665=CARTESIAN_POINT('Ctrl Pts',(18.2155405293451,18.700118449349,1.56034406141925));
#50666=CARTESIAN_POINT('Ctrl Pts',(18.2125143152344,18.7071997153523,1.55667574268882));
#50667=CARTESIAN_POINT('Ctrl Pts',(18.2094813141992,18.7142910609668,1.55302370505177));
#50668=CARTESIAN_POINT('Ctrl Pts',(18.2064417088042,18.7213921460605,1.54938813161792));
#50669=CARTESIAN_POINT('Ctrl Pts',(18.198677267509,18.7395313290066,1.54010133519732));
#50670=CARTESIAN_POINT('Ctrl Pts',(18.1908700725115,18.7577334941773,1.53092223109942));
#50671=CARTESIAN_POINT('Ctrl Pts',(18.1830206415079,18.7759989510875,1.52185095427166));
#50672=CARTESIAN_POINT('Ctrl Pts',(18.1781063167304,18.7874344790161,1.51617166357434));
#50673=CARTESIAN_POINT('Ctrl Pts',(18.1731754349275,18.7988948155038,1.51053465364943));
#50674=CARTESIAN_POINT('Ctrl Pts',(18.1682293461457,18.8103771802602,1.5049413900067));
#50675=CARTESIAN_POINT('Ctrl Pts',(18.1652752687015,18.8172350827825,1.50160078398545));
#50676=CARTESIAN_POINT('Ctrl Pts',(18.1623177029271,18.8240963542693,1.49827795144323));
#50677=CARTESIAN_POINT('Ctrl Pts',(18.1593568281399,18.8309606733165,1.49497297744696));
#50678=CARTESIAN_POINT('Ctrl Pts',(18.1463365332697,18.8611461639232,1.48043952397064));
#50679=CARTESIAN_POINT('Ctrl Pts',(18.1332465050168,18.8914039864737,1.46624494618778));
#50680=CARTESIAN_POINT('Ctrl Pts',(18.1200901414679,18.9217340445751,1.45238407310797));
#50681=CARTESIAN_POINT('Ctrl Pts',(18.1172443145164,18.9282946793938,1.44938585509466));
#50682=CARTESIAN_POINT('Ctrl Pts',(18.1143953877743,18.934858692716,1.4464032417234));
#50683=CARTESIAN_POINT('Ctrl Pts',(18.1115433909991,18.9414260850989,1.44343619124119));
#50684=CARTESIAN_POINT('Ctrl Pts',(18.082026041729,19.0093967141136,1.41272806907662));
#50685=CARTESIAN_POINT('Ctrl Pts',(18.0521796023943,19.0777294006106,1.38368689482883));
#50686=CARTESIAN_POINT('Ctrl Pts',(18.0220380007022,19.1464249078126,1.35626665519777));
#50687=CARTESIAN_POINT('Ctrl Pts',(17.9866754333215,19.227019480291,1.32409682953767));
#50688=CARTESIAN_POINT('Ctrl Pts',(17.9509084798126,19.3081127623388,1.29415358338591));
#50689=CARTESIAN_POINT('Ctrl Pts',(17.9147779185929,19.3897109870291,1.26639573762749));
#50690=CARTESIAN_POINT('Ctrl Pts',(17.8833654764719,19.4606536855018,1.2422626576571));
#50691=CARTESIAN_POINT('Ctrl Pts',(17.8516776321339,19.531977766523,1.21978161321308));
#50692=CARTESIAN_POINT('Ctrl Pts',(17.8197410752445,19.6036866097686,1.19892627464732));
#50693=CARTESIAN_POINT('Ctrl Pts',(17.7836341935295,19.6847593042972,1.17534761382524));
#50694=CARTESIAN_POINT('Ctrl Pts',(17.7472091082188,19.7663238553438,1.15384744917031));
#50695=CARTESIAN_POINT('Ctrl Pts',(17.7104897656853,19.8483907356608,1.13442371693699));
#50696=CARTESIAN_POINT('Ctrl Pts',(17.6773925085894,19.9223623388952,1.11691598898944));
#50697=CARTESIAN_POINT('Ctrl Pts',(17.6440561966807,19.9967417246677,1.10109534075644));
#50698=CARTESIAN_POINT('Ctrl Pts',(17.6104984919182,20.0715363698375,1.0869606873673));
#50699=CARTESIAN_POINT('Ctrl Pts',(17.5738959008892,20.1531175693769,1.0715435144408));
#50700=CARTESIAN_POINT('Ctrl Pts',(17.5370292830112,20.2351941866344,1.05813195497465));
#50701=CARTESIAN_POINT('Ctrl Pts',(17.4999100362541,20.317778319276,1.04675761316854));
#50702=CARTESIAN_POINT('Origin',(6.61363325216158E-15,53.,-24.));
#50703=CARTESIAN_POINT('',(4.1991313379145,53.,-27.5520833333334));
#50704=CARTESIAN_POINT('',(-4.19913133791448,53.,-27.5520833333334));
#50705=CARTESIAN_POINT('Origin',(6.61363325216158E-15,53.,-24.));
#50706=CARTESIAN_POINT('',(3.43565291283914,52.,-26.90625));
#50707=CARTESIAN_POINT('Origin',(3.43565291283914,53.,-26.90625));
#50708=CARTESIAN_POINT('',(-3.43565291283912,52.,-26.90625));
#50709=CARTESIAN_POINT('Origin',(6.61363325216158E-15,52.,-24.));
#50710=CARTESIAN_POINT('Origin',(-3.43565291283912,53.,-26.90625));
#50711=CARTESIAN_POINT('Origin',(5.2045770037451E-16,8.5,0.));
#50712=CARTESIAN_POINT('',(-1.83698839911727E-15,9.00000000000001,19.5));
#50713=CARTESIAN_POINT('Origin',(-1.86760355796283E-15,8.50000000000001,
19.5));
#50714=CARTESIAN_POINT('Origin',(5.51072859220069E-16,9.,-1.70652395450943E-16));
#50715=CARTESIAN_POINT('Ctrl Pts',(-14.1696709084508,34.2228423347593,-8.45401835497186));
#50716=CARTESIAN_POINT('Ctrl Pts',(-14.4598881528388,34.2800112558736,-7.96758898230353));
#50717=CARTESIAN_POINT('Ctrl Pts',(-15.0284388422964,34.3091931864527,-7.97011831445158));
#50718=CARTESIAN_POINT('Ctrl Pts',(-14.1687509928547,34.2417094783908,-8.45556021361394));
#50719=CARTESIAN_POINT('Ctrl Pts',(-14.4590195349379,34.2974823791094,-7.96916514970434));
#50720=CARTESIAN_POINT('Ctrl Pts',(-15.027463174257,34.3259639809838,-7.97157191635228));
#50721=CARTESIAN_POINT('Ctrl Pts',(-14.1678668544491,34.2605265108349,-8.45704153677041));
#50722=CARTESIAN_POINT('Ctrl Pts',(-14.4581845937863,34.3149090256939,-7.97067959720386));
#50723=CARTESIAN_POINT('Ctrl Pts',(-15.0265254516828,34.3426902318517,-7.97296845218914));
#50724=CARTESIAN_POINT('Ctrl Pts',(-14.1661635328208,34.2981938523499,-8.45989441550156));
#50725=CARTESIAN_POINT('Ctrl Pts',(-14.4565759909218,34.3497943960948,-7.97359633424001));
#50726=CARTESIAN_POINT('Ctrl Pts',(-15.024718898452,34.3761723132014,-7.97565803480127));
#50727=CARTESIAN_POINT('Ctrl Pts',(-14.1653454356421,34.3170219168472,-8.46126415076535));
#50728=CARTESIAN_POINT('Ctrl Pts',(-14.4558033400937,34.3672326811367,-7.97499678944735));
#50729=CARTESIAN_POINT('Ctrl Pts',(-15.0238512196152,34.3929083705295,-7.97694936773952));
#50730=CARTESIAN_POINT('Ctrl Pts',(-14.1629917065432,34.373489337447,-8.46520379440197));
#50731=CARTESIAN_POINT('Ctrl Pts',(-14.4535804037852,34.41953098386,-7.97902465759217));
#50732=CARTESIAN_POINT('Ctrl Pts',(-15.0213548402835,34.4431016332889,-7.98066350984471));
#50733=CARTESIAN_POINT('Ctrl Pts',(-14.1615566384215,34.4111119211253,-8.4676041477937));
#50734=CARTESIAN_POINT('Ctrl Pts',(-14.4522248265318,34.454380888302,-7.98147914140516));
#50735=CARTESIAN_POINT('Ctrl Pts',(-15.0198327983173,34.4765439298872,-7.98292646932796));
#50736=CARTESIAN_POINT('Ctrl Pts',(-14.1576526183944,34.5239129308506,-8.47413110853782));
#50737=CARTESIAN_POINT('Ctrl Pts',(-14.4485372614658,34.5588642949711,-7.98815276719896));
#50738=CARTESIAN_POINT('Ctrl Pts',(-15.0156921710414,34.5768114940933,-7.98907983290995));
#50739=CARTESIAN_POINT('Ctrl Pts',(-14.1555848703909,34.5990246231075,-8.47758373051289));
#50740=CARTESIAN_POINT('Ctrl Pts',(-14.446583355318,34.6284571865908,-7.99168420593832));
#50741=CARTESIAN_POINT('Ctrl Pts',(-15.0134991049499,34.6435774427604,-7.99233483016131));
#50742=CARTESIAN_POINT('Ctrl Pts',(-14.1509771790097,34.8240952679178,-8.4852743386372));
#50743=CARTESIAN_POINT('Ctrl Pts',(-14.4422301623517,34.8369697425827,-7.99954874151129));
#50744=CARTESIAN_POINT('Ctrl Pts',(-15.008612159576,34.8436402381527,-7.99958523498254));
#50745=CARTESIAN_POINT('Ctrl Pts',(-14.1500330992177,34.9737899010413,-8.48684678418226));
#50746=CARTESIAN_POINT('Ctrl Pts',(-14.4413373565372,34.9757252603891,-8.00115815623579));
#50747=CARTESIAN_POINT('Ctrl Pts',(-15.0076108628144,34.9767021342601,-8.00106767539272));
#50748=CARTESIAN_POINT('Ctrl Pts',(-14.1534989333457,35.4218322689878,-8.48106645017854));
#50749=CARTESIAN_POINT('Ctrl Pts',(-14.4446127086534,35.3909181528281,-7.99524560707017));
#50750=CARTESIAN_POINT('Ctrl Pts',(-15.0112867474724,35.3749620168757,-7.99561820204977));
#50751=CARTESIAN_POINT('Ctrl Pts',(-14.1642118082204,35.7191401530233,-8.46324178895702));
#50752=CARTESIAN_POINT('Ctrl Pts',(-14.454761563286,35.6666794668494,-7.97697017454646));
#50753=CARTESIAN_POINT('Ctrl Pts',(-15.0226488876287,35.6392356915726,-7.97881380780291));
#50754=CARTESIAN_POINT('Ctrl Pts',(-14.2018700963651,36.3110245203784,-8.3998954453284));
#50755=CARTESIAN_POINT('Ctrl Pts',(-14.4903036805241,36.2145680745722,-7.91223236340415));
#50756=CARTESIAN_POINT('Ctrl Pts',(-15.0625894960227,36.1653551292289,-7.91909334909917));
#50757=CARTESIAN_POINT('Ctrl Pts',(-14.2288151924285,36.6056011119585,-8.35437505244428));
#50758=CARTESIAN_POINT('Ctrl Pts',(-14.5157733460828,36.4872920363756,-7.86562765440656));
#50759=CARTESIAN_POINT('Ctrl Pts',(-15.0911676285592,36.4272009883655,-7.87617850054425));
#50760=CARTESIAN_POINT('Ctrl Pts',(-14.2678515285549,36.9354562627635,-8.28724846986359));
#50761=CARTESIAN_POINT('Ctrl Pts',(-14.5524221273012,36.7911880341194,-7.7973135407053));
#50762=CARTESIAN_POINT('Ctrl Pts',(-15.1325698029845,36.7204055669061,-7.81289418035236));
#50763=CARTESIAN_POINT('Ctrl Pts',(-14.272310834891,36.9720923458365,-8.27956682548256));
#50764=CARTESIAN_POINT('Ctrl Pts',(-14.5566164314028,36.8250040101967,-7.78948085637131));
#50765=CARTESIAN_POINT('Ctrl Pts',(-15.1372993703662,36.7529709740877,-7.80565222610578));
#50766=CARTESIAN_POINT('Ctrl Pts',(-14.2814663750741,37.0452925529125,-8.26376437000761));
#50767=CARTESIAN_POINT('Ctrl Pts',(-14.5652251137911,36.8925526698609,-7.77337133120969));
#50768=CARTESIAN_POINT('Ctrl Pts',(-15.1470097917179,36.8180378248002,-7.79075428816105));
#50769=CARTESIAN_POINT('Ctrl Pts',(-14.2861536017617,37.081785083136,-8.25565910563603));
#50770=CARTESIAN_POINT('Ctrl Pts',(-14.5696312954759,36.9262202981498,-7.76510980926654));
#50771=CARTESIAN_POINT('Ctrl Pts',(-15.1519810928061,36.850475629465,-7.78311296160134));
#50772=CARTESIAN_POINT('Ctrl Pts',(-14.3005366026303,37.1909436147287,-8.23073635121615));
#50773=CARTESIAN_POINT('Ctrl Pts',(-14.5831518360579,37.0269359064794,-7.7397041366779));
#50774=CARTESIAN_POINT('Ctrl Pts',(-15.1672357906114,36.9475054352928,-7.7596167619714));
#50775=CARTESIAN_POINT('Ctrl Pts',(-14.3105536680637,37.263290615546,-8.21331202705747));
#50776=CARTESIAN_POINT('Ctrl Pts',(-14.5925608990619,37.0936355928615,-7.7219524972774));
#50777=CARTESIAN_POINT('Ctrl Pts',(-15.1778599510383,37.0118138805059,-7.74318978992613));
#50778=CARTESIAN_POINT('Ctrl Pts',(-14.3418348010998,37.4790826477386,-8.15864801908498));
#50779=CARTESIAN_POINT('Ctrl Pts',(-14.6219410641221,37.2926085843646,-7.66625367882849));
#50780=CARTESIAN_POINT('Ctrl Pts',(-15.211036910134,37.2036290201708,-7.69165469791198));
#50781=CARTESIAN_POINT('Ctrl Pts',(-14.3643283878283,37.6212795682079,-8.11901917638115));
#50782=CARTESIAN_POINT('Ctrl Pts',(-14.6430362895773,37.4235089284438,-7.62591654935295));
#50783=CARTESIAN_POINT('Ctrl Pts',(-15.2348937448071,37.3300262828855,-7.65429417319524));
#50784=CARTESIAN_POINT('Ctrl Pts',(-14.4363019502445,38.0430610597211,-7.9907944336361));
#50785=CARTESIAN_POINT('Ctrl Pts',(-14.7105067497658,37.8118623201918,-7.49538846499181));
#50786=CARTESIAN_POINT('Ctrl Pts',(-15.3112293408869,37.7049431641283,-7.53340889331172));
#50787=CARTESIAN_POINT('Ctrl Pts',(-14.49026980554,38.3178484315225,-7.8928871878268));
#50788=CARTESIAN_POINT('Ctrl Pts',(-14.7609541970719,38.0639420611781,-7.39588717756517));
#50789=CARTESIAN_POINT('Ctrl Pts',(-15.3684679759171,37.9491986058153,-7.44110576650622));
#50790=CARTESIAN_POINT('Ctrl Pts',(-14.6080482783172,38.8552917835711,-7.67271221247472));
#50791=CARTESIAN_POINT('Ctrl Pts',(-14.8703740139742,38.5549584396854,-7.17322618837634));
#50792=CARTESIAN_POINT('Ctrl Pts',(-15.4933845372648,38.4269260298234,-7.2335333987612));
#50793=CARTESIAN_POINT('Ctrl Pts',(-14.6718611162741,39.1179471327802,-7.55044413842592));
#50794=CARTESIAN_POINT('Ctrl Pts',(-14.9295100780991,38.794189655202,-7.04967693049274));
#50795=CARTESIAN_POINT('Ctrl Pts',(-15.5610648206959,38.6603974512983,-7.11826383427611));
#50796=CARTESIAN_POINT('Ctrl Pts',(-14.7480666188548,39.4067715675604,-7.3989787087425));
#50797=CARTESIAN_POINT('Ctrl Pts',(-14.999316825149,39.0547855952716,-6.89817098281311));
#50798=CARTESIAN_POINT('Ctrl Pts',(-15.6418888381287,38.9171302822837,-6.97546814291349));
#50799=CARTESIAN_POINT('Ctrl Pts',(-14.7565941785648,39.4387656880567,-7.38195749962283));
#50800=CARTESIAN_POINT('Ctrl Pts',(-15.0071581686653,39.0837656036217,-6.88107637534832));
#50801=CARTESIAN_POINT('Ctrl Pts',(-15.6509332197322,38.9455695005142,-6.95942121181813));
#50802=CARTESIAN_POINT('Ctrl Pts',(-14.7737256022962,39.502412269052,-7.34761186407861));
#50803=CARTESIAN_POINT('Ctrl Pts',(-15.0228997481459,39.1413825527381,-6.84659981861948));
#50804=CARTESIAN_POINT('Ctrl Pts',(-15.6691029114839,39.002144239138,-6.92704148796774));
#50805=CARTESIAN_POINT('Ctrl Pts',(-14.7823346424693,39.5340844533758,-7.33027717344031));
#50806=CARTESIAN_POINT('Ctrl Pts',(-15.0308049908594,39.1700375342947,-6.82920681792526));
#50807=CARTESIAN_POINT('Ctrl Pts',(-15.6782337117527,39.0302972919077,-6.91069901878126));
#50808=CARTESIAN_POINT('Ctrl Pts',(-14.808284656594,39.6286524867301,-7.27779013265149));
#50809=CARTESIAN_POINT('Ctrl Pts',(-15.0546319241823,39.2556023565078,-6.77653515305077));
#50810=CARTESIAN_POINT('Ctrl Pts',(-15.7057564538778,39.1143577659461,-6.8612162865755));
#50811=CARTESIAN_POINT('Ctrl Pts',(-14.8257484822497,39.6910999140348,-7.24215491242092));
#50812=CARTESIAN_POINT('Ctrl Pts',(-15.0706345822693,39.31199951062,-6.74082930478049));
#50813=CARTESIAN_POINT('Ctrl Pts',(-15.7242786933826,39.1698665902847,-6.8276207929431));
#50814=CARTESIAN_POINT('Ctrl Pts',(-14.8785762907581,39.876683136037,-7.1333351875412));
#50815=CARTESIAN_POINT('Ctrl Pts',(-15.1190327204018,39.4796219387076,-6.63176677641015));
#50816=CARTESIAN_POINT('Ctrl Pts',(-15.7803081869927,39.3348294541919,-6.72502980625943));
#50817=CARTESIAN_POINT('Ctrl Pts',(-14.9143760584171,39.9980613049761,-7.05823809590922));
#50818=CARTESIAN_POINT('Ctrl Pts',(-15.1516954791241,39.5888243403568,-6.5567294842393));
#50819=CARTESIAN_POINT('Ctrl Pts',(-15.8182776378986,39.4427211600206,-6.65423120166715));
#50820=CARTESIAN_POINT('Ctrl Pts',(-15.0231004266237,40.3553871225062,-6.82537958602282));
#50821=CARTESIAN_POINT('Ctrl Pts',(-15.2508296348633,39.9103610239103,-6.3239951350709));
#50822=CARTESIAN_POINT('Ctrl Pts',(-15.9335913612037,39.7603441088107,-6.43470129294701));
#50823=CARTESIAN_POINT('Ctrl Pts',(-15.0973449297501,40.5845463158894,-6.66007288714214));
#50824=CARTESIAN_POINT('Ctrl Pts',(-15.31792988494,40.114768031037,-6.15976330372408));
#50825=CARTESIAN_POINT('Ctrl Pts',(-16.0123355319573,39.9640411696614,-6.2788565940716));
#50826=CARTESIAN_POINT('Ctrl Pts',(-15.2472968949109,41.0254173108877,-6.30922595793956));
#50827=CARTESIAN_POINT('Ctrl Pts',(-15.4523126364001,40.5055857309467,-5.81354666702777));
#50828=CARTESIAN_POINT('Ctrl Pts',(-16.1713754941982,40.3559264985848,-5.94809181206602));
#50829=CARTESIAN_POINT('Ctrl Pts',(-15.3230087426575,41.2371284648137,-6.12368686448347));
#50830=CARTESIAN_POINT('Ctrl Pts',(-15.5196455447178,40.6918988399555,-5.63122192702778));
#50831=CARTESIAN_POINT('Ctrl Pts',(-16.2516759396333,40.5441141908017,-5.77317280154761));
#50832=CARTESIAN_POINT('Ctrl Pts',(-15.4173521697931,41.4908768942127,-5.87860618526534));
#50833=CARTESIAN_POINT('Ctrl Pts',(-15.6023498902727,40.9125245108878,-5.39340306565551));
#50834=CARTESIAN_POINT('Ctrl Pts',(-16.3517371496677,40.7696683504473,-5.54212030933746));
#50835=CARTESIAN_POINT('Ctrl Pts',(-15.4362061333438,41.541080480963,-5.82893036895881));
#50836=CARTESIAN_POINT('Ctrl Pts',(-15.6189216498825,40.9563040712589,-5.34503370394812));
#50837=CARTESIAN_POINT('Ctrl Pts',(-16.3717337779055,40.814293760811,-5.49528788992432));
#50838=CARTESIAN_POINT('Ctrl Pts',(-15.4644422759024,41.6155621820111,-5.75341180123559));
#50839=CARTESIAN_POINT('Ctrl Pts',(-15.6436600403385,41.0210733659742,-5.27169025022555));
#50840=CARTESIAN_POINT('Ctrl Pts',(-16.4016812016563,40.8804997173657,-5.42409193382638));
#50841=CARTESIAN_POINT('Ctrl Pts',(-15.4738394697509,41.6402325166288,-5.72809098740203));
#50842=CARTESIAN_POINT('Ctrl Pts',(-15.6518901269291,41.042522534143,-5.24709833812979));
#50843=CARTESIAN_POINT('Ctrl Pts',(-16.4116479225022,40.9024289036886,-5.40022045953334));
#50844=CARTESIAN_POINT('Ctrl Pts',(-15.4925703942472,41.689181898316,-5.67723496738244));
#50845=CARTESIAN_POINT('Ctrl Pts',(-15.6682749940766,41.0850380021743,-5.1977485436834));
#50846=CARTESIAN_POINT('Ctrl Pts',(-16.4315140544655,40.9459394651512,-5.35227539009512));
#50847=CARTESIAN_POINT('Ctrl Pts',(-15.5019086640392,41.7134729307954,-5.65168764188966));
#50848=CARTESIAN_POINT('Ctrl Pts',(-15.6764336314637,41.1061140969787,-5.17297859437461));
#50849=CARTESIAN_POINT('Ctrl Pts',(-16.4414182800811,40.967531494057,-5.32819036948575));
#50850=CARTESIAN_POINT('Ctrl Pts',(-15.5484555651202,41.8340156143712,-5.52335553940722));
#50851=CARTESIAN_POINT('Ctrl Pts',(-15.7171539857794,41.2108612547213,-5.04834447526745));
#50852=CARTESIAN_POINT('Ctrl Pts',(-16.4907862052723,41.074680546041,-5.20720387542547));
#50853=CARTESIAN_POINT('Ctrl Pts',(-15.5852305114518,41.9275319640208,-5.41878553611691));
#50854=CARTESIAN_POINT('Ctrl Pts',(-15.7490791740827,41.2915492195499,-4.94737813664718));
#50855=CARTESIAN_POINT('Ctrl Pts',(-16.5297899365528,41.1578061902771,-5.10861936072794));
#50856=CARTESIAN_POINT('Ctrl Pts',(-15.6938508583456,42.199498468939,-5.0993756835597));
#50857=CARTESIAN_POINT('Ctrl Pts',(-15.8432282443095,41.526068650345,-4.63908945210971));
#50858=CARTESIAN_POINT('Ctrl Pts',(-16.64499333428,41.3995541945398,-4.80749222676696));
#50859=CARTESIAN_POINT('Ctrl Pts',(-15.7639910093299,42.369390564411,-4.87885064391805));
#50860=CARTESIAN_POINT('Ctrl Pts',(-15.9031097774975,41.6705184443034,-4.42842552480797));
#50861=CARTESIAN_POINT('Ctrl Pts',(-16.7193844041967,41.5505693905269,-4.59958983270443));
#50862=CARTESIAN_POINT('Ctrl Pts',(-15.8980969848804,42.6866289429011,-4.42234195955402));
#50863=CARTESIAN_POINT('Ctrl Pts',(-16.0164770439618,41.938203868012,-3.99591210397994));
#50864=CARTESIAN_POINT('Ctrl Pts',(-16.8616180139052,41.8325590604172,-4.16921127494601));
#50865=CARTESIAN_POINT('Ctrl Pts',(-15.9620670091645,42.8339757168234,-4.18635981457349));
#50866=CARTESIAN_POINT('Ctrl Pts',(-16.069837618137,42.061051465547,-3.77409145591909));
#50867=CARTESIAN_POINT('Ctrl Pts',(-16.9294650101271,41.9635339702937,-3.94673652549938));
#50868=CARTESIAN_POINT('Ctrl Pts',(-16.0521582726785,43.037709823846,-3.82021108244197));
#50869=CARTESIAN_POINT('Ctrl Pts',(-16.1440256404094,42.2291011383052,-3.43385778245536));
#50870=CARTESIAN_POINT('Ctrl Pts',(-17.0250163496069,42.1446309546378,-3.60154580164102));
#50871=CARTESIAN_POINT('Ctrl Pts',(-16.0812108244472,43.102733976819,-3.69612831892062));
#50872=CARTESIAN_POINT('Ctrl Pts',(-16.1678670548505,42.2825951618778,-3.31868636626619));
#50873=CARTESIAN_POINT('Ctrl Pts',(-17.0558296625103,42.2024302014641,-3.48456541848317));
#50874=CARTESIAN_POINT('Ctrl Pts',(-16.1231583043917,43.1958323041313,-3.50684228674254));
#50875=CARTESIAN_POINT('Ctrl Pts',(-16.2020593980967,42.358743766398,-3.14397959827399));
#50876=CARTESIAN_POINT('Ctrl Pts',(-17.1003194136399,42.2851842704153,-3.30611394037726));
#50877=CARTESIAN_POINT('Ctrl Pts',(-16.1368688153599,43.2261249913638,-3.44321966940264));
#50878=CARTESIAN_POINT('Ctrl Pts',(-16.2132166154573,42.3834909358494,-3.0852944650872));
#50879=CARTESIAN_POINT('Ctrl Pts',(-17.1148608648885,42.3121111033463,-3.24613302164169));
#50880=CARTESIAN_POINT('Ctrl Pts',(-16.1570050576291,43.2704363362883,-3.3469780073553));
#50881=CARTESIAN_POINT('Ctrl Pts',(-16.2295461487012,42.4195814461551,-2.99676810231204));
#50882=CARTESIAN_POINT('Ctrl Pts',(-17.1362174853078,42.3514989656337,-3.15540014162311));
#50883=CARTESIAN_POINT('Ctrl Pts',(-16.1636460804533,43.2850199841448,-3.31476016326283));
#50884=CARTESIAN_POINT('Ctrl Pts',(-16.234927397343,42.4314525764685,-2.96714277235139));
#50885=CARTESIAN_POINT('Ctrl Pts',(-17.1432609944394,42.3644622081519,-3.12502641655731));
#50886=CARTESIAN_POINT('Ctrl Pts',(-16.176779066406,43.3138032530051,-3.25006285951472));
#50887=CARTESIAN_POINT('Ctrl Pts',(-16.2455540938229,42.4548543838694,-2.90771276300664));
#50888=CARTESIAN_POINT('Ctrl Pts',(-17.1571899188963,42.3900473359813,-3.0640323254552));
#50889=CARTESIAN_POINT('Ctrl Pts',(-16.1832563592051,43.3279707317643,-3.21765573302902));
#50890=CARTESIAN_POINT('Ctrl Pts',(-16.2507873073283,42.4663580683418,-2.87797525515983));
#50891=CARTESIAN_POINT('Ctrl Pts',(-17.164059774934,42.4026406504781,-3.03348015236247));
#50892=CARTESIAN_POINT('Ctrl Pts',(-16.2407423662139,43.4534701977211,-2.92546660438112));
#50893=CARTESIAN_POINT('Ctrl Pts',(-16.2973926330638,42.5686355463496,-2.60882804918763));
#50894=CARTESIAN_POINT('Ctrl Pts',(-17.2250297821921,42.5141957311396,-2.75801565386698));
#50895=CARTESIAN_POINT('Ctrl Pts',(-16.2860851710674,43.5507845829967,-2.66201787685001));
#50896=CARTESIAN_POINT('Ctrl Pts',(-16.3334056853608,42.6464652770683,-2.36955567429105));
#50897=CARTESIAN_POINT('Ctrl Pts',(-17.27312063616,42.6006974071258,-2.50964648325415));
#50898=CARTESIAN_POINT('Ctrl Pts',(-16.3644674413509,43.7174968151427,-2.12770174998652));
#50899=CARTESIAN_POINT('Ctrl Pts',(-16.395286619085,42.7792030237934,-1.88723589636282));
#50900=CARTESIAN_POINT('Ctrl Pts',(-17.3562533467079,42.7488860578871,-2.00591410770285));
#50901=CARTESIAN_POINT('Ctrl Pts',(-16.3975090775376,43.7868935216046,-1.85683435243505));
#50902=CARTESIAN_POINT('Ctrl Pts',(-16.4209906605381,42.8337387768024,-1.64478289056291));
#50903=CARTESIAN_POINT('Ctrl Pts',(-17.3912975066884,42.810572019061,-1.75055090464328));
#50904=CARTESIAN_POINT('Ctrl Pts',(-16.4371973244655,43.8698191922474,-1.44484551307843));
#50905=CARTESIAN_POINT('Ctrl Pts',(-16.4517290374466,42.8986843931254,-1.27807359738039));
#50906=CARTESIAN_POINT('Ctrl Pts',(-17.4333911016012,42.8842837265137,-1.36214391805839));
#50907=CARTESIAN_POINT('Ctrl Pts',(-16.4487802554229,43.8939261909356,-1.30656641831514));
#50908=CARTESIAN_POINT('Ctrl Pts',(-16.4606689802262,42.9175109064172,-1.15517368833686));
#50909=CARTESIAN_POINT('Ctrl Pts',(-17.4456760285918,42.9057121696064,-1.23177978830181));
#50910=CARTESIAN_POINT('Ctrl Pts',(-16.4685324538335,43.9349488754536,-1.02806931366241));
#50911=CARTESIAN_POINT('Ctrl Pts',(-16.4758894976883,42.9495081386978,-0.908068000066032));
#50912=CARTESIAN_POINT('Ctrl Pts',(-17.4666253297105,42.9421767782951,-0.969223595380726));
#50913=CARTESIAN_POINT('Ctrl Pts',(-16.4767018066094,43.9518647448791,-0.887851353093695));
#50914=CARTESIAN_POINT('Ctrl Pts',(-16.4821582142198,42.9626536650404,-0.783956213361243));
#50915=CARTESIAN_POINT('Ctrl Pts',(-17.4752897950108,42.9572131064008,-0.837031578665104));
#50916=CARTESIAN_POINT('Ctrl Pts',(-16.4862967209135,43.9717089312722,-0.676029616417883));
#50917=CARTESIAN_POINT('Ctrl Pts',(-16.4895137451409,42.9780633749711,-0.596718279805704));
#50918=CARTESIAN_POINT('Ctrl Pts',(-17.4854662190897,42.9748523834323,-0.637334318512984));
#50919=CARTESIAN_POINT('Ctrl Pts',(-16.4890517437789,43.977401569991,-0.605173122314613));
#50920=CARTESIAN_POINT('Ctrl Pts',(-16.4916238230334,42.9824805634447,-0.534110465633991));
#50921=CARTESIAN_POINT('Ctrl Pts',(-17.4883882131625,42.9799125065679,-0.57053358332299));
#50922=CARTESIAN_POINT('Ctrl Pts',(-16.492506023628,43.9845357058383,-0.498508314718125));
#50923=CARTESIAN_POINT('Ctrl Pts',(-16.4942681869357,42.9880140786458,-0.439912398698345));
#50924=CARTESIAN_POINT('Ctrl Pts',(-17.49205184321,42.9862539607906,-0.469974168759785));
#50925=CARTESIAN_POINT('Ctrl Pts',(-16.4935448911152,43.9866805929804,-0.462870708599939));
#50926=CARTESIAN_POINT('Ctrl Pts',(-16.4950632373273,42.9896773373646,-0.408444310922235));
#50927=CARTESIAN_POINT('Ctrl Pts',(-17.4931536723775,42.9881605271315,-0.436376425617608));
#50928=CARTESIAN_POINT('Ctrl Pts',(-16.495392016117,43.9904934577505,-0.391554086603203));
#50929=CARTESIAN_POINT('Ctrl Pts',(-16.4964765826267,42.9926335814917,-0.345482344139571));
#50930=CARTESIAN_POINT('Ctrl Pts',(-17.4951127443838,42.9915497401849,-0.36914189982643));
#50931=CARTESIAN_POINT('Ctrl Pts',(-16.4961991039929,43.9921590221803,-0.355925418204801));
#50932=CARTESIAN_POINT('Ctrl Pts',(-16.4970939068081,42.9939245371181,-0.314034598998794));
#50933=CARTESIAN_POINT('Ctrl Pts',(-17.4959687466422,42.9930302419732,-0.335552582820379));
#50934=CARTESIAN_POINT('Ctrl Pts',(-16.4996553193878,43.9992904788907,-0.177929344977772));
#50935=CARTESIAN_POINT('Ctrl Pts',(-16.499737824245,42.9994528692837,-0.156906377895304));
#50936=CARTESIAN_POINT('Ctrl Pts',(-17.4996344297213,42.9993693144289,-0.167744837011927));
#50937=CARTESIAN_POINT('Ctrl Pts',(-16.5005671676994,44.0011697501096,-0.0360034841747721));
#50938=CARTESIAN_POINT('Ctrl Pts',(-16.5004336035839,43.0009063138008,-0.0317784680747621));
#50939=CARTESIAN_POINT('Ctrl Pts',(-17.5006015414388,43.0010397779723,-0.0339426786824198));
#50940=CARTESIAN_POINT('Ctrl Pts',(-16.4978545553025,43.9955752404001,0.388390909530019));
#50941=CARTESIAN_POINT('Ctrl Pts',(-16.4983604076717,42.9965730007167,0.34258128637437));
#50942=CARTESIAN_POINT('Ctrl Pts',(-17.4977245284721,42.9960668801614,0.366159780026568));
#50943=CARTESIAN_POINT('Ctrl Pts',(-16.488785846129,43.9768969118701,0.669479171266392));
#50944=CARTESIAN_POINT('Ctrl Pts',(-16.4914621272788,42.9821709666193,0.590248849637306));
#50945=CARTESIAN_POINT('Ctrl Pts',(-17.488106200346,42.9794639216913,0.631158814660471));
#50946=CARTESIAN_POINT('Ctrl Pts',(-16.4566137829713,43.9102406346531,1.22805693613211));
#50947=CARTESIAN_POINT('Ctrl Pts',(-16.4667388442969,42.9303002753056,1.08490481084554));
#50948=CARTESIAN_POINT('Ctrl Pts',(-17.4539843153664,42.9202138974404,1.15776411487348));
#50949=CARTESIAN_POINT('Ctrl Pts',(-16.4335093295897,43.8622622073091,1.50554633472257));
#50950=CARTESIAN_POINT('Ctrl Pts',(-16.4489907660971,42.8929980278654,1.33109833842561));
#50951=CARTESIAN_POINT('Ctrl Pts',(-17.4294795919199,42.8775664063642,1.41937028185803));
#50952=CARTESIAN_POINT('Ctrl Pts',(-16.3960891495453,43.783793740335,1.85015317363005));
#50953=CARTESIAN_POINT('Ctrl Pts',(-16.4197798825902,42.8310926576272,1.63991769895437));
#50954=CARTESIAN_POINT('Ctrl Pts',(-17.3897915222624,42.8078166581088,1.74425215023244));
#50955=CARTESIAN_POINT('Ctrl Pts',(-16.3881779026531,43.767173088473,1.91896157031875));
#50956=CARTESIAN_POINT('Ctrl Pts',(-16.4136093423201,42.817995097094,1.70150596722071));
#50957=CARTESIAN_POINT('Ctrl Pts',(-17.3814008058283,42.7930427452666,1.80912201914365));
#50958=CARTESIAN_POINT('Ctrl Pts',(-16.375673948842,43.740841555206,2.0220039170481));
#50959=CARTESIAN_POINT('Ctrl Pts',(-16.4038270264028,42.7971893690875,1.79393530076847));
#50960=CARTESIAN_POINT('Ctrl Pts',(-17.3681390366586,42.7696369379822,1.90626631910862));
#50961=CARTESIAN_POINT('Ctrl Pts',(-16.3713997812811,43.7318309227685,2.05632298830878));
#50962=CARTESIAN_POINT('Ctrl Pts',(-16.4004812785263,42.7900667948439,1.82472882562818));
#50963=CARTESIAN_POINT('Ctrl Pts',(-17.3636058286238,42.7616274868815,1.93862099907206));
#50964=CARTESIAN_POINT('Ctrl Pts',(-16.3626396751579,43.7133407089755,2.12490420765856));
#50965=CARTESIAN_POINT('Ctrl Pts',(-16.3936154941633,42.7754354074154,1.88631707234903));
#50966=CARTESIAN_POINT('Ctrl Pts',(-17.3543148069932,42.7451917413354,2.0032766940958));
#50967=CARTESIAN_POINT('Ctrl Pts',(-16.3581504674953,43.7038542075336,2.15919050412873));
#50968=CARTESIAN_POINT('Ctrl Pts',(-16.3900932136698,42.7679218136654,1.9171321516777));
#50969=CARTESIAN_POINT('Ctrl Pts',(-17.3495535260841,42.7367592956301,2.03560047527918));
#50970=CARTESIAN_POINT('Ctrl Pts',(-16.335218649852,43.6553329579177,2.33016678950607));
#50971=CARTESIAN_POINT('Ctrl Pts',(-16.3721055730023,42.7295090646878,2.07069458061821));
#50972=CARTESIAN_POINT('Ctrl Pts',(-17.3252319015473,42.6936292957481,2.19679023923976));
#50973=CARTESIAN_POINT('Ctrl Pts',(-16.315354751774,43.6131097667714,2.46525055695651));
#50974=CARTESIAN_POINT('Ctrl Pts',(-16.3564409704719,42.6959272836267,2.19259820200646));
#50975=CARTESIAN_POINT('Ctrl Pts',(-17.3041641304931,42.6560975705951,2.32414193923568));
#50976=CARTESIAN_POINT('Ctrl Pts',(-16.2515056057596,43.4765147512805,2.8655905997197));
#50977=CARTESIAN_POINT('Ctrl Pts',(-16.3058885440615,42.5869423044208,2.55446830067613));
#50978=CARTESIAN_POINT('Ctrl Pts',(-17.2364453397946,42.5346797786526,2.7015668953238));
#50979=CARTESIAN_POINT('Ctrl Pts',(-16.2032672081898,43.3722448995847,3.12594764367366));
#50980=CARTESIAN_POINT('Ctrl Pts',(-16.2673330709852,42.5030995032564,2.7919929023725));
#50981=CARTESIAN_POINT('Ctrl Pts',(-17.1852834023163,42.441995466392,2.94702134755456));
#50982=CARTESIAN_POINT('Ctrl Pts',(-16.0968875664402,43.1381380127393,3.63422998231717));
#50983=CARTESIAN_POINT('Ctrl Pts',(-16.1809970935074,42.3122776252218,3.25988799511517));
#50984=CARTESIAN_POINT('Ctrl Pts',(-17.07245651017,42.2339004556738,3.42621008435598));
#50985=CARTESIAN_POINT('Ctrl Pts',(-16.0387426559475,43.0082992884229,3.88215383492437));
#50986=CARTESIAN_POINT('Ctrl Pts',(-16.1333904856796,42.2057238967836,3.48991370242924));
#50987=CARTESIAN_POINT('Ctrl Pts',(-17.0107876651219,42.118488256322,3.65994300926234));
#50988=CARTESIAN_POINT('Ctrl Pts',(-15.9607089630699,42.8300074294681,4.18445557032663));
#50989=CARTESIAN_POINT('Ctrl Pts',(-16.0682434684036,42.0567601433772,3.77421115204722));
#50990=CARTESIAN_POINT('Ctrl Pts',(-16.9280246578707,41.9600066039851,3.94494127844591));
#50991=CARTESIAN_POINT('Ctrl Pts',(-15.9448345125254,42.7935473084438,4.2445349020985));
#50992=CARTESIAN_POINT('Ctrl Pts',(-16.0550169591108,42.026372413421,3.83055888715714));
#50993=CARTESIAN_POINT('Ctrl Pts',(-16.9111881192775,41.9275976074833,4.00158172585483));
#50994=CARTESIAN_POINT('Ctrl Pts',(-15.9125710995365,42.7190148602521,4.3639323057479));
#50995=CARTESIAN_POINT('Ctrl Pts',(-16.0280522148975,41.964087720814,3.94277369967183));
#50996=CARTESIAN_POINT('Ctrl Pts',(-16.8769693480609,41.8613465424687,4.1141449347411));
#50997=CARTESIAN_POINT('Ctrl Pts',(-15.8961777996028,42.6809324048149,4.42326572017825));
#50998=CARTESIAN_POINT('Ctrl Pts',(-16.0143130159987,41.9321895117794,3.99865250806258));
#50999=CARTESIAN_POINT('Ctrl Pts',(-16.8595825146128,41.8274954710167,4.17008216045151));
#51000=CARTESIAN_POINT('Ctrl Pts',(-15.8462844618934,42.5643109368609,4.60002845907672));
#51001=CARTESIAN_POINT('Ctrl Pts',(-15.9724388258778,41.8344100525786,4.16519179553658));
#51002=CARTESIAN_POINT('Ctrl Pts',(-16.8066653386068,41.723831943736,4.33672716677812));
#51003=CARTESIAN_POINT('Ctrl Pts',(-15.8122905956358,42.4839122053499,4.71544824060082));
#51004=CARTESIAN_POINT('Ctrl Pts',(-15.9437057928047,41.7665897154923,4.27457431431909));
#51005=CARTESIAN_POINT('Ctrl Pts',(-16.7706112375754,41.652366404853,4.44554042885686));
#51006=CARTESIAN_POINT('Ctrl Pts',(-15.708466257085,42.2349319229732,5.05470392926197));
#51007=CARTESIAN_POINT('Ctrl Pts',(-15.8557182823553,41.5561640523473,4.59624091151791));
#51008=CARTESIAN_POINT('Ctrl Pts',(-16.6604945155305,41.4310505980033,4.76537744171326));
#51009=CARTESIAN_POINT('Ctrl Pts',(-15.6367937805477,42.0585895493903,5.27155542705688));
#51010=CARTESIAN_POINT('Ctrl Pts',(-15.7941524221352,41.4054489545328,4.80429063353521));
#51011=CARTESIAN_POINT('Ctrl Pts',(-16.5844782517039,41.274301821729,4.96981656414753));
#51012=CARTESIAN_POINT('Ctrl Pts',(-15.490346672854,41.6855007303992,5.68751055477781));
#51013=CARTESIAN_POINT('Ctrl Pts',(-15.6669541386688,41.0833353282907,5.20593767654318));
#51014=CARTESIAN_POINT('Ctrl Pts',(-16.42915556251,40.9426673158617,5.36196281266631));
#51015=CARTESIAN_POINT('Ctrl Pts',(-15.4155675047962,41.4887542028889,5.88661251495239));
#51016=CARTESIAN_POINT('Ctrl Pts',(-15.6013785695094,40.9122288799408,5.39970005563699));
#51017=CARTESIAN_POINT('Ctrl Pts',(-16.3498443229104,40.7677815136044,5.54966836406231));
#51018=CARTESIAN_POINT('Ctrl Pts',(-15.3024448812762,41.1779991716065,6.17216839972268));
#51019=CARTESIAN_POINT('Ctrl Pts',(-15.5009241601739,40.6387285873814,5.6799934650858));
#51020=CARTESIAN_POINT('Ctrl Pts',(-16.2298657833509,40.4915548192431,5.81887929950314));
#51021=CARTESIAN_POINT('Ctrl Pts',(-15.2645790020526,41.0718024829547,6.26516634094168));
#51022=CARTESIAN_POINT('Ctrl Pts',(-15.4672614165944,40.5452444380058,5.77127906622756));
#51023=CARTESIAN_POINT('Ctrl Pts',(-16.1897050020046,40.3971577625623,5.90655412600363));
#51024=CARTESIAN_POINT('Ctrl Pts',(-15.2077254227751,40.9084929741541,6.4013676517502));
#51025=CARTESIAN_POINT('Ctrl Pts',(-15.4164278105277,40.4007199180155,5.90553521152224));
#51026=CARTESIAN_POINT('Ctrl Pts',(-16.1294057515143,40.2519937548357,6.03495940239176));
#51027=CARTESIAN_POINT('Ctrl Pts',(-15.1887651989012,40.853386989109,6.44621852703614));
#51028=CARTESIAN_POINT('Ctrl Pts',(-15.3994674120309,40.3519488749432,5.94974031533987));
#51029=CARTESIAN_POINT('Ctrl Pts',(-16.1092964229923,40.2030106569473,6.07724305571356));
#51030=CARTESIAN_POINT('Ctrl Pts',(-15.1508585131677,40.7418148130405,6.53481506085914));
#51031=CARTESIAN_POINT('Ctrl Pts',(-15.365491794666,40.2530328359572,6.03717495128596));
#51032=CARTESIAN_POINT('Ctrl Pts',(-16.0690923625353,40.1038353894078,6.16076840762205));
#51033=CARTESIAN_POINT('Ctrl Pts',(-15.1319787469483,40.685544542223,6.57840481672826));
#51034=CARTESIAN_POINT('Ctrl Pts',(-15.348535637605,40.2030632212813,6.08025593853515));
#51035=CARTESIAN_POINT('Ctrl Pts',(-16.0490683678638,40.0538173708934,6.20186312687394));
#51036=CARTESIAN_POINT('Ctrl Pts',(-15.0380664911524,40.4019030685421,6.79276143414887));
#51037=CARTESIAN_POINT('Ctrl Pts',(-15.2644245680603,39.9519367964584,6.29138993605124));
#51038=CARTESIAN_POINT('Ctrl Pts',(-15.9494644607597,39.8016916163679,6.40395017364007));
#51039=CARTESIAN_POINT('Ctrl Pts',(-14.9644461532019,40.1675514041411,6.95288768593992));
#51040=CARTESIAN_POINT('Ctrl Pts',(-15.1976171693671,39.7421821058477,6.45092268656129));
#51041=CARTESIAN_POINT('Ctrl Pts',(-15.8713822833035,39.5933790259089,6.55491094954876));
#51042=CARTESIAN_POINT('Ctrl Pts',(-14.8222211698946,39.6838140960417,7.25114166432459));
#51043=CARTESIAN_POINT('Ctrl Pts',(-15.06786594057,39.3068953284827,6.74885869506734));
#51044=CARTESIAN_POINT('Ctrl Pts',(-15.7205376048291,39.1633903075869,6.83609315171071));
#51045=CARTESIAN_POINT('Ctrl Pts',(-14.7536128479239,39.4344290298586,7.38926853498414));
#51046=CARTESIAN_POINT('Ctrl Pts',(-15.0048054725226,39.0812939904251,6.88766092280371));
#51047=CARTESIAN_POINT('Ctrl Pts',(-15.6477712019922,38.9417146931311,6.96631377005003));
#51048=CARTESIAN_POINT('Ctrl Pts',(-14.6235443336384,38.9199395169773,7.64345031191053));
#51049=CARTESIAN_POINT('Ctrl Pts',(-14.8848011659622,38.6139543580119,7.14351801279062));
#51050=CARTESIAN_POINT('Ctrl Pts',(-15.5098197481496,38.4843906818341,7.20594642230858));
#51051=CARTESIAN_POINT('Ctrl Pts',(-14.5620800221653,38.6548384656211,7.7595087284317));
#51052=CARTESIAN_POINT('Ctrl Pts',(-14.827716689627,38.3720620877045,7.26095612384862));
#51053=CARTESIAN_POINT('Ctrl Pts',(-15.4446303262328,38.2487453026412,7.31536176370244));
#51054=CARTESIAN_POINT('Ctrl Pts',(-14.4912109590877,38.3128451067789,7.89022745753408));
#51055=CARTESIAN_POINT('Ctrl Pts',(-14.7615399553527,38.0581196581985,7.39373762359809));
#51056=CARTESIAN_POINT('Ctrl Pts',(-15.369466168806,37.944751206059,7.43859827658201));
#51057=CARTESIAN_POINT('Ctrl Pts',(-14.4773360216078,38.2439139811986,7.91565127929397));
#51058=CARTESIAN_POINT('Ctrl Pts',(-14.7486090785329,37.9949822886081,7.41950389459761));
#51059=CARTESIAN_POINT('Ctrl Pts',(-15.3547503258741,37.883479094363,7.46256686250324));
#51060=CARTESIAN_POINT('Ctrl Pts',(-14.4570026893877,38.1396985883734,7.95268958299778));
#51061=CARTESIAN_POINT('Ctrl Pts',(-14.7296347176249,37.8994093453111,7.45707777466083));
#51062=CARTESIAN_POINT('Ctrl Pts',(-15.3331846705994,37.7908431896831,7.49748512881753));
#51063=CARTESIAN_POINT('Ctrl Pts',(-14.4502995623675,38.1047958815478,7.9648621653037));
#51064=CARTESIAN_POINT('Ctrl Pts',(-14.7233795289916,37.8674039475413,7.46942463090051));
#51065=CARTESIAN_POINT('Ctrl Pts',(-15.326075293378,37.7598185613842,7.50896096392519));
#51066=CARTESIAN_POINT('Ctrl Pts',(-14.4370862536553,38.0348626145466,7.98878759631039));
#51067=CARTESIAN_POINT('Ctrl Pts',(-14.711044089513,37.8032526976823,7.49369902639856));
#51068=CARTESIAN_POINT('Ctrl Pts',(-15.3120611781612,37.6976556573663,7.531516925812));
#51069=CARTESIAN_POINT('Ctrl Pts',(-14.430578191227,37.9998443555349,8.00053668324475));
#51070=CARTESIAN_POINT('Ctrl Pts',(-14.7049654891278,37.7711173950731,7.50562346769514));
#51071=CARTESIAN_POINT('Ctrl Pts',(-15.3051586876244,37.6665283160382,7.54259350608998));
#51072=CARTESIAN_POINT('Ctrl Pts',(-14.3985378950991,37.8244951111472,8.05821896776018));
#51073=CARTESIAN_POINT('Ctrl Pts',(-14.6750683621745,37.6103672676509,7.56410181532715));
#51074=CARTESIAN_POINT('Ctrl Pts',(-15.2711765555705,37.5106623209909,7.59697411101706));
#51075=CARTESIAN_POINT('Ctrl Pts',(-14.3745058364078,37.6833906877742,8.10096493484399));
#51076=CARTESIAN_POINT('Ctrl Pts',(-14.652561930448,37.4806229720141,7.60757184213281));
#51077=CARTESIAN_POINT('Ctrl Pts',(-15.2456880081703,37.3852361669233,7.63727333921995));
#51078=CARTESIAN_POINT('Ctrl Pts',(-14.3074780704631,37.2575991659697,8.21914076587046));
#51079=CARTESIAN_POINT('Ctrl Pts',(-14.5898331467566,37.0893377713944,7.72760627073598));
#51080=CARTESIAN_POINT('Ctrl Pts',(-15.1745979538034,37.0067548141695,7.74868489717074));
#51081=CARTESIAN_POINT('Ctrl Pts',(-14.2695523034726,36.9704386282229,8.28453464061196));
#51082=CARTESIAN_POINT('Ctrl Pts',(-14.5540974775854,36.8241663199945,7.79441727640368));
#51083=CARTESIAN_POINT('Ctrl Pts',(-15.1343736550051,36.7515010028509,7.81033568794618));
#51084=CARTESIAN_POINT('Ctrl Pts',(-14.2086105787285,36.3893814021093,8.38862459376293));
#51085=CARTESIAN_POINT('Ctrl Pts',(-14.4967075641971,36.2872858361014,7.90063819784113));
#51086=CARTESIAN_POINT('Ctrl Pts',(-15.069738492784,36.2350056907777,7.90846763065641));
#51087=CARTESIAN_POINT('Ctrl Pts',(-14.1855946049829,36.0954849072401,8.42732167623407));
#51088=CARTESIAN_POINT('Ctrl Pts',(-14.474938277723,36.0150460990806,7.94027178393654));
#51089=CARTESIAN_POINT('Ctrl Pts',(-15.04532761125,35.9737643619689,7.94494972814297));
#51090=CARTESIAN_POINT('Ctrl Pts',(-14.1632592796937,35.6493675288365,8.46476803043535));
#51091=CARTESIAN_POINT('Ctrl Pts',(-14.4538374531707,35.601719694416,7.97857185535198));
#51092=CARTESIAN_POINT('Ctrl Pts',(-15.0216386300259,35.5772155811991,7.98025268877251));
#51093=CARTESIAN_POINT('Ctrl Pts',(-14.1578452220156,35.4997817266829,8.47381023741147));
#51094=CARTESIAN_POINT('Ctrl Pts',(-14.4487195544893,35.4631107873063,7.98782407910831));
#51095=CARTESIAN_POINT('Ctrl Pts',(-15.0158964475708,35.4442504237115,7.98877732802181));
#51096=CARTESIAN_POINT('Ctrl Pts',(-14.1528931524912,35.2740434072532,8.48207673460457));
#51097=CARTESIAN_POINT('Ctrl Pts',(-14.4440400975708,35.2539384493497,7.99627922136717));
#51098=CARTESIAN_POINT('Ctrl Pts',(-15.0106442526529,35.2435941397839,7.99657065897525));
#51099=CARTESIAN_POINT('Ctrl Pts',(-14.1517706094402,35.1985706100121,8.48394895723216));
#51100=CARTESIAN_POINT('Ctrl Pts',(-14.442979184077,35.184001549869,7.9981943881281));
#51101=CARTESIAN_POINT('Ctrl Pts',(-15.0094536766753,35.1765072088985,7.99833571715932));
#51102=CARTESIAN_POINT('Ctrl Pts',(-14.1508941306251,35.0850155880073,8.4854107517919));
#51103=CARTESIAN_POINT('Ctrl Pts',(-14.4421509241428,35.078778187705,7.99968953263258));
#51104=CARTESIAN_POINT('Ctrl Pts',(-15.0085240779375,35.0755694115626,7.99971384012147));
#51105=CARTESIAN_POINT('Ctrl Pts',(-14.150736560916,35.0470814239072,8.48567350216556));
#51106=CARTESIAN_POINT('Ctrl Pts',(-14.4420020169164,35.0436268600821,7.99995828626213));
#51107=CARTESIAN_POINT('Ctrl Pts',(-15.0083569585472,35.0418501545842,7.99996155087807));
#51108=CARTESIAN_POINT('Ctrl Pts',(-14.150692918513,34.9712377388823,8.48574627995365));
#51109=CARTESIAN_POINT('Ctrl Pts',(-14.4419607755292,34.9733482312172,8.0000327238654));
#51110=CARTESIAN_POINT('Ctrl Pts',(-15.0083106711502,34.9744335456731,8.00003016290435));
#51111=CARTESIAN_POINT('Ctrl Pts',(-14.1508066226917,34.9333329107061,8.48555667952094));
#51112=CARTESIAN_POINT('Ctrl Pts',(-14.4420682290436,34.9382240120611,7.99983879114063));
#51113=CARTESIAN_POINT('Ctrl Pts',(-15.0084312664928,34.940740365072,7.99985141504979));
#51114=CARTESIAN_POINT('Ctrl Pts',(-14.1520509011363,34.7438936238919,8.48348153993902));
#51115=CARTESIAN_POINT('Ctrl Pts',(-14.4432440959225,34.7626780463408,7.99771623713472));
#51116=CARTESIAN_POINT('Ctrl Pts',(-15.0097509557443,34.7723498879043,7.9978950544351));
#51117=CARTESIAN_POINT('Ctrl Pts',(-14.1552091806869,34.5926136214512,8.4782167591127));
#51118=CARTESIAN_POINT('Ctrl Pts',(-14.4462304856527,34.6224662811345,7.99232810421143));
#51119=CARTESIAN_POINT('Ctrl Pts',(-15.0131006462177,34.6378787746227,7.99293162477818));
#51120=CARTESIAN_POINT('Ctrl Pts',(-14.1631498026642,34.366097861864,8.46494029855902));
#51121=CARTESIAN_POINT('Ctrl Pts',(-14.4537301008296,34.4126736274608,7.97875461899514));
#51122=CARTESIAN_POINT('Ctrl Pts',(-15.0215225179599,34.4365314327682,7.98041509627186));
#51123=CARTESIAN_POINT('Ctrl Pts',(-14.1663304572642,34.2906600038508,8.45961782992988));
#51124=CARTESIAN_POINT('Ctrl Pts',(-14.4567347009781,34.34279668575,7.97331176954809));
#51125=CARTESIAN_POINT('Ctrl Pts',(-15.0248959395469,34.3694755589792,7.975397280748));
#51126=CARTESIAN_POINT('Ctrl Pts',(-14.1718962020967,34.1776041375939,8.45028822882502));
#51127=CARTESIAN_POINT('Ctrl Pts',(-14.4619896761171,34.2381138641883,7.96377525778024));
#51128=CARTESIAN_POINT('Ctrl Pts',(-15.0307990022117,34.2689814556387,7.96660169720576));
#51129=CARTESIAN_POINT('Ctrl Pts',(-14.1738839055404,34.1399356702887,8.44695401845093));
#51130=CARTESIAN_POINT('Ctrl Pts',(-14.4638665061005,34.2032333257984,7.96036678089891));
#51131=CARTESIAN_POINT('Ctrl Pts',(-15.0329071725568,34.2354983735906,7.96345833389448));
#51132=CARTESIAN_POINT('Ctrl Pts',(-14.1781231744824,34.0646323657967,8.43983651540518));
#51133=CARTESIAN_POINT('Ctrl Pts',(-14.4678686428001,34.1335117477056,7.95309163191476));
#51134=CARTESIAN_POINT('Ctrl Pts',(-15.0374033668614,34.1685621029298,7.95674823001028));
#51135=CARTESIAN_POINT('Ctrl Pts',(-14.1803761277451,34.026976116557,8.43605088762219));
#51136=CARTESIAN_POINT('Ctrl Pts',(-14.4699954006696,34.0986496666099,7.9492223146372));
#51137=CARTESIAN_POINT('Ctrl Pts',(-15.039792862775,34.1350898813783,7.953179288052));
#51138=CARTESIAN_POINT('Ctrl Pts',(-14.2018025764259,33.6887269670264,8.40001146214908));
#51139=CARTESIAN_POINT('Ctrl Pts',(-14.4902406725494,33.7851897713294,7.91234974711415));
#51140=CARTESIAN_POINT('Ctrl Pts',(-15.062517883968,33.8344239707358,7.91920272479425));
#51141=CARTESIAN_POINT('Ctrl Pts',(-14.2289622534947,33.3934618841932,8.35411823426493));
#51142=CARTESIAN_POINT('Ctrl Pts',(-14.5159096719755,33.5118586162235,7.86536934014895));
#51143=CARTESIAN_POINT('Ctrl Pts',(-15.091323602403,33.5719661192377,7.87593638279283));
#51144=CARTESIAN_POINT('Ctrl Pts',(-14.297587136116,32.8129757621643,8.2361192541527));
#51145=CARTESIAN_POINT('Ctrl Pts',(-14.5804718486074,32.975939942154,7.74503244923851));
#51146=CARTESIAN_POINT('Ctrl Pts',(-15.1641075683963,33.0559784553022,7.76469155241571));
#51147=CARTESIAN_POINT('Ctrl Pts',(-14.3390533631708,32.5277562904371,8.16400873147055));
#51148=CARTESIAN_POINT('Ctrl Pts',(-14.6194905451471,32.7128565901746,7.67142630106037));
#51149=CARTESIAN_POINT('Ctrl Pts',(-15.2080869006233,32.8024500359307,7.6967085685757));
#51150=CARTESIAN_POINT('Ctrl Pts',(-14.4344512245411,31.9668958072417,7.99412958149491));
#51151=CARTESIAN_POINT('Ctrl Pts',(-14.7087759143519,32.1972833069676,7.49877760542043));
#51152=CARTESIAN_POINT('Ctrl Pts',(-15.3092664499803,32.3039073842282,7.53655314061732));
#51153=CARTESIAN_POINT('Ctrl Pts',(-14.4883838105694,31.691255013237,7.89636074701349));
#51154=CARTESIAN_POINT('Ctrl Pts',(-14.7592010426945,31.9443746233512,7.39939956315832));
#51155=CARTESIAN_POINT('Ctrl Pts',(-15.3664676782412,32.0588933451493,7.44438050229219));
#51156=CARTESIAN_POINT('Ctrl Pts',(-14.5550635668316,31.3864313723232,7.77176756628671));
#51157=CARTESIAN_POINT('Ctrl Pts',(-14.8209199446041,31.6669143175934,7.27386759669347));
#51158=CARTESIAN_POINT('Ctrl Pts',(-15.4371886314425,31.7879389976144,7.32691891770422));
#51159=CARTESIAN_POINT('Ctrl Pts',(-14.5625558613898,31.352635473547,7.75772049298618));
#51160=CARTESIAN_POINT('Ctrl Pts',(-14.827877420134,31.6360499048315,7.25966604997201));
#51161=CARTESIAN_POINT('Ctrl Pts',(-15.4451350045509,31.7578981987159,7.31367588564878));
#51162=CARTESIAN_POINT('Ctrl Pts',(-14.5777038502899,31.2851903557158,7.72921800162461));
#51163=CARTESIAN_POINT('Ctrl Pts',(-14.8419359589025,31.5744837961381,7.2308617271771));
#51164=CARTESIAN_POINT('Ctrl Pts',(-15.4612010532912,31.697946982851,7.28680485001122));
#51165=CARTESIAN_POINT('Ctrl Pts',(-14.5853648004003,31.2515184553974,7.71475260653216));
#51166=CARTESIAN_POINT('Ctrl Pts',(-14.849042235293,31.543760796002,7.21624805914054));
#51167=CARTESIAN_POINT('Ctrl Pts',(-15.469326303495,31.6680164047788,7.2731674405612));
#51168=CARTESIAN_POINT('Ctrl Pts',(-14.6085452032034,31.1509057610832,7.67082157327148));
#51169=CARTESIAN_POINT('Ctrl Pts',(-14.8705436711721,31.4519516854403,7.171859977806));
#51170=CARTESIAN_POINT('Ctrl Pts',(-15.4939115790748,31.5785828987784,7.2317509780494));
#51171=CARTESIAN_POINT('Ctrl Pts',(-14.6242529880176,31.0844047949656,7.64083891095088));
#51172=CARTESIAN_POINT('Ctrl Pts',(-14.8850903709531,31.3913603681064,7.14160216923058));
#51173=CARTESIAN_POINT('Ctrl Pts',(-15.5105713510105,31.5194709288242,7.20348449527989));
#51174=CARTESIAN_POINT('Ctrl Pts',(-14.6720790763943,30.8865851637151,7.54883265535859));
#51175=CARTESIAN_POINT('Ctrl Pts',(-14.929376159556,31.2110903439192,7.04872760978158));
#51176=CARTESIAN_POINT('Ctrl Pts',(-15.5612959899498,31.3436312567038,7.11674459069576));
#51177=CARTESIAN_POINT('Ctrl Pts',(-14.7048994575313,30.7569483641181,7.48475247389081));
#51178=CARTESIAN_POINT('Ctrl Pts',(-14.95966877612,31.0933259986506,6.98419535501427));
#51179=CARTESIAN_POINT('Ctrl Pts',(-15.5961054854356,31.2283985458312,7.05633229878906));
#51180=CARTESIAN_POINT('Ctrl Pts',(-14.8057173802565,30.3745068040017,7.28444119078806));
#51181=CARTESIAN_POINT('Ctrl Pts',(-15.052677543726,30.7458140689667,6.78241054451384));
#51182=CARTESIAN_POINT('Ctrl Pts',(-15.7030335847703,30.888450492549,6.86748664417107));
#51183=CARTESIAN_POINT('Ctrl Pts',(-14.8760647694745,30.1281517423914,7.14016324914458));
#51184=CARTESIAN_POINT('Ctrl Pts',(-15.1171363078512,30.5235314070459,6.63773030177344));
#51185=CARTESIAN_POINT('Ctrl Pts',(-15.7776444528623,30.6694682154397,6.73146703642075));
#51186=CARTESIAN_POINT('Ctrl Pts',(-15.0208334639485,29.6517703450343,6.83035843117765));
#51187=CARTESIAN_POINT('Ctrl Pts',(-15.2487759421767,30.0960400709944,6.32894683063836));
#51188=CARTESIAN_POINT('Ctrl Pts',(-15.9311870068286,30.2460180844943,6.43939515378203));
#51189=CARTESIAN_POINT('Ctrl Pts',(-15.0952589444123,29.4217455787918,6.66483128140236));
#51190=CARTESIAN_POINT('Ctrl Pts',(-15.3160581108554,29.8908120505933,6.16445964685839));
#51191=CARTESIAN_POINT('Ctrl Pts',(-16.0101231232976,30.0415516256819,6.28334262225704));
#51192=CARTESIAN_POINT('Ctrl Pts',(-15.1895776666482,29.1442442832826,6.4443022486447));
#51193=CARTESIAN_POINT('Ctrl Pts',(-15.4001942830716,29.6459545222953,5.94785171931794));
#51194=CARTESIAN_POINT('Ctrl Pts',(-16.1101581311846,29.79488380734,6.07543646335386));
#51195=CARTESIAN_POINT('Ctrl Pts',(-15.2085060076969,29.0892469278519,6.39951354132192));
#51196=CARTESIAN_POINT('Ctrl Pts',(-15.4171256703624,29.5972806483711,5.90370851153158));
#51197=CARTESIAN_POINT('Ctrl Pts',(-16.1302336446393,29.745997269232,6.03321141943556));
#51198=CARTESIAN_POINT('Ctrl Pts',(-15.2369722744217,29.0075062116329,6.33129394724583));
#51199=CARTESIAN_POINT('Ctrl Pts',(-15.4425151412656,29.5251196490867,5.83662745356123));
#51200=CARTESIAN_POINT('Ctrl Pts',(-16.160425139482,29.6733388547696,5.96889665059839));
#51201=CARTESIAN_POINT('Ctrl Pts',(-15.246473323653,28.980385210548,6.30838130181911));
#51202=CARTESIAN_POINT('Ctrl Pts',(-15.4509873595446,29.5011789547939,5.81409473052649));
#51203=CARTESIAN_POINT('Ctrl Pts',(-16.170502009992,29.6492312982821,5.94729550340031));
#51204=CARTESIAN_POINT('Ctrl Pts',(-15.2654961612181,28.926395398229,6.26220810975159));
#51205=CARTESIAN_POINT('Ctrl Pts',(-15.4679323239667,29.4535620737581,5.76872117594484));
#51206=CARTESIAN_POINT('Ctrl Pts',(-16.1906777466895,29.601240353964,5.90376522131281));
#51207=CARTESIAN_POINT('Ctrl Pts',(-15.2750230398706,28.8995124220965,6.23893492398287));
#51208=CARTESIAN_POINT('Ctrl Pts',(-15.4764096537653,29.4298736780045,5.74586728371073));
#51209=CARTESIAN_POINT('Ctrl Pts',(-16.2007820120252,29.5773443751773,5.88182417079429));
#51210=CARTESIAN_POINT('Ctrl Pts',(-15.3225922161938,28.7660296571919,6.12195830143935));
#51211=CARTESIAN_POINT('Ctrl Pts',(-15.5187963268113,29.3120701815224,5.63080434349472));
#51212=CARTESIAN_POINT('Ctrl Pts',(-16.2512341685254,29.4586930286934,5.77154317966401));
#51213=CARTESIAN_POINT('Ctrl Pts',(-15.3604967735573,28.6620554042277,6.02628494806573));
#51214=CARTESIAN_POINT('Ctrl Pts',(-15.552341978002,29.22088933467,5.5371846231952));
#51215=CARTESIAN_POINT('Ctrl Pts',(-16.2914359721255,29.3662714703737,5.68134607909259));
#51216=CARTESIAN_POINT('Ctrl Pts',(-15.4734024711476,28.3583437765312,5.73303598356708));
#51217=CARTESIAN_POINT('Ctrl Pts',(-15.6521452749257,28.9546179419119,5.25025045759224));
#51218=CARTESIAN_POINT('Ctrl Pts',(-16.4111844387542,29.0963055792408,5.40488240853399));
#51219=CARTESIAN_POINT('Ctrl Pts',(-15.5475928105337,28.166793334864,5.52924812560617));
#51220=CARTESIAN_POINT('Ctrl Pts',(-15.716867186315,28.7887594038429,5.0526403038573));
#51221=CARTESIAN_POINT('Ctrl Pts',(-16.4898711630596,28.9260385198999,5.21275917575155));
#51222=CARTESIAN_POINT('Ctrl Pts',(-15.6920332500668,27.804967416518,5.10493090212559));
#51223=CARTESIAN_POINT('Ctrl Pts',(-15.8416653101424,28.4777545766966,4.64442044202835));
#51224=CARTESIAN_POINT('Ctrl Pts',(-16.6430655678803,28.6044154813285,4.8127294699215));
#51225=CARTESIAN_POINT('Ctrl Pts',(-15.7622877731009,27.6346927109898,4.88440241921411));
#51226=CARTESIAN_POINT('Ctrl Pts',(-15.9016653391294,28.3329345034696,4.43369484971485));
#51227=CARTESIAN_POINT('Ctrl Pts',(-16.7175779415832,28.4530601877117,4.6048238295626));
#51228=CARTESIAN_POINT('Ctrl Pts',(-15.8634153592665,27.3953869383753,4.54052076838177));
#51229=CARTESIAN_POINT('Ctrl Pts',(-15.9868838517309,28.1316515312056,4.10893296665195));
#51230=CARTESIAN_POINT('Ctrl Pts',(-16.8248344717416,28.2403439451399,4.280625640225));
#51231=CARTESIAN_POINT('Ctrl Pts',(-15.8964154242514,27.3183086387693,4.42370773816891));
#51232=CARTESIAN_POINT('Ctrl Pts',(-16.0146143413019,28.0669533026489,3.99868427600105));
#51233=CARTESIAN_POINT('Ctrl Pts',(-16.8598345410939,28.1718299012522,4.17049887771516));
#51234=CARTESIAN_POINT('Ctrl Pts',(-15.9446833059184,27.2068010501802,4.24510042840518));
#51235=CARTESIAN_POINT('Ctrl Pts',(-16.0548906467027,27.9739186191265,3.83109036355919));
#51236=CARTESIAN_POINT('Ctrl Pts',(-16.9110277485907,28.0727120445427,4.00211488200807));
#51237=CARTESIAN_POINT('Ctrl Pts',(-15.9605671695884,27.1703172329925,4.18499971903105));
#51238=CARTESIAN_POINT('Ctrl Pts',(-16.0681256678962,27.9435097431242,3.7747202284785));
#51239=CARTESIAN_POINT('Ctrl Pts',(-16.9278742708902,28.0402819849552,3.94545428055366));
#51240=CARTESIAN_POINT('Ctrl Pts',(-15.9840630498228,27.1166326670936,4.09398463298263));
#51241=CARTESIAN_POINT('Ctrl Pts',(-16.0876324266849,27.8989052244231,3.68960145288528));
#51242=CARTESIAN_POINT('Ctrl Pts',(-16.9527941436941,27.9925623707134,3.85964881224669));
#51243=CARTESIAN_POINT('Ctrl Pts',(-15.9918400182461,27.098911365518,4.06350224576308));
#51244=CARTESIAN_POINT('Ctrl Pts',(-16.0940844067552,27.8841885644318,3.66110082717283));
#51245=CARTESIAN_POINT('Ctrl Pts',(-16.9610424436527,27.9768101027221,3.83091120811858));
#51246=CARTESIAN_POINT('Ctrl Pts',(-16.0072802673827,27.0638183876329,4.00224638321511));
#51247=CARTESIAN_POINT('Ctrl Pts',(-16.1068754781049,27.8550811453129,3.60388755733143));
#51248=CARTESIAN_POINT('Ctrl Pts',(-16.9774184653475,27.9456163445231,3.77316157340969));
#51249=CARTESIAN_POINT('Ctrl Pts',(-16.0149484597681,27.0464356133835,3.97145286285566));
#51250=CARTESIAN_POINT('Ctrl Pts',(-16.11321832627,27.8406819961272,3.57515643717542));
#51251=CARTESIAN_POINT('Ctrl Pts',(-16.9855513967497,27.9301649896533,3.74413064513307));
#51252=CARTESIAN_POINT('Ctrl Pts',(-16.0833253347986,26.8918211440726,3.69342860679508));
#51253=CARTESIAN_POINT('Ctrl Pts',(-16.1700064472163,27.7120571742295,3.3145971632474));
#51254=CARTESIAN_POINT('Ctrl Pts',(-17.0580723245784,27.7927299060094,3.48202023522934));
#51255=CARTESIAN_POINT('Ctrl Pts',(-16.1392489563977,26.7681000791065,3.44139585389464));
#51256=CARTESIAN_POINT('Ctrl Pts',(-16.2154998129262,27.611079704592,3.08181765987248));
#51257=CARTESIAN_POINT('Ctrl Pts',(-17.1173852570175,27.6827556258494,3.24441359968121));
#51258=CARTESIAN_POINT('Ctrl Pts',(-16.2403199527415,26.5474550953827,2.92755360879577));
#51259=CARTESIAN_POINT('Ctrl Pts',(-16.2970459414564,27.4321275309776,2.61077340535992));
#51260=CARTESIAN_POINT('Ctrl Pts',(-17.2245817678271,27.4866267514743,2.7599832001616));
#51261=CARTESIAN_POINT('Ctrl Pts',(-16.2854701813921,26.4505327273823,2.66574409615585));
#51262=CARTESIAN_POINT('Ctrl Pts',(-16.3329171219314,27.3545890540287,2.37293766614214));
#51263=CARTESIAN_POINT('Ctrl Pts',(-17.272468374468,27.4004735355853,2.51315941724635));
#51264=CARTESIAN_POINT('Ctrl Pts',(-16.3638891417636,26.2837240365077,2.13210289884751));
#51265=CARTESIAN_POINT('Ctrl Pts',(-16.3948333150909,27.2217630392128,1.89119238259305));
#51266=CARTESIAN_POINT('Ctrl Pts',(-17.3556399985759,27.252199143428,2.01006333898577));
#51267=CARTESIAN_POINT('Ctrl Pts',(-16.3971609665106,26.2138347665803,1.86027258862789));
#51268=CARTESIAN_POINT('Ctrl Pts',(-16.4207214647061,27.1668306081169,1.64783726428005));
#51269=CARTESIAN_POINT('Ctrl Pts',(-17.3909282981186,27.1900753483798,1.75379233941467));
#51270=CARTESIAN_POINT('Ctrl Pts',(-16.4372282316227,26.1301157641184,1.44461189527185));
#51271=CARTESIAN_POINT('Ctrl Pts',(-16.4517534962573,27.1012636221844,1.27786031263812));
#51272=CARTESIAN_POINT('Ctrl Pts',(-17.4334238818719,27.1156584568399,1.36192367232642));
#51273=CARTESIAN_POINT('Ctrl Pts',(-16.4489425836071,26.1057357203802,1.30473676381471));
#51274=CARTESIAN_POINT('Ctrl Pts',(-16.4607946572,27.0822242725002,1.15354204459136));
#51275=CARTESIAN_POINT('Ctrl Pts',(-17.4458481948988,27.0939873072066,1.23005486149115));
#51276=CARTESIAN_POINT('Ctrl Pts',(-16.4614235356195,26.0798156556365,1.12817920332052));
#51277=CARTESIAN_POINT('Ctrl Pts',(-16.4704032550175,27.0620254439469,0.997028004066201));
#51278=CARTESIAN_POINT('Ctrl Pts',(-17.4590855680403,27.0709472494042,1.06360328933017));
#51279=CARTESIAN_POINT('Ctrl Pts',(-16.4638105601819,26.074861696503,1.09279299652423));
#51280=CARTESIAN_POINT('Ctrl Pts',(-16.4722410434965,27.0581642796167,0.965648605363661));
#51281=CARTESIAN_POINT('Ctrl Pts',(-17.4616172607913,27.0665437301925,1.03024255564937));
#51282=CARTESIAN_POINT('Ctrl Pts',(-16.4683507346043,26.0654443842168,1.02209528756755));
#51283=CARTESIAN_POINT('Ctrl Pts',(-16.4757345383337,27.0508278725685,0.902983985062077));
#51284=CARTESIAN_POINT('Ctrl Pts',(-17.4664325973152,27.0581727860028,0.963591516895074));
#51285=CARTESIAN_POINT('Ctrl Pts',(-16.470506063436,26.0609765048028,0.986753620408229));
#51286=CARTESIAN_POINT('Ctrl Pts',(-16.4773917386444,27.047349490258,0.871673646590079));
#51287=CARTESIAN_POINT('Ctrl Pts',(-17.4687185521219,27.0542013375728,0.930272773451819));
#51288=CARTESIAN_POINT('Ctrl Pts',(-16.4766286018102,26.0482910800257,0.880750072548012));
#51289=CARTESIAN_POINT('Ctrl Pts',(-16.4820979767805,27.0374753525219,0.777776718980477));
#51290=CARTESIAN_POINT('Ctrl Pts',(-17.4752121534494,27.0429254045267,0.830336768726166));
#51291=CARTESIAN_POINT('Ctrl Pts',(-16.4802523787863,26.0407916272951,0.810109642405695));
#51292=CARTESIAN_POINT('Ctrl Pts',(-16.4848785011,27.0316471633613,0.715279089642234));
#51293=CARTESIAN_POINT('Ctrl Pts',(-17.4790555532451,27.0362592242133,0.763739730217897));
#51294=CARTESIAN_POINT('Ctrl Pts',(-16.4897560121036,26.0211373031105,0.598273404163521));
#51295=CARTESIAN_POINT('Ctrl Pts',(-16.4921690314085,27.0163743171162,0.527896985305773));
#51296=CARTESIAN_POINT('Ctrl Pts',(-17.4891351643784,27.0187887139739,0.564028798530454));
#51297=CARTESIAN_POINT('Ctrl Pts',(-16.4942684087839,26.0118246449525,0.457162601989202));
#51298=CARTESIAN_POINT('Ctrl Pts',(-16.4956179815424,27.0091615199262,0.403342719886046));
#51299=CARTESIAN_POINT('Ctrl Pts',(-17.4939210395996,27.0105107954566,0.430995045648165));
#51300=CARTESIAN_POINT('Ctrl Pts',(-16.4996728834952,26.0006733566253,0.175164846125518));
#51301=CARTESIAN_POINT('Ctrl Pts',(-16.4997511923146,27.0005192273558,0.154469345431858));
#51302=CARTESIAN_POINT('Ctrl Pts',(-17.4996530582721,27.0005985392793,0.165138575470091));
#51303=CARTESIAN_POINT('Ctrl Pts',(-16.5005649496479,25.9988348222276,0.0342778948658427));
#51304=CARTESIAN_POINT('Ctrl Pts',(-16.5004319098763,26.9990972249887,0.0302562756544078));
#51305=CARTESIAN_POINT('Ctrl Pts',(-17.5005991890068,26.9989642864088,0.0323158604794608));
#51306=CARTESIAN_POINT('Ctrl Pts',(-16.4978390182597,26.0044568076987,-0.388049293380772));
#51307=CARTESIAN_POINT('Ctrl Pts',(-16.4983485327184,27.0034518225239,-0.342280149680354));
#51308=CARTESIAN_POINT('Ctrl Pts',(-17.4977080496968,27.0039616068747,-0.365837717665129));
#51309=CARTESIAN_POINT('Ctrl Pts',(-16.4888223219516,26.0230271690527,-0.669156567504712));
#51310=CARTESIAN_POINT('Ctrl Pts',(-16.4914905865413,27.0177691015244,-0.589955966903106));
#51311=CARTESIAN_POINT('Ctrl Pts',(-17.4881448869157,27.020468594845,-0.630854676420441));
#51312=CARTESIAN_POINT('Ctrl Pts',(-16.4645479010849,26.0733210916423,-1.09014697727432));
#51313=CARTESIAN_POINT('Ctrl Pts',(-16.4728185592198,27.0569442887207,-0.963125072170838));
#51314=CARTESIAN_POINT('Ctrl Pts',(-17.4623992890308,27.0651743036164,-1.02774799205062));
#51315=CARTESIAN_POINT('Ctrl Pts',(-16.4546639962014,26.0938323280556,-1.23036518951515));
#51316=CARTESIAN_POINT('Ctrl Pts',(-16.4652151995949,27.0729175749462,-1.08745697835527));
#51317=CARTESIAN_POINT('Ctrl Pts',(-17.4519163596122,27.0834065139337,-1.15994024599047));
#51318=CARTESIAN_POINT('Ctrl Pts',(-16.4400673858426,26.1242298032478,-1.40549624934421));
#51319=CARTESIAN_POINT('Ctrl Pts',(-16.4539221087833,27.0967120128198,-1.2433380557798));
#51320=CARTESIAN_POINT('Ctrl Pts',(-17.4364351061955,27.1104264917492,-1.32504696908299));
#51321=CARTESIAN_POINT('Ctrl Pts',(-16.4370359610415,26.130547367242,-1.44051537232677));
#51322=CARTESIAN_POINT('Ctrl Pts',(-16.4515773822401,27.1016553378582,-1.27449396665141));
#51323=CARTESIAN_POINT('Ctrl Pts',(-17.433219958682,27.1160421042443,-1.35806163047139));
#51324=CARTESIAN_POINT('Ctrl Pts',(-16.4307488113996,26.1436611143959,-1.51053938021269));
#51325=CARTESIAN_POINT('Ctrl Pts',(-16.4467096966894,27.1119250811992,-1.33683413188026));
#51326=CARTESIAN_POINT('Ctrl Pts',(-17.4265517696646,27.1276987683228,-1.42407753017187));
#51327=CARTESIAN_POINT('Ctrl Pts',(-16.4274906111759,26.1504624708553,-1.54556967700777));
#51328=CARTESIAN_POINT('Ctrl Pts',(-16.4441850672634,27.1172550250431,-1.36803947412004));
#51329=CARTESIAN_POINT('Ctrl Pts',(-17.4230961027206,27.1337444184933,-1.45710272580348));
#51330=CARTESIAN_POINT('Ctrl Pts',(-16.4173982522689,26.1715491252668,-1.65044486531198));
#51331=CARTESIAN_POINT('Ctrl Pts',(-16.43635996178,27.1337879226008,-1.46149208806462));
#51332=CARTESIAN_POINT('Ctrl Pts',(-17.4123920858232,27.1524881114378,-1.55597495718666));
#51333=CARTESIAN_POINT('Ctrl Pts',(-16.4102542800575,26.186500310749,-1.72000002026246));
#51334=CARTESIAN_POINT('Ctrl Pts',(-16.4308099461936,27.1455302764211,-1.52357398570511));
#51335=CARTESIAN_POINT('Ctrl Pts',(-17.4048151454351,27.1657780539216,-1.62154884066042));
#51336=CARTESIAN_POINT('Ctrl Pts',(-16.3725127956242,26.2656547133766,-2.06599962503883));
#51337=CARTESIAN_POINT('Ctrl Pts',(-16.4014953816007,27.2076634406906,-1.83207874075241));
#51338=CARTESIAN_POINT('Ctrl Pts',(-17.3647862987107,27.2361375233113,-1.94774375420961));
#51339=CARTESIAN_POINT('Ctrl Pts',(-16.3358579567688,26.3430155684638,-2.33712916293811));
#51340=CARTESIAN_POINT('Ctrl Pts',(-16.3728357498743,27.2687196259979,-2.07564354115728));
#51341=CARTESIAN_POINT('Ctrl Pts',(-17.3259099538696,27.3049027273893,-2.20335409300917));
#51342=CARTESIAN_POINT('Ctrl Pts',(-16.2509489421038,26.5246876648651,-2.86863842077008));
#51343=CARTESIAN_POINT('Ctrl Pts',(-16.3054421715168,27.4140279801895,-2.55725670467926));
#51344=CARTESIAN_POINT('Ctrl Pts',(-17.2358549388741,27.4663890355697,-2.70444026200191));
#51345=CARTESIAN_POINT('Ctrl Pts',(-16.2026914231958,26.6290018643058,-3.12901661081332));
#51346=CARTESIAN_POINT('Ctrl Pts',(-16.2668736654531,27.4979009908363,-2.79478543759917));
#51347=CARTESIAN_POINT('Ctrl Pts',(-17.1846727213246,27.5591127682956,-2.94991464986886));
#51348=CARTESIAN_POINT('Ctrl Pts',(-16.1224929527533,26.8055233058917,-3.511724585575));
#51349=CARTESIAN_POINT('Ctrl Pts',(-16.2015927972012,27.6422088112504,-3.14811650491222));
#51350=CARTESIAN_POINT('Ctrl Pts',(-17.099613737892,27.7160207163362,-3.31071678104154));
#51351=CARTESIAN_POINT('Ctrl Pts',(-16.0944573592689,26.8677122005455,-3.6379817080266));
#51352=CARTESIAN_POINT('Ctrl Pts',(-16.1787224577041,27.6931119961222,-3.2648130549793));
#51353=CARTESIAN_POINT('Ctrl Pts',(-17.0698790172897,27.7712997338665,-3.42974706475798));
#51354=CARTESIAN_POINT('Ctrl Pts',(-16.0578742587549,26.9496675749635,-3.79416704657873));
#51355=CARTESIAN_POINT('Ctrl Pts',(-16.1486081613594,27.7607465434304,-3.4101345555538));
#51356=CARTESIAN_POINT('Ctrl Pts',(-17.0310787593147,27.844148955511,-3.57699250183713));
#51357=CARTESIAN_POINT('Ctrl Pts',(-16.0504807062728,26.9662697489414,-3.82532226629593));
#51358=CARTESIAN_POINT('Ctrl Pts',(-16.1425271619055,27.7744328577361,-3.43908652601369));
#51359=CARTESIAN_POINT('Ctrl Pts',(-17.0232371126848,27.8589064435178,-3.60636442612413));
#51360=CARTESIAN_POINT('Ctrl Pts',(-16.0355419811776,26.999897690748,-3.88746893406826));
#51361=CARTESIAN_POINT('Ctrl Pts',(-16.1302215604399,27.8021911773562,-3.49689960574396));
#51362=CARTESIAN_POINT('Ctrl Pts',(-17.0073930103687,27.8887979473173,-3.66495387724952));
#51363=CARTESIAN_POINT('Ctrl Pts',(-16.0279925473271,27.0169331053863,-3.91847760489801));
#51364=CARTESIAN_POINT('Ctrl Pts',(-16.1239938076285,27.8162702352096,-3.52577621154247));
#51365=CARTESIAN_POINT('Ctrl Pts',(-16.9993860349865,27.9039405380826,-3.69418764098899));
#51366=CARTESIAN_POINT('Ctrl Pts',(-16.005151309949,27.0686067279126,-4.01113187201297));
#51367=CARTESIAN_POINT('Ctrl Pts',(-16.1051372201557,27.8589989859183,-3.61208369701427));
#51368=CARTESIAN_POINT('Ctrl Pts',(-16.9751604803637,27.9498726471105,-3.78153846518201));
#51369=CARTESIAN_POINT('Ctrl Pts',(-15.9896858552224,27.1037684311926,-4.07232971282369));
#51370=CARTESIAN_POINT('Ctrl Pts',(-16.0923233519077,27.8881659099294,-3.66925480659103));
#51371=CARTESIAN_POINT('Ctrl Pts',(-16.9587577251248,27.9811274943278,-3.8392333993061));
#51372=CARTESIAN_POINT('Ctrl Pts',(-15.9112419315778,27.2830923847797,-4.37551697666845));
#51373=CARTESIAN_POINT('Ctrl Pts',(-16.0274373719239,28.0366047023604,-3.95173322375266));
#51374=CARTESIAN_POINT('Ctrl Pts',(-16.875559624845,28.1405265645112,-4.1250665099463));
#51375=CARTESIAN_POINT('Ctrl Pts',(-15.844918315659,27.4377681716844,-4.60912492170408));
#51376=CARTESIAN_POINT('Ctrl Pts',(-15.9717543805869,28.166270657865,-4.1723242724571));
#51377=CARTESIAN_POINT('Ctrl Pts',(-16.8052163950039,28.2780161525077,-4.34530295645177));
#51378=CARTESIAN_POINT('Ctrl Pts',(-15.7069099448858,27.7688775711428,-5.05949097805553));
#51379=CARTESIAN_POINT('Ctrl Pts',(-15.8543812193166,28.447094636339,-4.60083479731583));
#51380=CARTESIAN_POINT('Ctrl Pts',(-16.6588438813315,28.5723356188943,-4.76989048439904));
#51381=CARTESIAN_POINT('Ctrl Pts',(-15.6352206245408,27.9453128342832,-5.27624649105232));
#51382=CARTESIAN_POINT('Ctrl Pts',(-15.7928000382307,28.5978883814961,-4.80878789175796));
#51383=CARTESIAN_POINT('Ctrl Pts',(-16.5828097529458,28.7291669638434,-4.97423911600232));
#51384=CARTESIAN_POINT('Ctrl Pts',(-15.5249581839362,28.2263776622186,-5.58908746041189));
#51385=CARTESIAN_POINT('Ctrl Pts',(-15.696693052097,28.8413995443161,-5.11191611245));
#51386=CARTESIAN_POINT('Ctrl Pts',(-16.4658647407159,28.9790023663985,-5.26917336342192));
#51387=CARTESIAN_POINT('Ctrl Pts',(-15.4877493740823,28.3228072898136,-5.69131489459601));
#51388=CARTESIAN_POINT('Ctrl Pts',(-15.6642132176884,28.9249883773396,-5.21099932125141));
#51389=CARTESIAN_POINT('Ctrl Pts',(-16.4264008511294,29.0647175909937,-5.36554939547687));
#51390=CARTESIAN_POINT('Ctrl Pts',(-15.431421554897,28.4716312472057,-5.84158285664235));
#51391=CARTESIAN_POINT('Ctrl Pts',(-15.6147184969787,29.0547764285091,-5.3573483822539));
#51392=CARTESIAN_POINT('Ctrl Pts',(-16.3666592249758,29.1970055530476,-5.50721616119523));
#51393=CARTESIAN_POINT('Ctrl Pts',(-15.4125599052749,28.5219362190851,-5.8911597188493));
#51394=CARTESIAN_POINT('Ctrl Pts',(-15.5981338876659,29.098657869549,-5.40563341726845));
#51395=CARTESIAN_POINT('Ctrl Pts',(-16.3466544449051,29.2417210836625,-5.55395529043817));
#51396=CARTESIAN_POINT('Ctrl Pts',(-15.3841604516061,28.5984513320056,-5.9647546987206));
#51397=CARTESIAN_POINT('Ctrl Pts',(-15.5730837024597,29.1655935118162,-5.47748185994016));
#51398=CARTESIAN_POINT('Ctrl Pts',(-16.3165338123512,29.3097345173226,-5.62333776313334));
#51399=CARTESIAN_POINT('Ctrl Pts',(-15.3746761425149,28.6241326720875,-5.98915795629746));
#51400=CARTESIAN_POINT('Ctrl Pts',(-15.5647153050045,29.1880623175047,-5.50130549482725));
#51401=CARTESIAN_POINT('Ctrl Pts',(-16.3064746965653,29.3325623752064,-5.64634420119125));
#51402=CARTESIAN_POINT('Ctrl Pts',(-15.3556755438085,28.6758503150148,-6.03770718948676));
#51403=CARTESIAN_POINT('Ctrl Pts',(-15.547931168814,29.2333546452359,-5.54873830674073));
#51404=CARTESIAN_POINT('Ctrl Pts',(-16.2863225465049,29.3785336133291,-5.69211452210701));
#51405=CARTESIAN_POINT('Ctrl Pts',(-15.3461631123057,28.7018763061624,-6.06184308744346));
#51406=CARTESIAN_POINT('Ctrl Pts',(-15.5395188506324,29.2561687234751,-5.57233816417615));
#51407=CARTESIAN_POINT('Ctrl Pts',(-16.2762336039025,29.4016678276794,-5.71486890398771));
#51408=CARTESIAN_POINT('Ctrl Pts',(-15.2606323097608,28.9371409426806,-6.27738721348527));
#51409=CARTESIAN_POINT('Ctrl Pts',(-15.4642290688267,29.4614132947124,-5.7820464495127));
#51410=CARTESIAN_POINT('Ctrl Pts',(-16.1855191168777,29.610791949213,-5.918075487456));
#51411=CARTESIAN_POINT('Ctrl Pts',(-15.1848342114096,29.1545099575102,-6.45796308382094));
#51412=CARTESIAN_POINT('Ctrl Pts',(-15.3964943458008,29.6534800554759,-5.96008229317087));
#51413=CARTESIAN_POINT('Ctrl Pts',(-16.1051271935059,29.8040088510832,-6.08831536510389));
#51414=CARTESIAN_POINT('Ctrl Pts',(-15.0356595911467,29.6056859311573,-6.79804515130241));
#51415=CARTESIAN_POINT('Ctrl Pts',(-15.2622391988625,30.0548640664217,-6.29665836970821));
#51416=CARTESIAN_POINT('Ctrl Pts',(-15.9469116879931,30.2050541610657,-6.40893145588782));
#51417=CARTESIAN_POINT('Ctrl Pts',(-14.9622788975724,29.8394929473934,-6.95754936214554));
#51418=CARTESIAN_POINT('Ctrl Pts',(-15.1956484255345,30.2641311892708,-6.45556673433959));
#51419=CARTESIAN_POINT('Ctrl Pts',(-15.8690836788716,30.4128826199675,-6.55930579570915));
#51420=CARTESIAN_POINT('Ctrl Pts',(-14.8199953655875,30.3240935251076,-7.25568882321979));
#51421=CARTESIAN_POINT('Ctrl Pts',(-15.0658271140403,30.7002416979089,-6.75341440551023));
#51422=CARTESIAN_POINT('Ctrl Pts',(-15.7181769032676,30.8436386889222,-6.8403800356117));
#51423=CARTESIAN_POINT('Ctrl Pts',(-14.7510880041712,30.5748839284072,-7.39432626488165));
#51424=CARTESIAN_POINT('Ctrl Pts',(-15.0024895581545,30.9271154442475,-6.89273010331883));
#51425=CARTESIAN_POINT('Ctrl Pts',(-15.645093337422,31.0665634920556,-6.9710820001448));
#51426=CARTESIAN_POINT('Ctrl Pts',(-14.6691811405517,30.8997312170887,-7.55423164883944));
#51427=CARTESIAN_POINT('Ctrl Pts',(-14.9266314159884,31.2233129771628,-7.0542966399533));
#51428=CARTESIAN_POINT('Ctrl Pts',(-15.5582224218811,31.3553166373777,-7.12183455119867));
#51429=CARTESIAN_POINT('Ctrl Pts',(-14.653011891398,30.9652703749227,-7.5855411589654));
#51430=CARTESIAN_POINT('Ctrl Pts',(-14.9116910431975,31.2829158941087,-7.08584557342882));
#51431=CARTESIAN_POINT('Ctrl Pts',(-15.5410732180678,31.4135736666364,-7.15135193426238));
#51432=CARTESIAN_POINT('Ctrl Pts',(-14.6291056146706,31.0644531496729,-7.63148523917637));
#51433=CARTESIAN_POINT('Ctrl Pts',(-14.8895640652671,31.3732579073334,-7.13220066227062));
#51434=CARTESIAN_POINT('Ctrl Pts',(-15.5157180762066,31.5017361330234,-7.19466621881002));
#51435=CARTESIAN_POINT('Ctrl Pts',(-14.6211948006132,31.0976597721854,-7.64662987407586));
#51436=CARTESIAN_POINT('Ctrl Pts',(-14.8822417942904,31.4035020137527,-7.14747837210504));
#51437=CARTESIAN_POINT('Ctrl Pts',(-15.507327818792,31.5312531308516,-7.20894398896686));
#51438=CARTESIAN_POINT('Ctrl Pts',(-14.6054941177937,31.1643679687753,-7.67657654190212));
#51439=CARTESIAN_POINT('Ctrl Pts',(-14.867701061467,31.4642882513809,-7.17769919573129));
#51440=CARTESIAN_POINT('Ctrl Pts',(-15.4906755795184,31.5905493055579,-7.23717653788107));
#51441=CARTESIAN_POINT('Ctrl Pts',(-14.5977025585871,31.1978776275757,-7.69138168422876));
#51442=CARTESIAN_POINT('Ctrl Pts',(-14.8604807256331,31.4948381920921,-7.19264621846369));
#51443=CARTESIAN_POINT('Ctrl Pts',(-15.4824118045141,31.6203356689469,-7.2511342477555));
#51444=CARTESIAN_POINT('Ctrl Pts',(-14.5591761411658,31.3656598443161,-7.76432516797013));
#51445=CARTESIAN_POINT('Ctrl Pts',(-14.8248199038901,31.6476138839898,-7.26619003874707));
#51446=CARTESIAN_POINT('Ctrl Pts',(-15.4415504529436,31.7694754172071,-7.31990251526702));
#51447=CARTESIAN_POINT('Ctrl Pts',(-14.5296413627691,31.5010285289678,-7.81939903927279));
#51448=CARTESIAN_POINT('Ctrl Pts',(-14.7973600530408,31.7713364293414,-7.32192638233487));
#51449=CARTESIAN_POINT('Ctrl Pts',(-15.4102256876126,31.8898031368429,-7.37182401004875));
#51450=CARTESIAN_POINT('Ctrl Pts',(-14.4452230147646,31.9105732769504,-7.97492632680715));
#51451=CARTESIAN_POINT('Ctrl Pts',(-14.7189160078809,32.1454427835541,-7.47912726165049));
#51452=CARTESIAN_POINT('Ctrl Pts',(-15.3206910766111,32.2538429128796,-7.51844906238992));
#51453=CARTESIAN_POINT('Ctrl Pts',(-14.394524204208,32.1881803100535,-8.06571177616595));
#51454=CARTESIAN_POINT('Ctrl Pts',(-14.6714240271853,32.4005576020766,-7.57152225977134));
#51455=CARTESIAN_POINT('Ctrl Pts',(-15.266919610253,32.5006047200686,-7.60403803792814));
#51456=CARTESIAN_POINT('Ctrl Pts',(-14.3060495457409,32.7527931145422,-8.22161662427291));
#51457=CARTESIAN_POINT('Ctrl Pts',(-14.5884881552083,32.9202575071458,-7.73013444004218));
#51458=CARTESIAN_POINT('Ctrl Pts',(-15.1730828518141,33.0024827684609,-7.75101903992668));
#51459=CARTESIAN_POINT('Ctrl Pts',(-14.2682728616157,33.0397984670644,-8.2867370209155));
#51460=CARTESIAN_POINT('Ctrl Pts',(-14.552893734404,33.1852802024212,-7.79666355226168));
#51461=CARTESIAN_POINT('Ctrl Pts',(-15.133016671222,33.2575986374368,-7.81241200590781));
#51462=CARTESIAN_POINT('Ctrl Pts',(-14.2226573712228,33.4777284594361,-8.36462327469889));
#51463=CARTESIAN_POINT('Ctrl Pts',(-14.5098903723144,33.5903491926421,-7.87622892641895));
#51464=CARTESIAN_POINT('Ctrl Pts',(-15.0846366059366,33.6468697416979,-7.8858401244665));
#51465=CARTESIAN_POINT('Ctrl Pts',(-14.2092942502116,33.6249441231039,-8.38727953342513));
#51466=CARTESIAN_POINT('Ctrl Pts',(-14.4972860759252,33.7265132279608,-7.8993776669338));
#51467=CARTESIAN_POINT('Ctrl Pts',(-15.0704635986376,33.7777281094489,-7.90719955992493));
#51468=CARTESIAN_POINT('Ctrl Pts',(-14.1921874059586,33.8476922922332,-8.41617145140093));
#51469=CARTESIAN_POINT('Ctrl Pts',(-14.4811437317631,33.9326839034157,-7.92890420892895));
#51470=CARTESIAN_POINT('Ctrl Pts',(-15.0523199760526,33.9757264819735,-7.93443773206372));
#51471=CARTESIAN_POINT('Ctrl Pts',(-14.1869748028688,33.9222626039221,-8.42495286656801));
#51472=CARTESIAN_POINT('Ctrl Pts',(-14.4762244556026,34.0017015413618,-7.93787844712968));
#51473=CARTESIAN_POINT('Ctrl Pts',(-15.0467914575584,34.0420112034973,-7.94271650708992));
#51474=CARTESIAN_POINT('Ctrl Pts',(-14.1799126492618,34.0346090885612,-8.43682988299433));
#51475=CARTESIAN_POINT('Ctrl Pts',(-14.4695579078732,34.105716008113,-7.95001849700854));
#51476=CARTESIAN_POINT('Ctrl Pts',(-15.0393012946864,34.1418747453823,-7.95391369446155));
#51477=CARTESIAN_POINT('Ctrl Pts',(-14.1776847259483,34.0721397627187,-8.44057300476486));
#51478=CARTESIAN_POINT('Ctrl Pts',(-14.4674547435269,34.1404623010022,-7.9538444086756));
#51479=CARTESIAN_POINT('Ctrl Pts',(-15.0369383456894,34.1752353446439,-7.95744256335628));
#51480=CARTESIAN_POINT('Ctrl Pts',(-14.1745348393834,34.1285598388531,-8.44586089729133));
#51481=CARTESIAN_POINT('Ctrl Pts',(-14.4644807945682,34.192704719503,-7.95924986164786));
#51482=CARTESIAN_POINT('Ctrl Pts',(-15.0335975569284,34.2253865234225,-7.96242778198736));
#51483=CARTESIAN_POINT('Ctrl Pts',(-14.173516877044,34.1473872089809,-8.4475690610768));
#51484=CARTESIAN_POINT('Ctrl Pts',(-14.4635196895548,34.2101377324663,-7.96099596612494));
#51485=CARTESIAN_POINT('Ctrl Pts',(-15.0325178998889,34.242121963541,-7.96403817202918));
#51486=CARTESIAN_POINT('Ctrl Pts',(-14.1720382860565,34.1756594493329,-8.45004921553296));
#51487=CARTESIAN_POINT('Ctrl Pts',(-14.4621235724204,34.2363181267017,-7.96353136267135));
#51488=CARTESIAN_POINT('Ctrl Pts',(-15.0309496973357,34.2672528438503,-7.96637636482709));
#51489=CARTESIAN_POINT('Ctrl Pts',(-14.171553481119,34.1850887269927,-8.45086225174429));
#51490=CARTESIAN_POINT('Ctrl Pts',(-14.4616658100524,34.2450496654721,-7.96436249848284));
#51491=CARTESIAN_POINT('Ctrl Pts',(-15.0304355102747,34.2756344239947,-7.96714286358229));
#51492=CARTESIAN_POINT('Ctrl Pts',(-14.1706000477243,34.2039577059635,-8.45246089334986));
#51493=CARTESIAN_POINT('Ctrl Pts',(-14.4607655369268,34.2625227778338,-7.96599675441144));
#51494=CARTESIAN_POINT('Ctrl Pts',(-15.029424293044,34.2924068497441,-7.96865000047954));
#51495=CARTESIAN_POINT('Ctrl Pts',(-14.1701308662489,34.2134087629436,-8.45324742565082));
#51496=CARTESIAN_POINT('Ctrl Pts',(-14.4603225019436,34.2712748866038,-7.96680082574036));
#51497=CARTESIAN_POINT('Ctrl Pts',(-15.028926676316,34.3008077891872,-7.96939151350123));
#51498=CARTESIAN_POINT('Ctrl Pts',(-14.1696709084508,34.2228423347593,-8.45401835497186));
#51499=CARTESIAN_POINT('Ctrl Pts',(-14.4598881528388,34.2800112558736,-7.96758898230353));
#51500=CARTESIAN_POINT('Ctrl Pts',(-15.0284388422964,34.3091931864527,-7.97011831445158));
#51501=CARTESIAN_POINT('',(-15.0295349626852,35.7093985134194,7.96848509795903));
#51502=CARTESIAN_POINT('Origin',(-15.0295349571007,35.7980733216376,8.96454566463309));
#51503=CARTESIAN_POINT('',(-15.0083310209395,35.,8.00000000518325));
#51504=CARTESIAN_POINT('Origin',(-18.7164865659616,34.9995400237305,2.47743854316487));
#51505=CARTESIAN_POINT('',(-15.0284388455888,34.309193186478,-7.97011831617931));
#51506=CARTESIAN_POINT('Ctrl Pts',(-15.02843884595,34.3091931861949,-7.97011831960585));
#51507=CARTESIAN_POINT('Ctrl Pts',(-15.0288142473897,34.3027403453849,-7.96955903236514));
#51508=CARTESIAN_POINT('Ctrl Pts',(-15.0291947892652,34.2962892726555,-7.96899201083835));
#51509=CARTESIAN_POINT('Ctrl Pts',(-15.0315956288302,34.2561423126393,-7.96541417925132));
#51510=CARTESIAN_POINT('Ctrl Pts',(-15.0423642144861,34.088032797569,-7.94935354892829));
#51511=CARTESIAN_POINT('Ctrl Pts',(-15.0678832016234,33.7888553500623,-7.91115853602496));
#51512=CARTESIAN_POINT('Ctrl Pts',(-15.114218766681,33.3969471600944,-7.84108497328952));
#51513=CARTESIAN_POINT('Ctrl Pts',(-15.1721070596644,33.0117857858136,-7.7523407744212));
#51514=CARTESIAN_POINT('Ctrl Pts',(-15.2408086828326,32.6331700775731,-7.64523216589167));
#51515=CARTESIAN_POINT('Ctrl Pts',(-15.3195994745813,32.2609429659519,-7.51990519357029));
#51516=CARTESIAN_POINT('Ctrl Pts',(-15.3783785863874,32.0169741706016,-7.42420221713392));
#51517=CARTESIAN_POINT('Ctrl Pts',(-15.4169230076772,31.86578574641,-7.36055550663997));
#51518=CARTESIAN_POINT('Ctrl Pts',(-15.4247222721703,31.8356127003689,-7.34763441565639));
#51519=CARTESIAN_POINT('Ctrl Pts',(-15.4404979287257,31.7753956529338,-7.32140733008937));
#51520=CARTESIAN_POINT('Ctrl Pts',(-15.4484765070148,31.7453435409324,-7.30809767333041));
#51521=CARTESIAN_POINT('Ctrl Pts',(-15.4645974622036,31.6854045749681,-7.28110802809177));
#51522=CARTESIAN_POINT('Ctrl Pts',(-15.480871160413,31.6256699667238,-7.25376683616002));
#51523=CARTESIAN_POINT('Ctrl Pts',(-15.4974424841611,31.5663386705606,-7.2257208865272));
#51524=CARTESIAN_POINT('Ctrl Pts',(-15.5391665422511,31.4187349680549,-7.15483721768336));
#51525=CARTESIAN_POINT('Ctrl Pts',(-15.6079136147756,31.186835748441,-7.03634156130629));
#51526=CARTESIAN_POINT('Ctrl Pts',(-15.7160167807744,30.8511654700391,-6.84373604076318));
#51527=CARTESIAN_POINT('Ctrl Pts',(-15.8281946598233,30.5271896294902,-6.63649390534299));
#51528=CARTESIAN_POINT('Ctrl Pts',(-15.9435979596967,30.2145457052581,-6.41469672516666));
#51529=CARTESIAN_POINT('Ctrl Pts',(-16.0614211773277,29.9129824016044,-6.17828945308345));
#51530=CARTESIAN_POINT('Ctrl Pts',(-16.1410674095684,29.7192296560954,-6.01081869654751));
#51531=CARTESIAN_POINT('Ctrl Pts',(-16.201024234375,29.5766379294931,-5.88143375879927));
#51532=CARTESIAN_POINT('Ctrl Pts',(-16.2310582334771,29.5060231437582,-5.81579531894369));
#51533=CARTESIAN_POINT('Ctrl Pts',(-16.2611403443223,29.4364318013772,-5.7487171537012));
#51534=CARTESIAN_POINT('Ctrl Pts',(-16.2812018557675,29.3902654189335,-5.70367582739167));
#51535=CARTESIAN_POINT('Ctrl Pts',(-16.2912418263893,29.3672829433228,-5.68098052707624));
#51536=CARTESIAN_POINT('Ctrl Pts',(-16.3413467073928,29.2531738137251,-5.56692428562546));
#51537=CARTESIAN_POINT('Ctrl Pts',(-16.4209752464494,29.0755663284312,-5.3805739525971));
#51538=CARTESIAN_POINT('Ctrl Pts',(-16.5380927043861,28.8237073710608,-5.08947253852862));
#51539=CARTESIAN_POINT('Ctrl Pts',(-16.6521988334264,28.5861941970401,-4.78670273079409));
#51540=CARTESIAN_POINT('Ctrl Pts',(-16.7626209181631,28.3629560370339,-4.47207657050143));
#51541=CARTESIAN_POINT('Ctrl Pts',(-16.8686811319134,28.1540567825967,-4.14530483840524));
#51542=CARTESIAN_POINT('Ctrl Pts',(-16.9360190919976,28.0244823886621,-3.91909753316576));
#51543=CARTESIAN_POINT('Ctrl Pts',(-16.9769015617865,27.9465993498682,-3.77499834205324));
#51544=CARTESIAN_POINT('Ctrl Pts',(-16.9850178352183,27.9311779156137,-3.74604241809553));
#51545=CARTESIAN_POINT('Ctrl Pts',(-16.9970989762738,27.9082802658396,-3.70240206850094));
#51546=CARTESIAN_POINT('Ctrl Pts',(-17.0011098039485,27.9006880857066,-3.68782323736656));
#51547=CARTESIAN_POINT('Ctrl Pts',(-17.0090894186416,27.8856019217284,-3.65863499164274));
#51548=CARTESIAN_POINT('Ctrl Pts',(-17.028939778303,27.8481194758509,-3.58556503300444));
#51549=CARTESIAN_POINT('Ctrl Pts',(-17.0792575849446,27.7536962530504,-3.39428879967496));
#51550=CARTESIAN_POINT('Ctrl Pts',(-17.1517487909967,27.6195487618826,-3.0952359728616));
#51551=CARTESIAN_POINT('Ctrl Pts',(-17.2303931111566,27.4762917371816,-2.72865648498313));
#51552=CARTESIAN_POINT('Ctrl Pts',(-17.3002063624287,27.350831933827,-2.35424175561368));
#51553=CARTESIAN_POINT('Ctrl Pts',(-17.3606800021804,27.2433944968016,-1.97181718960462));
#51554=CARTESIAN_POINT('Ctrl Pts',(-17.3944075483594,27.1840391028347,-1.71137069546056));
#51555=CARTESIAN_POINT('Ctrl Pts',(-17.4133058696165,27.1508915270291,-1.54681069615592));
#51556=CARTESIAN_POINT('Ctrl Pts',(-17.4169764213736,27.1444596371577,-1.51380958994713));
#51557=CARTESIAN_POINT('Ctrl Pts',(-17.4223161454289,27.1351108602685,-1.46417290182852));
#51558=CARTESIAN_POINT('Ctrl Pts',(-17.4240680925248,27.1320449314045,-1.44760711706817));
#51559=CARTESIAN_POINT('Ctrl Pts',(-17.427510627014,27.1260229673048,-1.41448547255394));
#51560=CARTESIAN_POINT('Ctrl Pts',(-17.4359672821553,27.1112359574074,-1.33167245686228));
#51561=CARTESIAN_POINT('Ctrl Pts',(-17.4560080530611,27.0762709715337,-1.11624288587473));
#51562=CARTESIAN_POINT('Ctrl Pts',(-17.4796590959817,27.0351914609743,-0.784389106663583));
#51563=CARTESIAN_POINT('Ctrl Pts',(-17.4965481041675,27.0059632073484,-0.385493539873767));
#51564=CARTESIAN_POINT('Ctrl Pts',(-17.5019201088062,26.9966828319197,0.0140704127324454));
#51565=CARTESIAN_POINT('Ctrl Pts',(-17.4957277861607,27.007381080892,0.414304207998967));
#51566=CARTESIAN_POINT('Ctrl Pts',(-17.4838428507605,27.0279532267182,0.68157702428669));
#51567=CARTESIAN_POINT('Ctrl Pts',(-17.4719965255021,27.0485072370931,0.882202975679014));
#51568=CARTESIAN_POINT('Ctrl Pts',(-17.4675589144571,27.0562131445112,0.949106860867802));
#51569=CARTESIAN_POINT('Ctrl Pts',(-17.46016565691,27.0690684279055,1.04950595922574));
#51570=CARTESIAN_POINT('Ctrl Pts',(-17.457576204753,27.0735734930765,1.08300512007203));
#51571=CARTESIAN_POINT('Ctrl Pts',(-17.452169990578,27.0829854940715,1.14979178074418));
#51572=CARTESIAN_POINT('Ctrl Pts',(-17.4380789555938,27.1075334506051,1.31633108380749));
#51573=CARTESIAN_POINT('Ctrl Pts',(-17.4076148154949,27.1607728178961,1.61230440878633));
#51574=CARTESIAN_POINT('Ctrl Pts',(-17.3566928471347,27.2504459678313,1.99913654017659));
#51575=CARTESIAN_POINT('Ctrl Pts',(-17.2959966478747,27.3583556678014,2.37840729450143));
#51576=CARTESIAN_POINT('Ctrl Pts',(-17.2260177544666,27.4842097230089,2.75029691761448));
#51577=CARTESIAN_POINT('Ctrl Pts',(-17.1472204053951,27.6278648478571,3.11493317863537));
#51578=CARTESIAN_POINT('Ctrl Pts',(-17.0891066131584,27.7355027829494,3.35324065006489));
#51579=CARTESIAN_POINT('Ctrl Pts',(-17.0435370411747,27.8207186810042,3.53018489758881));
#51580=CARTESIAN_POINT('Ctrl Pts',(-17.0280164627851,27.8498722743193,3.58886846092364));
#51581=CARTESIAN_POINT('Ctrl Pts',(-17.0042530981179,27.8947333077787,3.67644679864269));
#51582=CARTESIAN_POINT('Ctrl Pts',(-16.9962509220472,27.9098766629836,3.70556736279662));
#51583=CARTESIAN_POINT('Ctrl Pts',(-16.9800906316592,27.9405369449744,3.76365014419879));
#51584=CARTESIAN_POINT('Ctrl Pts',(-16.939385630851,28.0179595915168,3.90815062897979));
#51585=CARTESIAN_POINT('Ctrl Pts',(-16.8634740930316,28.1641956124784,4.1619841373753));
#51586=CARTESIAN_POINT('Ctrl Pts',(-16.7573535075419,28.373470605273,4.48761501859039));
#51587=CARTESIAN_POINT('Ctrl Pts',(-16.6470263387764,28.5968114902901,4.80086397909257));
#51588=CARTESIAN_POINT('Ctrl Pts',(-16.5331726018234,28.8341259880668,5.1020516925123));
#51589=CARTESIAN_POINT('Ctrl Pts',(-16.4164677141308,29.085452957734,5.39139609998198));
#51590=CARTESIAN_POINT('Ctrl Pts',(-16.337218745459,29.2624588306839,5.57647684233942));
#51591=CARTESIAN_POINT('Ctrl Pts',(-16.2774164172135,29.3988358675752,5.71236190400463));
#51592=CARTESIAN_POINT('Ctrl Pts',(-16.2474239466557,29.4679305471591,5.77957270791569));
#51593=CARTESIAN_POINT('Ctrl Pts',(-16.2173288684335,29.5384043436101,5.84568321462317));
#51594=CARTESIAN_POINT('Ctrl Pts',(-16.1972465822248,29.5856958608511,5.88951186843353));
#51595=CARTESIAN_POINT('Ctrl Pts',(-16.1871956371008,29.6094971671554,5.91130422498456));
#51596=CARTESIAN_POINT('Ctrl Pts',(-16.1370259930167,29.7289888135984,6.01938988251468));
#51597=CARTESIAN_POINT('Ctrl Pts',(-16.057104001546,29.9237370570165,6.18715440328565));
#51598=CARTESIAN_POINT('Ctrl Pts',(-15.9390297178621,30.2265601706113,6.42365959173941));
#51599=CARTESIAN_POINT('Ctrl Pts',(-15.8235394373094,30.5402010295723,6.64525502413354));
#51600=CARTESIAN_POINT('Ctrl Pts',(-15.711436219916,30.8648784241873,6.85203405066681));
#51601=CARTESIAN_POINT('Ctrl Pts',(-15.6035641544746,31.2009178880349,7.04395106973463));
#51602=CARTESIAN_POINT('Ctrl Pts',(-15.5350683010191,31.4328114844198,7.16186232008555));
#51603=CARTESIAN_POINT('Ctrl Pts',(-15.4935287834857,31.5803222487406,7.23234907826555));
#51604=CARTESIAN_POINT('Ctrl Pts',(-15.4852844648543,31.6099533781527,7.24628590532913));
#51605=CARTESIAN_POINT('Ctrl Pts',(-15.4730173574796,31.6545961141017,7.2669485838441));
#51606=CARTESIAN_POINT('Ctrl Pts',(-15.4689437668496,31.6695138682647,7.27379758384884));
#51607=CARTESIAN_POINT('Ctrl Pts',(-15.4608410564491,31.6993756590486,7.28739653528903));
#51608=CARTESIAN_POINT('Ctrl Pts',(-15.4406901777392,31.7741145411665,7.32115558985279));
#51609=CARTESIAN_POINT('Ctrl Pts',(-15.389690259883,31.9695362055099,7.40582888847468));
#51610=CARTESIAN_POINT('Ctrl Pts',(-15.3165927362425,32.2742629280338,7.524737233672));
#51611=CARTESIAN_POINT('Ctrl Pts',(-15.2381817484458,32.6465557331785,7.64936422964285));
#51612=CARTESIAN_POINT('Ctrl Pts',(-15.1698145869288,33.0256109638998,7.7558817690875));
#51613=CARTESIAN_POINT('Ctrl Pts',(-15.1122465540415,33.4116170399966,7.84408549932686));
#51614=CARTESIAN_POINT('Ctrl Pts',(-15.0815844573055,33.6737462095084,7.8904344550347));
#51615=CARTESIAN_POINT('Ctrl Pts',(-15.0616818008391,33.8722127061586,7.92038964138432));
#51616=CARTESIAN_POINT('Ctrl Pts',(-15.0525040437334,33.9719135555013,7.9341649509122));
#51617=CARTESIAN_POINT('Ctrl Pts',(-15.0445252090246,34.0723315773334,7.946104162559));
#51618=CARTESIAN_POINT('Ctrl Pts',(-15.0407388713525,34.1226615238385,7.95176472328057));
#51619=CARTESIAN_POINT('Ctrl Pts',(-15.0395104426334,34.1394609432997,7.95360031025226));
#51620=CARTESIAN_POINT('Ctrl Pts',(-15.0371247553386,34.1730579141521,7.95716360868016));
#51621=CARTESIAN_POINT('Ctrl Pts',(-15.0267058342764,34.3242805352842,7.9727176126038));
#51622=CARTESIAN_POINT('Ctrl Pts',(-15.0126958765289,34.6050757151467,7.99353488525137));
#51623=CARTESIAN_POINT('Ctrl Pts',(-15.008331055905,34.8700262357082,8.00000016462761));
#51624=CARTESIAN_POINT('Ctrl Pts',(-15.0083310220457,35.,8.00000001022362));
#51625=CARTESIAN_POINT('Origin',(-15.0284388422963,34.2228423347594,-8.96638310375809));
#51626=CARTESIAN_POINT('Origin',(6.61363325216158E-15,51.,8.67361737988404E-16));
#51627=CARTESIAN_POINT('',(-5.94976035341753,52.,-16.457531763205));
#51628=CARTESIAN_POINT('Ctrl Pts',(-5.94976035341754,52.,-16.457531763205));
#51629=CARTESIAN_POINT('Ctrl Pts',(-5.92091018747472,52.,-16.3699833162058));
#51630=CARTESIAN_POINT('Ctrl Pts',(-5.88058573380552,51.9872720702992,-16.2882956005765));
#51631=CARTESIAN_POINT('Ctrl Pts',(-5.76788919698701,51.9323282975261,-16.1199790028325));
#51632=CARTESIAN_POINT('Ctrl Pts',(-5.6925630693955,51.8844425112493,-16.041953238066));
#51633=CARTESIAN_POINT('Ctrl Pts',(-5.5029792070492,51.7471294583736,-15.8953437672898));
#51634=CARTESIAN_POINT('Ctrl Pts',(-5.3784566649255,51.6448478052855,-15.8348531695271));
#51635=CARTESIAN_POINT('Ctrl Pts',(-5.07172747130897,51.3688831050111,-15.7570153376578));
#51636=CARTESIAN_POINT('Ctrl Pts',(-4.8896501126788,51.1882155912351,-15.7607283411234));
#51637=CARTESIAN_POINT('Ctrl Pts',(-4.71705612317004,51.0029762705271,-15.8113722756368));
#51638=CARTESIAN_POINT('Ctrl Pts',(-4.71567047028168,51.0014881341726,-15.8117821292766));
#51639=CARTESIAN_POINT('Ctrl Pts',(-4.71428571428572,51.,-15.8121949837485));
#51640=CARTESIAN_POINT('',(-11.,52.,-13.6106575888162));
#51641=CARTESIAN_POINT('Origin',(6.61363325216158E-15,52.,8.67361737988404E-16));
#51642=CARTESIAN_POINT('Origin',(-11.,51.,-13.6106575888162));
#51643=CARTESIAN_POINT('Origin',(-39.,35.,5.80048162279745E-15));
#51644=CARTESIAN_POINT('',(-39.,35.,8.00000000000001));
#51645=CARTESIAN_POINT('Origin',(-39.,35.,5.80048162279745E-15));
#51646=CARTESIAN_POINT('',(-39.,35.,8.00000000000001));
#51647=CARTESIAN_POINT('',(-15.0083310198037,35.0000000000015,-8.));
#51648=CARTESIAN_POINT('Ctrl Pts',(-15.0295349695495,35.7093985242134,7.96848522340063));
#51649=CARTESIAN_POINT('Ctrl Pts',(-15.0317433566877,35.7463665553888,7.9651940122473));
#51650=CARTESIAN_POINT('Ctrl Pts',(-15.0426551625308,35.9157991681627,7.94891905114317));
#51651=CARTESIAN_POINT('Ctrl Pts',(-15.0683544668512,36.2154241996097,7.91044832409081));
#51652=CARTESIAN_POINT('Ctrl Pts',(-15.114523084639,36.6052396991958,7.84062095850993));
#51653=CARTESIAN_POINT('Ctrl Pts',(-15.172467467588,36.9904539840521,7.75178521528497));
#51654=CARTESIAN_POINT('Ctrl Pts',(-15.2185721709881,37.244239624975,7.67989792119497));
#51655=CARTESIAN_POINT('Ctrl Pts',(-15.2558111371868,37.4334547433118,7.62119799676034));
#51656=CARTESIAN_POINT('Ctrl Pts',(-15.268667511965,37.4963390291725,7.60083353802511));
#51657=CARTESIAN_POINT('Ctrl Pts',(-15.2885991240044,37.5903849273567,7.56908189171299));
#51658=CARTESIAN_POINT('Ctrl Pts',(-15.2953521390605,37.6216927344669,7.55829506683936));
#51659=CARTESIAN_POINT('Ctrl Pts',(-15.3090652550016,37.6841895101737,7.53632694253893));
#51660=CARTESIAN_POINT('Ctrl Pts',(-15.3160188918469,37.7153492440176,7.52515600677147));
#51661=CARTESIAN_POINT('Ctrl Pts',(-15.3301157600136,37.7774928123971,7.50244147730046));
#51662=CARTESIAN_POINT('Ctrl Pts',(-15.3372528052153,37.8084492084351,7.49090783546308));
#51663=CARTESIAN_POINT('Ctrl Pts',(-15.3516906205381,37.8701004077745,7.46750369133237));
#51664=CARTESIAN_POINT('Ctrl Pts',(-15.3735964730095,37.9622016702459,7.43188662647507));
#51665=CARTESIAN_POINT('Ctrl Pts',(-15.426398756667,38.1745080970591,7.34522943759552));
#51666=CARTESIAN_POINT('Ctrl Pts',(-15.5063260286961,38.4705902033911,7.21146276609788));
#51667=CARTESIAN_POINT('Ctrl Pts',(-15.6084646962283,38.8148708775374,7.03535999982788));
#51668=CARTESIAN_POINT('Ctrl Pts',(-15.7159292600327,39.1485423724363,6.84388495360455));
#51669=CARTESIAN_POINT('Ctrl Pts',(-15.8278724895593,39.4719107714082,6.63710017888903));
#51670=CARTESIAN_POINT('Ctrl Pts',(-15.9434872372281,39.7851866573214,6.41492553412863));
#51671=CARTESIAN_POINT('Ctrl Pts',(-16.0224930219074,39.9873883122765,6.25640141129698));
#51672=CARTESIAN_POINT('Ctrl Pts',(-16.0673335103357,40.0992617711462,6.16423464647279));
#51673=CARTESIAN_POINT('Ctrl Pts',(-16.0723213408302,40.111666233097,6.15395223729438));
#51674=CARTESIAN_POINT('Ctrl Pts',(-16.0823076167348,40.136423295282,6.13330380375607));
#51675=CARTESIAN_POINT('Ctrl Pts',(-16.0873075880137,40.1487796487392,6.12293460055931));
#51676=CARTESIAN_POINT('Ctrl Pts',(-16.1023100598661,40.1857398541654,6.09172739208938));
#51677=CARTESIAN_POINT('Ctrl Pts',(-16.132319613612,40.2592118635954,6.02892668369661));
#51678=CARTESIAN_POINT('Ctrl Pts',(-16.2023323628313,40.427529809084,5.87969014002514));
#51679=CARTESIAN_POINT('Ctrl Pts',(-16.3020784722276,40.6592297618689,5.6588095006758));
#51680=CARTESIAN_POINT('Ctrl Pts',(-16.4205991740581,40.9235914790975,5.38144641910375));
#51681=CARTESIAN_POINT('Ctrl Pts',(-16.5372329513425,41.1744683699975,5.09166133998441));
#51682=CARTESIAN_POINT('Ctrl Pts',(-16.6512801927899,41.4119248014439,4.78923193375775));
#51683=CARTESIAN_POINT('Ctrl Pts',(-16.7251214017859,41.5612405737725,4.57896164840507));
#51684=CARTESIAN_POINT('Ctrl Pts',(-16.7795021298059,41.6698078920636,4.41790160529719));
#51685=CARTESIAN_POINT('Ctrl Pts',(-16.8064423804818,41.7232361946865,4.336531809764));
#51686=CARTESIAN_POINT('Ctrl Pts',(-16.8329729212215,41.7753671959408,4.25387627744134));
#51687=CARTESIAN_POINT('Ctrl Pts',(-16.8505649915887,41.8098310331041,4.19848369345172));
#51688=CARTESIAN_POINT('Ctrl Pts',(-16.8593017075143,41.8268946495008,4.17068006136599));
#51689=CARTESIAN_POINT('Ctrl Pts',(-16.9026451868541,41.9113027791667,4.03124011453002));
#51690=CARTESIAN_POINT('Ctrl Pts',(-16.9698918351146,42.0406829901195,3.80520340150321));
#51691=CARTESIAN_POINT('Ctrl Pts',(-17.0639163620806,42.2178935594719,3.45729388963807));
#51692=CARTESIAN_POINT('Ctrl Pts',(-17.1505544674681,42.3782570628572,3.10040997734272));
#51693=CARTESIAN_POINT('Ctrl Pts',(-17.2292496749196,42.5216412285864,2.73436563138696));
#51694=CARTESIAN_POINT('Ctrl Pts',(-17.2760301884329,42.6057249429385,2.48405897740466));
#51695=CARTESIAN_POINT('Ctrl Pts',(-17.308829068095,42.6643630785034,2.29389163401185));
#51696=CARTESIAN_POINT('Ctrl Pts',(-17.3246567295576,42.6925754012235,2.19819833775785));
#51697=CARTESIAN_POINT('Ctrl Pts',(-17.3395957513147,42.7191006585463,2.10157180807124));
#51698=CARTESIAN_POINT('Ctrl Pts',(-17.3469144880934,42.732079591568,2.05310130046466));
#51699=CARTESIAN_POINT('Ctrl Pts',(-17.349329687354,42.7363599449743,2.0369130602982));
#51700=CARTESIAN_POINT('Ctrl Pts',(-17.3541024826582,42.7448134688302,2.00453109096472));
#51701=CARTESIAN_POINT('Ctrl Pts',(-17.3753269002319,42.7823820652959,1.85874834776437));
#51702=CARTESIAN_POINT('Ctrl Pts',(-17.4111077681713,42.8453498665281,1.58229806305072));
#51703=CARTESIAN_POINT('Ctrl Pts',(-17.4506671612683,42.9144491571661,1.18931724193939));
#51704=CARTESIAN_POINT('Ctrl Pts',(-17.4791159589772,42.9638671728884,0.793641063198546));
#51705=CARTESIAN_POINT('Ctrl Pts',(-17.4962775848125,42.9935694415057,0.395255512641708));
#51706=CARTESIAN_POINT('Ctrl Pts',(-17.5019512435747,43.0033708970284,-0.00587045182199218));
#51707=CARTESIAN_POINT('Ctrl Pts',(-17.4979229030629,42.996411578592,-0.275147149881629));
#51708=CARTESIAN_POINT('Ctrl Pts',(-17.4929099765896,42.9877388633763,-0.444040376574195));
#51709=CARTESIAN_POINT('Ctrl Pts',(-17.4917847507504,42.9857917334257,-0.477774124639363));
#51710=CARTESIAN_POINT('Ctrl Pts',(-17.4892933114556,42.9814790647192,-0.54509646113387));
#51711=CARTESIAN_POINT('Ctrl Pts',(-17.4851939707346,42.9743815215779,-0.645889850217576));
#51712=CARTESIAN_POINT('Ctrl Pts',(-17.4731187517648,42.9534521747222,-0.879754014765898));
#51713=CARTESIAN_POINT('Ctrl Pts',(-17.4488480317093,42.9112815338686,-1.21014039122987));
#51714=CARTESIAN_POINT('Ctrl Pts',(-17.4089265646358,42.8415254430959,-1.60084195832246));
#51715=CARTESIAN_POINT('Ctrl Pts',(-17.3586077045064,42.7529391960171,-1.98590605797735));
#51716=CARTESIAN_POINT('Ctrl Pts',(-17.298261825805,42.6456925923558,-2.36541901410585));
#51717=CARTESIAN_POINT('Ctrl Pts',(-17.2515785247746,42.5617707505403,-2.6147603356838));
#51718=CARTESIAN_POINT('Ctrl Pts',(-17.2142296691155,42.4941394755673,-2.80039473020187));
#51719=CARTESIAN_POINT('Ctrl Pts',(-17.1949710995766,42.459150835844,-2.89286890143597));
#51720=CARTESIAN_POINT('Ctrl Pts',(-17.1714983596828,42.4162647832962,-3.00015440654776));
#51721=CARTESIAN_POINT('Ctrl Pts',(-17.1612252823544,42.3974405676299,-3.04600495601648));
#51722=CARTESIAN_POINT('Ctrl Pts',(-17.1543293677358,42.3847921027298,-3.07654331078785));
#51723=CARTESIAN_POINT('Ctrl Pts',(-17.1508564955136,42.3784159555916,-3.09180387440957));
#51724=CARTESIAN_POINT('Ctrl Pts',(-17.1194193072583,42.3206396331724,-3.22888779505685));
#51725=CARTESIAN_POINT('Ctrl Pts',(-17.0610778277326,42.2125971495852,-3.46837047222968));
#51726=CARTESIAN_POINT('Ctrl Pts',(-16.9669450105092,42.0350669660386,-3.81550142136755));
#51727=CARTESIAN_POINT('Ctrl Pts',(-16.8668826707291,41.8424294075684,-4.15099303803763));
#51728=CARTESIAN_POINT('Ctrl Pts',(-16.7615498700067,41.6348972977722,-4.47519454537473));
#51729=CARTESIAN_POINT('Ctrl Pts',(-16.6515873621956,41.4125459881677,-4.78836072736283));
#51730=CARTESIAN_POINT('Ctrl Pts',(-16.5376307394374,41.1753160084247,-5.0906578673893));
#51731=CARTESIAN_POINT('Ctrl Pts',(-16.459424578268,41.0071134947669,-5.28499714012445));
#51732=CARTESIAN_POINT('Ctrl Pts',(-16.4149293360004,40.9096091132394,-5.3922889034193));
#51733=CARTESIAN_POINT('Ctrl Pts',(-16.4099784223582,40.8987351149821,-5.40418207913157));
#51734=CARTESIAN_POINT('Ctrl Pts',(-16.4000630421998,40.8769064826911,-5.42791213035301));
#51735=CARTESIAN_POINT('Ctrl Pts',(-16.3950971987479,40.8659487935054,-5.43975226059081));
#51736=CARTESIAN_POINT('Ctrl Pts',(-16.3801965514582,40.8329910004454,-5.47514895551087));
#51737=CARTESIAN_POINT('Ctrl Pts',(-16.3503724304234,40.7667142379802,-5.54547291492612));
#51738=CARTESIAN_POINT('Ctrl Pts',(-16.2806640395699,40.6095423595599,-5.70629895921682));
#51739=CARTESIAN_POINT('Ctrl Pts',(-16.180974215943,40.3778254119992,-5.92688153012738));
#51740=CARTESIAN_POINT('Ctrl Pts',(-16.0619208336956,40.0882521359279,-6.17725540907027));
#51741=CARTESIAN_POINT('Ctrl Pts',(-15.9441997798774,39.7870400491607,-6.41351604010334));
#51742=CARTESIAN_POINT('Ctrl Pts',(-15.8285960066714,39.4739510666078,-6.63574626677591));
#51743=CARTESIAN_POINT('Ctrl Pts',(-15.7534876620311,39.257070777687,-6.77451562138855));
#51744=CARTESIAN_POINT('Ctrl Pts',(-15.6981121142448,39.0912312910581,-6.87502762908889));
#51745=CARTESIAN_POINT('Ctrl Pts',(-15.6752382613982,39.0214687498039,-6.91616449658992));
#51746=CARTESIAN_POINT('Ctrl Pts',(-15.6526439888158,38.9508583499558,-6.95636275137005));
#51747=CARTESIAN_POINT('Ctrl Pts',(-15.6436292758259,38.9225459338593,-6.97236673066097));
#51748=CARTESIAN_POINT('Ctrl Pts',(-15.6391322617862,38.9083519028867,-6.98033309486872));
#51749=CARTESIAN_POINT('Ctrl Pts',(-15.6256917526769,38.8657149425293,-7.00409230751034));
#51750=CARTESIAN_POINT('Ctrl Pts',(-15.5812090766541,38.723169271701,-7.08238741852476));
#51751=CARTESIAN_POINT('Ctrl Pts',(-15.5041012479151,38.462781160908,-7.21524325503216));
#51752=CARTESIAN_POINT('Ctrl Pts',(-15.4083955592681,38.1073501930475,-7.37530469795503));
#51753=CARTESIAN_POINT('Ctrl Pts',(-15.3206097549118,37.7434785335194,-7.51827869502257));
#51754=CARTESIAN_POINT('Ctrl Pts',(-15.2415938895141,37.3709035407501,-7.64400026688226));
#51755=CARTESIAN_POINT('Ctrl Pts',(-15.1953577523619,37.1164948243452,-7.71609520162805));
#51756=CARTESIAN_POINT('Ctrl Pts',(-15.163332038576,36.9233246794636,-7.76564492189045));
#51757=CARTESIAN_POINT('Ctrl Pts',(-15.1530988410459,36.8585404781279,-7.78140743483318));
#51758=CARTESIAN_POINT('Ctrl Pts',(-15.1408856330674,36.7770549489708,-7.8001509829503));
#51759=CARTESIAN_POINT('Ctrl Pts',(-15.1384724307588,36.7607358821017,-7.80385089936044));
#51760=CARTESIAN_POINT('Ctrl Pts',(-15.1337109333127,36.7280919295432,-7.81114447537864));
#51761=CARTESIAN_POINT('Ctrl Pts',(-15.1266636736583,36.6791013644423,-7.82192932151362));
#51762=CARTESIAN_POINT('Ctrl Pts',(-15.101872893652,36.4991978119273,-7.85976165441412));
#51763=CARTESIAN_POINT('Ctrl Pts',(-15.067082344028,36.2033290107109,-7.91236253990328));
#51764=CARTESIAN_POINT('Ctrl Pts',(-15.0334448413432,35.8056518925192,-7.96269982722361));
#51765=CARTESIAN_POINT('Ctrl Pts',(-15.0197896913276,35.5383826286899,-7.98299411499247));
#51766=CARTESIAN_POINT('Ctrl Pts',(-15.0129323471145,35.3371095966479,-7.99317645517523));
#51767=CARTESIAN_POINT('Ctrl Pts',(-15.0103495943628,35.2362677516597,-7.99700746106585));
#51768=CARTESIAN_POINT('Ctrl Pts',(-15.0088365703435,35.1182557469141,-7.99925059538832));
#51769=CARTESIAN_POINT('Ctrl Pts',(-15.0084304452709,35.0549371823108,-7.99985262131205));
#51770=CARTESIAN_POINT('Ctrl Pts',(-15.0083513612805,35.0253618023294,-7.9999698476096));
#51771=CARTESIAN_POINT('Ctrl Pts',(-15.0083332807496,35.0084550273716,-7.99999664859286));
#51772=CARTESIAN_POINT('Ctrl Pts',(-15.0083310198037,35.0042389907688,-8.));
#51773=CARTESIAN_POINT('Ctrl Pts',(-15.0083310198037,35.,-8.));
#51774=CARTESIAN_POINT('Origin',(-18.7165753455904,35.0004252159185,-2.47873660745326));
#51775=CARTESIAN_POINT('Origin',(33.,35.,5.81688018065629E-15));
#51776=CARTESIAN_POINT('',(17.3292735477736,26.271682819109,2.19464782253529));
#51777=CARTESIAN_POINT('',(14.3614066597098,35.,-9.00000016129458));
#51778=CARTESIAN_POINT('Ctrl Pts',(17.3292737690855,26.2716828205678,2.19464785677071));
#51779=CARTESIAN_POINT('Ctrl Pts',(17.3511060669366,26.2365725392203,2.0550110257917));
#51780=CARTESIAN_POINT('Ctrl Pts',(17.3906663845752,26.1732400003362,1.7748105293247));
#51781=CARTESIAN_POINT('Ctrl Pts',(17.437569987258,26.0986411319388,1.35174774880715));
#51782=CARTESIAN_POINT('Ctrl Pts',(17.4718892370587,26.0443244871895,0.925925340728199));
#51783=CARTESIAN_POINT('Ctrl Pts',(17.4934501269048,26.0103138422386,0.497330371512314));
#51784=CARTESIAN_POINT('Ctrl Pts',(17.5020487821195,25.9967743670159,0.0659341336017064));
#51785=CARTESIAN_POINT('Ctrl Pts',(17.4989814353938,26.0016030072543,-0.223560920629813));
#51786=CARTESIAN_POINT('Ctrl Pts',(17.4947294175519,26.0083037272082,-0.386947362930728));
#51787=CARTESIAN_POINT('Ctrl Pts',(17.4942218702242,26.0091036288164,-0.405108992107224));
#51788=CARTESIAN_POINT('Ctrl Pts',(17.493136378926,26.0108145533485,-0.441447458433586));
#51789=CARTESIAN_POINT('Ctrl Pts',(17.4914016205574,26.0135490847956,-0.496002228547374));
#51790=CARTESIAN_POINT('Ctrl Pts',(17.4866302308682,26.0210726538394,-0.622967538857688));
#51791=CARTESIAN_POINT('Ctrl Pts',(17.4742213411114,26.0406537166651,-0.875588561273599));
#51792=CARTESIAN_POINT('Ctrl Pts',(17.4484604427764,26.0813805487345,-1.23279551020348));
#51793=CARTESIAN_POINT('Ctrl Pts',(17.4051428383694,26.1501709226248,-1.65571464127194));
#51794=CARTESIAN_POINT('Ctrl Pts',(17.3498265631662,26.2385485648806,-2.07302547248468));
#51795=CARTESIAN_POINT('Ctrl Pts',(17.2828820574345,26.346327540878,-2.48481427818531));
#51796=CARTESIAN_POINT('Ctrl Pts',(17.2307282660594,26.4310836356844,-2.75569454847502));
#51797=CARTESIAN_POINT('Ctrl Pts',(17.1888715420821,26.49951298051,-2.9574931035026));
#51798=CARTESIAN_POINT('Ctrl Pts',(17.1744623540533,26.5231335077224,-3.0245322647391));
#51799=CARTESIAN_POINT('Ctrl Pts',(17.1521727950165,26.5597867238486,-3.12475040445865));
#51800=CARTESIAN_POINT('Ctrl Pts',(17.1446270920639,26.5722135398249,-3.15811347120182));
#51801=CARTESIAN_POINT('Ctrl Pts',(17.1293335457261,26.5974404738732,-3.22463311481988));
#51802=CARTESIAN_POINT('Ctrl Pts',(17.1060876109449,26.6358447593403,-3.32411522776261));
#51803=CARTESIAN_POINT('Ctrl Pts',(17.0819389615532,26.6759341796544,-3.42271126226114));
#51804=CARTESIAN_POINT('Ctrl Pts',(17.0489628351658,26.7308759359264,-3.55339434614476));
#51805=CARTESIAN_POINT('Ctrl Pts',(17.0321251263301,26.7590259608061,-3.6181906858736));
#51806=CARTESIAN_POINT('Ctrl Pts',(16.9806303848643,26.8454473156521,-3.81091830589896));
#51807=CARTESIAN_POINT('Ctrl Pts',(16.9093393110058,26.9659542661823,-4.06352061760149));
#51808=CARTESIAN_POINT('Ctrl Pts',(16.7952622185118,27.1620749385031,-4.42989921625676));
#51809=CARTESIAN_POINT('Ctrl Pts',(16.6747509585551,27.3732294139522,-4.78421811769584));
#51810=CARTESIAN_POINT('Ctrl Pts',(16.5484803841572,27.5992268215029,-5.12684327183664));
#51811=CARTESIAN_POINT('Ctrl Pts',(16.4171069086335,27.8400050159176,-5.45805051992441));
#51812=CARTESIAN_POINT('Ctrl Pts',(16.281282026911,28.0956280558873,-5.77803208192815));
#51813=CARTESIAN_POINT('Ctrl Pts',(16.1882039368748,28.2760687412164,-5.98394349483031));
#51814=CARTESIAN_POINT('Ctrl Pts',(16.1352639128197,28.3804481175221,-6.09769030982974));
#51815=CARTESIAN_POINT('Ctrl Pts',(16.1293735897666,28.3920858784171,-6.11029996086992));
#51816=CARTESIAN_POINT('Ctrl Pts',(16.1175772019141,28.4154417739722,-6.13546148370861));
#51817=CARTESIAN_POINT('Ctrl Pts',(16.1116694515318,28.4271632637811,-6.14801691836739));
#51818=CARTESIAN_POINT('Ctrl Pts',(16.0939372564988,28.4624208921774,-6.18556695599072));
#51819=CARTESIAN_POINT('Ctrl Pts',(16.0584429638702,28.533296920399,-6.26018989631675));
#51820=CARTESIAN_POINT('Ctrl Pts',(15.9754558171471,28.701195284815,-6.4309991232647));
#51821=CARTESIAN_POINT('Ctrl Pts',(15.8566650947646,28.9482353299555,-6.66570732687656));
#51822=CARTESIAN_POINT('Ctrl Pts',(15.7145096352823,29.2562207641436,-6.93284443275944));
#51823=CARTESIAN_POINT('Ctrl Pts',(15.5735379528705,29.5758923245201,-7.18571569707291));
#51824=CARTESIAN_POINT('Ctrl Pts',(15.4345728291732,29.9075078732476,-7.42444661746228));
#51825=CARTESIAN_POINT('Ctrl Pts',(15.3438463154491,30.1367964068834,-7.57417606209572));
#51826=CARTESIAN_POINT('Ctrl Pts',(15.2767533263472,30.3119673663242,-7.68290785298914));
#51827=CARTESIAN_POINT('Ctrl Pts',(15.2434450761117,30.4003545024313,-7.73638191511748));
#51828=CARTESIAN_POINT('Ctrl Pts',(15.2105406590842,30.4899725877742,-7.7885075658178));
#51829=CARTESIAN_POINT('Ctrl Pts',(15.1886995006888,30.5499950542398,-7.82295681597048));
#51830=CARTESIAN_POINT('Ctrl Pts',(15.1778240237092,30.5801516665408,-7.84003469134717));
#51831=CARTESIAN_POINT('Ctrl Pts',(15.1237240865472,30.731563564408,-7.92462632761097));
#51832=CARTESIAN_POINT('Ctrl Pts',(15.0393580935828,30.9766684727028,-8.05421723123254));
#51833=CARTESIAN_POINT('Ctrl Pts',(14.9202834898964,31.3530424540673,-8.23149492286624));
#51834=CARTESIAN_POINT('Ctrl Pts',(14.8096155182678,31.73838151464,-8.39167232422591));
#51835=CARTESIAN_POINT('Ctrl Pts',(14.7083363206634,32.1330068510787,-8.53460644040646));
#51836=CARTESIAN_POINT('Ctrl Pts',(14.6477694189893,32.4025470501747,-8.6181996854931));
#51837=CARTESIAN_POINT('Ctrl Pts',(14.6052284867057,32.6072444536737,-8.67639054024899));
#51838=CARTESIAN_POINT('Ctrl Pts',(14.5846793849461,32.7102290861197,-8.70435921933926));
#51839=CARTESIAN_POINT('Ctrl Pts',(14.5652670414341,32.8141936760557,-8.73060894583011));
#51840=CARTESIAN_POINT('Ctrl Pts',(14.5525843754099,32.8837243142594,-8.74772307933595));
#51841=CARTESIAN_POINT('Ctrl Pts',(14.5463699486225,32.9186159013033,-8.75609070595351));
#51842=CARTESIAN_POINT('Ctrl Pts',(14.5160511941617,33.0931020531445,-8.79683395861055));
#51843=CARTESIAN_POINT('Ctrl Pts',(14.4722201586652,33.373221817893,-8.85521402989592));
#51844=CARTESIAN_POINT('Ctrl Pts',(14.4210060853739,33.7962428049278,-8.92256078015134));
#51845=CARTESIAN_POINT('Ctrl Pts',(14.384787810699,34.2221320089307,-8.96973958641945));
#51846=CARTESIAN_POINT('Ctrl Pts',(14.3653246092572,34.6234681282666,-8.99493795043249));
#51847=CARTESIAN_POINT('Ctrl Pts',(14.3614067526773,34.8834816469066,-9.00000050730076));
#51848=CARTESIAN_POINT('Ctrl Pts',(14.3614066597098,35.,-9.00000016129458));
#51849=CARTESIAN_POINT('',(14.3614066770412,34.9999999999574,9.00000209879965));
#51850=CARTESIAN_POINT('Ctrl Pts',(14.3614066597098,35.,-9.00000016129458));
#51851=CARTESIAN_POINT('Ctrl Pts',(14.3614066376026,35.0277074310129,-9.00000007901619));
#51852=CARTESIAN_POINT('Ctrl Pts',(14.3615056095479,35.0554333238382,-8.99987205272605));
#51853=CARTESIAN_POINT('Ctrl Pts',(14.3622202944309,35.1553869208446,-8.99894824492613));
#51854=CARTESIAN_POINT('Ctrl Pts',(14.364004617662,35.2638890175708,-8.99664193507595));
#51855=CARTESIAN_POINT('Ctrl Pts',(14.3678708568023,35.3908080930607,-8.99163943659494));
#51856=CARTESIAN_POINT('Ctrl Pts',(14.3699119521736,35.4452738325292,-8.98899671792919));
#51857=CARTESIAN_POINT('Ctrl Pts',(14.3713582357703,35.4816003408514,-8.98712367181897));
#51858=CARTESIAN_POINT('Ctrl Pts',(14.3721244547376,35.4997776671369,-8.98613114393334));
#51859=CARTESIAN_POINT('Ctrl Pts',(14.3793930408947,35.6631611333616,-8.97671315535948));
#51860=CARTESIAN_POINT('Ctrl Pts',(14.3976438853735,35.9514328119009,-8.95303591956361));
#51861=CARTESIAN_POINT('Ctrl Pts',(14.4402174756958,36.3775287174802,-8.89738550077062));
#51862=CARTESIAN_POINT('Ctrl Pts',(14.4972001649901,36.7975284738977,-8.82208837920263));
#51863=CARTESIAN_POINT('Ctrl Pts',(14.5678058281868,37.2116143810925,-8.72746905651757));
#51864=CARTESIAN_POINT('Ctrl Pts',(14.6512515007626,37.6199371740426,-8.61369740670257));
#51865=CARTESIAN_POINT('Ctrl Pts',(14.714922695497,37.8883901560955,-8.52509406629469));
#51866=CARTESIAN_POINT('Ctrl Pts',(14.7823561461911,38.1549915000705,-8.43006851499351));
#51867=CARTESIAN_POINT('Ctrl Pts',(14.8529334900639,38.4173124396441,-8.32948876487167));
#51868=CARTESIAN_POINT('Ctrl Pts',(14.9670194458454,38.7987124669293,-8.16253453804374));
#51869=CARTESIAN_POINT('Ctrl Pts',(15.0882207409183,39.168649536036,-7.97989226158918));
#51870=CARTESIAN_POINT('Ctrl Pts',(15.2155193643328,39.5276214399999,-7.78180070283411));
#51871=CARTESIAN_POINT('Ctrl Pts',(15.347968056224,39.8760186490394,-7.56835432810572));
#51872=CARTESIAN_POINT('Ctrl Pts',(15.4846761045389,40.2141337582382,-7.33951102833573));
#51873=CARTESIAN_POINT('Ctrl Pts',(15.5780895672648,40.432822845256,-7.17656656886614));
#51874=CARTESIAN_POINT('Ctrl Pts',(15.6487987361288,40.5943470971465,-7.05038640806119));
#51875=CARTESIAN_POINT('Ctrl Pts',(15.6724766893401,40.6477728571003,-7.00766401323145));
#51876=CARTESIAN_POINT('Ctrl Pts',(15.708130928521,40.7272893866598,-6.94257369952877));
#51877=CARTESIAN_POINT('Ctrl Pts',(15.7200453127601,40.7537060004307,-6.92069658004402));
#51878=CARTESIAN_POINT('Ctrl Pts',(15.7438699413295,40.8062312885166,-6.87668903736941));
#51879=CARTESIAN_POINT('Ctrl Pts',(15.8034316480523,40.9367982438501,-6.76601855320207));
#51880=CARTESIAN_POINT('Ctrl Pts',(15.9105449908361,41.165170585149,-6.56096252460349));
#51881=CARTESIAN_POINT('Ctrl Pts',(16.0523683483239,41.4558963118018,-6.27508605292446));
#51882=CARTESIAN_POINT('Ctrl Pts',(16.1924509552874,41.7331271079221,-5.97664957951226));
#51883=CARTESIAN_POINT('Ctrl Pts',(16.3300700330948,41.9970137913492,-5.66546287973468));
#51884=CARTESIAN_POINT('Ctrl Pts',(16.4645126454744,42.2475866322906,-5.34123484264189));
#51885=CARTESIAN_POINT('Ctrl Pts',(16.551545459628,42.4056990482232,-5.11612309781091));
#51886=CARTESIAN_POINT('Ctrl Pts',(16.6156629556038,42.5208783365345,-4.94380041397795));
#51887=CARTESIAN_POINT('Ctrl Pts',(16.6421374084707,42.5681598955139,-4.87127202341161));
#51888=CARTESIAN_POINT('Ctrl Pts',(16.6682856596061,42.6145438657752,-4.79781450748127));
#51889=CARTESIAN_POINT('Ctrl Pts',(16.6787183539013,42.6330253866751,-4.76835671677202));
#51890=CARTESIAN_POINT('Ctrl Pts',(16.6839221782026,42.6422314870762,-4.75358816492742));
#51891=CARTESIAN_POINT('Ctrl Pts',(16.6994733659498,42.6697067160829,-4.70922595173132));
#51892=CARTESIAN_POINT('Ctrl Pts',(16.7509399347112,42.7603918942034,-4.56088716452504));
#51893=CARTESIAN_POINT('Ctrl Pts',(16.8401806635805,42.9155723226508,-4.28969471768694));
#51894=CARTESIAN_POINT('Ctrl Pts',(16.9513843119186,43.1054544466778,-3.91911439587559));
#51895=CARTESIAN_POINT('Ctrl Pts',(17.0542658268551,43.2783291427594,-3.53941810887066));
#51896=CARTESIAN_POINT('Ctrl Pts',(17.1482703302904,43.4340806289113,-3.15042074269136));
#51897=CARTESIAN_POINT('Ctrl Pts',(17.2328153607806,43.5724565750841,-2.75187368374423));
#51898=CARTESIAN_POINT('Ctrl Pts',(17.2824584153442,43.6528595920182,-2.4795973691923));
#51899=CARTESIAN_POINT('Ctrl Pts',(17.3170018972331,43.7085800734727,-2.27282393995594));
#51900=CARTESIAN_POINT('Ctrl Pts',(17.3308346565766,43.7308418656642,-2.18613345094775));
#51901=CARTESIAN_POINT('Ctrl Pts',(17.3439433873367,43.7518874172268,-2.09875922302458));
#51902=CARTESIAN_POINT('Ctrl Pts',(17.3491284574022,43.7602078189126,-2.06375449351543));
#51903=CARTESIAN_POINT('Ctrl Pts',(17.3516928181856,43.7643207749255,-2.04621739953348));
#51904=CARTESIAN_POINT('Ctrl Pts',(17.3592888703892,43.7764982940174,-1.99358342260552));
#51905=CARTESIAN_POINT('Ctrl Pts',(17.3839574521878,43.8160064938899,-1.81802250396776));
#51906=CARTESIAN_POINT('Ctrl Pts',(17.4224896102278,43.8774204221013,-1.50098745610886));
#51907=CARTESIAN_POINT('Ctrl Pts',(17.4612538851346,43.9388668744836,-1.07610201267747));
#51908=CARTESIAN_POINT('Ctrl Pts',(17.4872946690239,43.9799852113784,-0.649047627026372));
#51909=CARTESIAN_POINT('Ctrl Pts',(17.5004730817091,44.0007455676255,-0.219815327381889));
#51910=CARTESIAN_POINT('Ctrl Pts',(17.5006202695435,44.0009772133248,0.211616086610037));
#51911=CARTESIAN_POINT('Ctrl Pts',(17.4918963684518,43.9872347552916,0.500725743964407));
#51912=CARTESIAN_POINT('Ctrl Pts',(17.4844632294961,43.9755071850327,0.663777591100614));
#51913=CARTESIAN_POINT('Ctrl Pts',(17.4836018344785,43.974147935278,0.68190836175621));
#51914=CARTESIAN_POINT('Ctrl Pts',(17.4818107925467,43.9713212685151,0.718139871596486));
#51915=CARTESIAN_POINT('Ctrl Pts',(17.4790225731436,43.9669201546786,0.772429726229226));
#51916=CARTESIAN_POINT('Ctrl Pts',(17.4718092998787,43.955528553035,0.898706242354752));
#51917=CARTESIAN_POINT('Ctrl Pts',(17.4545856479766,43.9282975565738,1.14967584344988));
#51918=CARTESIAN_POINT('Ctrl Pts',(17.4221701314698,43.8769122363278,1.5037659231055));
#51919=CARTESIAN_POINT('Ctrl Pts',(17.3713030937696,43.7958350818669,1.9218003241365));
#51920=CARTESIAN_POINT('Ctrl Pts',(17.3089465433007,43.6957424080558,2.33313911665655));
#51921=CARTESIAN_POINT('Ctrl Pts',(17.2355404985145,43.5768880716263,2.73791691800328));
#51922=CARTESIAN_POINT('Ctrl Pts',(17.1514946160016,43.4393880418327,3.13622814947783));
#51923=CARTESIAN_POINT('Ctrl Pts',(17.0886288004399,43.3352780146074,3.3974953294847));
#51924=CARTESIAN_POINT('Ctrl Pts',(17.0390093050541,43.2524898553595,3.59184767367111));
#51925=CARTESIAN_POINT('Ctrl Pts',(17.0220577526584,43.2241091652068,3.65636534982383));
#51926=CARTESIAN_POINT('Ctrl Pts',(16.9873464535774,43.1657674455286,3.78486738977431));
#51927=CARTESIAN_POINT('Ctrl Pts',(16.969665761866,43.1359391994175,3.84855910124427));
#51928=CARTESIAN_POINT('Ctrl Pts',(16.9157105946208,43.044537870347,4.0379531574931));
#51929=CARTESIAN_POINT('Ctrl Pts',(16.8413257578772,42.9175434522878,4.28603888103889));
#51930=CARTESIAN_POINT('Ctrl Pts',(16.7231644518036,42.7121100049819,4.64542937874511));
#51931=CARTESIAN_POINT('Ctrl Pts',(16.5991255965279,42.492026743552,4.99254748112345));
#51932=CARTESIAN_POINT('Ctrl Pts',(16.4698875992596,42.2574533175684,5.32775738380935));
#51933=CARTESIAN_POINT('Ctrl Pts',(16.3361146386698,42.008423365498,5.65133134784423));
#51934=CARTESIAN_POINT('Ctrl Pts',(16.198469624878,41.7448458160864,5.96345545550853));
#51935=CARTESIAN_POINT('Ctrl Pts',(16.1045744613366,41.5592829957575,6.16397321657772));
#51936=CARTESIAN_POINT('Ctrl Pts',(16.0512901439369,41.4520682654557,6.27464008616567));
#51937=CARTESIAN_POINT('Ctrl Pts',(16.0453631674068,41.4401161028038,6.28690688131533));
#51938=CARTESIAN_POINT('Ctrl Pts',(16.0334966898785,41.4161326615954,6.31138140352268));
#51939=CARTESIAN_POINT('Ctrl Pts',(16.0275562424261,41.4040994470756,6.32359104718472));
#51940=CARTESIAN_POINT('Ctrl Pts',(16.0097365606481,41.3679208424132,6.36009103590755));
#51941=CARTESIAN_POINT('Ctrl Pts',(15.9740858574141,41.2952115292935,6.43261248131344));
#51942=CARTESIAN_POINT('Ctrl Pts',(15.890863814573,41.1230941910587,6.59850667395035));
#51943=CARTESIAN_POINT('Ctrl Pts',(15.7721103718677,40.8701837370035,6.82615055965585));
#51944=CARTESIAN_POINT('Ctrl Pts',(15.6306036959951,40.5553723531171,7.08471028746543));
#51945=CARTESIAN_POINT('Ctrl Pts',(15.4908983764982,40.2290636660933,7.32887233497747));
#51946=CARTESIAN_POINT('Ctrl Pts',(15.3538348876611,39.8909717055415,7.55872848618295));
#51947=CARTESIAN_POINT('Ctrl Pts',(15.2648147848089,39.6574545255017,7.70240667061981));
#51948=CARTESIAN_POINT('Ctrl Pts',(15.1991730514431,39.479138636835,7.80653923747221));
#51949=CARTESIAN_POINT('Ctrl Pts',(15.1666333112585,39.3891856742346,7.85769847361585));
#51950=CARTESIAN_POINT('Ctrl Pts',(15.134563221709,39.2980104232192,7.90748435211918));
#51951=CARTESIAN_POINT('Ctrl Pts',(15.1132930875125,39.2369516244807,7.94036795803072));
#51952=CARTESIAN_POINT('Ctrl Pts',(15.102709165511,39.2062731431645,7.95666206124221));
#51953=CARTESIAN_POINT('Ctrl Pts',(15.0501936888608,39.0525234864699,8.03718433153651));
#51954=CARTESIAN_POINT('Ctrl Pts',(14.9685896006955,38.8037728772036,8.16021179815972));
#51955=CARTESIAN_POINT('Ctrl Pts',(14.8543402338744,38.4222100538624,8.32745277700717));
#51956=CARTESIAN_POINT('Ctrl Pts',(14.7491820596274,38.0319615605815,8.47736748319502));
#51957=CARTESIAN_POINT('Ctrl Pts',(14.6540967740514,37.6327106633516,8.6097776148454));
#51958=CARTESIAN_POINT('Ctrl Pts',(14.5981130579524,37.3602821844718,8.68615604995556));
#51959=CARTESIAN_POINT('Ctrl Pts',(14.5591779822573,37.1534953483407,8.73885104080071));
#51960=CARTESIAN_POINT('Ctrl Pts',(14.5435912348191,37.0668202536551,8.75985069153186));
#51961=CARTESIAN_POINT('Ctrl Pts',(14.5288373475413,36.9794852908176,8.77963320861684));
#51962=CARTESIAN_POINT('Ctrl Pts',(14.5230032029764,36.9444981306421,8.78744833921318));
#51963=CARTESIAN_POINT('Ctrl Pts',(14.5201189478982,36.9269725000721,8.79130815741546));
#51964=CARTESIAN_POINT('Ctrl Pts',(14.5115747072029,36.8743539284632,8.80273172881855));
#51965=CARTESIAN_POINT('Ctrl Pts',(14.4838437603909,36.6988470726635,8.83973528280585));
#51966=CARTESIAN_POINT('Ctrl Pts',(14.4407294163151,36.3819306417377,8.89671331084956));
#51967=CARTESIAN_POINT('Ctrl Pts',(14.3981597821212,35.9572273355899,8.95236357748849));
#51968=CARTESIAN_POINT('Ctrl Pts',(14.3708736668771,35.5303620255068,8.98776686292775));
#51969=CARTESIAN_POINT('Ctrl Pts',(14.3621758928815,35.2107881186055,8.99900502627832));
#51970=CARTESIAN_POINT('Ctrl Pts',(14.3614066471014,35.0336685389156,9.0000000921457));
#51971=CARTESIAN_POINT('Ctrl Pts',(14.3614066770504,35.,9.00000019077833));
#51972=CARTESIAN_POINT('',(16.6650252178838,27.3912428642034,4.80695514514033));
#51973=CARTESIAN_POINT('Ctrl Pts',(14.361406677032,34.9999999999149,9.00000400682097));
#51974=CARTESIAN_POINT('Ctrl Pts',(14.3614067455746,34.9229644059056,9.00000228894048));
#51975=CARTESIAN_POINT('Ctrl Pts',(14.3621716465734,34.8458222221036,8.99901109367336));
#51976=CARTESIAN_POINT('Ctrl Pts',(14.3637083702908,34.7685726083627,8.99702402811064));
#51977=CARTESIAN_POINT('Ctrl Pts',(14.3643637517259,34.7356272180259,8.99617658503076));
#51978=CARTESIAN_POINT('Ctrl Pts',(14.3651594087391,34.7026622701312,8.99514768134809));
#51979=CARTESIAN_POINT('Ctrl Pts',(14.3660957379539,34.6696776740137,8.99393635384563));
#51980=CARTESIAN_POINT('Ctrl Pts',(14.368141414638,34.5976134703744,8.99128986542116));
#51981=CARTESIAN_POINT('Ctrl Pts',(14.3708587724685,34.5254555542841,8.98777262053586));
#51982=CARTESIAN_POINT('Ctrl Pts',(14.3742519630813,34.4532030581254,8.98337457196089));
#51983=CARTESIAN_POINT('Ctrl Pts',(14.3759485583877,34.417076810046,8.98117554767339));
#51984=CARTESIAN_POINT('Ctrl Pts',(14.3778141118918,34.3809269179434,8.97875632244572));
#51985=CARTESIAN_POINT('Ctrl Pts',(14.3798490775206,34.3447532465993,8.97611563701531));
#51986=CARTESIAN_POINT('Ctrl Pts',(14.3802164760517,34.3382223482266,8.97563888009407));
#51987=CARTESIAN_POINT('Ctrl Pts',(14.3805894168745,34.3316902734701,8.97515487505152));
#51988=CARTESIAN_POINT('Ctrl Pts',(14.3809678929735,34.3251572486695,8.97466362940566));
#51989=CARTESIAN_POINT('Ctrl Pts',(14.3826857394991,34.2955048241586,8.97243393873792));
#51990=CARTESIAN_POINT('Ctrl Pts',(14.3845179468002,34.2658321669791,8.97005452374758));
#51991=CARTESIAN_POINT('Ctrl Pts',(14.38645825802,34.2362277317391,8.9675331717211));
#51992=CARTESIAN_POINT('Ctrl Pts',(14.386942240259,34.2288433386044,8.96690425735596));
#51993=CARTESIAN_POINT('Ctrl Pts',(14.3874330028229,34.2214622199065,8.9662664337034));
#51994=CARTESIAN_POINT('Ctrl Pts',(14.3879304679243,34.2140854288794,8.96561979379566));
#51995=CARTESIAN_POINT('Ctrl Pts',(14.3904231202817,34.1771224831559,8.96237967004474));
#51996=CARTESIAN_POINT('Ctrl Pts',(14.3930858453617,34.1402354993775,8.95891587155103));
#51997=CARTESIAN_POINT('Ctrl Pts',(14.3959161528055,34.1034250643409,8.95523050427782));
#51998=CARTESIAN_POINT('Ctrl Pts',(14.401578406325,34.0297828825382,8.94785763605516));
#51999=CARTESIAN_POINT('Ctrl Pts',(14.4079114196966,33.9564470634377,8.93959804622122));
#52000=CARTESIAN_POINT('Ctrl Pts',(14.4148947404169,33.8834224278753,8.93046776632826));
#52001=CARTESIAN_POINT('Ctrl Pts',(14.4173568644703,33.8576759787415,8.92724868437009));
#52002=CARTESIAN_POINT('Ctrl Pts',(14.4198998096941,33.8319681413001,8.92392166901741));
#52003=CARTESIAN_POINT('Ctrl Pts',(14.4225226656181,33.8062991668918,8.92048723942206));
#52004=CARTESIAN_POINT('Ctrl Pts',(14.437045367563,33.6641705577073,8.90147086993391));
#52005=CARTESIAN_POINT('Ctrl Pts',(14.4540204796619,33.5232058055879,8.87915783660387));
#52006=CARTESIAN_POINT('Ctrl Pts',(14.4733045744892,33.3833637054076,8.85362171218632));
#52007=CARTESIAN_POINT('Ctrl Pts',(14.4901043922947,33.2615367892057,8.83137528363922));
#52008=CARTESIAN_POINT('Ctrl Pts',(14.5086565400091,33.1405622247914,8.80668273620936));
#52009=CARTESIAN_POINT('Ctrl Pts',(14.528867066016,33.0204133534421,8.77959205822056));
#52010=CARTESIAN_POINT('Ctrl Pts',(14.531855702318,33.0026463107421,8.77558601782092));
#52011=CARTESIAN_POINT('Ctrl Pts',(14.5348806033553,32.9848973261678,8.77152752638015));
#52012=CARTESIAN_POINT('Ctrl Pts',(14.5379414711734,32.9671663399968,8.76741662665445));
#52013=CARTESIAN_POINT('Ctrl Pts',(14.5617013275574,32.8295303132215,8.73550594220284));
#52014=CARTESIAN_POINT('Ctrl Pts',(14.5876282298979,32.6929783895085,8.70043733105985));
#52015=CARTESIAN_POINT('Ctrl Pts',(14.6155833207169,32.5574832879918,8.66223041570325));
#52016=CARTESIAN_POINT('Ctrl Pts',(14.6414955457034,32.4318897215896,8.62681553570283));
#52017=CARTESIAN_POINT('Ctrl Pts',(14.6691503114154,32.3072043916037,8.58870433773101));
#52018=CARTESIAN_POINT('Ctrl Pts',(14.6984381586483,32.1834048098462,8.54791153059053));
#52019=CARTESIAN_POINT('Ctrl Pts',(14.7007471515061,32.1736447087435,8.54469551066296));
#52020=CARTESIAN_POINT('Ctrl Pts',(14.7030662966404,32.1638901210945,8.54146278887225));
#52021=CARTESIAN_POINT('Ctrl Pts',(14.7053955412755,32.1541410394164,8.53821335745142));
#52022=CARTESIAN_POINT('Ctrl Pts',(14.7358712935118,32.0265844087048,8.49569791472005));
#52023=CARTESIAN_POINT('Ctrl Pts',(14.7680697416918,31.8999932610587,8.45033074738783));
#52024=CARTESIAN_POINT('Ctrl Pts',(14.8018905719573,31.7742858516999,8.40206928282887));
#52025=CARTESIAN_POINT('Ctrl Pts',(14.8034422614015,31.7685184338504,8.39985506145912));
#52026=CARTESIAN_POINT('Ctrl Pts',(14.8049972754406,31.7627532434756,8.39763487044287));
#52027=CARTESIAN_POINT('Ctrl Pts',(14.8065554841667,31.7569906915724,8.39540887856089));
#52028=CARTESIAN_POINT('Ctrl Pts',(14.8109956259332,31.7405702037661,8.38906587754876));
#52029=CARTESIAN_POINT('Ctrl Pts',(14.8154614065699,31.7241722485225,8.38267618919588));
#52030=CARTESIAN_POINT('Ctrl Pts',(14.8199480661342,31.7078127299217,8.37624629491226));
#52031=CARTESIAN_POINT('Ctrl Pts',(14.8231269392599,31.6962217381641,8.37169060758047));
#52032=CARTESIAN_POINT('Ctrl Pts',(14.8263172701105,31.6846464233617,8.36711332261336));
#52033=CARTESIAN_POINT('Ctrl Pts',(14.8295180624613,31.6730898846996,8.36251571506522));
#52034=CARTESIAN_POINT('Ctrl Pts',(14.8308348664555,31.6683355318386,8.36062426216231));
#52035=CARTESIAN_POINT('Ctrl Pts',(14.8321535683165,31.6635838810361,8.35872918832101));
#52036=CARTESIAN_POINT('Ctrl Pts',(14.8334741645343,31.6588349038253,8.35683048833469));
#52037=CARTESIAN_POINT('Ctrl Pts',(14.8414870867154,31.6300197487316,8.34530983195877));
#52038=CARTESIAN_POINT('Ctrl Pts',(14.8495681210058,31.6013090652414,8.33365808856993));
#52039=CARTESIAN_POINT('Ctrl Pts',(14.8577151002777,31.5727014456243,8.32187626795633));
#52040=CARTESIAN_POINT('Ctrl Pts',(14.8587809289823,31.5689588532916,8.32033491107015));
#52041=CARTESIAN_POINT('Ctrl Pts',(14.8598478861308,31.5652180246215,8.3187913282688));
#52042=CARTESIAN_POINT('Ctrl Pts',(14.860915967039,31.5614789566801,8.31724552153602));
#52043=CARTESIAN_POINT('Ctrl Pts',(14.8788752197154,31.4986083769142,8.29125354518811));
#52044=CARTESIAN_POINT('Ctrl Pts',(14.8971521820891,31.4362355887263,8.26463281026042));
#52045=CARTESIAN_POINT('Ctrl Pts',(14.9157246632579,31.3743466445316,8.23739265459531));
#52046=CARTESIAN_POINT('Ctrl Pts',(14.9544372820573,31.2453448658929,8.18061307018132));
#52047=CARTESIAN_POINT('Ctrl Pts',(14.9944326799355,31.11844401031,8.12114416072383));
#52048=CARTESIAN_POINT('Ctrl Pts',(15.0355234592335,30.9935371441862,8.05904804735394));
#52049=CARTESIAN_POINT('Ctrl Pts',(15.0760595854004,30.8703163007073,7.9977901221201));
#52050=CARTESIAN_POINT('Ctrl Pts',(15.1176617289772,30.7490358453888,7.9339756818053));
#52051=CARTESIAN_POINT('Ctrl Pts',(15.1601642196892,30.6296142683619,7.86763807383431));
#52052=CARTESIAN_POINT('Ctrl Pts',(15.1622801068849,30.6236691441707,7.86433561101518));
#52053=CARTESIAN_POINT('Ctrl Pts',(15.1643982264691,30.6177286273639,7.8610268947962));
#52054=CARTESIAN_POINT('Ctrl Pts',(15.1665185580527,30.6117927080271,7.85771192922444));
#52055=CARTESIAN_POINT('Ctrl Pts',(15.2069899929977,30.4984919511389,7.79443814010604));
#52056=CARTESIAN_POINT('Ctrl Pts',(15.2482654107132,30.3868625031313,7.72889267421188));
#52057=CARTESIAN_POINT('Ctrl Pts',(15.2902163323872,30.2768573280646,7.6610740248339));
#52058=CARTESIAN_POINT('Ctrl Pts',(15.3343650971648,30.1610888918886,7.58970230093732));
#52059=CARTESIAN_POINT('Ctrl Pts',(15.3792620199167,30.0471197248531,7.51581318575337));
#52060=CARTESIAN_POINT('Ctrl Pts',(15.4247582257832,29.9348963054931,7.43940391248849));
#52061=CARTESIAN_POINT('Ctrl Pts',(15.4300526658116,29.9218367513552,7.43051208717671));
#52062=CARTESIAN_POINT('Ctrl Pts',(15.4353552375342,29.908800835701,7.42158612927335));
#52063=CARTESIAN_POINT('Ctrl Pts',(15.440665704816,29.8957884768768,7.41262603449125));
#52064=CARTESIAN_POINT('Ctrl Pts',(15.4809891688668,29.7969829753231,7.34459020248898));
#52065=CARTESIAN_POINT('Ctrl Pts',(15.521768751821,29.6995358217372,7.27458636392175));
#52066=CARTESIAN_POINT('Ctrl Pts',(15.5629098190841,29.6034324184065,7.20258197486916));
#52067=CARTESIAN_POINT('Ctrl Pts',(15.6094690292766,29.4946725136796,7.12109484515398));
#52068=CARTESIAN_POINT('Ctrl Pts',(15.6564915273396,29.3876340000113,7.03704588777083));
#52069=CARTESIAN_POINT('Ctrl Pts',(15.703842272904,29.2822954725418,6.95038626702666));
#52070=CARTESIAN_POINT('Ctrl Pts',(15.7126024692674,29.2628071588042,6.93435367270424));
#52071=CARTESIAN_POINT('Ctrl Pts',(15.7213742769299,29.2433762270171,6.91823105084803));
#52072=CARTESIAN_POINT('Ctrl Pts',(15.7301564025366,29.2240035134661,6.90201887765802));
#52073=CARTESIAN_POINT('Ctrl Pts',(15.7424356426793,29.1969164262891,6.8793508839684));
#52074=CARTESIAN_POINT('Ctrl Pts',(15.7547351390208,29.1699434975136,6.85650729420062));
#52075=CARTESIAN_POINT('Ctrl Pts',(15.7670514039235,29.1430872338644,6.83348906854163));
#52076=CARTESIAN_POINT('Ctrl Pts',(15.769732737634,29.1372404446284,6.82847784599135));
#52077=CARTESIAN_POINT('Ctrl Pts',(15.7724151604062,29.1313985509808,6.82345778883465));
#52078=CARTESIAN_POINT('Ctrl Pts',(15.7750984165171,29.125562052055,6.8184293232226));
#52079=CARTESIAN_POINT('Ctrl Pts',(15.7847409247004,29.1045880986464,6.80035910599041));
#52080=CARTESIAN_POINT('Ctrl Pts',(15.7943975342148,29.0836765829379,6.78217404645932));
#52081=CARTESIAN_POINT('Ctrl Pts',(15.8040544431734,29.0628549878643,6.76389747888537));
#52082=CARTESIAN_POINT('Ctrl Pts',(15.8063269600534,29.0579551356988,6.75959653657584));
#52083=CARTESIAN_POINT('Ctrl Pts',(15.8085992529191,29.0530607734459,6.75529098841496));
#52084=CARTESIAN_POINT('Ctrl Pts',(15.8108712747456,29.0481719632851,6.75098089791873));
#52085=CARTESIAN_POINT('Ctrl Pts',(15.822798101834,29.0225084803134,6.72835536523916));
#52086=CARTESIAN_POINT('Ctrl Pts',(15.8347196337546,28.9969933066434,6.70560053229536));
#52087=CARTESIAN_POINT('Ctrl Pts',(15.8466338279487,28.9716252925335,6.68271643277414));
#52088=CARTESIAN_POINT('Ctrl Pts',(15.8571030335415,28.9493339859734,6.66260778431756));
#52089=CARTESIAN_POINT('Ctrl Pts',(15.8675665712898,28.9271563224226,6.64239933651428));
#52090=CARTESIAN_POINT('Ctrl Pts',(15.878023046609,28.9050915408951,6.62209112555336));
#52091=CARTESIAN_POINT('Ctrl Pts',(15.9151653987023,28.8267154285495,6.54995451174513));
#52092=CARTESIAN_POINT('Ctrl Pts',(15.9522184036771,28.7497626995228,6.47655981315418));
#52093=CARTESIAN_POINT('Ctrl Pts',(15.9891221859866,28.6742076578655,6.40190252027229));
#52094=CARTESIAN_POINT('Ctrl Pts',(16.0011265531405,28.6496304897914,6.37761737933574));
#52095=CARTESIAN_POINT('Ctrl Pts',(16.0131151358443,28.625201237453,6.35319865790895));
#52096=CARTESIAN_POINT('Ctrl Pts',(16.0250858673743,28.6009190188436,6.3286461898737));
#52097=CARTESIAN_POINT('Ctrl Pts',(16.0602757174407,28.5295376141228,6.25647034441588));
#52098=CARTESIAN_POINT('Ctrl Pts',(16.0953109612591,28.4594239273951,6.18314101673159));
#52099=CARTESIAN_POINT('Ctrl Pts',(16.1301419128974,28.3905688719057,6.10864380381399));
#52100=CARTESIAN_POINT('Ctrl Pts',(16.1768215075451,28.2982910004001,6.00880445008361));
#52101=CARTESIAN_POINT('Ctrl Pts',(16.2231343215003,28.2082737170057,5.90686754549628));
#52102=CARTESIAN_POINT('Ctrl Pts',(16.2689599967263,28.1204965528934,5.80279824132711));
#52103=CARTESIAN_POINT('Ctrl Pts',(16.2836188628206,28.0924181080365,5.76950821369913));
#52104=CARTESIAN_POINT('Ctrl Pts',(16.298227901363,28.0645688821045,5.73599997077043));
#52105=CARTESIAN_POINT('Ctrl Pts',(16.3127831594297,28.0369482046737,5.70227232738003));
#52106=CARTESIAN_POINT('Ctrl Pts',(16.3437296833362,27.9782227632899,5.63056261823559));
#52107=CARTESIAN_POINT('Ctrl Pts',(16.374433714844,27.9205304328504,5.5578613637537));
#52108=CARTESIAN_POINT('Ctrl Pts',(16.4048575296364,27.8638776557143,5.48414645965917));
#52109=CARTESIAN_POINT('Ctrl Pts',(16.4495907536865,27.7805790493436,5.375760797204));
#52110=CARTESIAN_POINT('Ctrl Pts',(16.4937185698648,27.6995280587495,5.26518414921598));
#52111=CARTESIAN_POINT('Ctrl Pts',(16.5371206449052,27.6207461836642,5.15234532909353));
#52112=CARTESIAN_POINT('Ctrl Pts',(16.553707506264,27.5906383135126,5.10922200230507));
#52113=CARTESIAN_POINT('Ctrl Pts',(16.5701882618752,27.5608617830849,5.0657681510329));
#52114=CARTESIAN_POINT('Ctrl Pts',(16.5865561886659,27.5314178413183,5.02197974299201));
#52115=CARTESIAN_POINT('Ctrl Pts',(16.6130174609297,27.4838171787808,4.95118904347443));
#52116=CARTESIAN_POINT('Ctrl Pts',(16.6391837396048,27.4370877369798,4.87952226067709));
#52117=CARTESIAN_POINT('Ctrl Pts',(16.665025217884,27.391242590013,4.8069553183639));
#52118=CARTESIAN_POINT('',(33.,27.3912430012986,4.80695505852859));
#52119=CARTESIAN_POINT('',(33.,27.3912430012986,4.80695505852859));
#52120=CARTESIAN_POINT('',(33.,26.2716828895474,2.19464813110884));
#52121=CARTESIAN_POINT('Origin',(33.,35.,5.81688018065629E-15));
#52122=CARTESIAN_POINT('',(33.,26.2716828895474,2.19464813110884));
#52123=CARTESIAN_POINT('Origin',(-37.5,48.4656487624794,-19.0077234952746));
#52124=CARTESIAN_POINT('',(-37.,47.5792333881917,-19.4706141780782));
#52125=CARTESIAN_POINT('',(-37.5,48.0436073736659,-18.7396170497563));
#52126=CARTESIAN_POINT('Ctrl Pts',(-37.5,48.0436073736659,-18.7396170497564));
#52127=CARTESIAN_POINT('Ctrl Pts',(-37.3614508889595,47.9693155542843,-18.8565639682411));
#52128=CARTESIAN_POINT('Ctrl Pts',(-37.1980436419056,47.8786620489552,-18.9992667339876));
#52129=CARTESIAN_POINT('Ctrl Pts',(-37.0447859999489,47.7259734976123,-19.2396223440145));
#52130=CARTESIAN_POINT('Ctrl Pts',(-37.,47.6475676678136,-19.3630453569726));
#52131=CARTESIAN_POINT('Ctrl Pts',(-37.,47.5792333881917,-19.4706141780782));
#52132=CARTESIAN_POINT('',(-37.,49.0018616535158,-18.1636407176477));
#52133=CARTESIAN_POINT('Origin',(-37.,48.4656487624794,-19.0077234952746));
#52134=CARTESIAN_POINT('',(-37.5,48.7337552079976,-18.5856821064611));
#52135=CARTESIAN_POINT('Origin',(-37.5,49.0018616535158,-18.1636407176477));
#52136=CARTESIAN_POINT('Origin',(-37.5,48.4656487624794,-19.0077234952746));
#52137=CARTESIAN_POINT('Origin',(3.49012810839377E-15,57.,-2.60208521396521E-14));
#52138=CARTESIAN_POINT('',(3.03365373473698E-15,20.5440037453175,14.5));
#52139=CARTESIAN_POINT('Origin',(1.25791587597333E-15,20.5440037453175,
-6.04998712603518E-15));
#52140=CARTESIAN_POINT('',(5.26586596715743E-15,57.,14.5));
#52141=CARTESIAN_POINT('',(5.26586596715743E-15,57.,14.5));
#52142=CARTESIAN_POINT('Origin',(3.49012810839377E-15,57.,-2.60208521396521E-14));
#52143=CARTESIAN_POINT('',(-14.5,38.9999999945948,6.54987201765396E-10));
#52144=CARTESIAN_POINT('',(-14.5,30.9999999945948,6.54993427017253E-10));
#52145=CARTESIAN_POINT('Ctrl Pts',(-14.5,38.9999999945948,6.54994392057517E-10));
#52146=CARTESIAN_POINT('Ctrl Pts',(-14.5000000000228,38.9999999945948,-0.505032330715858));
#52147=CARTESIAN_POINT('Ctrl Pts',(-14.4709879985074,38.8985352188743,-1.04196886987578));
#52148=CARTESIAN_POINT('Ctrl Pts',(-14.3661925074414,38.4894942453939,-2.0267475502792));
#52149=CARTESIAN_POINT('Ctrl Pts',(-14.2917945289831,38.1820590487641,-2.47479519466809));
#52150=CARTESIAN_POINT('Ctrl Pts',(-14.1511159999958,37.4747208857634,-3.18213335766881));
#52151=CARTESIAN_POINT('Ctrl Pts',(-14.0754408854234,37.0267038181377,-3.48951080938327));
#52152=CARTESIAN_POINT('Ctrl Pts',(-13.9676894199724,36.0420348868828,-3.8985094040844));
#52153=CARTESIAN_POINT('Ctrl Pts',(-13.9373598649543,35.5051384419502,-3.99999999934501));
#52154=CARTESIAN_POINT('Ctrl Pts',(-13.9373598649543,34.4948615472385,-3.99999999934501));
#52155=CARTESIAN_POINT('Ctrl Pts',(-13.9676894199725,33.9579651023051,-3.89850940408406));
#52156=CARTESIAN_POINT('Ctrl Pts',(-14.0754408854238,32.973296171049,-3.48951080938169));
#52157=CARTESIAN_POINT('Ctrl Pts',(-14.1511159999964,32.5252791034228,-3.18213335766633));
#52158=CARTESIAN_POINT('Ctrl Pts',(-14.2917945289836,31.817940940423,-2.47479519466472));
#52159=CARTESIAN_POINT('Ctrl Pts',(-14.3661925074417,31.5105057437941,-2.02674755027626));
#52160=CARTESIAN_POINT('Ctrl Pts',(-14.4709879985075,31.1014647703149,-1.04196886987411));
#52161=CARTESIAN_POINT('Ctrl Pts',(-14.5000000000228,30.9999999945948,-0.505032330715019));
#52162=CARTESIAN_POINT('Ctrl Pts',(-14.5,30.9999999945948,6.5499272672298E-10));
#52163=CARTESIAN_POINT('Ctrl Pts',(-14.5,30.9999999945948,6.54993420612371E-10));
#52164=CARTESIAN_POINT('Ctrl Pts',(-14.4999999999772,30.9999999945948,0.505032332030019));
#52165=CARTESIAN_POINT('Ctrl Pts',(-14.4709879984128,31.1014647703167,1.04196887119144));
#52166=CARTESIAN_POINT('Ctrl Pts',(-14.3661925072559,31.5105057437989,2.02674755159486));
#52167=CARTESIAN_POINT('Ctrl Pts',(-14.2917945287556,31.8179409404289,2.4747951959824));
#52168=CARTESIAN_POINT('Ctrl Pts',(-14.1511159997011,32.5252791034279,3.18213335897963));
#52169=CARTESIAN_POINT('Ctrl Pts',(-14.0754408850987,32.9732961710517,3.48951081069302));
#52170=CARTESIAN_POINT('Ctrl Pts',(-13.967689419607,33.9579651023049,3.89850940539377));
#52171=CARTESIAN_POINT('Ctrl Pts',(-13.9373598645784,34.4948615472378,4.000000000655));
#52172=CARTESIAN_POINT('Ctrl Pts',(-13.9373598645784,34.9999999945948,4.000000000655));
#52173=CARTESIAN_POINT('Ctrl Pts',(-13.9373598645784,35.5051384419526,4.000000000655));
#52174=CARTESIAN_POINT('Ctrl Pts',(-13.9676894196071,36.0420348868864,3.89850940539344));
#52175=CARTESIAN_POINT('Ctrl Pts',(-14.0754408850991,37.0267038181408,3.48951081069144));
#52176=CARTESIAN_POINT('Ctrl Pts',(-14.1511159997017,37.474720885765,3.18213335897715));
#52177=CARTESIAN_POINT('Ctrl Pts',(-14.2917945287562,38.1820590487631,2.47479519597904));
#52178=CARTESIAN_POINT('Ctrl Pts',(-14.3661925072563,38.4894942453923,2.02674755159192));
#52179=CARTESIAN_POINT('Ctrl Pts',(-14.4709879984129,38.8985352188732,1.04196887118977));
#52180=CARTESIAN_POINT('Ctrl Pts',(-14.4999999999772,38.9999999945948,0.505032332029179));
#52181=CARTESIAN_POINT('Ctrl Pts',(-14.5,38.9999999945948,6.54993420612371E-10));
#52182=CARTESIAN_POINT('',(14.5,38.9999999945947,6.54966782784404E-10));
#52183=CARTESIAN_POINT('',(14.5,30.9999999945948,6.54993843350887E-10));
#52184=CARTESIAN_POINT('Ctrl Pts',(14.5,38.9999999945948,6.54992587945102E-10));
#52185=CARTESIAN_POINT('Ctrl Pts',(14.4999999999772,38.9999999945948,0.505032332030019));
#52186=CARTESIAN_POINT('Ctrl Pts',(14.4709879984128,38.8985352188729,1.04196887119144));
#52187=CARTESIAN_POINT('Ctrl Pts',(14.3661925072559,38.4894942453907,2.02674755159486));
#52188=CARTESIAN_POINT('Ctrl Pts',(14.2917945287556,38.1820590487606,2.4747951959824));
#52189=CARTESIAN_POINT('Ctrl Pts',(14.1511159997011,37.4747208857617,3.18213335897963));
#52190=CARTESIAN_POINT('Ctrl Pts',(14.0754408850987,37.0267038181379,3.48951081069302));
#52191=CARTESIAN_POINT('Ctrl Pts',(13.967689419607,36.0420348868847,3.89850940539377));
#52192=CARTESIAN_POINT('Ctrl Pts',(13.9373598645784,35.5051384419518,4.000000000655));
#52193=CARTESIAN_POINT('Ctrl Pts',(13.9373598645784,34.9999999945948,4.000000000655));
#52194=CARTESIAN_POINT('Ctrl Pts',(13.9373598645784,34.4948615472378,4.000000000655));
#52195=CARTESIAN_POINT('Ctrl Pts',(13.967689419607,33.9579651023049,3.89850940539377));
#52196=CARTESIAN_POINT('Ctrl Pts',(14.0754408850987,32.9732961710517,3.48951081069302));
#52197=CARTESIAN_POINT('Ctrl Pts',(14.1511159997011,32.5252791034279,3.18213335897963));
#52198=CARTESIAN_POINT('Ctrl Pts',(14.2917945287556,31.8179409404289,2.4747951959824));
#52199=CARTESIAN_POINT('Ctrl Pts',(14.3661925072559,31.5105057437989,2.02674755159486));
#52200=CARTESIAN_POINT('Ctrl Pts',(14.4709879984128,31.1014647703167,1.04196887119144));
#52201=CARTESIAN_POINT('Ctrl Pts',(14.4999999999772,30.9999999945948,0.50503233203002));
#52202=CARTESIAN_POINT('Ctrl Pts',(14.5,30.9999999945948,6.54994253279639E-10));
#52203=CARTESIAN_POINT('Ctrl Pts',(14.5,30.9999999945948,6.54993975723883E-10));
#52204=CARTESIAN_POINT('Ctrl Pts',(14.5000000000228,30.9999999945948,-0.505032330715018));
#52205=CARTESIAN_POINT('Ctrl Pts',(14.4709879985075,31.1014647703149,-1.04196886987411));
#52206=CARTESIAN_POINT('Ctrl Pts',(14.3661925074417,31.5105057437941,-2.02674755027626));
#52207=CARTESIAN_POINT('Ctrl Pts',(14.2917945289836,31.817940940423,-2.47479519466472));
#52208=CARTESIAN_POINT('Ctrl Pts',(14.1511159999964,32.5252791034228,-3.18213335766633));
#52209=CARTESIAN_POINT('Ctrl Pts',(14.0754408854238,32.973296171049,-3.48951080938169));
#52210=CARTESIAN_POINT('Ctrl Pts',(13.9676894199725,33.9579651023051,-3.89850940408406));
#52211=CARTESIAN_POINT('Ctrl Pts',(13.9373598649543,34.4948615472385,-3.99999999934501));
#52212=CARTESIAN_POINT('Ctrl Pts',(13.9373598649543,35.5051384419511,-3.99999999934501));
#52213=CARTESIAN_POINT('Ctrl Pts',(13.9676894199725,36.0420348868845,-3.89850940408406));
#52214=CARTESIAN_POINT('Ctrl Pts',(14.0754408854238,37.0267038181406,-3.48951080938169));
#52215=CARTESIAN_POINT('Ctrl Pts',(14.1511159999964,37.4747208857667,-3.18213335766633));
#52216=CARTESIAN_POINT('Ctrl Pts',(14.2917945289836,38.1820590487666,-2.47479519466473));
#52217=CARTESIAN_POINT('Ctrl Pts',(14.3661925074418,38.4894942453955,-2.02674755027626));
#52218=CARTESIAN_POINT('Ctrl Pts',(14.4709879985075,38.8985352188747,-1.0419688698741));
#52219=CARTESIAN_POINT('Ctrl Pts',(14.5000000000228,38.9999999945948,-0.505032330715019));
#52220=CARTESIAN_POINT('Ctrl Pts',(14.5,38.9999999945948,6.5499272672298E-10));
#52221=CARTESIAN_POINT('Ctrl Pts',(0.321034048597817,44.2777095070773,-16.496876587392));
#52222=CARTESIAN_POINT('Ctrl Pts',(0.334078182671872,44.0705712895835,-16.4966227447236));
#52223=CARTESIAN_POINT('Ctrl Pts',(0.346147593727982,43.9243235322772,-16.6433959637249));
#52224=CARTESIAN_POINT('Ctrl Pts',(0.307535768851996,44.2768333852379,-16.497139267868));
#52225=CARTESIAN_POINT('Ctrl Pts',(0.32115157242211,44.0697030498192,-16.4968849768605));
#52226=CARTESIAN_POINT('Ctrl Pts',(0.333504576783726,43.9234749343164,-16.6436941271133));
#52227=CARTESIAN_POINT('Ctrl Pts',(0.294017346932686,44.2758981934479,-16.4973857263738));
#52228=CARTESIAN_POINT('Ctrl Pts',(0.308206040614918,44.0687776043361,-16.4971323872042));
#52229=CARTESIAN_POINT('Ctrl Pts',(0.320842694094729,43.9225707071434,-16.6439790196373));
#52230=CARTESIAN_POINT('Ctrl Pts',(0.267039396841221,44.27391662747,-16.4978444642199));
#52231=CARTESIAN_POINT('Ctrl Pts',(0.282371646107752,44.0668191614445,-16.4975958245399));
#52232=CARTESIAN_POINT('Ctrl Pts',(0.295574090707277,43.9206577286911,-16.6445202461941));
#52233=CARTESIAN_POINT('Ctrl Pts',(0.253563318677811,44.2728691821441,-16.4980570656251));
#52234=CARTESIAN_POINT('Ctrl Pts',(0.269466916331725,44.0657850965016,-16.4978121729084));
#52235=CARTESIAN_POINT('Ctrl Pts',(0.282951868731823,43.9196479380401,-16.644776944703));
#52236=CARTESIAN_POINT('Ctrl Pts',(0.213173600931101,44.2695576149692,-16.4986448596443));
#52237=CARTESIAN_POINT('Ctrl Pts',(0.230789208343801,44.0625190499157,-16.4984153937458));
#52238=CARTESIAN_POINT('Ctrl Pts',(0.245121279113449,43.9164593690092,-16.6455055488628));
#52239=CARTESIAN_POINT('Ctrl Pts',(0.186298475258698,44.2671242747577,-16.4989700430965));
#52240=CARTESIAN_POINT('Ctrl Pts',(0.205054254630706,44.0601233301731,-16.4987564104361));
#52241=CARTESIAN_POINT('Ctrl Pts',(0.219948985085661,43.9141214063132,-16.6459359637993));
#52242=CARTESIAN_POINT('Ctrl Pts',(0.105825878010724,44.2591529071548,-16.4997478557418));
#52243=CARTESIAN_POINT('Ctrl Pts',(0.127994124910921,44.0522861114256,-16.4995982912245));
#52244=CARTESIAN_POINT('Ctrl Pts',(0.144575202554741,43.906475946942,-16.6470632548686));
#52245=CARTESIAN_POINT('Ctrl Pts',(0.0523811410166356,44.2529437369118,
-16.5000027615431));
#52246=CARTESIAN_POINT('Ctrl Pts',(0.0768198248561238,44.0461951243862,
-16.4999178604957));
#52247=CARTESIAN_POINT('Ctrl Pts',(0.0945167711882191,43.9005370741829,
-16.6475961824246));
#52248=CARTESIAN_POINT('Ctrl Pts',(-0.107350614477069,44.2316680864431,
-16.4999944092424));
#52249=CARTESIAN_POINT('Ctrl Pts',(-0.0761321294294826,44.0253574854767,
-16.5001684527276));
#52250=CARTESIAN_POINT('Ctrl Pts',(-0.0550942394312359,43.8802288896034,
-16.6485550431313));
#52251=CARTESIAN_POINT('Ctrl Pts',(-0.213035833808924,44.2139564350666,
-16.4989582457926));
#52252=CARTESIAN_POINT('Ctrl Pts',(-0.177314759062477,44.0080500010336,
-16.4993908078766));
#52253=CARTESIAN_POINT('Ctrl Pts',(-0.154083150146027,43.8633708391614,
-16.6483410814393));
#52254=CARTESIAN_POINT('Ctrl Pts',(-0.422829790157967,44.1715971665048,
-16.4949150477184));
#52255=CARTESIAN_POINT('Ctrl Pts',(-0.378133313017958,43.9667246375007,
-16.4960324415121));
#52256=CARTESIAN_POINT('Ctrl Pts',(-0.350584376434533,43.8231263425323,
-16.6462901344215));
#52257=CARTESIAN_POINT('Ctrl Pts',(-0.526938468414131,44.1469492910955,
-16.491907937397));
#52258=CARTESIAN_POINT('Ctrl Pts',(-0.477778440005314,43.9427009960084,
-16.4934505609926));
#52259=CARTESIAN_POINT('Ctrl Pts',(-0.448096637091592,43.7997396541264,
-16.6444530862772));
#52260=CARTESIAN_POINT('Ctrl Pts',(-0.733587594662706,44.0907445802113,
-16.4840086388606));
#52261=CARTESIAN_POINT('Ctrl Pts',(-0.675522285528619,43.8879685573675,
-16.4865649802999));
#52262=CARTESIAN_POINT('Ctrl Pts',(-0.641652292512058,43.7464596423238,
-16.6392391144044));
#52263=CARTESIAN_POINT('Ctrl Pts',(-0.836128020523552,44.0591876523663,
-16.4791163820797));
#52264=CARTESIAN_POINT('Ctrl Pts',(-0.773630842788747,43.85725253155,-16.4822597770412));
#52265=CARTESIAN_POINT('Ctrl Pts',(-0.737695666593328,43.7165662342863,
-16.6358621269656));
#52266=CARTESIAN_POINT('Ctrl Pts',(-0.988754343263762,44.0066257334661,
-16.4704268781621));
#52267=CARTESIAN_POINT('Ctrl Pts',(-0.919592667679679,43.8061296100387,
-16.4745719708769));
#52268=CARTESIAN_POINT('Ctrl Pts',(-0.880651450997229,43.6668004399974,
-16.62970542955));
#52269=CARTESIAN_POINT('Ctrl Pts',(-1.03943225076959,43.988233336078,-16.4673051794513));
#52270=CARTESIAN_POINT('Ctrl Pts',(-0.968061533919264,43.7882402439072,
-16.471803341561));
#52271=CARTESIAN_POINT('Ctrl Pts',(-0.92811836158864,43.6493902559039,-16.6274713470767));
#52272=CARTESIAN_POINT('Ctrl Pts',(-1.11515046567206,43.9593254565497,-16.462292648905));
#52273=CARTESIAN_POINT('Ctrl Pts',(-1.04046157511159,43.760131242437,-16.4673503544702));
#52274=CARTESIAN_POINT('Ctrl Pts',(-0.999039003666644,43.6220311175392,
-16.6238556629229));
#52275=CARTESIAN_POINT('Ctrl Pts',(-1.14034008702055,43.9494695740836,-16.4605668083992));
#52276=CARTESIAN_POINT('Ctrl Pts',(-1.06454821112494,43.7505474186053,-16.4658157518771));
#52277=CARTESIAN_POINT('Ctrl Pts',(-1.02263258838498,43.6127040541935,-16.6226063432779));
#52278=CARTESIAN_POINT('Ctrl Pts',(-1.19061925892548,43.9293155100069,-16.4570064394505));
#52279=CARTESIAN_POINT('Ctrl Pts',(-1.11262228707775,43.7309512076575,-16.4626476168865));
#52280=CARTESIAN_POINT('Ctrl Pts',(-1.06972602765263,43.5936328230074,-16.6200209173139));
#52281=CARTESIAN_POINT('Ctrl Pts',(-1.21573107838862,43.9190077883623,-16.4551701883059));
#52282=CARTESIAN_POINT('Ctrl Pts',(-1.13663118653057,43.7209293797071,-16.4610125155677));
#52283=CARTESIAN_POINT('Ctrl Pts',(-1.09324674012034,43.5838796294641,-16.618683550189));
#52284=CARTESIAN_POINT('Ctrl Pts',(-1.3406740926079,43.8665114056024,-16.4457484072491));
#52285=CARTESIAN_POINT('Ctrl Pts',(-1.25611592982861,43.6698761529651,-16.4526150324278));
#52286=CARTESIAN_POINT('Ctrl Pts',(-1.21027325465697,43.5342106859547,-16.6118037002477));
#52287=CARTESIAN_POINT('Ctrl Pts',(-1.43874378672612,43.8214268381111,-16.4374378027854));
#52288=CARTESIAN_POINT('Ctrl Pts',(-1.34984750421121,43.6260493224596,-16.445193094768));
#52289=CARTESIAN_POINT('Ctrl Pts',(-1.3021291667423,43.4915646194171,-16.6056797596469));
#52290=CARTESIAN_POINT('Ctrl Pts',(-1.72749788443196,43.6771991720061,-16.4104580032492));
#52291=CARTESIAN_POINT('Ctrl Pts',(-1.62585456299005,43.4858144841423,-16.4210581992283));
#52292=CARTESIAN_POINT('Ctrl Pts',(-1.5725875499331,43.3551562723534,-16.5857017103286));
#52293=CARTESIAN_POINT('Ctrl Pts',(-1.9127446936616,43.5691113883,-16.3897439917078));
#52294=CARTESIAN_POINT('Ctrl Pts',(-1.80274205830027,43.3807393221566,-16.4024878858354));
#52295=CARTESIAN_POINT('Ctrl Pts',(-1.74609695837727,43.2529516481594,-16.5702431598975));
#52296=CARTESIAN_POINT('Ctrl Pts',(-2.1801557392676,43.3896071926388,-16.3555799666888));
#52297=CARTESIAN_POINT('Ctrl Pts',(-2.05760446502451,43.2064579036073,-16.3718931324892));
#52298=CARTESIAN_POINT('Ctrl Pts',(-1.99656460420932,43.0832067018407,-16.5448031114995));
#52299=CARTESIAN_POINT('Ctrl Pts',(-2.26754491058278,43.3268692367125,-16.3436754924434));
#52300=CARTESIAN_POINT('Ctrl Pts',(-2.14090553035905,43.1454987345458,-16.3612235417513));
#52301=CARTESIAN_POINT('Ctrl Pts',(-2.07841672068826,43.0238779812105,-16.5359471304104));
#52302=CARTESIAN_POINT('Ctrl Pts',(-2.39602241125449,43.2284104250473,-16.3251630538784));
#52303=CARTESIAN_POINT('Ctrl Pts',(-2.26324112913542,43.0498815519994,-16.3446457798798));
#52304=CARTESIAN_POINT('Ctrl Pts',(-2.19875377361068,42.9307615436581,-16.5222160833336));
#52305=CARTESIAN_POINT('Ctrl Pts',(-2.4384136297981,43.1948651021794,-16.3188829280199));
#52306=CARTESIAN_POINT('Ctrl Pts',(-2.30360778271325,43.0172911666837,-16.3390206470251));
#52307=CARTESIAN_POINT('Ctrl Pts',(-2.23845904720143,42.8990351188427,-16.5175645484453));
#52308=CARTESIAN_POINT('Ctrl Pts',(-2.5013483955168,43.1434553651894,-16.3093134885055));
#52309=CARTESIAN_POINT('Ctrl Pts',(-2.36350239470388,42.9673565647272,-16.3304535133341));
#52310=CARTESIAN_POINT('Ctrl Pts',(-2.29740621067309,42.8504103436033,-16.5104900878419));
#52311=CARTESIAN_POINT('Ctrl Pts',(-2.52221795974619,43.1261368034609,-16.3060987995381));
#52312=CARTESIAN_POINT('Ctrl Pts',(-2.38336413494237,42.9505314385688,-16.3275753119188));
#52313=CARTESIAN_POINT('Ctrl Pts',(-2.31695346092089,42.8340295394261,-16.508115741492));
#52314=CARTESIAN_POINT('Ctrl Pts',(-2.56373951624231,43.0911348998851,-16.2996221180008));
#52315=CARTESIAN_POINT('Ctrl Pts',(-2.42287279694903,42.9165270650644,-16.321777494731));
#52316=CARTESIAN_POINT('Ctrl Pts',(-2.3558441749912,42.8009219471062,-16.5033371082496));
#52317=CARTESIAN_POINT('Ctrl Pts',(-2.58440772848289,43.0734372910358,-16.2963575090795));
#52318=CARTESIAN_POINT('Ctrl Pts',(-2.44253529767474,42.8993336069646,-16.3188554855158));
#52319=CARTESIAN_POINT('Ctrl Pts',(-2.37520283114705,42.7841816631336,-16.5009308965196));
#52320=CARTESIAN_POINT('Ctrl Pts',(-2.76898876271576,42.9129091805958,-16.2668469274607));
#52321=CARTESIAN_POINT('Ctrl Pts',(-2.61835540789446,42.7431513199272,-16.2924080344925));
#52322=CARTESIAN_POINT('Ctrl Pts',(-2.54808864778449,42.6323323225514,-16.4792048254679));
#52323=CARTESIAN_POINT('Ctrl Pts',(-2.92301708649477,42.7613001461326,-16.2396947338131));
#52324=CARTESIAN_POINT('Ctrl Pts',(-2.76462847126197,42.5957682985728,-16.2681310777436));
#52325=CARTESIAN_POINT('Ctrl Pts',(-2.69235760204375,42.488886199182,-16.4593927479317));
#52326=CARTESIAN_POINT('Ctrl Pts',(-3.21259129366432,42.4414613853005,-16.1848994780706));
#52327=CARTESIAN_POINT('Ctrl Pts',(-3.03897378350019,42.2850128986459,-16.2192940222789));
#52328=CARTESIAN_POINT('Ctrl Pts',(-2.96358413143859,42.1861517320565,-16.4200413247235));
#52329=CARTESIAN_POINT('Ctrl Pts',(-3.34812899112022,42.2732247223232,-16.1572537757578));
#52330=CARTESIAN_POINT('Ctrl Pts',(-3.16707816112672,42.1214334676319,-16.1947098049125));
#52331=CARTESIAN_POINT('Ctrl Pts',(-3.09053404151204,42.0268568930642,-16.4004996968118));
#52332=CARTESIAN_POINT('Ctrl Pts',(-3.53828868842179,42.0088979382797,-16.1162873356813));
#52333=CARTESIAN_POINT('Ctrl Pts',(-3.34597462567252,41.8649168770618,-16.1584948890192));
#52334=CARTESIAN_POINT('Ctrl Pts',(-3.26864505239508,41.7764635010048,-16.3722252421456));
#52335=CARTESIAN_POINT('Ctrl Pts',(-3.5994799346103,41.9187901440346,-16.1027143504919));
#52336=CARTESIAN_POINT('Ctrl Pts',(-3.40351260983138,41.7773425460961,-16.1465055224545));
#52337=CARTESIAN_POINT('Ctrl Pts',(-3.32595916749315,41.6910871652366,-16.362972412406));
#52338=CARTESIAN_POINT('Ctrl Pts',(-3.67327289887432,41.8036856256223,-16.0859347036074));
#52339=CARTESIAN_POINT('Ctrl Pts',(-3.47268299468521,41.6656131275086,-16.1317391824527));
#52340=CARTESIAN_POINT('Ctrl Pts',(-3.3950765443778,41.5820004939642,-16.3517021387782));
#52341=CARTESIAN_POINT('Ctrl Pts',(-3.68790324489889,41.7805305132082,-16.0825865601582));
#52342=CARTESIAN_POINT('Ctrl Pts',(-3.48640397870713,41.6431129782816,-16.1287915877042));
#52343=CARTESIAN_POINT('Ctrl Pts',(-3.40877989888389,41.5600546868429,-16.3494618416137));
#52344=CARTESIAN_POINT('Ctrl Pts',(-3.71686467531462,41.7340227710879,-16.0759179456141));
#52345=CARTESIAN_POINT('Ctrl Pts',(-3.51355022417322,41.5979213056804,-16.122924842068));
#52346=CARTESIAN_POINT('Ctrl Pts',(-3.43590630737669,41.5159732371528,-16.3450174403968));
#52347=CARTESIAN_POINT('Ctrl Pts',(-3.73118318182571,41.7106906886745,-16.0726003938663));
#52348=CARTESIAN_POINT('Ctrl Pts',(-3.52696370022908,41.5752492629553,-16.1200082324879));
#52349=CARTESIAN_POINT('Ctrl Pts',(-3.44931758085173,41.493857071485,-16.3428152733996));
#52350=CARTESIAN_POINT('Ctrl Pts',(-3.77365910783509,41.6404628298273,-16.0627003448006));
#52351=CARTESIAN_POINT('Ctrl Pts',(-3.56674649451528,41.5069837011863,-16.1113077604514));
#52352=CARTESIAN_POINT('Ctrl Pts',(-3.48910219450987,41.427285026544,-16.3362710369363));
#52353=CARTESIAN_POINT('Ctrl Pts',(-3.80133703055952,41.5933354841588,-16.0561704793561));
#52354=CARTESIAN_POINT('Ctrl Pts',(-3.59262873818026,41.4611883744804,-16.105579589636));
#52355=CARTESIAN_POINT('Ctrl Pts',(-3.51502641995466,41.3826056395206,-16.3319912551902));
#52356=CARTESIAN_POINT('Ctrl Pts',(-3.93661737229858,41.3561924516797,-16.0239016028219));
#52357=CARTESIAN_POINT('Ctrl Pts',(-3.71926534359318,41.2302267666986,-16.0772522172006));
#52358=CARTESIAN_POINT('Ctrl Pts',(-3.64173527925152,41.1577530499255,-16.3110349773682));
#52359=CARTESIAN_POINT('Ctrl Pts',(-4.03491747293985,41.1616690216634,-15.9993106710039));
#52360=CARTESIAN_POINT('Ctrl Pts',(-3.8105351856191,41.0410889990247,-16.0558581848326));
#52361=CARTESIAN_POINT('Ctrl Pts',(-3.73380699989436,40.9732232360452,-16.2956924811267));
#52362=CARTESIAN_POINT('Ctrl Pts',(-4.21346560575097,40.7637707951905,-15.9532193788555));
#52363=CARTESIAN_POINT('Ctrl Pts',(-3.97517918815052,40.6545075845859,-16.0161173849287));
#52364=CARTESIAN_POINT('Ctrl Pts',(-3.90104216471963,40.5955698374873,-16.2684493117706));
#52365=CARTESIAN_POINT('Ctrl Pts',(-4.29370773194948,40.5603934046897,-15.9317175178876));
#52366=CARTESIAN_POINT('Ctrl Pts',(-4.04850396862992,40.4567958249106,-15.9977704901831));
#52367=CARTESIAN_POINT('Ctrl Pts',(-3.97620007983221,40.4024438484038,-16.2565472800635));
#52368=CARTESIAN_POINT('Ctrl Pts',(-4.40146481480481,40.2490824569658,-15.9021537778166));
#52369=CARTESIAN_POINT('Ctrl Pts',(-4.14571728004939,40.1550827275247,-15.9729333571334));
#52370=CARTESIAN_POINT('Ctrl Pts',(-4.0771295784449,40.1066679258703,-16.2416226946648));
#52371=CARTESIAN_POINT('Ctrl Pts',(-4.43527916848801,40.1442697315678,-15.8927463879809));
#52372=CARTESIAN_POINT('Ctrl Pts',(-4.17607991924084,40.0532812588022,-15.965075967575));
#52373=CARTESIAN_POINT('Ctrl Pts',(-4.10880142516048,40.007059981848,-16.2371350135424));
#52374=CARTESIAN_POINT('Ctrl Pts',(-4.47498970331547,40.0119814226891,-15.8815784864466));
#52375=CARTESIAN_POINT('Ctrl Pts',(-4.21141132770978,39.9250565429304,-15.955847181276));
#52376=CARTESIAN_POINT('Ctrl Pts',(-4.14599586533176,39.8813077925278,-16.2321648104482));
#52377=CARTESIAN_POINT('Ctrl Pts',(-4.48280713505993,39.9854484820733,-15.8793735332333));
#52378=CARTESIAN_POINT('Ctrl Pts',(-4.21836394867178,39.8992957517518,-15.9540264515764));
#52379=CARTESIAN_POINT('Ctrl Pts',(-4.15331797782398,39.8560841569777,-16.2312023454786));
#52380=CARTESIAN_POINT('Ctrl Pts',(-4.49815720553132,39.9323631382508,-15.8750321376815));
#52381=CARTESIAN_POINT('Ctrl Pts',(-4.23198682506552,39.8477579670653,-15.9504505711255));
#52382=CARTESIAN_POINT('Ctrl Pts',(-4.16769545413477,39.805615099322,-16.2293456787121));
#52383=CARTESIAN_POINT('Ctrl Pts',(-4.50569299128003,39.9058006819841,-15.8728948158664));
#52384=CARTESIAN_POINT('Ctrl Pts',(-4.23865969846769,39.8219707212385,-15.9486947308374));
#52385=CARTESIAN_POINT('Ctrl Pts',(-4.1747537660165,39.7803601224423,-16.2284510688984));
#52386=CARTESIAN_POINT('Ctrl Pts',(-4.52788908225558,39.8260548181995,-15.8665830325155));
#52387=CARTESIAN_POINT('Ctrl Pts',(-4.25828083324603,39.7445109973632,-15.9435203785516));
#52388=CARTESIAN_POINT('Ctrl Pts',(-4.19554349286319,39.7045346637349,-16.2258684245472));
#52389=CARTESIAN_POINT('Ctrl Pts',(-4.54213820519509,39.7728129265089,-15.8625087615832));
#52390=CARTESIAN_POINT('Ctrl Pts',(-4.27080745248769,39.6928283677743,-15.9402013833087));
#52391=CARTESIAN_POINT('Ctrl Pts',(-4.20888977911923,39.6539036641976,-16.2242815829051));
#52392=CARTESIAN_POINT('Ctrl Pts',(-4.61072350551952,39.5062243012366,-15.8428055513534));
#52393=CARTESIAN_POINT('Ctrl Pts',(-4.33101064476337,39.4331423066517,-15.9241892497505));
#52394=CARTESIAN_POINT('Ctrl Pts',(-4.27312945361112,39.4003554433727,-16.2170217104017));
#52395=CARTESIAN_POINT('Ctrl Pts',(-4.65710151667135,39.2917430094221,-15.8291830985343));
#52396=CARTESIAN_POINT('Ctrl Pts',(-4.37047377111817,39.2249262086857,-15.9134966630587));
#52397=CARTESIAN_POINT('Ctrl Pts',(-4.3165689141374,39.1962612675561,-16.2133735716419));
#52398=CARTESIAN_POINT('Ctrl Pts',(-4.73455890330831,38.860584008785,-15.8061881582692));
#52399=CARTESIAN_POINT('Ctrl Pts',(-4.43416228480996,38.806836206605,-15.8961542515918));
#52400=CARTESIAN_POINT('Ctrl Pts',(-4.38911853157358,38.7857773011577,-16.2103568495108));
#52401=CARTESIAN_POINT('Ctrl Pts',(-4.7656335172996,38.6439056908728,-15.7968150887316));
#52402=CARTESIAN_POINT('Ctrl Pts',(-4.45824992940577,38.596715083291,-15.8895386759589));
#52403=CARTESIAN_POINT('Ctrl Pts',(-4.41822423140701,38.5793869570085,-16.2109877211159));
#52404=CARTESIAN_POINT('Ctrl Pts',(-4.81366277021719,38.2085119119448,-15.7822457370113));
#52405=CARTESIAN_POINT('Ctrl Pts',(-4.49228715046657,38.1750784013236,-15.8802583836643));
#52406=CARTESIAN_POINT('Ctrl Pts',(-4.46321030786492,38.1644661155498,-16.2164498115114));
#52407=CARTESIAN_POINT('Ctrl Pts',(-4.83061473177268,37.989796110882,-15.7770490650161));
#52408=CARTESIAN_POINT('Ctrl Pts',(-4.50207912059962,37.963297937123,-15.8776364690345));
#52409=CARTESIAN_POINT('Ctrl Pts',(-4.47908817873774,37.9559353121758,-16.2212806621887));
#52410=CARTESIAN_POINT('Ctrl Pts',(-4.85119740418559,37.5504372754616,-15.7707323746352));
#52411=CARTESIAN_POINT('Ctrl Pts',(-4.50825772146479,37.5385831425256,-15.8762196986871));
#52412=CARTESIAN_POINT('Ctrl Pts',(-4.49836671444632,37.5368431558517,-16.2350392361057));
#52413=CARTESIAN_POINT('Ctrl Pts',(-4.85482680237322,37.3297940775806,-15.7696120833341));
#52414=CARTESIAN_POINT('Ctrl Pts',(-4.50446088793284,37.3253626831583,-15.8774765117451));
#52415=CARTESIAN_POINT('Ctrl Pts',(-4.50176615109278,37.3262816596819,-16.2439666982713));
#52416=CARTESIAN_POINT('Ctrl Pts',(-4.85133542686646,37.0528279294366,-15.7706862599499));
#52417=CARTESIAN_POINT('Ctrl Pts',(-4.49167305004904,37.059789020437,-15.8813246755956));
#52418=CARTESIAN_POINT('Ctrl Pts',(-4.49849599207902,37.0618545761177,-16.2576124902641));
#52419=CARTESIAN_POINT('Ctrl Pts',(-4.85023355700303,36.9973424024009,-15.7710252327459));
#52420=CARTESIAN_POINT('Ctrl Pts',(-4.4886839703737,37.0062991010676,-15.8822165992224));
#52421=CARTESIAN_POINT('Ctrl Pts',(-4.49746393778067,37.0088752437307,-16.2604679296177));
#52422=CARTESIAN_POINT('Ctrl Pts',(-4.84724165567112,36.8866091092228,-15.7719450538262));
#52423=CARTESIAN_POINT('Ctrl Pts',(-4.48191083668474,36.8995910435531,-15.884223449632));
#52424=CARTESIAN_POINT('Ctrl Pts',(-4.49466160577087,36.9031322050459,-16.2664058785488));
#52425=CARTESIAN_POINT('Ctrl Pts',(-4.84535166014932,36.8313248270939,-15.7725258903161));
#52426=CARTESIAN_POINT('Ctrl Pts',(-4.47812221634299,36.846334338376,-15.8853396943));
#52427=CARTESIAN_POINT('Ctrl Pts',(-4.49289136220764,36.8503336431165,-16.2694900363544));
#52428=CARTESIAN_POINT('Ctrl Pts',(-4.83852205833163,36.6657142912634,-15.7746228790373));
#52429=CARTESIAN_POINT('Ctrl Pts',(-4.46555605276301,36.6865436945369,-15.8890228148251));
#52430=CARTESIAN_POINT('Ctrl Pts',(-4.48649448972876,36.6921526528426,-16.2790801157266));
#52431=CARTESIAN_POINT('Ctrl Pts',(-4.83242355820479,36.5556302061425,-15.7764934506682));
#52432=CARTESIAN_POINT('Ctrl Pts',(-4.45560823761615,36.5806099310771,-15.8919151266673));
#52433=CARTESIAN_POINT('Ctrl Pts',(-4.48078239625453,36.5869847872263,-16.2859235908837));
#52434=CARTESIAN_POINT('Ctrl Pts',(-4.80964445731595,36.2263139098162,-15.7834588216173));
#52435=CARTESIAN_POINT('Ctrl Pts',(-4.42108305755237,36.2626839420804,-15.9018687747033));
#52436=CARTESIAN_POINT('Ctrl Pts',(-4.45944659885922,36.2723112115469,-16.3077427542653));
#52437=CARTESIAN_POINT('Ctrl Pts',(-4.78849025521988,36.0080156926272,-15.7899064986773));
#52438=CARTESIAN_POINT('Ctrl Pts',(-4.39194405386607,36.0530811161892,-15.9101712621084));
#52439=CARTESIAN_POINT('Ctrl Pts',(-4.43963274611102,36.0636336832212,-16.3240065044515));
#52440=CARTESIAN_POINT('Ctrl Pts',(-4.73479895287024,35.5737873220669,-15.806089492256));
#52441=CARTESIAN_POINT('Ctrl Pts',(-4.32221309888832,35.6372576288513,-15.9296899223679));
#52442=CARTESIAN_POINT('Ctrl Pts',(-4.38934337165934,35.6483850846731,-16.3596596636497));
#52443=CARTESIAN_POINT('Ctrl Pts',(-4.70226083470289,35.3578573765994,-15.8158250321208));
#52444=CARTESIAN_POINT('Ctrl Pts',(-4.28136065754713,35.4308416469974,-15.9409730418437));
#52445=CARTESIAN_POINT('Ctrl Pts',(-4.35886689759704,35.4418142023149,-16.3790492831481));
#52446=CARTESIAN_POINT('Ctrl Pts',(-4.62604323000226,34.9283028530584,-15.838285969081));
#52447=CARTESIAN_POINT('Ctrl Pts',(-4.18843254356921,35.0215742894843,-15.9661140402609));
#52448=CARTESIAN_POINT('Ctrl Pts',(-4.28747850736095,35.030732994809,-16.4206641704048));
#52449=CARTESIAN_POINT('Ctrl Pts',(-4.58236381820235,34.7146782724582,-15.851011583154));
#52450=CARTESIAN_POINT('Ctrl Pts',(-4.13606020425487,34.8185183918786,-15.9800423530578));
#52451=CARTESIAN_POINT('Ctrl Pts',(-4.24656666166447,34.8262226570115,-16.4428896521688));
#52452=CARTESIAN_POINT('Ctrl Pts',(-4.48381152977406,34.2897290978801,-15.8791706501668));
#52453=CARTESIAN_POINT('Ctrl Pts',(-4.02005922178393,34.4162818436401,-16.0101335970749));
#52454=CARTESIAN_POINT('Ctrl Pts',(-4.15425873313437,34.4192706098088,-16.489899151371));
#52455=CARTESIAN_POINT('Ctrl Pts',(-4.42893989399129,34.0784042783794,-15.8946043422336));
#52456=CARTESIAN_POINT('Ctrl Pts',(-3.95608545255841,34.2168878693719,-16.0263702668423));
#52457=CARTESIAN_POINT('Ctrl Pts',(-4.10286381244933,34.2168286739799,-16.5146834150258));
#52458=CARTESIAN_POINT('Ctrl Pts',(-4.30763827259879,33.6581098781651,-15.9279065885377));
#52459=CARTESIAN_POINT('Ctrl Pts',(-3.81658438476888,33.822448010845,-16.0607242667002));
#52460=CARTESIAN_POINT('Ctrl Pts',(-3.9892479689298,33.814078955275,-16.5665395015097));
#52461=CARTESIAN_POINT('Ctrl Pts',(-4.24121110891681,33.4491397713452,-15.9457754442683));
#52462=CARTESIAN_POINT('Ctrl Pts',(-3.7406469800499,33.6271818424222,-16.0789181512321));
#52463=CARTESIAN_POINT('Ctrl Pts',(-3.92702968859027,33.6137706563386,-16.593611645947));
#52464=CARTESIAN_POINT('Ctrl Pts',(-4.15956467569048,33.2154445308089,-15.9670945891216));
#52465=CARTESIAN_POINT('Ctrl Pts',(-3.64949552390511,33.4129433397945,-16.0999721147917));
#52466=CARTESIAN_POINT('Ctrl Pts',(-3.8505564455756,33.3896995093833,-16.6252009188576));
#52467=CARTESIAN_POINT('Ctrl Pts',(-4.15039805956273,33.189502508749,-15.9694798681321));
#52468=CARTESIAN_POINT('Ctrl Pts',(-3.63914933651993,33.3888967259962,-16.102351301209));
#52469=CARTESIAN_POINT('Ctrl Pts',(-3.84197063429969,33.3648249628758,-16.6287259546484));
#52470=CARTESIAN_POINT('Ctrl Pts',(-4.13189835567043,33.1377349934672,-15.9742764246118));
#52471=CARTESIAN_POINT('Ctrl Pts',(-3.61829077577786,33.3409526006064,-16.1071260478771));
#52472=CARTESIAN_POINT('Ctrl Pts',(-3.82464308795729,33.3151858843453,-16.635796298032));
#52473=CARTESIAN_POINT('Ctrl Pts',(-4.12256202229053,33.111900164225,-15.9766885508706));
#52474=CARTESIAN_POINT('Ctrl Pts',(-3.60777388976757,33.3170463264599,-16.1095225753306));
#52475=CARTESIAN_POINT('Ctrl Pts',(-3.81589831288601,33.2904124009369,-16.6393428649039));
#52476=CARTESIAN_POINT('Ctrl Pts',(-4.09429258351795,33.0345428662843,-15.9839653076811));
#52477=CARTESIAN_POINT('Ctrl Pts',(-3.57590653652943,33.2454014404084,-16.1167504752498));
#52478=CARTESIAN_POINT('Ctrl Pts',(-3.78942005068434,33.2162305590499,-16.6500155854832));
#52479=CARTESIAN_POINT('Ctrl Pts',(-4.07509908358835,32.9831675632239,-15.9888703159868));
#52480=CARTESIAN_POINT('Ctrl Pts',(-3.55434588845088,33.1979873053765,-16.1215955300393));
#52481=CARTESIAN_POINT('Ctrl Pts',(-3.77144266781143,33.1669607859179,-16.6571747604242));
#52482=CARTESIAN_POINT('Ctrl Pts',(-4.01646745258513,32.829634429189,-16.0037375413478));
#52483=CARTESIAN_POINT('Ctrl Pts',(-3.48838399516754,33.0560510137945,-16.1362734133368));
#52484=CARTESIAN_POINT('Ctrl Pts',(-3.71652598867197,33.0197101694359,-16.6787750251782));
#52485=CARTESIAN_POINT('Ctrl Pts',(-3.9759789438393,32.728068962807,-16.0138519706474));
#52486=CARTESIAN_POINT('Ctrl Pts',(-3.44313323859855,32.9628501297851,-16.1461489724732));
#52487=CARTESIAN_POINT('Ctrl Pts',(-3.67860286745824,32.9222876367011,-16.6933388861798));
#52488=CARTESIAN_POINT('Ctrl Pts',(-3.85020901317665,32.4257893774983,-16.0447294945566));
#52489=CARTESIAN_POINT('Ctrl Pts',(-3.30213588601185,32.6845768004043,-16.1762600178974));
#52490=CARTESIAN_POINT('Ctrl Pts',(-3.56080183062287,32.6323019776143,-16.7374460185429));
#52491=CARTESIAN_POINT('Ctrl Pts',(-3.76063777621999,32.2274841877532,-16.0660275892435));
#52492=CARTESIAN_POINT('Ctrl Pts',(-3.20289234856102,32.5050107524786,-16.1965656821621));
#52493=CARTESIAN_POINT('Ctrl Pts',(-3.47690590589959,32.4420132288924,-16.767405951522));
#52494=CARTESIAN_POINT('Ctrl Pts',(-3.56918607340305,31.8377243308601,-16.1096415154308));
#52495=CARTESIAN_POINT('Ctrl Pts',(-2.99311023840048,32.1562009537945,-16.2372785343144));
#52496=CARTESIAN_POINT('Ctrl Pts',(-3.29758475214954,32.0679272033942,-16.8280153427249));
#52497=CARTESIAN_POINT('Ctrl Pts',(-3.46731167512559,31.6462664711462,-16.1319583909726));
#52498=CARTESIAN_POINT('Ctrl Pts',(-2.88201843494523,31.9870356344035,-16.2577213825395));
#52499=CARTESIAN_POINT('Ctrl Pts',(-3.20216520503585,31.8841268311116,-16.8586659752245));
#52500=CARTESIAN_POINT('Ctrl Pts',(-3.24986431304015,31.2709079333655,-16.1771664307246));
#52501=CARTESIAN_POINT('Ctrl Pts',(-2.6480156494036,31.6607525771679,-16.2980633785119));
#52502=CARTESIAN_POINT('Ctrl Pts',(-2.99849550013316,31.5237128636391,-16.9201885252478));
#52503=CARTESIAN_POINT('Ctrl Pts',(-3.13430309790084,31.087001037092,-16.2000593106867));
#52504=CARTESIAN_POINT('Ctrl Pts',(-2.52446501017816,31.5038249498316,-16.3179747703128));
#52505=CARTESIAN_POINT('Ctrl Pts',(-2.89025634469189,31.3470932540427,-16.9510624162517));
#52506=CARTESIAN_POINT('Ctrl Pts',(-2.97992813214864,30.8625464320075,-16.2287095736517));
#52507=CARTESIAN_POINT('Ctrl Pts',(-2.36471133653988,31.3195585189969,-16.3416730253026));
#52508=CARTESIAN_POINT('Ctrl Pts',(-2.74566271341961,31.1314993826496,-16.9894416021804));
#52509=CARTESIAN_POINT('Ctrl Pts',(-2.94855445916935,30.817928300523,-16.2344410657162));
#52510=CARTESIAN_POINT('Ctrl Pts',(-2.33186814409271,31.2826216760433,-16.3464413005094));
#52511=CARTESIAN_POINT('Ctrl Pts',(-2.71627690378355,31.0886409312827,-16.9971064561535));
#52512=CARTESIAN_POINT('Ctrl Pts',(-2.88476410492296,30.7292614499473,-16.2458975182613));
#52513=CARTESIAN_POINT('Ctrl Pts',(-2.26536475661494,31.2097212908695,-16.3558796919869));
#52514=CARTESIAN_POINT('Ctrl Pts',(-2.65652836285939,31.0034678637871,-17.0124038567864));
#52515=CARTESIAN_POINT('Ctrl Pts',(-2.85231509096079,30.6851711096193,-16.2516279588096));
#52516=CARTESIAN_POINT('Ctrl Pts',(-2.23166075706606,31.1737321819387,-16.3605534424715));
#52517=CARTESIAN_POINT('Ctrl Pts',(-2.62613534683824,30.9611132622823,-17.0200436860762));
#52518=CARTESIAN_POINT('Ctrl Pts',(-2.75371586507387,30.5543032513299,-16.2687276605509));
#52519=CARTESIAN_POINT('Ctrl Pts',(-2.12916708502008,31.0671513308951,-16.3744245592637));
#52520=CARTESIAN_POINT('Ctrl Pts',(-2.53378345502449,30.8353931303199,-17.0428092866419));
#52521=CARTESIAN_POINT('Ctrl Pts',(-2.68624145339725,30.4688168020419,-16.280019596665));
#52522=CARTESIAN_POINT('Ctrl Pts',(-2.05994523352376,30.9990432166992,-16.3833298319653));
#52523=CARTESIAN_POINT('Ctrl Pts',(-2.47058428125334,30.7532636055963,-17.057800327605));
#52524=CARTESIAN_POINT('Ctrl Pts',(-2.54757388740944,30.3015880840125,-16.3022942711121));
#52525=CARTESIAN_POINT('Ctrl Pts',(-1.9192454319902,30.8681341748231,-16.4004596153518));
#52526=CARTESIAN_POINT('Ctrl Pts',(-2.34070281481905,30.5925930259895,-17.0873081301815));
#52527=CARTESIAN_POINT('Ctrl Pts',(-2.476381206771,30.2198453486412,-16.3132771209141));
#52528=CARTESIAN_POINT('Ctrl Pts',(-1.84771884517628,30.8054525230851,-16.4086687974615));
#52529=CARTESIAN_POINT('Ctrl Pts',(-2.27402096482143,30.5140515215888,-17.1018250250437));
#52530=CARTESIAN_POINT('Ctrl Pts',(-2.32998205788182,30.0603897553416,-16.334829595528));
#52531=CARTESIAN_POINT('Ctrl Pts',(-1.70258673578777,30.6857855527938,-16.4242870257666));
#52532=CARTESIAN_POINT('Ctrl Pts',(-2.13689779545945,30.3608345647763,-17.1302692409457));
#52533=CARTESIAN_POINT('Ctrl Pts',(-2.25477627281575,29.982676223402,-16.345399374049));
#52534=CARTESIAN_POINT('Ctrl Pts',(-1.62894510471729,30.6289401059803,-16.4316764817347));
#52535=CARTESIAN_POINT('Ctrl Pts',(-2.06645711480206,30.2861584632619,-17.1441967467396));
#52536=CARTESIAN_POINT('Ctrl Pts',(-2.09997874346892,29.831641210054,-16.3660070272072));
#52537=CARTESIAN_POINT('Ctrl Pts',(-1.47982485477628,30.5213540438189,-16.4455349971866));
#52538=CARTESIAN_POINT('Ctrl Pts',(-1.92146769383922,30.1410235804603,-17.1713290042148));
#52539=CARTESIAN_POINT('Ctrl Pts',(-2.02038800914664,29.7583187312675,-16.3760451220302));
#52540=CARTESIAN_POINT('Ctrl Pts',(-1.40432964804446,30.4707756283822,-16.4519799689631));
#52541=CARTESIAN_POINT('Ctrl Pts',(-1.84691989810708,30.0705638387238,-17.1845340213945));
#52542=CARTESIAN_POINT('Ctrl Pts',(-1.89735688368434,29.6519763755937,-16.3905992032782));
#52543=CARTESIAN_POINT('Ctrl Pts',(-1.29061421420031,30.4002010119293,-16.4608187862555));
#52544=CARTESIAN_POINT('Ctrl Pts',(-1.73168413361204,29.9683736297906,-17.2036812816511));
#52545=CARTESIAN_POINT('Ctrl Pts',(-1.855738117802,29.6171366953533,-16.3953665421613));
#52546=CARTESIAN_POINT('Ctrl Pts',(-1.25230151783671,30.3773864795662,-16.4636476099762));
#52547=CARTESIAN_POINT('Ctrl Pts',(-1.69270236914862,29.9348943080071,-17.2099534441512));
#52548=CARTESIAN_POINT('Ctrl Pts',(-1.79234339952953,29.5658416895116,-16.4023765699238));
#52549=CARTESIAN_POINT('Ctrl Pts',(-1.19475183342288,30.3445305772294,-16.4676726412067));
#52550=CARTESIAN_POINT('Ctrl Pts',(-1.63332439632481,29.8856025996842,-17.2191791942467));
#52551=CARTESIAN_POINT('Ctrl Pts',(-1.77105066057652,29.5489041771658,-16.4046897342604));
#52552=CARTESIAN_POINT('Ctrl Pts',(-1.17547199819176,30.333762872091,-16.4689831252204));
#52553=CARTESIAN_POINT('Ctrl Pts',(-1.6133807839376,29.8693266444902,-17.2222240118077));
#52554=CARTESIAN_POINT('Ctrl Pts',(-1.72813291087157,29.5153605402291,-16.409266356606));
#52555=CARTESIAN_POINT('Ctrl Pts',(-1.13683610528857,30.3126589001511,-16.4715332981359));
#52556=CARTESIAN_POINT('Ctrl Pts',(-1.57318234083472,29.8370933859026,-17.2282496978405));
#52557=CARTESIAN_POINT('Ctrl Pts',(-1.70649633572161,29.4987461608599,-16.4115309334004));
#52558=CARTESIAN_POINT('Ctrl Pts',(-1.11747086839056,30.3023210014394,-16.4727730500227));
#52559=CARTESIAN_POINT('Ctrl Pts',(-1.5529166780537,29.8211281512158,-17.231232043014));
#52560=CARTESIAN_POINT('Ctrl Pts',(-1.59782880094616,29.416805054283,-16.4226849288261));
#52561=CARTESIAN_POINT('Ctrl Pts',(-1.01994827144306,30.2514460679374,-16.4788242146341));
#52562=CARTESIAN_POINT('Ctrl Pts',(-1.45113441423997,29.7423892766781,-17.2459262700218));
#52563=CARTESIAN_POINT('Ctrl Pts',(-1.50908967345445,29.3546606084382,-16.4310964828382));
#52564=CARTESIAN_POINT('Ctrl Pts',(-0.94294827805055,30.2151476418465,-16.4829741135679));
#52565=CARTESIAN_POINT('Ctrl Pts',(-1.36801787580905,29.6826756493925,-17.2570235387147));
#52566=CARTESIAN_POINT('Ctrl Pts',(-1.32773854032885,29.2376739642212,-16.446744165317));
#52567=CARTESIAN_POINT('Ctrl Pts',(-0.789958819385205,30.1499851126795,
-16.4900488930594));
#52568=CARTESIAN_POINT('Ctrl Pts',(-1.19815731065464,29.570273767709,-17.2777301553418));
#52569=CARTESIAN_POINT('Ctrl Pts',(-1.23512712642901,29.1828306555037,-16.4539805128856));
#52570=CARTESIAN_POINT('Ctrl Pts',(-0.714148771847181,30.1213547087018,
-16.4929390217047));
#52571=CARTESIAN_POINT('Ctrl Pts',(-1.11141383725493,29.5175844450748,-17.2873397728772));
#52572=CARTESIAN_POINT('Ctrl Pts',(-1.04569979909049,29.0810615938186,-16.4671043497951));
#52573=CARTESIAN_POINT('Ctrl Pts',(-0.564018986317464,30.0710934810012,
-16.4975516672181));
#52574=CARTESIAN_POINT('Ctrl Pts',(-0.933988792708237,29.4198266340564,
-17.3048725518148));
#52575=CARTESIAN_POINT('Ctrl Pts',(-0.948884762668731,29.0341341932451,
-16.4729921490482));
#52576=CARTESIAN_POINT('Ctrl Pts',(-0.489933276919771,30.0496744036365,
-16.4992439979384));
#52577=CARTESIAN_POINT('Ctrl Pts',(-0.843308041987629,29.3747565609294,
-17.3127960973893));
#52578=CARTESIAN_POINT('Ctrl Pts',(-0.800191680576077,28.9702716007703,
-16.4806600727396));
#52579=CARTESIAN_POINT('Ctrl Pts',(-0.380586307990408,30.0223765474346,
-16.5009885630312));
#52580=CARTESIAN_POINT('Ctrl Pts',(-0.704036284927813,29.3134377089103,
-17.3232401222866));
#52581=CARTESIAN_POINT('Ctrl Pts',(-0.750048107089607,28.9500736446709,
-16.483021826383));
#52582=CARTESIAN_POINT('Ctrl Pts',(-0.344229360090164,30.014052241189,-16.5014375482369));
#52583=CARTESIAN_POINT('Ctrl Pts',(-0.657069852279363,29.2940472367443,
-17.3264809285521));
#52584=CARTESIAN_POINT('Ctrl Pts',(-0.673915805988587,28.9215008203245,
-16.486251322221));
#52585=CARTESIAN_POINT('Ctrl Pts',(-0.290130099099646,30.0026923249378,
-16.501926978582));
#52586=CARTESIAN_POINT('Ctrl Pts',(-0.585761361026588,29.2666219330869,
-17.3309558082814));
#52587=CARTESIAN_POINT('Ctrl Pts',(-0.648385485598382,28.91226401611,-16.4872756105357));
#52588=CARTESIAN_POINT('Ctrl Pts',(-0.272119298069543,29.9990851554066,
-16.5020595144662));
#52589=CARTESIAN_POINT('Ctrl Pts',(-0.561848664151634,29.2577570144913,
-17.3323830214636));
#52590=CARTESIAN_POINT('Ctrl Pts',(-0.597010216853532,28.8943818767733,
-16.4892158575437));
#52591=CARTESIAN_POINT('Ctrl Pts',(-0.2362023844278,29.9922245088925,-16.5022661141874));
#52592=CARTESIAN_POINT('Ctrl Pts',(-0.513728577814346,29.2405968337917,
-17.3351040222603));
#52593=CARTESIAN_POINT('Ctrl Pts',(-0.571233147511417,28.8857606891544,
-16.4901291611817));
#52594=CARTESIAN_POINT('Ctrl Pts',(-0.218349366931985,29.9889826962993,
-16.5023396092702));
#52595=CARTESIAN_POINT('Ctrl Pts',(-0.4895847662591,29.2323247467198,-17.3363941024547));
#52596=CARTESIAN_POINT('Ctrl Pts',(-0.442166073327688,28.8443554178395,
-16.4943979018314));
#52597=CARTESIAN_POINT('Ctrl Pts',(-0.129239837306087,29.9735906916381,
-16.5025703106399));
#52598=CARTESIAN_POINT('Ctrl Pts',(-0.368695495698975,29.1926016196164,
-17.342474342916));
#52599=CARTESIAN_POINT('Ctrl Pts',(-0.338061778022354,28.8165747708187,
-16.4968705077674));
#52600=CARTESIAN_POINT('Ctrl Pts',(-0.0605317814243137,29.9642648979254,
-16.5023091130787));
#52601=CARTESIAN_POINT('Ctrl Pts',(-0.271187340267436,29.1659679325416,
-17.3461688365462));
#52602=CARTESIAN_POINT('Ctrl Pts',(-0.128108295013126,28.7719728676628,
-16.499836683451));
#52603=CARTESIAN_POINT('Ctrl Pts',(0.074456716006171,29.94974338385,-16.5011651314723));
#52604=CARTESIAN_POINT('Ctrl Pts',(-0.0745366950826016,29.1232544765027,
-17.3511133431508));
#52605=CARTESIAN_POINT('Ctrl Pts',(-0.0222591829595038,28.755151135902,
-16.5003303276454));
#52606=CARTESIAN_POINT('Ctrl Pts',(0.140356992327616,29.9446203245694,-16.5002807332538));
#52607=CARTESIAN_POINT('Ctrl Pts',(0.0246057239760995,29.1071742509764,
-17.3523634528138));
#52608=CARTESIAN_POINT('Ctrl Pts',(0.191245793985154,28.7328543901453,-16.499236995659));
#52609=CARTESIAN_POINT('Ctrl Pts',(0.27161304708856,29.937520037568,-16.4980385051));
#52610=CARTESIAN_POINT('Ctrl Pts',(0.224582837315142,29.0859421960738,-17.3523016800784));
#52611=CARTESIAN_POINT('Ctrl Pts',(0.298901540034271,28.7273786281084,-16.4976501104633));
#52612=CARTESIAN_POINT('Ctrl Pts',(0.336593949719366,29.9355704487499,-16.496686377349));
#52613=CARTESIAN_POINT('Ctrl Pts',(0.325417420428351,29.080789649795,-17.3509899235518));
#52614=CARTESIAN_POINT('Ctrl Pts',(0.434652344247154,28.7279511908531,-16.4942964360642));
#52615=CARTESIAN_POINT('Ctrl Pts',(0.41904432966663,29.9349828888683,-16.4946901599378));
#52616=CARTESIAN_POINT('Ctrl Pts',(0.452566934002955,29.0814932456998,-17.3476656555962));
#52617=CARTESIAN_POINT('Ctrl Pts',(0.461791435185215,28.7284371115372,-16.4935588164354));
#52618=CARTESIAN_POINT('Ctrl Pts',(0.435530517342106,29.9349612139799,-16.4942766579394));
#52619=CARTESIAN_POINT('Ctrl Pts',(0.477986468216754,29.0819916232635,-17.3469181407489));
#52620=CARTESIAN_POINT('Ctrl Pts',(0.515943690984539,28.7301437164452,-16.4919536704588));
#52621=CARTESIAN_POINT('Ctrl Pts',(0.468495969700064,29.9351121018813,-16.4934206136822));
#52622=CARTESIAN_POINT('Ctrl Pts',(0.528707589352712,29.0836958274767,-17.3452619533545));
#52623=CARTESIAN_POINT('Ctrl Pts',(0.542973446398712,28.7313644483332,-16.4910857384778));
#52624=CARTESIAN_POINT('Ctrl Pts',(0.484979151558676,29.9352844403668,-16.4929780058774));
#52625=CARTESIAN_POINT('Ctrl Pts',(0.554024715635541,29.084901718379,-17.344352879355));
#52626=CARTESIAN_POINT('Ctrl Pts',(0.623924958202809,28.7361181266015,-16.4882877715005));
#52627=CARTESIAN_POINT('Ctrl Pts',(0.534479466208411,29.9361010848821,-16.4916034160629));
#52628=CARTESIAN_POINT('Ctrl Pts',(0.629847068288364,29.0895703548083,-17.3413850837553));
#52629=CARTESIAN_POINT('Ctrl Pts',(0.677708990090665,28.7407423067484,-16.4861635783227));
#52630=CARTESIAN_POINT('Ctrl Pts',(0.567561890649228,29.9370419497641,-16.490624834322));
#52631=CARTESIAN_POINT('Ctrl Pts',(0.680223296507896,29.0940838248501,-17.339085810858));
#52632=CARTESIAN_POINT('Ctrl Pts',(0.838519927256103,28.7589030127749,-16.4790291084593));
#52633=CARTESIAN_POINT('Ctrl Pts',(0.667392543733618,29.9411882626693,-16.4874678461666));
#52634=CARTESIAN_POINT('Ctrl Pts',(0.830845110920096,29.1117531657169,-17.3312437799614));
#52635=CARTESIAN_POINT('Ctrl Pts',(0.945006106505387,28.7767241011346,-16.4732571040723));
#52636=CARTESIAN_POINT('Ctrl Pts',(0.734797573094118,29.9456748746285,-16.4850736283494));
#52637=CARTESIAN_POINT('Ctrl Pts',(0.930584232001352,29.1290345185376,-17.3247571305769));
#52638=CARTESIAN_POINT('Ctrl Pts',(1.07723807457993,28.8059438373021,-16.4648188690481));
#52639=CARTESIAN_POINT('Ctrl Pts',(0.821934628374837,29.9543140629695,-16.481507158621));
#52640=CARTESIAN_POINT('Ctrl Pts',(1.05443786599453,29.1573212640841,-17.315130200981));
#52641=CARTESIAN_POINT('Ctrl Pts',(1.10366391397319,28.8121410610613,-16.4630684410996));
#52642=CARTESIAN_POINT('Ctrl Pts',(0.839404777360703,29.9561838764168,-16.4807692180936));
#52643=CARTESIAN_POINT('Ctrl Pts',(1.07918934093606,29.1633187716124,-17.3131270133982));
#52644=CARTESIAN_POINT('Ctrl Pts',(1.15632374754114,28.8252003709767,-16.4594535730141));
#52645=CARTESIAN_POINT('Ctrl Pts',(0.874521011859752,29.9602382847319,-16.4792360955938));
#52646=CARTESIAN_POINT('Ctrl Pts',(1.12851260097818,29.1759537682257,-17.3089782907615));
#52647=CARTESIAN_POINT('Ctrl Pts',(1.18250126727682,28.8320477321608,-16.4575931395356));
#52648=CARTESIAN_POINT('Ctrl Pts',(0.892123466946685,29.9624166282505,-16.4784430213444));
#52649=CARTESIAN_POINT('Ctrl Pts',(1.15303149003764,29.1825770131165,-17.3068373640129));
#52650=CARTESIAN_POINT('Ctrl Pts',(1.26059001577615,28.8535152040682,-16.4518581803553));
#52651=CARTESIAN_POINT('Ctrl Pts',(0.945006269189896,29.9694228223987,-16.4759818429639));
#52652=CARTESIAN_POINT('Ctrl Pts',(1.22617246651459,29.2033372707004,-17.3002214041692));
#52653=CARTESIAN_POINT('Ctrl Pts',(1.31205768956044,28.8690601669617,-16.4478300726312));
#52654=CARTESIAN_POINT('Ctrl Pts',(0.980523921137524,29.974736003371,-16.4742254675058));
#52655=CARTESIAN_POINT('Ctrl Pts',(1.27437910322739,29.2183642879055,-17.2955532864967));
#52656=CARTESIAN_POINT('Ctrl Pts',(1.4647831287284,28.9191944472757,-16.43517107612));
#52657=CARTESIAN_POINT('Ctrl Pts',(1.08747216242771,29.9927517710206,-16.4685881506749));
#52658=CARTESIAN_POINT('Ctrl Pts',(1.41742772376219,29.2668125837537,-17.2808247001297));
#52659=CARTESIAN_POINT('Ctrl Pts',(1.56436648530266,28.957276499474,-16.4259664459877));
#52660=CARTESIAN_POINT('Ctrl Pts',(1.15996351383399,30.0075731994565,-16.4643154615969));
#52661=CARTESIAN_POINT('Ctrl Pts',(1.51070139131698,29.3035947033487,-17.2700412085024));
#52662=CARTESIAN_POINT('Ctrl Pts',(1.75949339397493,29.0418768304825,-16.4062122131103));
#52663=CARTESIAN_POINT('Ctrl Pts',(1.30740732628336,30.0440019520787,-16.4545229469892));
#52664=CARTESIAN_POINT('Ctrl Pts',(1.69346488679426,29.385274695068,-17.246768023877));
#52665=CARTESIAN_POINT('Ctrl Pts',(1.85503603822308,29.0883970101933,-16.3956623294501));
#52666=CARTESIAN_POINT('Ctrl Pts',(1.38208746912005,30.0654311191767,-16.449040555324));
#52667=CARTESIAN_POINT('Ctrl Pts',(1.78295386512358,29.4301743920079,-17.2342779633839));
#52668=CARTESIAN_POINT('Ctrl Pts',(2.04241537792939,29.1891877116256,-16.3733759911771));
#52669=CARTESIAN_POINT('Ctrl Pts',(1.53349668675425,30.1157894070632,-16.4367176133733));
#52670=CARTESIAN_POINT('Ctrl Pts',(1.95846068444071,29.5274274114621,-17.2077786001255));
#52671=CARTESIAN_POINT('Ctrl Pts',(2.13425146341608,29.2434595083696,-16.3616393385331));
#52672=CARTESIAN_POINT('Ctrl Pts',(1.61000429268926,30.1445060379138,-16.4299192937042));
#52673=CARTESIAN_POINT('Ctrl Pts',(2.04447795482465,29.5797819581103,-17.1937690407036));
#52674=CARTESIAN_POINT('Ctrl Pts',(2.3144828178405,29.3592119103105,-16.3371184864176));
#52675=CARTESIAN_POINT('Ctrl Pts',(1.76445361782877,30.2098541291851,-16.4149279831066));
#52676=CARTESIAN_POINT('Ctrl Pts',(2.21328969153138,29.6914212472574,-17.1643920201756));
#52677=CARTESIAN_POINT('Ctrl Pts',(2.40287766710257,29.4206933906018,-16.3243341414413));
#52678=CARTESIAN_POINT('Ctrl Pts',(1.84222493333582,30.2462536617642,-16.4067789597616));
#52679=CARTESIAN_POINT('Ctrl Pts',(2.29608376542315,29.7507068302044,-17.1490243729861));
#52680=CARTESIAN_POINT('Ctrl Pts',(2.51135285252538,29.5017829309144,-16.3077769328132));
#52681=CARTESIAN_POINT('Ctrl Pts',(1.94077379223057,30.2972459914495,-16.3956391132683));
#52682=CARTESIAN_POINT('Ctrl Pts',(2.39768586735591,29.8288858890433,-17.1290549495678));
#52683=CARTESIAN_POINT('Ctrl Pts',(2.53290170127805,29.5181794566019,-16.3044434790811));
#52684=CARTESIAN_POINT('Ctrl Pts',(1.96028897303141,30.3075771594425,-16.3933941774779));
#52685=CARTESIAN_POINT('Ctrl Pts',(2.41786936214229,29.8446932300906,-17.1250312972996));
#52686=CARTESIAN_POINT('Ctrl Pts',(2.57565545767622,29.5512731693992,-16.2977442351459));
#52687=CARTESIAN_POINT('Ctrl Pts',(1.99921568638862,30.3286552806381,-16.3888383057235));
#52688=CARTESIAN_POINT('Ctrl Pts',(2.45791420271846,29.8765964221614,-17.1169385254278));
#52689=CARTESIAN_POINT('Ctrl Pts',(2.59687024481893,29.5679777347785,-16.2943769383145));
#52690=CARTESIAN_POINT('Ctrl Pts',(2.01863572271277,30.3394038774272,-16.3865268648834));
#52691=CARTESIAN_POINT('Ctrl Pts',(2.47778480237176,29.8926993859692,-17.1128675875488));
#52692=CARTESIAN_POINT('Ctrl Pts',(2.66004324798223,29.6185503436459,-16.2842251711301));
#52693=CARTESIAN_POINT('Ctrl Pts',(2.07658934638655,30.3721820016165,-16.3795138210175));
#52694=CARTESIAN_POINT('Ctrl Pts',(2.53695510817887,29.9414486673533,-17.100584863834));
#52695=CARTESIAN_POINT('Ctrl Pts',(2.70153038913429,29.6528770266069,-16.2773908679428));
#52696=CARTESIAN_POINT('Ctrl Pts',(2.11515348080612,30.3949183678539,-16.3746953336256));
#52697=CARTESIAN_POINT('Ctrl Pts',(2.57581358773611,29.9745351098867,-17.0923032197876));
#52698=CARTESIAN_POINT('Ctrl Pts',(2.82421530443451,29.7575890425693,-16.2567120771395));
#52699=CARTESIAN_POINT('Ctrl Pts',(2.22956819594977,30.4651684504852,-16.3599495397914));
#52700=CARTESIAN_POINT('Ctrl Pts',(2.69072507829928,30.0754559176024,-17.0672065911949));
#52701=CARTESIAN_POINT('Ctrl Pts',(2.90364008546083,29.8297029496513,-16.2426922301433));
#52702=CARTESIAN_POINT('Ctrl Pts',(2.30547175408465,30.5154143020214,-16.3495803497904));
#52703=CARTESIAN_POINT('Ctrl Pts',(2.7651174356246,30.1449484959329,-17.0501405710026));
#52704=CARTESIAN_POINT('Ctrl Pts',(3.05823671500216,29.9780894969754,-16.2142950763844));
#52705=CARTESIAN_POINT('Ctrl Pts',(2.45531918886263,30.6220505261989,-16.3279618812435));
#52706=CARTESIAN_POINT('Ctrl Pts',(2.90991868602117,30.2879200951006,-17.0154679498268));
#52707=CARTESIAN_POINT('Ctrl Pts',(3.13340755103014,30.0543631118974,-16.1999176059517));
#52708=CARTESIAN_POINT('Ctrl Pts',(2.52928950864992,30.6782919897607,-16.316734700869));
#52709=CARTESIAN_POINT('Ctrl Pts',(2.98032663199793,30.3614000520084,-16.9978611399441));
#52710=CARTESIAN_POINT('Ctrl Pts',(3.27987015132021,30.210715992756,-16.1709005658607));
#52711=CARTESIAN_POINT('Ctrl Pts',(2.67504196758113,30.7964541736505,-16.2935360824409));
#52712=CARTESIAN_POINT('Ctrl Pts',(3.11750923246245,30.5120049089877,-16.9622167722053));
#52713=CARTESIAN_POINT('Ctrl Pts',(3.35116123035258,30.2907959175364,-16.156260881267));
#52714=CARTESIAN_POINT('Ctrl Pts',(2.74686657696321,30.8582478680463,-16.2815815826731));
#52715=CARTESIAN_POINT('Ctrl Pts',(3.18428324621236,30.5891304417996,-16.9441790683909));
#52716=CARTESIAN_POINT('Ctrl Pts',(3.55966298596679,30.5363244595009,-16.1120758578107));
#52717=CARTESIAN_POINT('Ctrl Pts',(2.95660210195659,31.049475646984,-16.2451814165979));
#52718=CARTESIAN_POINT('Ctrl Pts',(3.37957414633138,30.8255678671554,-16.8895639888451));
#52719=CARTESIAN_POINT('Ctrl Pts',(3.69152422416695,30.7070404100115,-16.0822670185369));
#52720=CARTESIAN_POINT('Ctrl Pts',(3.0935680110286,31.188233012752,-16.2194870411642));
#52721=CARTESIAN_POINT('Ctrl Pts',(3.50308054074258,30.9899200073615,-16.8524880403649));
#52722=CARTESIAN_POINT('Ctrl Pts',(3.84850625888578,30.9282217390845,-16.0449381752436));
#52723=CARTESIAN_POINT('Ctrl Pts',(3.2607646882954,31.3759330382798,-16.1859089389379));
#52724=CARTESIAN_POINT('Ctrl Pts',(3.6501160551046,31.2027958226833,-16.8057225066586));
#52725=CARTESIAN_POINT('Ctrl Pts',(3.87953256866694,30.9728856431268,-16.0374628392411));
#52726=CARTESIAN_POINT('Ctrl Pts',(3.29342662187892,31.4134934654484,-16.1792418772485));
#52727=CARTESIAN_POINT('Ctrl Pts',(3.67917651069663,31.2457796337213,-16.7963405521398));
#52728=CARTESIAN_POINT('Ctrl Pts',(3.94058434545197,31.0626285007038,-16.022571026142));
#52729=CARTESIAN_POINT('Ctrl Pts',(3.35787539127852,31.4893981914476,-16.1658790869078));
#52730=CARTESIAN_POINT('Ctrl Pts',(3.73635999288582,31.3321406834297,-16.7776156643026));
#52731=CARTESIAN_POINT('Ctrl Pts',(3.97063463723664,31.1077409109996,-16.0151487999533));
#52732=CARTESIAN_POINT('Ctrl Pts',(3.38969847622929,31.5277649299416,-16.1591781972395));
#52733=CARTESIAN_POINT('Ctrl Pts',(3.76450627188365,31.3755501268062,-16.7682655550614));
#52734=CARTESIAN_POINT('Ctrl Pts',(4.05941717087094,31.2437732562028,-15.9929626480247));
#52735=CARTESIAN_POINT('Ctrl Pts',(3.48351050644036,31.6435098716445,-16.1391308660064));
#52736=CARTESIAN_POINT('Ctrl Pts',(3.84766346564603,31.5064382047407,-16.7402628285028));
#52737=CARTESIAN_POINT('Ctrl Pts',(4.1167828254897,31.3353874419429,-15.978279338896));
#52738=CARTESIAN_POINT('Ctrl Pts',(3.54479499845881,31.7226089412723,-16.1256471238317));
#52739=CARTESIAN_POINT('Ctrl Pts',(3.90139438215665,31.5945757570875,-16.7216579368768));
#52740=CARTESIAN_POINT('Ctrl Pts',(4.28380788594745,31.6128203257638,-15.9346238064299));
#52741=CARTESIAN_POINT('Ctrl Pts',(3.72231473431664,31.9620905398297,-16.0855354656462));
#52742=CARTESIAN_POINT('Ctrl Pts',(4.05783658707824,31.8614425296594,-16.6661133987202));
#52743=CARTESIAN_POINT('Ctrl Pts',(4.3884148581878,31.8012197189447,-15.9060466319014));
#52744=CARTESIAN_POINT('Ctrl Pts',(3.83587999076983,32.1288604724229,-16.0584933410282));
#52745=CARTESIAN_POINT('Ctrl Pts',(4.15581556986088,32.0426166386068,-16.6294449643945));
#52746=CARTESIAN_POINT('Ctrl Pts',(4.58567200756637,32.1841943988468,-15.8503033618542));
#52747=CARTESIAN_POINT('Ctrl Pts',(4.05086579113235,32.4720636118671,-16.0050120263636));
#52748=CARTESIAN_POINT('Ctrl Pts',(4.34057433194744,32.4107939451974,-16.5572151315481));
#52749=CARTESIAN_POINT('Ctrl Pts',(4.67831544203237,32.3787729501169,-15.8231365471297));
#52750=CARTESIAN_POINT('Ctrl Pts',(4.152839616667,32.6484592325927,-15.9785118187779));
#52751=CARTESIAN_POINT('Ctrl Pts',(4.4273477970609,32.5978002916929,-16.5216528747722));
#52752=CARTESIAN_POINT('Ctrl Pts',(4.8526074647995,32.7736749069825,-15.7705575791359));
#52753=CARTESIAN_POINT('Ctrl Pts',(4.34531777018242,33.0096063680591,-15.9266467671527));
#52754=CARTESIAN_POINT('Ctrl Pts',(4.59059652338769,32.9772145356856,-16.4519928922655));
#52755=CARTESIAN_POINT('Ctrl Pts',(4.93425250225085,32.9740000075212,-15.7451448786754));
#52756=CARTESIAN_POINT('Ctrl Pts',(4.43629332140126,33.1943793675723,-15.9012113154715));
#52757=CARTESIAN_POINT('Ctrl Pts',(4.66706845943702,33.1696240761953,-16.4178945495574));
#52758=CARTESIAN_POINT('Ctrl Pts',(5.08711281849313,33.3801631316144,-15.6964237384943));
#52759=CARTESIAN_POINT('Ctrl Pts',(4.60722078767624,33.5714101157215,-15.8519572579756));
#52760=CARTESIAN_POINT('Ctrl Pts',(4.81024341123228,33.5596069464454,-16.3515167576984));
#52761=CARTESIAN_POINT('Ctrl Pts',(5.15832642133817,33.5860019204558,-15.6731147994769));
#52762=CARTESIAN_POINT('Ctrl Pts',(4.68757869339825,33.7637237962017,-15.8280627301349));
#52763=CARTESIAN_POINT('Ctrl Pts',(4.87694485739314,33.7571810298932,-16.3192367814774));
#52764=CARTESIAN_POINT('Ctrl Pts',(5.24097629968965,33.8467036990582,-15.6455255940079));
#52765=CARTESIAN_POINT('Ctrl Pts',(4.78213072770676,34.0107071083605,-15.7992314731343));
#52766=CARTESIAN_POINT('Ctrl Pts',(4.95435796666611,34.0073247840893,-16.2802535152582));
#52767=CARTESIAN_POINT('Ctrl Pts',(5.25719362818707,33.8990359684241,-15.6400829974654));
#52768=CARTESIAN_POINT('Ctrl Pts',(4.80054957120818,34.0598870173825,-15.793578275618));
#52769=CARTESIAN_POINT('Ctrl Pts',(4.96954775094229,34.0575332013725,-16.2725221393888));
#52770=CARTESIAN_POINT('Ctrl Pts',(5.28896226944923,34.0039467757404,-15.6293684812982));
#52771=CARTESIAN_POINT('Ctrl Pts',(4.83669604861666,34.1585897884646,-15.7824156043202));
#52772=CARTESIAN_POINT('Ctrl Pts',(4.99930350304212,34.1581771173989,-16.2572160497018));
#52773=CARTESIAN_POINT('Ctrl Pts',(5.30449626492683,34.0564670383293,-15.624102431784));
#52774=CARTESIAN_POINT('Ctrl Pts',(4.85440974566674,34.2080603224636,-15.7769108872987));
#52775=CARTESIAN_POINT('Ctrl Pts',(5.0138532509136,34.208556714705,-16.2496497575703));
#52776=CARTESIAN_POINT('Ctrl Pts',(5.3500593030389,34.2142207349753,-15.6085840212356));
#52777=CARTESIAN_POINT('Ctrl Pts',(4.90631386646526,34.3563731632076,-15.7606865923713));
#52778=CARTESIAN_POINT('Ctrl Pts',(5.05652937471128,34.3598665463188,-16.2272172272366));
#52779=CARTESIAN_POINT('Ctrl Pts',(5.37905002720047,34.3196469683343,-15.598611350614));
#52780=CARTESIAN_POINT('Ctrl Pts',(4.9396069834735,34.4560073796611,-15.7501529654412));
#52781=CARTESIAN_POINT('Ctrl Pts',(5.08368322108408,34.460967717809,-16.2126172924642));
#52782=CARTESIAN_POINT('Ctrl Pts',(5.46194078461707,34.6366877503115,-15.569862681342));
#52783=CARTESIAN_POINT('Ctrl Pts',(5.03466043352864,34.7544911380799,-15.7197631997284));
#52784=CARTESIAN_POINT('Ctrl Pts',(5.16132194699471,34.7649439115857,-16.1699328633975));
#52785=CARTESIAN_POINT('Ctrl Pts',(5.51176846617966,34.8490627904254,-15.5522551143952));
#52786=CARTESIAN_POINT('Ctrl Pts',(5.09291260313501,34.9564096240105,-15.7007118502892));
#52787=CARTESIAN_POINT('Ctrl Pts',(5.2079925027011,34.968490137579,-16.1429629194519));
#52788=CARTESIAN_POINT('Ctrl Pts',(5.60071361456991,35.275833071767,-15.5204457982229));
#52789=CARTESIAN_POINT('Ctrl Pts',(5.19800485837501,35.3631027727456,-15.6657772117967));
#52790=CARTESIAN_POINT('Ctrl Pts',(5.29130200819381,35.3773514622423,-16.0922807281473));
#52791=CARTESIAN_POINT('Ctrl Pts',(5.63983069135891,35.4902283652519,-15.5062438204224));
#52792=CARTESIAN_POINT('Ctrl Pts',(5.24514293116004,35.5680932299173,-15.649807466499));
#52793=CARTESIAN_POINT('Ctrl Pts',(5.32794059231136,35.5826666215459,-16.0685682530086));
#52794=CARTESIAN_POINT('Ctrl Pts',(5.70722219029865,35.9210809846202,-15.4815665394735));
#52795=CARTESIAN_POINT('Ctrl Pts',(5.32796042195972,35.9807456339375,-15.6213886714218));
#52796=CARTESIAN_POINT('Ctrl Pts',(5.39106210676183,35.9950907162295,-16.0247146511509));
#52797=CARTESIAN_POINT('Ctrl Pts',(5.73549725525296,36.1375381840345,-15.4710909455289));
#52798=CARTESIAN_POINT('Ctrl Pts',(5.36389926796403,36.1886130621991,-15.6088583771076));
#52799=CARTESIAN_POINT('Ctrl Pts',(5.41754563828522,36.2021995446388,-16.004573243818));
#52800=CARTESIAN_POINT('Ctrl Pts',(5.78078346060784,36.5726077638088,-15.4542268131215));
#52801=CARTESIAN_POINT('Ctrl Pts',(5.42398393004534,36.606935192749,-15.5876972584938));
#52802=CARTESIAN_POINT('Ctrl Pts',(5.45996247023453,36.6182830146743,-15.9682119674733));
#52803=CARTESIAN_POINT('Ctrl Pts',(5.7977963957715,36.7912198164816,-15.4478378834369));
#52804=CARTESIAN_POINT('Ctrl Pts',(5.44836047329696,36.8175859984048,-15.5789899469686));
#52805=CARTESIAN_POINT('Ctrl Pts',(5.47589745022953,36.8272573619824,-15.9519917284049));
#52806=CARTESIAN_POINT('Ctrl Pts',(5.81430843554853,37.1208676336436,-15.4416272457358));
#52807=CARTESIAN_POINT('Ctrl Pts',(5.47569053932407,37.1367087944884,-15.5691295274642));
#52808=CARTESIAN_POINT('Ctrl Pts',(5.49136327314324,37.1422120437367,-15.9308997542));
#52809=CARTESIAN_POINT('Ctrl Pts',(5.81830852011158,37.2310390122662,-15.4401195822918));
#52810=CARTESIAN_POINT('Ctrl Pts',(5.48324669152352,37.243039155561,-15.5663815273683));
#52811=CARTESIAN_POINT('Ctrl Pts',(5.49510990843326,37.2474462392647,-15.924409220868));
#52812=CARTESIAN_POINT('Ctrl Pts',(5.8219552680468,37.3967483415922,-15.4387447204924));
#52813=CARTESIAN_POINT('Ctrl Pts',(5.49218973652234,37.4033363287178,-15.5630995045285));
#52814=CARTESIAN_POINT('Ctrl Pts',(5.49852559552139,37.4056877138083,-15.9155248418178));
#52815=CARTESIAN_POINT('Ctrl Pts',(5.82277787197035,37.4520779924035,-15.4384344431652));
#52816=CARTESIAN_POINT('Ctrl Pts',(5.49476863526362,37.4567795900761,-15.5621468243714));
#52817=CARTESIAN_POINT('Ctrl Pts',(5.49929607838327,37.4585169113888,-15.9127047089119));
#52818=CARTESIAN_POINT('Ctrl Pts',(5.82361937406439,37.5625395576871,-15.438117035061));
#52819=CARTESIAN_POINT('Ctrl Pts',(5.49909810504416,37.5635003468084,-15.5605340956755));
#52820=CARTESIAN_POINT('Ctrl Pts',(5.50008426225533,37.5639723612738,-15.9073715669842));
#52821=CARTESIAN_POINT('Ctrl Pts',(5.82363950904436,37.6177133458351,-15.438109438589));
#52822=CARTESIAN_POINT('Ctrl Pts',(5.5008542982352,37.6168225419558,-15.5598720284282));
#52823=CARTESIAN_POINT('Ctrl Pts',(5.50010312136638,37.6166386057181,-15.9048561966123));
#52824=CARTESIAN_POINT('Ctrl Pts',(5.8217154307924,37.893294229626,-15.4388351940587));
#52825=CARTESIAN_POINT('Ctrl Pts',(5.50752491944064,37.881853217054,-15.5573104201885));
#52826=CARTESIAN_POINT('Ctrl Pts',(5.49830095467151,37.8796590971548,-15.8930435523112));
#52827=CARTESIAN_POINT('Ctrl Pts',(5.8137104043734,38.1128388502149,-15.4418594419708));
#52828=CARTESIAN_POINT('Ctrl Pts',(5.50636898532151,38.0944392377558,-15.5575651542258));
#52829=CARTESIAN_POINT('Ctrl Pts',(5.49080313325399,38.0890827853353,-15.886038511744));
#52830=CARTESIAN_POINT('Ctrl Pts',(5.7840049154644,38.5499825598019,-15.4530106720142));
#52831=CARTESIAN_POINT('Ctrl Pts',(5.48999166329811,38.5177567680441,-15.5630532663817));
#52832=CARTESIAN_POINT('Ctrl Pts',(5.46297981094671,38.5058340924418,-15.8771352552735));
#52833=CARTESIAN_POINT('Ctrl Pts',(5.76230703860224,38.7675819658764,-15.4611377904124));
#52834=CARTESIAN_POINT('Ctrl Pts',(5.47493356768806,38.7287614510696,-15.568229955048));
#52835=CARTESIAN_POINT('Ctrl Pts',(5.44265672992744,38.7131620074787,-15.8752371590965));
#52836=CARTESIAN_POINT('Ctrl Pts',(5.70407395336722,39.2006823460781,-15.4827163158072));
#52837=CARTESIAN_POINT('Ctrl Pts',(5.42972855746396,39.1486876692357,-15.5837780636752));
#52838=CARTESIAN_POINT('Ctrl Pts',(5.38811334519547,39.1255654423464,-15.8767726336669));
#52839=CARTESIAN_POINT('Ctrl Pts',(5.66754335828454,39.4161838894492,-15.4961678890182));
#52840=CARTESIAN_POINT('Ctrl Pts',(5.39972357971351,39.3578660216,-15.5941025574047));
#52841=CARTESIAN_POINT('Ctrl Pts',(5.35389735978674,39.3306414973316,-15.88020634219));
#52842=CARTESIAN_POINT('Ctrl Pts',(5.60039918974671,39.7377021629651,-15.5205056507883));
#52843=CARTESIAN_POINT('Ctrl Pts',(5.34213771584874,39.6706104721975,-15.6136918367253));
#52844=CARTESIAN_POINT('Ctrl Pts',(5.29100750584286,39.6364055190875,-15.8895273598811));
#52845=CARTESIAN_POINT('Ctrl Pts',(5.57595554966988,39.8445853883982,-15.5293116329089));
#52846=CARTESIAN_POINT('Ctrl Pts',(5.32093394283459,39.7743589127886,-15.6208743387635));
#52847=CARTESIAN_POINT('Ctrl Pts',(5.26811263571756,39.7380180145649,-15.8933294601772));
#52848=CARTESIAN_POINT('Ctrl Pts',(5.53599851525571,40.004450203368,-15.5435813267104));
#52849=CARTESIAN_POINT('Ctrl Pts',(5.28579906825781,39.929705256497,-15.632690927334));
#52850=CARTESIAN_POINT('Ctrl Pts',(5.23068731473301,39.8899479695032,-15.9000967087543));
#52851=CARTESIAN_POINT('Ctrl Pts',(5.5221305599358,40.0576617611033,-15.5485146750299));
#52852=CARTESIAN_POINT('Ctrl Pts',(5.27355459719845,39.9813594979742,-15.6367961486595));
#52853=CARTESIAN_POINT('Ctrl Pts',(5.2176980449392,39.9405097816184,-15.9025298069678));
#52854=CARTESIAN_POINT('Ctrl Pts',(5.50047699149048,40.1373603819414,-15.556182420383));
#52855=CARTESIAN_POINT('Ctrl Pts',(5.25432923497206,40.0587687077115,-15.6432168973992));
#52856=CARTESIAN_POINT('Ctrl Pts',(5.19741646594872,40.0162266424403,-15.9064481481372));
#52857=CARTESIAN_POINT('Ctrl Pts',(5.49311741536451,40.1639050501549,-15.5587828592327));
#52858=CARTESIAN_POINT('Ctrl Pts',(5.24778336468827,40.0845377385951,-15.6453990618431));
#52859=CARTESIAN_POINT('Ctrl Pts',(5.19052319892915,40.041442951149,-15.907799028716));
#52860=CARTESIAN_POINT('Ctrl Pts',(5.47814593729634,40.2168282263209,-15.5640605270417));
#52861=CARTESIAN_POINT('Ctrl Pts',(5.23443708951077,40.1359150171577,-15.649839332167));
#52862=CARTESIAN_POINT('Ctrl Pts',(5.17650032697911,40.0917133649177,-15.9105838634));
#52863=CARTESIAN_POINT('Ctrl Pts',(5.470529823742,40.2432224288697,-15.5667392494243));
#52864=CARTESIAN_POINT('Ctrl Pts',(5.22763310795184,40.1615391166161,-15.6520986436733));
#52865=CARTESIAN_POINT('Ctrl Pts',(5.16936677702167,40.1167823811518,-15.9120185729299));
#52866=CARTESIAN_POINT('Ctrl Pts',(5.40080286686056,40.4801601691466,-15.5912040190124));
#52867=CARTESIAN_POINT('Ctrl Pts',(5.1654386504834,40.3907259377088,-15.672707312104));
#52868=CARTESIAN_POINT('Ctrl Pts',(5.10405778192814,40.3418044912576,-15.9253090687417));
#52869=CARTESIAN_POINT('Ctrl Pts',(5.33043670111554,40.6864411445816,-15.6154875831029));
#52870=CARTESIAN_POINT('Ctrl Pts',(5.10156582395526,40.5911762940015,-15.6935809949587));
#52871=CARTESIAN_POINT('Ctrl Pts',(5.03815007775546,40.5375718116029,-15.9398148438705));
#52872=CARTESIAN_POINT('Ctrl Pts',(5.17171535959732,41.0898251595944,-15.6687704725657));
#52873=CARTESIAN_POINT('Ctrl Pts',(4.9558472522213,40.9828549133869,-15.739985220476));
#52874=CARTESIAN_POINT('Ctrl Pts',(4.88948546120424,40.9201248480408,-15.9738813871344));
#52875=CARTESIAN_POINT('Ctrl Pts',(5.08336558250042,41.2869305832741,-15.6977708167442));
#52876=CARTESIAN_POINT('Ctrl Pts',(4.87405064261176,41.1743746865059,-15.7655101753502));
#52877=CARTESIAN_POINT('Ctrl Pts',(4.80673360287453,41.1069127909073,-15.9934430495542));
#52878=CARTESIAN_POINT('Ctrl Pts',(4.88694399553687,41.671218731313,-15.7600251473423));
#52879=CARTESIAN_POINT('Ctrl Pts',(4.69092137437619,41.5474552367694,-15.8207627043341));
#52880=CARTESIAN_POINT('Ctrl Pts',(4.62275746195378,41.4708178044506,-16.0372007396695));
#52881=CARTESIAN_POINT('Ctrl Pts',(4.77888228918939,41.858405974228,-15.7932806671364));
#52882=CARTESIAN_POINT('Ctrl Pts',(4.58961749308463,41.7292760041513,-15.8504958068979));
#52883=CARTESIAN_POINT('Ctrl Pts',(4.5215426392795,41.6479391144314,-16.0613980705431));
#52884=CARTESIAN_POINT('Ctrl Pts',(4.64482519461143,42.0628061930575,-15.8327458139082));
#52885=CARTESIAN_POINT('Ctrl Pts',(4.46310917160174,41.9280541129356,-15.8860546410961));
#52886=CARTESIAN_POINT('Ctrl Pts',(4.39597952121523,41.8412001847982,-16.0909199817576));
#52887=CARTESIAN_POINT('Ctrl Pts',(4.62976965412125,42.0854096858801,-15.8371551458627));
#52888=CARTESIAN_POINT('Ctrl Pts',(4.44892446825342,41.9499886943975,-15.8900217942609));
#52889=CARTESIAN_POINT('Ctrl Pts',(4.38187791293436,41.8625697484028,-16.0942290007409));
#52890=CARTESIAN_POINT('Ctrl Pts',(4.59939878543121,42.1303067904093,-15.8460020502624));
#52891=CARTESIAN_POINT('Ctrl Pts',(4.42029652797858,41.9935550766478,-15.8979866657635));
#52892=CARTESIAN_POINT('Ctrl Pts',(4.35343136929109,41.9050117576583,-16.1008888977657));
#52893=CARTESIAN_POINT('Ctrl Pts',(4.58407427222009,42.1526144588579,-15.8504423301015));
#52894=CARTESIAN_POINT('Ctrl Pts',(4.40584455629757,42.0152010592343,-15.9019868666117));
#52895=CARTESIAN_POINT('Ctrl Pts',(4.3390778307107,41.9260974941438,-16.1042417996911));
#52896=CARTESIAN_POINT('Ctrl Pts',(4.53768208250935,42.2191142602777,-15.8638103017682));
#52897=CARTESIAN_POINT('Ctrl Pts',(4.36208642108868,42.0797067591165,-15.914033937939));
#52898=CARTESIAN_POINT('Ctrl Pts',(4.2956250910933,41.9889485291262,-16.1143660947964));
#52899=CARTESIAN_POINT('Ctrl Pts',(4.50619581303838,42.2628832431857,-15.8727851349316));
#52900=CARTESIAN_POINT('Ctrl Pts',(4.33235251838812,42.1221742523451,-15.9221344733298));
#52901=CARTESIAN_POINT('Ctrl Pts',(4.26613381932855,42.0303077037197,-16.121203084525));
#52902=CARTESIAN_POINT('Ctrl Pts',(4.41004926624052,42.3924912295783,-15.8998710702299));
#52903=CARTESIAN_POINT('Ctrl Pts',(4.24153152750805,42.2478448168248,-15.9465961576241));
#52904=CARTESIAN_POINT('Ctrl Pts',(4.1760792026318,42.1527559308387,-16.1419500461017));
#52905=CARTESIAN_POINT('Ctrl Pts',(4.34370225939985,42.4766322174293,-15.9181437877767));
#52906=CARTESIAN_POINT('Ctrl Pts',(4.17872361398144,42.3294747743511,-15.9631463234755));
#52907=CARTESIAN_POINT('Ctrl Pts',(4.11393600041315,42.2322165809747,-16.1560961451583));
#52908=CARTESIAN_POINT('Ctrl Pts',(4.13777251537753,42.7221794291726,-15.9733854419649));
#52909=CARTESIAN_POINT('Ctrl Pts',(3.98370692807761,42.5673833142134,-16.0132260504743));
#52910=CARTESIAN_POINT('Ctrl Pts',(3.92105414688791,42.4640154815466,-16.1992634768941));
#52911=CARTESIAN_POINT('Ctrl Pts',(3.99132195149594,42.8767293832158,-16.0107821043782));
#52912=CARTESIAN_POINT('Ctrl Pts',(3.84451111612512,42.7173047864165,-16.0473039779341));
#52913=CARTESIAN_POINT('Ctrl Pts',(3.78388281919657,42.6097890780496,-16.2290170151344));
#52914=CARTESIAN_POINT('Ctrl Pts',(3.75700972962784,43.0941951466418,-16.0667771043254));
#52915=CARTESIAN_POINT('Ctrl Pts',(3.62129524685035,42.9281698633173,-16.0984923203175));
#52916=CARTESIAN_POINT('Ctrl Pts',(3.56441682684187,42.8147476794126,-16.2742016702415));
#52917=CARTESIAN_POINT('Ctrl Pts',(3.67646144559015,43.1642860455141,-16.0854244903344));
#52918=CARTESIAN_POINT('Ctrl Pts',(3.54454660494019,42.9960786893441,-16.115553648241));
#52919=CARTESIAN_POINT('Ctrl Pts',(3.48897215266966,42.8807793342241,-16.2893548851606));
#52920=CARTESIAN_POINT('Ctrl Pts',(3.55180835016696,43.2656968454944,-16.1132389634261));
#52921=CARTESIAN_POINT('Ctrl Pts',(3.42566053370466,43.0943214418982,-16.1410401047175));
#52922=CARTESIAN_POINT('Ctrl Pts',(3.37221718759655,42.9762779466704,-16.3121000330166));
#52923=CARTESIAN_POINT('Ctrl Pts',(3.50961052575669,43.2988851470272,-16.122485966165));
#52924=CARTESIAN_POINT('Ctrl Pts',(3.38541262458361,43.1264600581356,-16.1495163495703));
#52925=CARTESIAN_POINT('Ctrl Pts',(3.33269305445803,43.0075246336688,-16.3196856337079));
#52926=CARTESIAN_POINT('Ctrl Pts',(3.4239361870611,43.3639679820918,-16.1408977680494));
#52927=CARTESIAN_POINT('Ctrl Pts',(3.30367271591507,43.189473362121,-16.1664034224739));
#52928=CARTESIAN_POINT('Ctrl Pts',(3.25244711732724,43.0687868973452,-16.3348347973778));
#52929=CARTESIAN_POINT('Ctrl Pts',(3.38069422093024,43.3956846955611,-16.1500121560905));
#52930=CARTESIAN_POINT('Ctrl Pts',(3.26240299114715,43.2201782549395,-16.1747684968875));
#52931=CARTESIAN_POINT('Ctrl Pts',(3.21194500033968,43.0986350973994,-16.3423568657999));
#52932=CARTESIAN_POINT('Ctrl Pts',(3.16247293665689,43.5501883769039,-16.1950777040967));
#52933=CARTESIAN_POINT('Ctrl Pts',(3.05423596689228,43.3696142664887,-16.2161210510762));
#52934=CARTESIAN_POINT('Ctrl Pts',(3.00755040891255,43.2440053764108,-16.3796546335878));
#52935=CARTESIAN_POINT('Ctrl Pts',(2.98147832252801,43.660776482398,-16.2295084233055));
#52936=CARTESIAN_POINT('Ctrl Pts',(2.88121816202138,43.4766418873115,-16.2478293654573));
#52937=CARTESIAN_POINT('Ctrl Pts',(2.83802377309921,43.3479542916528,-16.4084895185999));
#52938=CARTESIAN_POINT('Ctrl Pts',(2.70037397572554,43.8074863821001,-16.277807578224));
#52939=CARTESIAN_POINT('Ctrl Pts',(2.61232205384454,43.6184982166501,-16.2923899551782));
#52940=CARTESIAN_POINT('Ctrl Pts',(2.57473044561691,43.4857336160062,-16.4493217081974));
#52941=CARTESIAN_POINT('Ctrl Pts',(2.60506670587299,43.8531862697985,-16.2933497575293));
#52942=CARTESIAN_POINT('Ctrl Pts',(2.52114721824606,43.6626594710407,-16.3067415552332));
#52943=CARTESIAN_POINT('Ctrl Pts',(2.48546192830491,43.528628365131,-16.4625297245561));
#52944=CARTESIAN_POINT('Ctrl Pts',(2.41119452256951,43.9381353686842,-16.3231663545269));
#52945=CARTESIAN_POINT('Ctrl Pts',(2.3356478240054,43.7447042632128,-16.3342999073));
#52946=CARTESIAN_POINT('Ctrl Pts',(2.3038736575641,43.6083197721399,-16.4879921624111));
#52947=CARTESIAN_POINT('Ctrl Pts',(2.31262977609044,43.9773848957545,-16.3374408791774));
#52948=CARTESIAN_POINT('Ctrl Pts',(2.24131140491693,43.7825970865653,-16.3475093049691));
#52949=CARTESIAN_POINT('Ctrl Pts',(2.21155406016932,43.6451167254636,-16.5002466751902));
#52950=CARTESIAN_POINT('Ctrl Pts',(2.16227751834144,44.0313312810579,-16.3577844977291));
#52951=CARTESIAN_POINT('Ctrl Pts',(2.09738048924219,43.8346499499766,-16.3663562334774));
#52952=CARTESIAN_POINT('Ctrl Pts',(2.07072825413426,43.6956582712672,-16.5178019271295));
#52953=CARTESIAN_POINT('Ctrl Pts',(2.11174227376284,44.0484914663749,-16.3643876348749));
#52954=CARTESIAN_POINT('Ctrl Pts',(2.04900260649854,43.8512017716587,-16.3724769498617));
#52955=CARTESIAN_POINT('Ctrl Pts',(2.02339496711712,43.7117292100671,-16.523515913095));
#52956=CARTESIAN_POINT('Ctrl Pts',(2.03530194931424,44.072981459843,-16.3740100616474));
#52957=CARTESIAN_POINT('Ctrl Pts',(1.97581878875163,43.8748161029352,-16.3814021297576));
#52958=CARTESIAN_POINT('Ctrl Pts',(1.95179796907649,43.7346553851609,-16.5318661099767));
#52959=CARTESIAN_POINT('Ctrl Pts',(2.00971557668972,44.0809363660402,-16.3771704866985));
#52960=CARTESIAN_POINT('Ctrl Pts',(1.95132227885587,43.8824850165059,-16.3843344340238));
#52961=CARTESIAN_POINT('Ctrl Pts',(1.92783277153264,43.742100695679,-16.5346127099434));
#52962=CARTESIAN_POINT('Ctrl Pts',(1.95832824291746,44.0964258747234,-16.3833946525917));
#52963=CARTESIAN_POINT('Ctrl Pts',(1.90212235254287,43.8974148464812,-16.3901112587382));
#52964=CARTESIAN_POINT('Ctrl Pts',(1.87970138457326,43.7565946460749,-16.5400299284974));
#52965=CARTESIAN_POINT('Ctrl Pts',(1.93251110054407,44.1039650287676,-16.3864602701835));
#52966=CARTESIAN_POINT('Ctrl Pts',(1.87740326220016,43.9046802305651,-16.392957550475));
#52967=CARTESIAN_POINT('Ctrl Pts',(1.85552003909345,43.7636475423924,-16.5427021859492));
#52968=CARTESIAN_POINT('Ctrl Pts',(1.8030633147258,44.1405497707181,-16.4015192016935));
#52969=CARTESIAN_POINT('Ctrl Pts',(1.75346736507588,43.9399264952154,-16.4069429652539));
#52970=CARTESIAN_POINT('Ctrl Pts',(1.73427417901659,43.7978641021233,-16.5558492664266));
#52971=CARTESIAN_POINT('Ctrl Pts',(1.69906639420128,44.1660683153088,-16.4126226120353));
#52972=CARTESIAN_POINT('Ctrl Pts',(1.65387335486775,43.9644920355918,-16.417272571238));
#52973=CARTESIAN_POINT('Ctrl Pts',(1.63686659515066,43.8217027186776,-16.5656092158287));
#52974=CARTESIAN_POINT('Ctrl Pts',(1.49021426166529,44.2098252495483,-16.4329020282884));
#52975=CARTESIAN_POINT('Ctrl Pts',(1.45386135654879,44.0065631227143,-16.4361701532582));
#52976=CARTESIAN_POINT('Ctrl Pts',(1.44124751778221,43.862520976467,-16.5835644832772));
#52977=CARTESIAN_POINT('Ctrl Pts',(1.38535902634819,44.2280633796216,-16.4420780728859));
#52978=CARTESIAN_POINT('Ctrl Pts',(1.35343204203413,44.0240714574058,-16.4447394017829));
#52979=CARTESIAN_POINT('Ctrl Pts',(1.34303600264843,43.8795003686096,-16.5917598520244));
#52980=CARTESIAN_POINT('Ctrl Pts',(1.17479908853176,44.2573750378148,-16.4584628106134));
#52981=CARTESIAN_POINT('Ctrl Pts',(1.15176493152459,44.0521448192979,-16.4600782830589));
#52982=CARTESIAN_POINT('Ctrl Pts',(1.14581732809311,43.906712349358,-16.6065414193849));
#52983=CARTESIAN_POINT('Ctrl Pts',(1.06909438111656,44.2684484921629,-16.4656715398477));
#52984=CARTESIAN_POINT('Ctrl Pts',(1.05051664045048,44.0627110998794,-16.4668487116589));
#52985=CARTESIAN_POINT('Ctrl Pts',(1.04681016412825,43.9169448659429,-16.6131276573267));
#52986=CARTESIAN_POINT('Ctrl Pts',(0.856834555596582,44.2834493850702,-16.4780804888865));
#52987=CARTESIAN_POINT('Ctrl Pts',(0.847217272305147,44.0769219395685,-16.4785516187993));
#52988=CARTESIAN_POINT('Ctrl Pts',(0.847999308275245,43.9306827648361,-16.6246496409757));
#52989=CARTESIAN_POINT('Ctrl Pts',(0.750279450442107,44.2873769285557,-16.4832807449414));
#52990=CARTESIAN_POINT('Ctrl Pts',(0.745156101872444,44.0805664549735,-16.483484482518));
#52991=CARTESIAN_POINT('Ctrl Pts',(0.748195628510673,43.9341882452755,-16.62958541764));
#52992=CARTESIAN_POINT('Ctrl Pts',(0.58980086051462,44.2878495874714,-16.4895421642784));
#52993=CARTESIAN_POINT('Ctrl Pts',(0.591467911154747,44.0807865596362,-16.4894752008505));
#52994=CARTESIAN_POINT('Ctrl Pts',(0.597885103513613,43.9343461853688,-16.6357218580272));
#52995=CARTESIAN_POINT('Ctrl Pts',(0.536200263354332,44.2871032596941,-16.4913727887242));
#52996=CARTESIAN_POINT('Ctrl Pts',(0.540132926138202,44.0799845128224,-16.4912375073698));
#52997=CARTESIAN_POINT('Ctrl Pts',(0.547680687440361,43.9335480497144,-16.6375561481366));
#52998=CARTESIAN_POINT('Ctrl Pts',(0.455636014550893,44.284613337201,-16.4937296454446));
#52999=CARTESIAN_POINT('Ctrl Pts',(0.462979747202555,44.0774546459417,-16.4935249270376));
#53000=CARTESIAN_POINT('Ctrl Pts',(0.47222106046037,43.9310609294277,-16.6399872269088));
#53001=CARTESIAN_POINT('Ctrl Pts',(0.428754034222533,44.2835549068502,-16.4944504159164));
#53002=CARTESIAN_POINT('Ctrl Pts',(0.437235366462993,44.0763900837954,-16.4942280935165));
#53003=CARTESIAN_POINT('Ctrl Pts',(0.447042346105144,43.9300168543709,-16.6407441942414));
#53004=CARTESIAN_POINT('Ctrl Pts',(0.388389950057066,44.2816222765731,-16.4954337434013));
#53005=CARTESIAN_POINT('Ctrl Pts',(0.398580882778724,44.0744592385522,-16.4951933304063));
#53006=CARTESIAN_POINT('Ctrl Pts',(0.409235765892974,43.9281260198428,-16.6417991152495));
#53007=CARTESIAN_POINT('Ctrl Pts',(0.374928402732455,44.2809205658472,-16.4957452143992));
#53008=CARTESIAN_POINT('Ctrl Pts',(0.385689351820399,44.0737599283669,-16.4955001651808));
#53009=CARTESIAN_POINT('Ctrl Pts',(0.396627154075427,43.9274416182168,-16.6421373338812));
#53010=CARTESIAN_POINT('Ctrl Pts',(0.347991554057913,44.2794017185444,-16.4963354525741));
#53011=CARTESIAN_POINT('Ctrl Pts',(0.359893363301771,44.072249540534,-16.4960839175124));
#53012=CARTESIAN_POINT('Ctrl Pts',(0.371397047876984,43.9259641674669,-16.6427868545954));
#53013=CARTESIAN_POINT('Ctrl Pts',(0.334532328343637,44.2785856289167,-16.4966139069159));
#53014=CARTESIAN_POINT('Ctrl Pts',(0.347004279162573,44.0714394948401,-16.496360523009));
#53015=CARTESIAN_POINT('Ctrl Pts',(0.358790610672238,43.925172130238,-16.6430978003365));
#53016=CARTESIAN_POINT('Ctrl Pts',(0.321034048597817,44.2777095070773,-16.496876587392));
#53017=CARTESIAN_POINT('Ctrl Pts',(0.334078182671872,44.0705712895835,-16.4966227447236));
#53018=CARTESIAN_POINT('Ctrl Pts',(0.346147593727982,43.9243235322772,-16.6433959637249));
#53019=CARTESIAN_POINT('',(0.730430568056981,29.0999736046314,-17.3364718010719));
#53020=CARTESIAN_POINT('Origin',(0.753473624776453,28.7467958754239,-16.9832940708441));
#53021=CARTESIAN_POINT('',(0.500000000000003,43.9319757376251,-16.6390920749471));
#53022=CARTESIAN_POINT('Ctrl Pts',(0.499999999999999,43.9319757373861,-16.6390920747081));
#53023=CARTESIAN_POINT('Ctrl Pts',(0.54757507396084,43.9335156191108,-16.637552201127));
#53024=CARTESIAN_POINT('Ctrl Pts',(0.595061829101537,43.9342864984895,-16.6358212644215));
#53025=CARTESIAN_POINT('Ctrl Pts',(0.642461141705286,43.9342958947873,-16.6339011638695));
#53026=CARTESIAN_POINT('Ctrl Pts',(0.644303763883716,43.9342962600632,-16.6338265210178));
#53027=CARTESIAN_POINT('Ctrl Pts',(0.646146253911932,43.9342954745885,-16.6337515922788));
#53028=CARTESIAN_POINT('Ctrl Pts',(0.647988611841277,43.9342935388005,-16.6336763777689));
#53029=CARTESIAN_POINT('Ctrl Pts',(0.748182861165585,43.9341882634795,-16.6295859340796));
#53030=CARTESIAN_POINT('Ctrl Pts',(0.847986714017941,43.9306837682061,-16.6246502377895));
#53031=CARTESIAN_POINT('Ctrl Pts',(0.947404736988193,43.9238138935806,-16.6188885708602));
#53032=CARTESIAN_POINT('Ctrl Pts',(0.94901269818106,43.9237027820189,-16.6187953831609));
#53033=CARTESIAN_POINT('Ctrl Pts',(0.950620558440654,43.923590790085,-16.618701979389));
#53034=CARTESIAN_POINT('Ctrl Pts',(0.952228317766542,43.923477917725,-16.6186083596307));
#53035=CARTESIAN_POINT('Ctrl Pts',(1.05000098985128,43.9166138106022,-16.6129150610295));
#53036=CARTESIAN_POINT('Ctrl Pts',(1.14740041286262,43.9064940712208,-16.6064226132333));
#53037=CARTESIAN_POINT('Ctrl Pts',(1.24442667068965,43.8931064533492,-16.5991505402067));
#53038=CARTESIAN_POINT('Ctrl Pts',(1.24945646130347,43.8924124462194,-16.5987735597328));
#53039=CARTESIAN_POINT('Ctrl Pts',(1.25448524909501,43.8917096574055,-16.5983944840538));
#53040=CARTESIAN_POINT('Ctrl Pts',(1.25951303346151,43.8909980790404,-16.5980133161075));
#53041=CARTESIAN_POINT('Ctrl Pts',(1.35304288501814,43.8777608727477,-16.5909226020196));
#53042=CARTESIAN_POINT('Ctrl Pts',(1.44622544709215,43.8614824877767,-16.5831073592102));
#53043=CARTESIAN_POINT('Ctrl Pts',(1.53905706853458,43.8421119644684,-16.5745867290311));
#53044=CARTESIAN_POINT('Ctrl Pts',(1.54747921114386,43.8403545750445,-16.5738136954314));
#53045=CARTESIAN_POINT('Ctrl Pts',(1.55589846523983,43.8385717359699,-16.573034855426));
#53046=CARTESIAN_POINT('Ctrl Pts',(1.56431482499405,43.836763377988,-16.5722502247802));
#53047=CARTESIAN_POINT('Ctrl Pts',(1.61490694532871,43.8258930412507,-16.5675336811424));
#53048=CARTESIAN_POINT('Ctrl Pts',(1.66539452408273,43.8141007838391,-16.5626077013854));
#53049=CARTESIAN_POINT('Ctrl Pts',(1.71577613901276,43.801371606282,-16.5574757157637));
#53050=CARTESIAN_POINT('Ctrl Pts',(1.74096694647778,43.7950070175034,-16.5549097229528));
#53051=CARTESIAN_POINT('Ctrl Pts',(1.76613180612446,43.7884080514811,-16.5522921712238));
#53052=CARTESIAN_POINT('Ctrl Pts',(1.79126896359321,43.7815732750681,-16.5496236439717));
#53053=CARTESIAN_POINT('Ctrl Pts',(1.80462156274624,43.7779427122307,-16.5482061497792));
#53054=CARTESIAN_POINT('Ctrl Pts',(1.81795404850408,43.774248976217,-16.5467755794718));
#53055=CARTESIAN_POINT('Ctrl Pts',(1.83127086873843,43.7704908653263,-16.5453315904083));
#53056=CARTESIAN_POINT('Ctrl Pts',(1.8430238497748,43.7671740820963,-16.5440571738599));
#53057=CARTESIAN_POINT('Ctrl Pts',(1.85475472764573,43.7638098150535,-16.542773365422));
#53058=CARTESIAN_POINT('Ctrl Pts',(1.8664611512278,43.7603990665573,-16.5414805958159));
#53059=CARTESIAN_POINT('Ctrl Pts',(1.87892371112219,43.7567680124509,-16.5401043241876));
#53060=CARTESIAN_POINT('Ctrl Pts',(1.89136121499753,43.7530834984364,-16.5387175946662));
#53061=CARTESIAN_POINT('Ctrl Pts',(1.90376708010395,43.7493476834398,-16.5373213058091));
#53062=CARTESIAN_POINT('Ctrl Pts',(1.92783628123464,43.7420996534339,-16.5346123002663));
#53063=CARTESIAN_POINT('Ctrl Pts',(1.95180155045399,43.7346542585673,-16.5318656721187));
#53064=CARTESIAN_POINT('Ctrl Pts',(1.9756636395166,43.727013352029,-16.5290826838497));
#53065=CARTESIAN_POINT('Ctrl Pts',(2.02341050023379,43.711724275734,-16.523514061886));
#53066=CARTESIAN_POINT('Ctrl Pts',(2.07074432095206,43.6956525615114,-16.5177998678728));
#53067=CARTESIAN_POINT('Ctrl Pts',(2.11767019917302,43.6788111378344,-16.5119501232939));
#53068=CARTESIAN_POINT('Ctrl Pts',(2.1320820175734,43.6736388203661,-16.5101535568842));
#53069=CARTESIAN_POINT('Ctrl Pts',(2.14645538566519,43.6683939604828,-16.5083442063354));
#53070=CARTESIAN_POINT('Ctrl Pts',(2.16079040024107,43.6630768264416,-16.5065223583721));
#53071=CARTESIAN_POINT('Ctrl Pts',(2.2399049257387,43.6337317194346,-16.4964676328341));
#53072=CARTESIAN_POINT('Ctrl Pts',(2.31785505285204,43.6021840003903,-16.4860316105865));
#53073=CARTESIAN_POINT('Ctrl Pts',(2.39466780777821,43.5684741281802,-16.4752608753432));
#53074=CARTESIAN_POINT('Ctrl Pts',(2.41141236199445,43.5611256509202,-16.4729129428885));
#53075=CARTESIAN_POINT('Ctrl Pts',(2.4281028618955,43.5536744165793,-16.4705491005035));
#53076=CARTESIAN_POINT('Ctrl Pts',(2.44473947828146,43.5461206147242,-16.4681698275028));
#53077=CARTESIAN_POINT('Ctrl Pts',(2.51837530250979,43.5126865069253,-16.4576388562759));
#53078=CARTESIAN_POINT('Ctrl Pts',(2.59095573626851,43.4772437713182,-16.4468047325651));
#53079=CARTESIAN_POINT('Ctrl Pts',(2.66249507797947,43.4398078078865,-16.4357102161998));
#53080=CARTESIAN_POINT('Ctrl Pts',(2.6812634654843,43.4299864613169,-16.4327995634409));
#53081=CARTESIAN_POINT('Ctrl Pts',(2.69996035641465,43.4200282774449,-16.4298709581876));
#53082=CARTESIAN_POINT('Ctrl Pts',(2.71858578544062,43.4099330595632,-16.4269251921389));
#53083=CARTESIAN_POINT('Ctrl Pts',(2.80820564226487,43.3613579647343,-16.4127510686246));
#53084=CARTESIAN_POINT('Ctrl Pts',(2.89617177777919,43.3096119447071,-16.3981772518944));
#53085=CARTESIAN_POINT('Ctrl Pts',(2.98248669111425,43.2546769047821,-16.3832893654412));
#53086=CARTESIAN_POINT('Ctrl Pts',(3.04624678339623,43.2140968580695,-16.3722918103552));
#53087=CARTESIAN_POINT('Ctrl Pts',(3.10910599739674,43.1717766342996,-16.3611228479354));
#53088=CARTESIAN_POINT('Ctrl Pts',(3.17106608205426,43.1277091532017,-16.3498164193575));
#53089=CARTESIAN_POINT('Ctrl Pts',(3.19298415920671,43.1121204971184,-16.3458168255019));
#53090=CARTESIAN_POINT('Ctrl Pts',(3.21478940308917,43.0963124984015,-16.3418000833344));
#53091=CARTESIAN_POINT('Ctrl Pts',(3.23648155363809,43.0802841038743,-16.337767760884));
#53092=CARTESIAN_POINT('Ctrl Pts',(3.25526256696086,43.0664067572977,-16.3342765855167));
#53093=CARTESIAN_POINT('Ctrl Pts',(3.27395704672654,43.0523655430299,-16.3307740629455));
#53094=CARTESIAN_POINT('Ctrl Pts',(3.29257008801342,43.0381557703974,-16.327260208633));
#53095=CARTESIAN_POINT('Ctrl Pts',(3.29452482545658,43.036663463246,-16.326891184437));
#53096=CARTESIAN_POINT('Ctrl Pts',(3.29647814310812,43.0351696939639,-16.3265221337238));
#53097=CARTESIAN_POINT('Ctrl Pts',(3.2984300462081,43.0336744612953,-16.3261530570622));
#53098=CARTESIAN_POINT('Ctrl Pts',(3.31896800193379,43.0179415991738,-16.32226962651));
#53099=CARTESIAN_POINT('Ctrl Pts',(3.33933859097246,43.0020550620894,-16.31838528869));
#53100=CARTESIAN_POINT('Ctrl Pts',(3.35954417450593,42.9860167729483,-16.3145016519096));
#53101=CARTESIAN_POINT('Ctrl Pts',(3.37686185179866,42.9722707747091,-16.311173088378));
#53102=CARTESIAN_POINT('Ctrl Pts',(3.3940591510392,42.9584126400607,-16.3078448597278));
#53103=CARTESIAN_POINT('Ctrl Pts',(3.41113553968154,42.9444451416336,-16.3045182205045));
#53104=CARTESIAN_POINT('Ctrl Pts',(3.43390726592552,42.9258191863946,-16.3000820765813));
#53105=CARTESIAN_POINT('Ctrl Pts',(3.45646665672014,42.9069969381795,-16.2956483038387));
#53106=CARTESIAN_POINT('Ctrl Pts',(3.47881642783259,42.8879810486537,-16.2912189212696));
#53107=CARTESIAN_POINT('Ctrl Pts',(3.53295111922232,42.8419215473818,-16.2804902539728));
#53108=CARTESIAN_POINT('Ctrl Pts',(3.58585566131758,42.7947261750183,-16.2697875919548));
#53109=CARTESIAN_POINT('Ctrl Pts',(3.63757222655503,42.7464282781409,-16.2591399074602));
#53110=CARTESIAN_POINT('Ctrl Pts',(3.66058117518797,42.7249403115052,-16.2544027014128));
#53111=CARTESIAN_POINT('Ctrl Pts',(3.6833554158427,42.703234527098,-16.2496764460396));
#53112=CARTESIAN_POINT('Ctrl Pts',(3.70589760765789,42.6813128786821,-16.2449634978511));
#53113=CARTESIAN_POINT('Ctrl Pts',(3.77910724856877,42.6101185590761,-16.2296573888739));
#53114=CARTESIAN_POINT('Ctrl Pts',(3.84987008319856,42.5366475241466,-16.2144909403196));
#53115=CARTESIAN_POINT('Ctrl Pts',(3.91827600714043,42.4609673017849,-16.1995435117613));
#53116=CARTESIAN_POINT('Ctrl Pts',(3.96306685152826,42.4114133908412,-16.189756231538));
#53117=CARTESIAN_POINT('Ctrl Pts',(4.00684717481627,42.3609123166451,-16.1800628313719));
#53118=CARTESIAN_POINT('Ctrl Pts',(4.04964204923807,42.3094828811653,-16.1704852557369));
#53119=CARTESIAN_POINT('Ctrl Pts',(4.07220479342806,42.2823677368346,-16.1654356699645));
#53120=CARTESIAN_POINT('Ctrl Pts',(4.0944930048392,42.2549939657261,-16.1604181756657));
#53121=CARTESIAN_POINT('Ctrl Pts',(4.11650923860563,42.2273632732543,-16.1554357947868));
#53122=CARTESIAN_POINT('Ctrl Pts',(4.15730666926082,42.1761619064796,-16.1462031376228));
#53123=CARTESIAN_POINT('Ctrl Pts',(4.19717010962387,42.1240783986472,-16.1370910810339));
#53124=CARTESIAN_POINT('Ctrl Pts',(4.23611561389655,42.0711237796144,-16.1281187379831));
#53125=CARTESIAN_POINT('Ctrl Pts',(4.25804971753198,42.0412997441184,-16.1230655153839));
#53126=CARTESIAN_POINT('Ctrl Pts',(4.27969252966859,42.0111992773893,-16.1180565875598));
#53127=CARTESIAN_POINT('Ctrl Pts',(4.30104638713536,41.9808238526934,-16.1130952728204));
#53128=CARTESIAN_POINT('Ctrl Pts',(4.30893484767529,41.9696026792137,-16.1112624828616));
#53129=CARTESIAN_POINT('Ctrl Pts',(4.31678390039683,41.9583439471152,-16.1094361833301));
#53130=CARTESIAN_POINT('Ctrl Pts',(4.3245935860754,41.947047841699,-16.1076165589678));
#53131=CARTESIAN_POINT('Ctrl Pts',(4.33908272363761,41.9260904265059,-16.1042406500284));
#53132=CARTESIAN_POINT('Ctrl Pts',(4.35343634228928,41.9050043553989,-16.1008877162269));
#53133=CARTESIAN_POINT('Ctrl Pts',(4.36765465067981,41.8837907656036,-16.0975589201664));
#53134=CARTESIAN_POINT('Ctrl Pts',(4.37456285478427,41.8734837864561,-16.095941568652));
#53135=CARTESIAN_POINT('Ctrl Pts',(4.38144114610487,41.8631435705445,-16.0943294377919));
#53136=CARTESIAN_POINT('Ctrl Pts',(4.38828623834093,41.8527753534199,-16.0927234372925));
#53137=CARTESIAN_POINT('Ctrl Pts',(4.3954180381469,41.8419728621857,-16.0910501692552));
#53138=CARTESIAN_POINT('Ctrl Pts',(4.40251835272474,41.831132964736,-16.0893825383176));
#53139=CARTESIAN_POINT('Ctrl Pts',(4.40957575112323,41.8202734186026,-16.0877232796263));
#53140=CARTESIAN_POINT('Ctrl Pts',(4.40969417252988,41.8200911980936,-16.0876954376742));
#53141=CARTESIAN_POINT('Ctrl Pts',(4.40981258274751,41.8199089706728,-16.0876675978901));
#53142=CARTESIAN_POINT('Ctrl Pts',(4.40993098176058,41.8197267363653,-16.0876397602783));
#53143=CARTESIAN_POINT('Ctrl Pts',(4.41686864658674,41.8090486022141,-16.0860085978618));
#53144=CARTESIAN_POINT('Ctrl Pts',(4.42376480089258,41.7983519052827,-16.0843856692356));
#53145=CARTESIAN_POINT('Ctrl Pts',(4.4306200950024,41.7876363110569,-16.082770920866));
#53146=CARTESIAN_POINT('Ctrl Pts',(4.50034296874691,41.6786516327428,-16.0663478622927));
#53147=CARTESIAN_POINT('Ctrl Pts',(4.56582956218176,41.5677267230489,-16.0507749291748));
#53148=CARTESIAN_POINT('Ctrl Pts',(4.62741559217832,41.4550012090001,-16.0361118852648));
#53149=CARTESIAN_POINT('Ctrl Pts',(4.6574401945597,41.4000449350247,-16.0289633149945));
#53150=CARTESIAN_POINT('Ctrl Pts',(4.686537451899,41.3446609425631,-16.022030998685));
#53151=CARTESIAN_POINT('Ctrl Pts',(4.71474554668843,41.288865313039,-16.0153218476222));
#53152=CARTESIAN_POINT('Ctrl Pts',(4.73282548062373,41.2531031921583,-16.0110216278136));
#53153=CARTESIAN_POINT('Ctrl Pts',(4.75053975868617,41.2171717968373,-16.0068130360076));
#53154=CARTESIAN_POINT('Ctrl Pts',(4.76789567688245,41.1810741471843,-16.0026974052181));
#53155=CARTESIAN_POINT('Ctrl Pts',(4.81233008924746,41.088657380065,-15.9921606169265));
#53156=CARTESIAN_POINT('Ctrl Pts',(4.85441591615076,40.9951507454576,-15.9822329668367));
#53157=CARTESIAN_POINT('Ctrl Pts',(4.89427385518969,40.9006052087616,-15.972936464702));
#53158=CARTESIAN_POINT('Ctrl Pts',(4.91825289509361,40.8437254188921,-15.9673435715162));
#53159=CARTESIAN_POINT('Ctrl Pts',(4.9414255696942,40.7864694656732,-15.9619791627489));
#53160=CARTESIAN_POINT('Ctrl Pts',(4.96381780586936,40.7288483629628,-15.9568479803831));
#53161=CARTESIAN_POINT('Ctrl Pts',(5.01586628024736,40.5949139731774,-15.9449210691176));
#53162=CARTESIAN_POINT('Ctrl Pts',(5.0636960184238,40.4590057943956,-15.934253853083));
#53163=CARTESIAN_POINT('Ctrl Pts',(5.10754371538125,40.3212231356076,-15.9248891748567));
#53164=CARTESIAN_POINT('Ctrl Pts',(5.12646876530576,40.2617549336898,-15.9208472977399));
#53165=CARTESIAN_POINT('Ctrl Pts',(5.1446505915391,40.201942005203,-15.9170483417049));
#53166=CARTESIAN_POINT('Ctrl Pts',(5.16211022828596,40.1417848426849,-15.9134952669358));
#53167=CARTESIAN_POINT('Ctrl Pts',(5.16936875516642,40.1167755949256,-15.9120181406304));
#53168=CARTESIAN_POINT('Ctrl Pts',(5.17650218662148,40.0917067297718,-15.9105834629293));
#53169=CARTESIAN_POINT('Ctrl Pts',(5.18351176949454,40.0665781629916,-15.9091914163543));
#53170=CARTESIAN_POINT('Ctrl Pts',(5.18757716154722,40.0520041893995,-15.9083840623097));
#53171=CARTESIAN_POINT('Ctrl Pts',(5.1916022197332,40.0374051221726,-15.9075907944438));
#53172=CARTESIAN_POINT('Ctrl Pts',(5.19558417075906,40.0227922606481,-15.9068122242068));
#53173=CARTESIAN_POINT('Ctrl Pts',(5.19847150744282,40.0121963867007,-15.9062476782363));
#53174=CARTESIAN_POINT('Ctrl Pts',(5.2013361339774,40.0015934265861,-15.9056908682819));
#53175=CARTESIAN_POINT('Ctrl Pts',(5.20417699410974,39.9909876901929,-15.9051420258653));
#53176=CARTESIAN_POINT('Ctrl Pts',(5.20806662989904,39.9764665768945,-15.9043905643337));
#53177=CARTESIAN_POINT('Ctrl Pts',(5.21191164472706,39.9619408105056,-15.9036540441075));
#53178=CARTESIAN_POINT('Ctrl Pts',(5.21571252195769,39.9474103684272,-15.9029324020479));
#53179=CARTESIAN_POINT('Ctrl Pts',(5.22228943303246,39.9222673765261,-15.9016836967186));
#53180=CARTESIAN_POINT('Ctrl Pts',(5.22873447988942,39.8971092606892,-15.9004794946389));
#53181=CARTESIAN_POINT('Ctrl Pts',(5.23505001568631,39.871936285293,-15.8993195153678));
#53182=CARTESIAN_POINT('Ctrl Pts',(5.23777825743765,39.8610618377893,-15.898818417127));
#53183=CARTESIAN_POINT('Ctrl Pts',(5.24048232982734,39.85018461934,-15.8983255720336));
#53184=CARTESIAN_POINT('Ctrl Pts',(5.24316242206404,39.8393046514301,-15.8978409575634));
#53185=CARTESIAN_POINT('Ctrl Pts',(5.25289048130553,39.7998131104588,-15.8960819291946));
#53186=CARTESIAN_POINT('Ctrl Pts',(5.26230280240304,39.7602853708674,-15.8944313398567));
#53187=CARTESIAN_POINT('Ctrl Pts',(5.27140738538964,39.7207223269442,-15.8928881139419));
#53188=CARTESIAN_POINT('Ctrl Pts',(5.28567394755738,39.6587284249165,-15.890469933067));
#53189=CARTESIAN_POINT('Ctrl Pts',(5.29918490214635,39.5966478567417,-15.8883153733681));
#53190=CARTESIAN_POINT('Ctrl Pts',(5.31197079084341,39.5344841787339,-15.8864203519859));
#53191=CARTESIAN_POINT('Ctrl Pts',(5.3408154874063,39.3942442257785,-15.8821452235183));
#53192=CARTESIAN_POINT('Ctrl Pts',(5.36597777759522,39.2535822868239,-15.8791908920713));
#53193=CARTESIAN_POINT('Ctrl Pts',(5.38773152176282,39.1125293717576,-15.8775113110921));
#53194=CARTESIAN_POINT('Ctrl Pts',(5.39764940999791,39.0482210377034,-15.8767455626166));
#53195=CARTESIAN_POINT('Ctrl Pts',(5.40685871578436,38.9838314856836,-15.8762448282014));
#53196=CARTESIAN_POINT('Ctrl Pts',(5.41538504850589,38.9193637310051,-15.8760048072301));
#53197=CARTESIAN_POINT('Ctrl Pts',(5.43385000474362,38.7797498656116,-15.8754850085222));
#53198=CARTESIAN_POINT('Ctrl Pts',(5.44911004070475,38.6397690160481,-15.8761878337851));
#53199=CARTESIAN_POINT('Ctrl Pts',(5.4613515310083,38.4994423268314,-15.8780708774594));
#53200=CARTESIAN_POINT('Ctrl Pts',(5.4672180666783,38.4321930371347,-15.8789732955971));
#53201=CARTESIAN_POINT('Ctrl Pts',(5.47239129984161,38.3648642685655,-15.8801468135981));
#53202=CARTESIAN_POINT('Ctrl Pts',(5.47689147490033,38.2974584401977,-15.8815868411561));
#53203=CARTESIAN_POINT('Ctrl Pts',(5.48611772124094,38.1592631990796,-15.8845391816348));
#53204=CARTESIAN_POINT('Ctrl Pts',(5.49251394881542,38.0207439405754,-15.8886116481605));
#53205=CARTESIAN_POINT('Ctrl Pts',(5.49620058929051,37.8819144998199,-15.893766360599));
#53206=CARTESIAN_POINT('Ctrl Pts',(5.49808097420446,37.8111040186317,-15.8963955411688));
#53207=CARTESIAN_POINT('Ctrl Pts',(5.49925641419002,37.7402128223893,-15.8993062934152));
#53208=CARTESIAN_POINT('Ctrl Pts',(5.49974268802741,37.6692427040055,-15.9024936677521));
#53209=CARTESIAN_POINT('Ctrl Pts',(5.49996561172688,37.6367076998042,-15.9039548635314));
#53210=CARTESIAN_POINT('Ctrl Pts',(5.50004339710141,37.6041560699435,-15.9054742042386));
#53211=CARTESIAN_POINT('Ctrl Pts',(5.49997719383551,37.5715879387439,-15.9070512284576));
#53212=CARTESIAN_POINT('Ctrl Pts',(5.49993631495294,37.5514779216182,-15.9080250019866));
#53213=CARTESIAN_POINT('Ctrl Pts',(5.4998405483016,37.531364539371,-15.9090206118804));
#53214=CARTESIAN_POINT('Ctrl Pts',(5.49969017010503,37.5112446362526,-15.9100381108086));
#53215=CARTESIAN_POINT('Ctrl Pts',(5.49945316022283,37.4795338166206,-15.9116417827945));
#53216=CARTESIAN_POINT('Ctrl Pts',(5.49908009391674,37.4477923382831,-15.9133006740155));
#53217=CARTESIAN_POINT('Ctrl Pts',(5.49857262658559,37.4160475576214,-15.9150128293562));
#53218=CARTESIAN_POINT('Ctrl Pts',(5.49823619185712,37.3950017759391,-15.9161479339861));
#53219=CARTESIAN_POINT('Ctrl Pts',(5.49784081050823,37.373963120172,-15.9173059703468));
#53220=CARTESIAN_POINT('Ctrl Pts',(5.49738703265501,37.3529405554518,-15.9184862796528));
#53221=CARTESIAN_POINT('Ctrl Pts',(5.49672206742468,37.3221341278296,-15.920215902736));
#53222=CARTESIAN_POINT('Ctrl Pts',(5.49593195327599,37.2913564447323,-15.92199354696));
#53223=CARTESIAN_POINT('Ctrl Pts',(5.4950180497321,37.2605988957863,-15.9238189832608));
#53224=CARTESIAN_POINT('Ctrl Pts',(5.49280147822436,37.1859998780916,-15.9282463761961));
#53225=CARTESIAN_POINT('Ctrl Pts',(5.48985732942819,37.1115441622757,-15.93295352956));
#53226=CARTESIAN_POINT('Ctrl Pts',(5.48620799883168,37.0372271498164,-15.9379304121376));
#53227=CARTESIAN_POINT('Ctrl Pts',(5.47973167176091,36.9053395975987,-15.9467626948023));
#53228=CARTESIAN_POINT('Ctrl Pts',(5.47103846329943,36.7738881771258,-15.9564438277391));
#53229=CARTESIAN_POINT('Ctrl Pts',(5.46021917404937,36.6428531857779,-15.9669233415353));
#53230=CARTESIAN_POINT('Ctrl Pts',(5.45380509725103,36.5651707726035,-15.9731359868158));
#53231=CARTESIAN_POINT('Ctrl Pts',(5.44664379103562,36.4876348301111,-15.9796292274412));
#53232=CARTESIAN_POINT('Ctrl Pts',(5.43875405388885,36.4102412795673,-15.9863926024135));
#53233=CARTESIAN_POINT('Ctrl Pts',(5.4258362108228,36.2835250504138,-15.9974662560553));
#53234=CARTESIAN_POINT('Ctrl Pts',(5.41096503287305,36.1571906423008,-16.0092641942867));
#53235=CARTESIAN_POINT('Ctrl Pts',(5.39418796878771,36.0312262694519,-16.0217459585996));
#53236=CARTESIAN_POINT('Ctrl Pts',(5.38340841350248,35.9502919704478,-16.0297657091224));
#53237=CARTESIAN_POINT('Ctrl Pts',(5.37184204285196,35.8695104675066,-16.0380677347448));
#53238=CARTESIAN_POINT('Ctrl Pts',(5.35950133781401,35.7888786668574,-16.0466413856611));
#53239=CARTESIAN_POINT('Ctrl Pts',(5.34090443967194,35.6673700999583,-16.0595614994072));
#53240=CARTESIAN_POINT('Ctrl Pts',(5.32054889691846,35.5462015292645,-16.0730985401622));
#53241=CARTESIAN_POINT('Ctrl Pts',(5.29844924191254,35.4253672803131,-16.0872199870259));
#53242=CARTESIAN_POINT('Ctrl Pts',(5.28302942198048,35.3410563550991,-16.0970730896087));
#53243=CARTESIAN_POINT('Ctrl Pts',(5.26676046322358,35.2569081691998,-16.1072106103974));
#53244=CARTESIAN_POINT('Ctrl Pts',(5.24964719740389,35.1729207936882,-16.1176215804705));
#53245=CARTESIAN_POINT('Ctrl Pts',(5.22595810725155,35.0566610142215,-16.132032997393));
#53246=CARTESIAN_POINT('Ctrl Pts',(5.20065131757863,34.9407093519288,-16.146968454176));
#53247=CARTESIAN_POINT('Ctrl Pts',(5.17371469820154,34.8250650313396,-16.1624016697516));
#53248=CARTESIAN_POINT('Ctrl Pts',(5.15327132250656,34.7372975108614,-16.1741146104059));
#53249=CARTESIAN_POINT('Ctrl Pts',(5.13188915865321,34.6497070193824,-16.186114219127));
#53250=CARTESIAN_POINT('Ctrl Pts',(5.10956274419647,34.5622931135843,-16.1983889759437));
#53251=CARTESIAN_POINT('Ctrl Pts',(5.08367992517983,34.4609549292693,-16.212618995268));
#53252=CARTESIAN_POINT('Ctrl Pts',(5.0565259540986,34.3598544368731,-16.2272190066503));
#53253=CARTESIAN_POINT('Ctrl Pts',(5.0280786240926,34.258993325232,-16.2421722431811));
#53254=CARTESIAN_POINT('Ctrl Pts',(5.02537462849238,34.2494062039783,-16.2435935887267));
#53255=CARTESIAN_POINT('Ctrl Pts',(5.02265894191753,34.2398212464829,-16.245018126109));
#53256=CARTESIAN_POINT('Ctrl Pts',(5.01993153885963,34.2302384553135,-16.246445841369));
#53257=CARTESIAN_POINT('Ctrl Pts',(5.00830961335107,34.18940456213,-16.2525295774528));
#53258=CARTESIAN_POINT('Ctrl Pts',(4.99647652389308,34.1486153304945,-16.2586702191085));
#53259=CARTESIAN_POINT('Ctrl Pts',(4.98442562639818,34.1078551593912,-16.2648690928362));
#53260=CARTESIAN_POINT('Ctrl Pts',(4.98191519828605,34.0993640507882,-16.2661604345703));
#53261=CARTESIAN_POINT('Ctrl Pts',(4.97939577749796,34.0908757952992,-16.2674540642285));
#53262=CARTESIAN_POINT('Ctrl Pts',(4.97686741013458,34.082390567841,-16.2687499417094));
#53263=CARTESIAN_POINT('Ctrl Pts',(4.96441142163706,34.0405881394636,-16.2751340752931));
#53264=CARTESIAN_POINT('Ctrl Pts',(4.95174642038967,33.9988861356218,-16.2815686233584));
#53265=CARTESIAN_POINT('Ctrl Pts',(4.93887533693539,33.9572960334576,-16.2880501468107));
#53266=CARTESIAN_POINT('Ctrl Pts',(4.9365923183524,33.9499189562716,-16.289199812147));
#53267=CARTESIAN_POINT('Ctrl Pts',(4.93430269704837,33.9425449476634,-16.2903510225307));
#53268=CARTESIAN_POINT('Ctrl Pts',(4.93200641902833,33.9351738636263,-16.2915037921635));
#53269=CARTESIAN_POINT('Ctrl Pts',(4.90152218935013,33.8373190669505,-16.3068073808168));
#53270=CARTESIAN_POINT('Ctrl Pts',(4.86988434782216,33.7400428634163,-16.3223755709518));
#53271=CARTESIAN_POINT('Ctrl Pts',(4.83707663711256,33.6433485724266,-16.3381886662497));
#53272=CARTESIAN_POINT('Ctrl Pts',(4.80536763875374,33.5498925205417,-16.3534721896045));
#53273=CARTESIAN_POINT('Ctrl Pts',(4.77256571792549,33.4569804742511,-16.3689838092686));
#53274=CARTESIAN_POINT('Ctrl Pts',(4.73865560426316,33.3646155432662,-16.3847048733899));
#53275=CARTESIAN_POINT('Ctrl Pts',(4.70239552922545,33.2658497484442,-16.4015154028498));
#53276=CARTESIAN_POINT('Ctrl Pts',(4.66486875936597,33.1677093269555,-16.4185655478469));
#53277=CARTESIAN_POINT('Ctrl Pts',(4.62603635930902,33.0702085181134,-16.4358333229825));
#53278=CARTESIAN_POINT('Ctrl Pts',(4.58826245515966,32.9753653922111,-16.4526304120599));
#53279=CARTESIAN_POINT('Ctrl Pts',(4.54925308469861,32.8811275612641,-16.4696332423119));
#53280=CARTESIAN_POINT('Ctrl Pts',(4.50897156414357,32.7875075156098,-16.4868216505679));
#53281=CARTESIAN_POINT('Ctrl Pts',(4.46911625428267,32.6948780448914,-16.5038281917218));
#53282=CARTESIAN_POINT('Ctrl Pts',(4.42801637606486,32.602852958373,-16.5210165527185));
#53283=CARTESIAN_POINT('Ctrl Pts',(4.38561383431928,32.5114558651078,-16.5383669400771));
#53284=CARTESIAN_POINT('Ctrl Pts',(4.34125546095837,32.415843049926,-16.5565176199356));
#53285=CARTESIAN_POINT('Ctrl Pts',(4.29547149890815,32.3209175705842,-16.5748455228508));
#53286=CARTESIAN_POINT('Ctrl Pts',(4.24819390138341,32.2267055569911,-16.5933281017443));
#53287=CARTESIAN_POINT('Ctrl Pts',(4.20460210136336,32.1398383837197,-16.6103697647129));
#53288=CARTESIAN_POINT('Ctrl Pts',(4.15974189040682,32.0535770633788,-16.6275431186279));
#53289=CARTESIAN_POINT('Ctrl Pts',(4.11353180757193,31.9679563275417,-16.6448290878375));
#53290=CARTESIAN_POINT('Ctrl Pts',(4.06536813475078,31.8787158662706,-16.6628458433664));
#53291=CARTESIAN_POINT('Ctrl Pts',(4.01573942477214,31.7901709205017,-16.6809872025155));
#53292=CARTESIAN_POINT('Ctrl Pts',(3.96454901579434,31.7023606031743,-16.6992276878768));
#53293=CARTESIAN_POINT('Ctrl Pts',(3.96088789420439,31.6960804375142,-16.7005322415247));
#53294=CARTESIAN_POINT('Ctrl Pts',(3.95721878771191,31.6898040285205,-16.7018373092452));
#53295=CARTESIAN_POINT('Ctrl Pts',(3.95354166156699,31.6835313901512,-16.7031428835095));
#53296=CARTESIAN_POINT('Ctrl Pts',(3.90580460039334,31.6020989590209,-16.720092065034));
#53297=CARTESIAN_POINT('Ctrl Pts',(3.85671222537039,31.5213038976113,-16.7371264023128));
#53298=CARTESIAN_POINT('Ctrl Pts',(3.80616156422669,31.4411903127911,-16.7542275028122));
#53299=CARTESIAN_POINT('Ctrl Pts',(3.80152842925821,31.4338476382764,-16.755794875126));
#53300=CARTESIAN_POINT('Ctrl Pts',(3.79688303941635,31.4265106877601,-16.7573628044737));
#53301=CARTESIAN_POINT('Ctrl Pts',(3.79222531430233,31.4191794949343,-16.7589312766305));
#53302=CARTESIAN_POINT('Ctrl Pts',(3.76951630087782,31.3834358320465,-16.7665784551122));
#53303=CARTESIAN_POINT('Ctrl Pts',(3.74651379434752,31.3478291722543,-16.7742385163404));
#53304=CARTESIAN_POINT('Ctrl Pts',(3.72320690339818,31.3123642118345,-16.7819096840143));
#53305=CARTESIAN_POINT('Ctrl Pts',(3.71807526776141,31.304555651905,-16.7835986968259));
#53306=CARTESIAN_POINT('Ctrl Pts',(3.71292915379114,31.2967543834909,-16.7852881565976));
#53307=CARTESIAN_POINT('Ctrl Pts',(3.70776825174835,31.2889601585938,-16.7869781081522));
#53308=CARTESIAN_POINT('Ctrl Pts',(3.69880543936009,31.2754241187919,-16.789913005696));
#53309=CARTESIAN_POINT('Ctrl Pts',(3.68979574239286,31.261906155841,-16.7928500917675));
#53310=CARTESIAN_POINT('Ctrl Pts',(3.68074182945706,31.2484112412283,-16.7957882205531));
#53311=CARTESIAN_POINT('Ctrl Pts',(3.66647455761765,31.2271457821284,-16.8004181614838));
#53312=CARTESIAN_POINT('Ctrl Pts',(3.65209323029816,31.2059313524667,-16.8050520521899));
#53313=CARTESIAN_POINT('Ctrl Pts',(3.63762484959751,31.1848118870779,-16.8096800639383));
#53314=CARTESIAN_POINT('Ctrl Pts',(3.63200035761215,31.1766018277581,-16.8114791743934));
#53315=CARTESIAN_POINT('Ctrl Pts',(3.62636141820263,31.1684042483615,-16.8132777791051));
#53316=CARTESIAN_POINT('Ctrl Pts',(3.62070890280921,31.1602206821355,-16.8150755350487));
#53317=CARTESIAN_POINT('Ctrl Pts',(3.5681995469857,31.0841989889676,-16.8317758887778));
#53318=CARTESIAN_POINT('Ctrl Pts',(3.51445248319197,31.0092691764222,-16.8484279478469));
#53319=CARTESIAN_POINT('Ctrl Pts',(3.45940003185614,30.9355222948858,-16.8650025248823));
#53320=CARTESIAN_POINT('Ctrl Pts',(3.39842130654987,30.8538367255372,-16.8833613182801));
#53321=CARTESIAN_POINT('Ctrl Pts',(3.33583572143396,30.7735927411555,-16.9016283924899));
#53322=CARTESIAN_POINT('Ctrl Pts',(3.2715207048759,30.6948919828411,-16.919757436288));
#53323=CARTESIAN_POINT('Ctrl Pts',(3.26416317733215,30.6858887511232,-16.921831367793));
#53324=CARTESIAN_POINT('Ctrl Pts',(3.25678303217922,30.6769057057008,-16.923903524439));
#53325=CARTESIAN_POINT('Ctrl Pts',(3.24938008678968,30.667942991644,-16.9259738497194));
#53326=CARTESIAN_POINT('Ctrl Pts',(3.19207100052512,30.5985591280577,-16.9420010448216));
#53327=CARTESIAN_POINT('Ctrl Pts',(3.13339174267546,30.5303974813926,-16.9579178841127));
#53328=CARTESIAN_POINT('Ctrl Pts',(3.07322940139954,30.4635532861489,-16.9736929964154));
#53329=CARTESIAN_POINT('Ctrl Pts',(3.06515238212777,30.4545792029975,-16.9758108642274));
#53330=CARTESIAN_POINT('Ctrl Pts',(3.05704861784992,30.4456288810808,-16.9779261567944));
#53331=CARTESIAN_POINT('Ctrl Pts',(3.0489178282833,30.4367025507343,-16.9800387987298));
#53332=CARTESIAN_POINT('Ctrl Pts',(2.98866251080745,30.3705516727029,-16.9956950778016));
#53333=CARTESIAN_POINT('Ctrl Pts',(2.92692378235327,30.3057176256009,-17.0112059694983));
#53334=CARTESIAN_POINT('Ctrl Pts',(2.86356125520061,30.242320131431,-17.026535619822));
#53335=CARTESIAN_POINT('Ctrl Pts',(2.85491055641671,30.2336646587035,-17.028628531727));
#53336=CARTESIAN_POINT('Ctrl Pts',(2.84622956753871,30.2250359814179,-17.0307180375992));
#53337=CARTESIAN_POINT('Ctrl Pts',(2.83751792073732,30.2164344038661,-17.0328040472932));
#53338=CARTESIAN_POINT('Ctrl Pts',(2.77381031096406,30.1535317221342,-17.0480588773613));
#53339=CARTESIAN_POINT('Ctrl Pts',(2.70846431693196,30.0920771826219,-17.0631269955375));
#53340=CARTESIAN_POINT('Ctrl Pts',(2.64130079839515,30.0322245558024,-17.0779660058408));
#53341=CARTESIAN_POINT('Ctrl Pts',(2.63227265442548,30.0241791444889,-17.0799606708658));
#53342=CARTESIAN_POINT('Ctrl Pts',(2.62321161946429,30.0161626708754,-17.0819511802079));
#53343=CARTESIAN_POINT('Ctrl Pts',(2.61411725538389,30.0081755240293,-17.0839374247674));
#53344=CARTESIAN_POINT('Ctrl Pts',(2.57585134947034,29.9745684013068,-17.0922948477565));
#53345=CARTESIAN_POINT('Ctrl Pts',(2.53699459987065,29.9414812576612,-17.1005766119967));
#53346=CARTESIAN_POINT('Ctrl Pts',(2.49750822445488,29.9089491590999,-17.1087733255147));
#53347=CARTESIAN_POINT('Ctrl Pts',(2.47779485825612,29.8927076792123,-17.1128654918254));
#53348=CARTESIAN_POINT('Ctrl Pts',(2.45792448501533,29.8766046168504,-17.1169364445262));
#53349=CARTESIAN_POINT('Ctrl Pts',(2.43789178185496,29.8606448267007,-17.1209849104469));
#53350=CARTESIAN_POINT('Ctrl Pts',(2.42694070914223,29.8519202516391,-17.1231980438576));
#53351=CARTESIAN_POINT('Ctrl Pts',(2.41593835595827,29.8432363635108,-17.1254050014128));
#53352=CARTESIAN_POINT('Ctrl Pts',(2.40488856363168,29.8345976778537,-17.1276046266254));
#53353=CARTESIAN_POINT('Ctrl Pts',(2.39574786529823,29.8274515146267,-17.1294242183354));
#53354=CARTESIAN_POINT('Ctrl Pts',(2.38657107919022,29.8203334707193,-17.131239509796));
#53355=CARTESIAN_POINT('Ctrl Pts',(2.37736544561913,29.8132500786786,-17.1330488320748));
#53356=CARTESIAN_POINT('Ctrl Pts',(2.37632716664283,29.8124511616915,-17.1332529007323));
#53357=CARTESIAN_POINT('Ctrl Pts',(2.37528863153933,29.8116527691013,-17.1334568720052));
#53358=CARTESIAN_POINT('Ctrl Pts',(2.3742498473769,29.8108549069625,-17.133660744308));
#53359=CARTESIAN_POINT('Ctrl Pts',(2.36400095054056,29.8029830053244,-17.1356721979616));
#53360=CARTESIAN_POINT('Ctrl Pts',(2.35372330622806,29.7951592975047,-17.1376748836086));
#53361=CARTESIAN_POINT('Ctrl Pts',(2.34341659203281,29.7873843072001,-17.1396686375351));
#53362=CARTESIAN_POINT('Ctrl Pts',(2.32280316364232,29.7718343265909,-17.1436561453881));
#53363=CARTESIAN_POINT('Ctrl Pts',(2.30207345556508,29.7564792140062,-17.1476079243563));
#53364=CARTESIAN_POINT('Ctrl Pts',(2.28122498144331,29.7413230169235,-17.1515229111162));
#53365=CARTESIAN_POINT('Ctrl Pts',(2.23952803319974,29.7110106227581,-17.1593528846361));
#53366=CARTESIAN_POINT('Ctrl Pts',(2.19735604974939,29.6814938543918,-17.1670356542043));
#53367=CARTESIAN_POINT('Ctrl Pts',(2.15468743215846,29.6528077790857,-17.1745600211926));
#53368=CARTESIAN_POINT('Ctrl Pts',(2.14610634444727,29.6470387211178,-17.1760732469952));
#53369=CARTESIAN_POINT('Ctrl Pts',(2.13750517566442,29.6413032676407,-17.1775800661172));
#53370=CARTESIAN_POINT('Ctrl Pts',(2.12888374364691,29.6356017004686,-17.1790803938992));
#53371=CARTESIAN_POINT('Ctrl Pts',(2.05176672426468,29.5846022997628,-17.1925005318074));
#53372=CARTESIAN_POINT('Ctrl Pts',(1.97302948507885,29.536311980985,-17.2054018294005));
#53373=CARTESIAN_POINT('Ctrl Pts',(1.892517709225,29.4909836117988,-17.2177138548144));
#53374=CARTESIAN_POINT('Ctrl Pts',(1.88526198991242,29.4868986202528,-17.2188234142499));
#53375=CARTESIAN_POINT('Ctrl Pts',(1.87799185081891,29.4828377056425,-17.2199281748248));
#53376=CARTESIAN_POINT('Ctrl Pts',(1.87070717006779,29.4788010572599,-17.2210280840153));
#53377=CARTESIAN_POINT('Ctrl Pts',(1.78812182725007,29.4330381745882,-17.2334975910074));
#53378=CARTESIAN_POINT('Ctrl Pts',(1.70366911987935,29.3903907672498,-17.2453443608244));
#53379=CARTESIAN_POINT('Ctrl Pts',(1.61713745716078,29.3512072939032,-17.2564775264755));
#53380=CARTESIAN_POINT('Ctrl Pts',(1.61212632952938,29.3489381431691,-17.2571222582681));
#53381=CARTESIAN_POINT('Ctrl Pts',(1.60710821712393,29.3466806272549,-17.2577645818538));
#53382=CARTESIAN_POINT('Ctrl Pts',(1.60208307676273,29.3444348146711,-17.2584044808196));
#53383=CARTESIAN_POINT('Ctrl Pts',(1.55989433998816,29.3255800187584,-17.2637767743458));
#53384=CARTESIAN_POINT('Ctrl Pts',(1.51721051394536,29.3075495812703,-17.2689782885513));
#53385=CARTESIAN_POINT('Ctrl Pts',(1.47400118885662,29.2903942144724,-17.2739973129508));
#53386=CARTESIAN_POINT('Ctrl Pts',(1.46191218168413,29.2855945247794,-17.2754015242371));
#53387=CARTESIAN_POINT('Ctrl Pts',(1.4497820516811,29.2808633184437,-17.2767914781327));
#53388=CARTESIAN_POINT('Ctrl Pts',(1.43761008083042,29.2762017723702,-17.2781668632123));
#53389=CARTESIAN_POINT('Ctrl Pts',(1.42543810997977,29.2715402262967,-17.2795422482919));
#53390=CARTESIAN_POINT('Ctrl Pts',(1.41321940491667,29.2669465835128,-17.280903591134));
#53391=CARTESIAN_POINT('Ctrl Pts',(1.40097815995123,29.2624310609538,-17.2822478952774));
#53392=CARTESIAN_POINT('Ctrl Pts',(1.37649567002035,29.2534000158358,-17.2849365035642));
#53393=CARTESIAN_POINT('Ctrl Pts',(1.35191025614907,29.2446764670801,-17.2875582881031));
#53394=CARTESIAN_POINT('Ctrl Pts',(1.32722006320831,29.2362657864039,-17.2901114789568));
#53395=CARTESIAN_POINT('Ctrl Pts',(1.32550120392183,29.2356802593236,-17.2902892246641));
#53396=CARTESIAN_POINT('Ctrl Pts',(1.32378183755517,29.2350962472779,-17.29046663934));
#53397=CARTESIAN_POINT('Ctrl Pts',(1.3220619635894,29.2345137519665,-17.2906437224965));
#53398=CARTESIAN_POINT('Ctrl Pts',(1.27437230137859,29.2183619843406,-17.2955539869008));
#53399=CARTESIAN_POINT('Ctrl Pts',(1.22629149643725,29.2033782518924,-17.3002089905994));
#53400=CARTESIAN_POINT('Ctrl Pts',(1.17780400163588,29.1896084456524,-17.3045965622765));
#53401=CARTESIAN_POINT('Ctrl Pts',(1.17767327582233,29.189571321253,-17.3046083914889));
#53402=CARTESIAN_POINT('Ctrl Pts',(1.17754254712066,29.189534205695,-17.3046202187513));
#53403=CARTESIAN_POINT('Ctrl Pts',(1.17741181552952,29.1894970989791,-17.3046320440637));
#53404=CARTESIAN_POINT('Ctrl Pts',(1.15299541258929,29.1825667731042,-17.3068406272224));
#53405=CARTESIAN_POINT('Ctrl Pts',(1.12847817746668,29.1759449661951,-17.3089811700638));
#53406=CARTESIAN_POINT('Ctrl Pts',(1.10385096834405,29.1696362782663,-17.311052643283));
#53407=CARTESIAN_POINT('Ctrl Pts',(1.10327398297119,29.1694884734282,-17.3111011753656));
#53408=CARTESIAN_POINT('Ctrl Pts',(1.10269696617672,29.1693408482817,-17.3111496670085));
#53409=CARTESIAN_POINT('Ctrl Pts',(1.10211991879364,29.1691934030318,-17.3111981181411));
#53410=CARTESIAN_POINT('Ctrl Pts',(1.0780259363015,29.1630369878481,-17.3132211422025));
#53411=CARTESIAN_POINT('Ctrl Pts',(1.05386293703712,29.1571899569309,-17.3151748891896));
#53412=CARTESIAN_POINT('Ctrl Pts',(1.02966713626784,29.1516639253954,-17.3170555760385));
#53413=CARTESIAN_POINT('Ctrl Pts',(1.02841708067243,29.1513784276469,-17.3171527401349));
#53414=CARTESIAN_POINT('Ctrl Pts',(1.02716688202533,29.1510937723588,-17.317249713827));
#53415=CARTESIAN_POINT('Ctrl Pts',(1.0259165361847,29.1508099590767,-17.3173464973055));
#53416=CARTESIAN_POINT('Ctrl Pts',(0.928167679757507,29.1286221588217,-17.3249127833967));
#53417=CARTESIAN_POINT('Ctrl Pts',(0.829681073359833,29.1116166132758,-17.3313043848515));
#53418=CARTESIAN_POINT('Ctrl Pts',(0.730430567978592,29.099973605139,-17.3364718005591));
#53419=CARTESIAN_POINT('',(0.346147593750904,43.9243235319994,-16.6433959640037));
#53420=CARTESIAN_POINT('Origin',(0.600919835348839,39.755200147935,-15.5793615221956));
#53421=CARTESIAN_POINT('Origin',(0.330762353100779,44.2777095070772,-16.996781938525));
#53422=CARTESIAN_POINT('Origin',(9.,24.,-29.5));
#53423=CARTESIAN_POINT('',(9.,26.1794494717703,-23.3762756430421));
#53424=CARTESIAN_POINT('',(8.9999999999999,26.1794494717706,-35.6237243569579));
#53425=CARTESIAN_POINT('Origin',(9.,24.,-29.5));
#53426=CARTESIAN_POINT('',(9.5,26.0117995124034,-23.847331362808));
#53427=CARTESIAN_POINT('Origin',(9.,26.0117995124034,-23.847331362808));
#53428=CARTESIAN_POINT('',(9.5,26.0117995124036,-35.1526686371918));
#53429=CARTESIAN_POINT('Origin',(9.5,24.,-29.5));
#53430=CARTESIAN_POINT('Origin',(9.,26.0117995124036,-35.1526686371918));
#53431=CARTESIAN_POINT('Origin',(-42.5,41.0197988065678,-24.9401265742657));
#53432=CARTESIAN_POINT('',(-44.9819347291981,45.7897031282913,-29.7473377789847));
#53433=CARTESIAN_POINT('',(-44.9819347291981,47.3983418014005,-27.2150894461039));
#53434=CARTESIAN_POINT('Origin',(-42.5,46.5940224648459,-28.4812136125442));
#53435=CARTESIAN_POINT('',(-45.2221315177632,45.635768184996,-29.057189944653));
#53436=CARTESIAN_POINT('Ctrl Pts',(-44.9819347291982,45.7897031282913,-29.7473377789846));
#53437=CARTESIAN_POINT('Ctrl Pts',(-45.0186376354568,45.8222670575131,-29.6960770721134));
#53438=CARTESIAN_POINT('Ctrl Pts',(-45.0556916549072,45.8482062072712,-29.6333175979576));
#53439=CARTESIAN_POINT('Ctrl Pts',(-45.1195835420918,45.8719268666396,-29.4987828001409));
#53440=CARTESIAN_POINT('Ctrl Pts',(-45.1465267698371,45.8695622104315,-29.4270318030083));
#53441=CARTESIAN_POINT('Ctrl Pts',(-45.1843416183679,45.8393623668559,-29.3030188626678));
#53442=CARTESIAN_POINT('Ctrl Pts',(-45.1988644063568,45.8129304583389,-29.2426178063836));
#53443=CARTESIAN_POINT('Ctrl Pts',(-45.2176939546586,45.7373723936762,-29.1363548938651));
#53444=CARTESIAN_POINT('Ctrl Pts',(-45.2221315177632,45.6882381055569,-29.0905220402035));
#53445=CARTESIAN_POINT('Ctrl Pts',(-45.2221315177632,45.635768184996,-29.0571899446529));
#53446=CARTESIAN_POINT('',(-45.2221315177632,43.1035198521152,-27.4485512715437));
#53447=CARTESIAN_POINT('',(-45.2221315177632,40.4835859155314,-25.7842093518926));
#53448=CARTESIAN_POINT('',(-44.9819347291981,42.4133720177836,-27.602486214839));
#53449=CARTESIAN_POINT('Ctrl Pts',(-45.2221315177632,43.1035198521152,-27.4485512715437));
#53450=CARTESIAN_POINT('Ctrl Pts',(-45.2221315177632,43.0496138985403,-27.4143069201879));
#53451=CARTESIAN_POINT('Ctrl Pts',(-45.2174539674018,42.9854710022637,-27.3889839513675));
#53452=CARTESIAN_POINT('Ctrl Pts',(-45.1976418506297,42.8537496937191,-27.3664815814561));
#53453=CARTESIAN_POINT('Ctrl Pts',(-45.182361508012,42.7861963762066,-27.3692838789625));
#53454=CARTESIAN_POINT('Ctrl Pts',(-45.1436039433344,42.6618963628359,-27.3970085410682));
#53455=CARTESIAN_POINT('Ctrl Pts',(-45.1169018514096,42.5979765578451,-27.4255404391954));
#53456=CARTESIAN_POINT('Ctrl Pts',(-45.0540257957218,42.4896281746961,-27.5033321310102));
#53457=CARTESIAN_POINT('Ctrl Pts',(-45.0177578429344,42.4451553684532,-27.5524542604343));
#53458=CARTESIAN_POINT('Ctrl Pts',(-44.9819347291981,42.4133720177835,-27.602486214839));
#53459=CARTESIAN_POINT('',(-44.9819347291981,44.0220106908928,-25.0702378819582));
#53460=CARTESIAN_POINT('Origin',(-42.5,43.2176913543382,-26.3363620483986));
#53461=CARTESIAN_POINT('',(-45.2221315177632,44.1759456341881,-25.7603857162899));
#53462=CARTESIAN_POINT('Ctrl Pts',(-44.9819347291982,44.0220106908928,-25.0702378819583));
#53463=CARTESIAN_POINT('Ctrl Pts',(-45.0186376354568,43.989446761671,-25.1214985888295));
#53464=CARTESIAN_POINT('Ctrl Pts',(-45.0556916549072,43.963507611913,-25.1842580629853));
#53465=CARTESIAN_POINT('Ctrl Pts',(-45.1195835420918,43.9397869525445,-25.318792860802));
#53466=CARTESIAN_POINT('Ctrl Pts',(-45.1465267698372,43.9421516087526,-25.3905438579346));
#53467=CARTESIAN_POINT('Ctrl Pts',(-45.1843416183679,43.9723514523282,-25.5145567982751));
#53468=CARTESIAN_POINT('Ctrl Pts',(-45.1988644063568,43.9987833608452,-25.5749578545593));
#53469=CARTESIAN_POINT('Ctrl Pts',(-45.2176939546586,44.0743414255079,-25.6812207670778));
#53470=CARTESIAN_POINT('Ctrl Pts',(-45.2221315177633,44.1234757136272,-25.7270536207394));
#53471=CARTESIAN_POINT('Ctrl Pts',(-45.2221315177633,44.1759456341881,-25.76038571629));
#53472=CARTESIAN_POINT('',(-45.2221315177632,46.7081939670689,-27.3690243893992));
#53473=CARTESIAN_POINT('',(-45.2221315177632,41.5560116976042,-24.0960437966388));
#53474=CARTESIAN_POINT('Ctrl Pts',(-45.2221315177632,46.7081939670689,-27.3690243893992));
#53475=CARTESIAN_POINT('Ctrl Pts',(-45.2221315177632,46.7606638876298,-27.4023564849497));
#53476=CARTESIAN_POINT('Ctrl Pts',(-45.2176939546586,46.8230322141941,-27.427356896653));
#53477=CARTESIAN_POINT('Ctrl Pts',(-45.1988644063568,46.9513316276602,-27.4505966947741));
#53478=CARTESIAN_POINT('Ctrl Pts',(-45.1843416183679,47.0172399166597,-27.4488557670715));
#53479=CARTESIAN_POINT('Ctrl Pts',(-45.1465267698371,47.1423318988987,-27.4234936712708));
#53480=CARTESIAN_POINT('Ctrl Pts',(-45.1195835420918,47.208286923191,-27.3951435044439));
#53481=CARTESIAN_POINT('Ctrl Pts',(-45.0556916549071,47.3199898635242,-27.3165004206706));
#53482=CARTESIAN_POINT('Ctrl Pts',(-45.0186376354568,47.3657778721787,-27.2663501529751));
#53483=CARTESIAN_POINT('Ctrl Pts',(-44.9819347291982,47.3983418014006,-27.2150894461039));
#53484=CARTESIAN_POINT('Origin',(-50.,46.9763004125871,-26.9469830005857));
#53485=CARTESIAN_POINT('',(-50.,46.7081939670689,-27.3690243893992));
#53486=CARTESIAN_POINT('',(-45.2221315177632,46.7081939670689,-27.3690243893992));
#53487=CARTESIAN_POINT('',(-49.5,47.3983418014005,-27.2150894461039));
#53488=CARTESIAN_POINT('Origin',(-49.5000000000004,46.9763004125864,-26.9469830005858));
#53489=CARTESIAN_POINT('',(-50.,47.3983418014005,-27.2150894461039));
#53490=CARTESIAN_POINT('Origin',(0.,12.,0.));
#53491=CARTESIAN_POINT('',(2.38806125833734E-15,12.,19.5));
#53492=CARTESIAN_POINT('Origin',(6.61325378140121E-15,20.5440037453176,
8.67361737988404E-16));
#53493=CARTESIAN_POINT('Ctrl Pts',(-12.9440892692056,20.5440037453176,10.2323288156136));
#53494=CARTESIAN_POINT('Ctrl Pts',(-12.9496367646674,20.4508539796772,10.2253111290467));
#53495=CARTESIAN_POINT('Ctrl Pts',(-12.9610165600406,20.3590140095801,10.2178819495937));
#53496=CARTESIAN_POINT('Ctrl Pts',(-12.9946219649296,20.1777741261809,10.2022098463961));
#53497=CARTESIAN_POINT('Ctrl Pts',(-13.0168498220794,20.0883747060241,10.1939668938316));
#53498=CARTESIAN_POINT('Ctrl Pts',(-13.0579271737774,19.9560174404499,10.1810048619498));
#53499=CARTESIAN_POINT('Ctrl Pts',(-13.0729108743488,19.912189091234,10.1765846465299));
#53500=CARTESIAN_POINT('Ctrl Pts',(-13.093226641434,19.857760815908,10.1709368410215));
#53501=CARTESIAN_POINT('Ctrl Pts',(-13.0973704642225,19.846889820709,10.1698008100038));
#53502=CARTESIAN_POINT('Ctrl Pts',(-13.1057990120293,19.8252268576759,10.1675211517166));
#53503=CARTESIAN_POINT('Ctrl Pts',(-13.1186586370485,19.7928359778532,10.1640887306089));
#53504=CARTESIAN_POINT('Ctrl Pts',(-13.1681680547971,19.6751954927419,10.1513630815639));
#53505=CARTESIAN_POINT('Ctrl Pts',(-13.2201296869753,19.5715707888266,10.1393814591848));
#53506=CARTESIAN_POINT('Ctrl Pts',(-13.2658111744658,19.4906334205523,10.1295681579593));
#53507=CARTESIAN_POINT('',(12.2613197119475,20.1060921583966,11.0892507440724));
#53508=CARTESIAN_POINT('Ctrl Pts',(12.3247145835032,19.4906334206159,11.2557233274532));
#53509=CARTESIAN_POINT('Ctrl Pts',(12.3240848130916,19.4937421807176,11.2546841768212));
#53510=CARTESIAN_POINT('Ctrl Pts',(12.3234588554608,19.49685286589,11.2536485098443));
#53511=CARTESIAN_POINT('Ctrl Pts',(12.3228366936365,19.4999654675381,11.252616310886));
#53512=CARTESIAN_POINT('Ctrl Pts',(12.3222145318121,19.5030780691863,11.2515841119277));
#53513=CARTESIAN_POINT('Ctrl Pts',(12.3215948199724,19.5062100227993,11.2505473287028));
#53514=CARTESIAN_POINT('Ctrl Pts',(12.320980850292,19.5093388049001,11.2495147887444));
#53515=CARTESIAN_POINT('Ctrl Pts',(12.3197529109312,19.5155963691016,11.2474497088275));
#53516=CARTESIAN_POINT('Ctrl Pts',(12.3185447508262,19.5218607187377,11.2453943141538));
#53517=CARTESIAN_POINT('Ctrl Pts',(12.3173562624689,19.5281318609459,11.2433486881666));
#53518=CARTESIAN_POINT('Ctrl Pts',(12.3168434298913,19.5308378580248,11.2424660008089));
#53519=CARTESIAN_POINT('Ctrl Pts',(12.3163342607863,19.5335451203528,11.2415851313079));
#53520=CARTESIAN_POINT('Ctrl Pts',(12.3158287470122,19.5362536487047,11.240706086076));
#53521=CARTESIAN_POINT('Ctrl Pts',(12.3139912066935,19.5460991372083,11.2375107605708));
#53522=CARTESIAN_POINT('Ctrl Pts',(12.3122019380873,19.5559613346833,11.2343395764923));
#53523=CARTESIAN_POINT('Ctrl Pts',(12.3104605724095,19.5658402918111,11.2311928321139));
#53524=CARTESIAN_POINT('Ctrl Pts',(12.3060197294663,19.5910336774419,11.2231679825694));
#53525=CARTESIAN_POINT('Ctrl Pts',(12.3018924452675,19.6163256808546,11.2153056087511));
#53526=CARTESIAN_POINT('Ctrl Pts',(12.2980766065538,19.6416802262003,11.2076214964828));
#53527=CARTESIAN_POINT('Ctrl Pts',(12.2904449291265,19.6923893168918,11.1922532719461));
#53528=CARTESIAN_POINT('Ctrl Pts',(12.284050670942,19.7433903721453,11.1775842317797));
#53529=CARTESIAN_POINT('Ctrl Pts',(12.2788349799084,19.7946878523301,11.1636514510574));
#53530=CARTESIAN_POINT('Ctrl Pts',(12.2717832670323,19.864043015281,11.144814068132));
#53531=CARTESIAN_POINT('Ctrl Pts',(12.2668823557172,19.933938143891,11.1273231458003));
#53532=CARTESIAN_POINT('Ctrl Pts',(12.2640266900014,20.0043963659391,11.1112869549714));
#53533=CARTESIAN_POINT('Ctrl Pts',(12.2626580572155,20.0381648256718,11.1036013017073));
#53534=CARTESIAN_POINT('Ctrl Pts',(12.26175954294,20.0720626786387,11.0962505061429));
#53535=CARTESIAN_POINT('Ctrl Pts',(12.2613198608839,20.1060920634664,11.0892508104087));
#53536=CARTESIAN_POINT('Ctrl Pts',(12.2613195356308,20.1060921539105,11.0892505197455));
#53537=CARTESIAN_POINT('Ctrl Pts',(12.2392211623119,20.1414234900087,11.1059128816441));
#53538=CARTESIAN_POINT('Ctrl Pts',(12.2176741954609,20.1770688828304,11.122757035389));
#53539=CARTESIAN_POINT('Ctrl Pts',(12.1967039557601,20.2130404789298,11.1397962358671));
#53540=CARTESIAN_POINT('Ctrl Pts',(12.1862188142041,20.2310263142123,11.1483158537427));
#53541=CARTESIAN_POINT('Ctrl Pts',(12.1758744707651,20.249099975504,11.1568872553953));
#53542=CARTESIAN_POINT('Ctrl Pts',(12.1656907253532,20.267233703068,11.1654983955483));
#53543=CARTESIAN_POINT('Ctrl Pts',(12.1555069799413,20.2853674306321,11.1741095357013));
#53544=CARTESIAN_POINT('Ctrl Pts',(12.1454820134063,20.30356413516,11.1827617704007));
#53545=CARTESIAN_POINT('Ctrl Pts',(12.1356187555891,20.3218245820165,11.1914566941426));
#53546=CARTESIAN_POINT('Ctrl Pts',(12.125569551754,20.3404292820032,11.2003155380087));
#53547=CARTESIAN_POINT('Ctrl Pts',(12.1156883444925,20.3591001188471,11.2092185790426));
#53548=CARTESIAN_POINT('Ctrl Pts',(12.1059782546267,20.3778380797799,11.2181678242057));
#53549=CARTESIAN_POINT('Ctrl Pts',(12.0966275071673,20.395882602849,11.2267858836294));
#53550=CARTESIAN_POINT('Ctrl Pts',(12.0874354743147,20.4139893872255,11.2354467144436));
#53551=CARTESIAN_POINT('Ctrl Pts',(12.0784054764407,20.432159179516,11.2441518495297));
#53552=CARTESIAN_POINT('Ctrl Pts',(12.0692019704499,20.4506780977408,11.2530242506126));
#53553=CARTESIAN_POINT('Ctrl Pts',(12.0601666863676,20.4692625077711,11.261942764992));
#53554=CARTESIAN_POINT('Ctrl Pts',(12.0513032693893,20.4879134104374,11.2709092728905));
#53555=CARTESIAN_POINT('Ctrl Pts',(12.0468715609001,20.4972388617706,11.2753925268398));
#53556=CARTESIAN_POINT('Ctrl Pts',(12.0424826470527,20.5065813207882,11.2798879696857));
#53557=CARTESIAN_POINT('Ctrl Pts',(12.0381381742578,20.5159383696529,11.2843946238478));
#53558=CARTESIAN_POINT('Ctrl Pts',(12.0359659378604,20.5206168940852,11.2866479509288));
#53559=CARTESIAN_POINT('Ctrl Pts',(12.0338048104555,20.5252990659819,11.2889040796134));
#53560=CARTESIAN_POINT('Ctrl Pts',(12.03165476243,20.5299850803084,11.2911631287932));
#53561=CARTESIAN_POINT('Ctrl Pts',(12.0305797384172,20.5323280874717,11.2922926533832));
#53562=CARTESIAN_POINT('Ctrl Pts',(12.0295073044338,20.5346731862636,11.2934231138684));
#53563=CARTESIAN_POINT('Ctrl Pts',(12.0284443643625,20.5370058241997,11.2945471759878));
#53564=CARTESIAN_POINT('Ctrl Pts',(12.0273814242911,20.5393384621358,11.2956712381073));
#53565=CARTESIAN_POINT('Ctrl Pts',(12.0263202972797,20.5416711025003,11.2967970058409));
#53566=CARTESIAN_POINT('Ctrl Pts',(12.0252610013046,20.5440037453176,11.2979244960981));
#53567=CARTESIAN_POINT('Origin',(-27.5,24.,-29.5));
#53568=CARTESIAN_POINT('',(-0.479749284976033,24.449552064594,-35.9844354373545));
#53569=CARTESIAN_POINT('',(-4.5,19.4038059222875,-34.0961940777126));
#53570=CARTESIAN_POINT('Ctrl Pts',(-0.479749284976206,24.4495520645939,
-35.9844354373545));
#53571=CARTESIAN_POINT('Ctrl Pts',(-0.487787721497241,24.4471112388692,
-35.9846046545909));
#53572=CARTESIAN_POINT('Ctrl Pts',(-0.495820774766061,24.4446422966896,
-35.9847744365369));
#53573=CARTESIAN_POINT('Ctrl Pts',(-0.83210386168481,24.3400450302139,-35.9919059041802));
#53574=CARTESIAN_POINT('Ctrl Pts',(-1.15106142213831,24.1908654782632,-35.9997450345785));
#53575=CARTESIAN_POINT('Ctrl Pts',(-2.0591668517866,23.6449502530038,-36.0004916773265));
#53576=CARTESIAN_POINT('Ctrl Pts',(-2.6011888924699,23.1493978597753,-35.964858749013));
#53577=CARTESIAN_POINT('Ctrl Pts',(-3.4592693304692,22.1493428393408,-35.7514047764218));
#53578=CARTESIAN_POINT('Ctrl Pts',(-3.84102577827634,21.5700258352893,-35.5628511467763));
#53579=CARTESIAN_POINT('Ctrl Pts',(-4.36201868849172,20.429896659423,-34.9696711241991));
#53580=CARTESIAN_POINT('Ctrl Pts',(-4.5,19.8699310744596,-34.5623192298848));
#53581=CARTESIAN_POINT('Ctrl Pts',(-4.5,19.4038059222874,-34.0961940777125));
#53582=CARTESIAN_POINT('',(5.47974928497604,19.0969304167095,-33.767306956549));
#53583=CARTESIAN_POINT('Ctrl Pts',(-4.5,19.4038059222874,-34.0961940777125));
#53584=CARTESIAN_POINT('Ctrl Pts',(-4.50000000000002,18.9376807701152,-33.6300689255403));
#53585=CARTESIAN_POINT('Ctrl Pts',(-4.36201868849172,18.5303288758009,-33.0701033405769));
#53586=CARTESIAN_POINT('Ctrl Pts',(-3.84102577827634,17.9371488532237,-31.9299741647106));
#53587=CARTESIAN_POINT('Ctrl Pts',(-3.4592693304692,17.7485952235782,-31.3506571606591));
#53588=CARTESIAN_POINT('Ctrl Pts',(-2.6011888924699,17.535141250987,-30.3506021402247));
#53589=CARTESIAN_POINT('Ctrl Pts',(-2.0591668517866,17.4995083226735,-29.8550497469961));
#53590=CARTESIAN_POINT('Ctrl Pts',(-1.15106142213831,17.5002549654215,-29.3091345217367));
#53591=CARTESIAN_POINT('Ctrl Pts',(-0.832103861684809,17.5080940958198,
-29.159954969786));
#53592=CARTESIAN_POINT('Ctrl Pts',(-0.175592799682984,17.5220165545405,
-28.9557542080835));
#53593=CARTESIAN_POINT('Ctrl Pts',(0.16214713396049,17.5276310629496,-28.9013011251849));
#53594=CARTESIAN_POINT('Ctrl Pts',(0.837852866039515,17.5276310629496,-28.9013011251849));
#53595=CARTESIAN_POINT('Ctrl Pts',(1.17559279968299,17.5220165545405,-28.9557542080835));
#53596=CARTESIAN_POINT('Ctrl Pts',(1.83210386168481,17.5080940958198,-29.159954969786));
#53597=CARTESIAN_POINT('Ctrl Pts',(2.15106142213831,17.5002549654215,-29.3091345217367));
#53598=CARTESIAN_POINT('Ctrl Pts',(3.05916685178659,17.4995083226735,-29.8550497469961));
#53599=CARTESIAN_POINT('Ctrl Pts',(3.6011888924699,17.535141250987,-30.3506021402247));
#53600=CARTESIAN_POINT('Ctrl Pts',(4.4592693304692,17.7485952235782,-31.3506571606591));
#53601=CARTESIAN_POINT('Ctrl Pts',(4.84102577827634,17.9371488532237,-31.9299741647106));
#53602=CARTESIAN_POINT('Ctrl Pts',(5.30317151084732,18.4633280213185,-32.9413234995576));
#53603=CARTESIAN_POINT('Ctrl Pts',(5.43322575640614,18.7577882106247,-33.3776378158014));
#53604=CARTESIAN_POINT('Ctrl Pts',(5.47974928497605,19.0969304167095,-33.767306956549));
#53605=CARTESIAN_POINT('',(6.46850196850286,19.4038059222874,-34.0961940777125));
#53606=CARTESIAN_POINT('Ctrl Pts',(6.46850196850286,19.4038059222874,-34.0961940777125));
#53607=CARTESIAN_POINT('Ctrl Pts',(6.42969677477097,19.387186062691,-34.0795742181161));
#53608=CARTESIAN_POINT('Ctrl Pts',(6.39051727695282,19.3709872335019,-34.0631950428732));
#53609=CARTESIAN_POINT('Ctrl Pts',(6.35094365239953,19.3552171637802,-34.0470861662623));
#53610=CARTESIAN_POINT('Ctrl Pts',(6.33115684012288,19.3473321289194,-34.0390317279569));
#53611=CARTESIAN_POINT('Ctrl Pts',(6.31127148089585,19.3395543228797,-34.0310448643094));
#53612=CARTESIAN_POINT('Ctrl Pts',(6.29128481869646,19.3318848880616,-34.023129591521));
#53613=CARTESIAN_POINT('Ctrl Pts',(6.27129815649708,19.3242154532436,-34.0152143187326));
#53614=CARTESIAN_POINT('Ctrl Pts',(6.25120089560369,19.3166511660681,-34.0073671890898));
#53615=CARTESIAN_POINT('Ctrl Pts',(6.23106051252081,19.3092186682823,-33.9996189280884));
#53616=CARTESIAN_POINT('Ctrl Pts',(6.15049898018926,19.279488677139,-33.9686258840826));
#53617=CARTESIAN_POINT('Ctrl Pts',(6.0690345181408,19.251780884441,-33.9391267241935));
#53618=CARTESIAN_POINT('Ctrl Pts',(5.98660180893713,19.226111117583,-33.9113473005207));
#53619=CARTESIAN_POINT('Ctrl Pts',(5.90416909973346,19.200441350725,-33.8835678768478));
#53620=CARTESIAN_POINT('Ctrl Pts',(5.82076819215945,19.1768094474068,-33.857508189391));
#53621=CARTESIAN_POINT('Ctrl Pts',(5.73632102160145,19.1552595186588,-33.8334154664541));
#53622=CARTESIAN_POINT('Ctrl Pts',(5.65187385104345,19.1337095899108,-33.8093227435172));
#53623=CARTESIAN_POINT('Ctrl Pts',(5.56638048594122,19.1142413799255,-33.7871969851001));
#53624=CARTESIAN_POINT('Ctrl Pts',(5.47974928497605,19.0969304167095,-33.767306956549));
#53625=CARTESIAN_POINT('',(9.,21.8205505282297,-35.623724356958));
#53626=CARTESIAN_POINT('Ctrl Pts',(9.00000000000001,21.8205505282297,-35.623724356958));
#53627=CARTESIAN_POINT('Ctrl Pts',(8.95346014289149,21.7244577489746,-35.5895246861726));
#53628=CARTESIAN_POINT('Ctrl Pts',(8.90405895499889,21.6302929744456,-35.5534659740372));
#53629=CARTESIAN_POINT('Ctrl Pts',(8.85183957948243,21.5379901961101,-35.515689114795));
#53630=CARTESIAN_POINT('Ctrl Pts',(8.8287249881567,21.4971329285086,-35.4989674161091));
#53631=CARTESIAN_POINT('Ctrl Pts',(8.8050575608266,21.4566406978177,-35.4819090745412));
#53632=CARTESIAN_POINT('Ctrl Pts',(8.78083801363281,21.416508970204,-35.4645263096883));
#53633=CARTESIAN_POINT('Ctrl Pts',(8.76110421713693,21.3838101199976,-35.4503630414241));
#53634=CARTESIAN_POINT('Ctrl Pts',(8.74100391086643,21.35135072485,-35.4359841712445));
#53635=CARTESIAN_POINT('Ctrl Pts',(8.72053669502811,21.3191288718177,-35.4213959497807));
#53636=CARTESIAN_POINT('Ctrl Pts',(8.70006947918979,21.2869070187855,-35.4068077283168));
#53637=CARTESIAN_POINT('Ctrl Pts',(8.67929735859121,21.2550205867036,-35.3920543871654));
#53638=CARTESIAN_POINT('Ctrl Pts',(8.65823682537814,21.2234794248792,-35.3771535198539));
#53639=CARTESIAN_POINT('Ctrl Pts',(8.61611575895202,21.1603971012304,-35.3473517852309));
#53640=CARTESIAN_POINT('Ctrl Pts',(8.57282604017638,21.0986702165659,-35.3169489172681));
#53641=CARTESIAN_POINT('Ctrl Pts',(8.52839379871621,21.0382364371097,-35.2860138780974));
#53642=CARTESIAN_POINT('Ctrl Pts',(8.46854242649671,20.9568305815868,-35.2443435845631));
#53643=CARTESIAN_POINT('Ctrl Pts',(8.40661847193035,20.8777689016067,-35.2017079160559));
#53644=CARTESIAN_POINT('Ctrl Pts',(8.34265344218604,20.8009353674463,-35.1582674769016));
#53645=CARTESIAN_POINT('Ctrl Pts',(8.31164622513931,20.7636901089089,-35.1372096093317));
#53646=CARTESIAN_POINT('Ctrl Pts',(8.28015866509545,20.7269687611952,-35.115962632633));
#53647=CARTESIAN_POINT('Ctrl Pts',(8.24819049410234,20.6907602051346,-35.0945448411895));
#53648=CARTESIAN_POINT('Ctrl Pts',(8.18110789572019,20.6147795046832,-35.0496013534325));
#53649=CARTESIAN_POINT('Ctrl Pts',(8.11191331368323,20.5410566675232,-35.003903946791));
#53650=CARTESIAN_POINT('Ctrl Pts',(8.04057741178885,20.469516804865,-34.9576259860006));
#53651=CARTESIAN_POINT('Ctrl Pts',(8.00778951765573,20.4366351648935,-34.9363553937911));
#53652=CARTESIAN_POINT('Ctrl Pts',(7.97454868755145,20.4042151472244,-34.914962155559));
#53653=CARTESIAN_POINT('Ctrl Pts',(7.94084935210846,20.3722519745585,-34.8934631048989));
#53654=CARTESIAN_POINT('Ctrl Pts',(7.8873402320094,20.3214996014792,-34.8593260731544));
#53655=CARTESIAN_POINT('Ctrl Pts',(7.83267546585817,20.2718982517448,-34.8249228107028));
#53656=CARTESIAN_POINT('Ctrl Pts',(7.77682107172572,20.2234349384799,-34.7903266757456));
#53657=CARTESIAN_POINT('Ctrl Pts',(7.76285747319261,20.2113191101637,-34.7816776420063));
#53658=CARTESIAN_POINT('Ctrl Pts',(7.74883069321957,20.1992842918547,-34.7730235674644));
#53659=CARTESIAN_POINT('Ctrl Pts',(7.73475444641459,20.1873416529407,-34.7643742580291));
#53660=CARTESIAN_POINT('Ctrl Pts',(7.72067819960961,20.1753990140267,-34.7557249485937));
#53661=CARTESIAN_POINT('Ctrl Pts',(7.70654820889115,20.1635448369695,-34.7470777562327));
#53662=CARTESIAN_POINT('Ctrl Pts',(7.6923643113654,20.1517783193376,-34.7384339183794));
#53663=CARTESIAN_POINT('Ctrl Pts',(7.66399651631389,20.1282452840736,-34.7211462426727));
#53664=CARTESIAN_POINT('Ctrl Pts',(7.63541313595312,20.1050628364807,-34.7038719849967));
#53665=CARTESIAN_POINT('Ctrl Pts',(7.60661239183694,20.0822251919125,-34.6866213041936));
#53666=CARTESIAN_POINT('Ctrl Pts',(7.52978950224896,20.0213082294883,-34.6406069671573));
#53667=CARTESIAN_POINT('Ctrl Pts',(7.45142280256881,19.9628419279767,-34.5947564545559));
#53668=CARTESIAN_POINT('Ctrl Pts',(7.37145495609334,19.9067437857951,-34.54928088283));
#53669=CARTESIAN_POINT('Ctrl Pts',(7.33150367449569,19.8787176130997,-34.5265616593933));
#53670=CARTESIAN_POINT('Ctrl Pts',(7.29115221492108,19.8512831242448,-34.5039360181928));
#53671=CARTESIAN_POINT('Ctrl Pts',(7.25039045889862,19.8244338918418,-34.4814302842056));
#53672=CARTESIAN_POINT('Ctrl Pts',(7.18921452103797,19.7841381064446,-34.4476532952272));
#53673=CARTESIAN_POINT('Ctrl Pts',(7.1271146527043,19.7451597465569,-34.4141481991929));
#53674=CARTESIAN_POINT('Ctrl Pts',(7.06404548727158,19.7074866640624,-34.3810173460166));
#53675=CARTESIAN_POINT('Ctrl Pts',(7.00097632183886,19.6698135815678,-34.3478864928404));
#53676=CARTESIAN_POINT('Ctrl Pts',(6.93693791838452,19.6334456770075,-34.3151298825222));
#53677=CARTESIAN_POINT('Ctrl Pts',(6.87187092606532,19.5983834435419,-34.2828624501986));
#53678=CARTESIAN_POINT('Ctrl Pts',(6.80680393374611,19.5633212100763,-34.250595017875));
#53679=CARTESIAN_POINT('Ctrl Pts',(6.74070843553403,19.5295644892472,-34.218816763546));
#53680=CARTESIAN_POINT('Ctrl Pts',(6.67350874794502,19.4971276142215,-34.1876584164691));
#53681=CARTESIAN_POINT('Ctrl Pts',(6.606309060356,19.4646907391959,-34.1565000693923));
#53682=CARTESIAN_POINT('Ctrl Pts',(6.53800530034302,19.4335734741426,-34.1259616295677));
#53683=CARTESIAN_POINT('Ctrl Pts',(6.46850196850286,19.4038059222874,-34.0961940777125));
#53684=CARTESIAN_POINT('',(9.,21.8205505282297,-23.3762756430421));
#53685=CARTESIAN_POINT('Origin',(9.,24.,-29.5));
#53686=CARTESIAN_POINT('',(-0.4749371855331,23.5,-23.0192593015922));
#53687=CARTESIAN_POINT('Ctrl Pts',(-0.474937185533098,23.5,-23.0192593015921));
#53688=CARTESIAN_POINT('Ctrl Pts',(-0.424823582743024,23.0013759479572,
-23.0577289823931));
#53689=CARTESIAN_POINT('Ctrl Pts',(-0.296594058108877,22.5028914382015,
-23.1564811915671));
#53690=CARTESIAN_POINT('Ctrl Pts',(0.15897422172366,21.4311680507649,-23.4946656308148));
#53691=CARTESIAN_POINT('Ctrl Pts',(0.540730669530802,20.8882015186037,-23.7709770626967));
#53692=CARTESIAN_POINT('Ctrl Pts',(1.3988111075301,20.0301210806044,-24.3271879977151));
#53693=CARTESIAN_POINT('Ctrl Pts',(1.9408331482134,19.6545163376753,-24.6524001701562));
#53694=CARTESIAN_POINT('Ctrl Pts',(2.84893857786169,19.2690239360916,-25.0389484840403));
#53695=CARTESIAN_POINT('Ctrl Pts',(3.16789613831519,19.1690811655562,-25.1499774591023));
#53696=CARTESIAN_POINT('Ctrl Pts',(3.82440720031701,19.0345340872051,-25.3042138673978));
#53697=CARTESIAN_POINT('Ctrl Pts',(4.16214713396049,19.,-25.346688068541));
#53698=CARTESIAN_POINT('Ctrl Pts',(4.83785286603951,19.,-25.346688068541));
#53699=CARTESIAN_POINT('Ctrl Pts',(5.17559279968299,19.0345340872051,-25.3042138673978));
#53700=CARTESIAN_POINT('Ctrl Pts',(5.83210386168481,19.1690811655562,-25.1499774591023));
#53701=CARTESIAN_POINT('Ctrl Pts',(6.15106142213831,19.2690239360916,-25.0389484840403));
#53702=CARTESIAN_POINT('Ctrl Pts',(7.0591668517866,19.6545163376753,-24.6524001701562));
#53703=CARTESIAN_POINT('Ctrl Pts',(7.6011888924699,20.0301210806044,-24.3271879977151));
#53704=CARTESIAN_POINT('Ctrl Pts',(8.40704600281358,20.8359781909481,-23.8048284181393));
#53705=CARTESIAN_POINT('Ctrl Pts',(8.74715233812993,21.2984854410813,-23.5620799693133));
#53706=CARTESIAN_POINT('Ctrl Pts',(9.00000000000001,21.8205505282297,-23.376275643042));
#53707=CARTESIAN_POINT('',(-27.5,23.5,-23.0192593015922));
#53708=CARTESIAN_POINT('',(-27.5,23.5,-23.0192593015922));
#53709=CARTESIAN_POINT('',(-27.5,24.5,-23.0192593015922));
#53710=CARTESIAN_POINT('Origin',(-27.5,24.,-29.5));
#53711=CARTESIAN_POINT('',(-2.16746515426235,24.5,-23.0192593015922));
#53712=CARTESIAN_POINT('',(-27.5,24.5,-23.0192593015922));
#53713=CARTESIAN_POINT('',(5.47974928497604,28.9030695832906,-25.2326930434511));
#53714=CARTESIAN_POINT('Ctrl Pts',(-2.16746515426287,24.5000000000004,-23.0192593015922));
#53715=CARTESIAN_POINT('Ctrl Pts',(-2.4880924621126,24.7655201130862,-23.0397446230579));
#53716=CARTESIAN_POINT('Ctrl Pts',(-2.78031808130512,25.0593693334481,-23.0797009860313));
#53717=CARTESIAN_POINT('Ctrl Pts',(-3.4592693304692,25.8506571606591,-23.2485952235782));
#53718=CARTESIAN_POINT('Ctrl Pts',(-3.84102577827635,26.4299741647106,-23.4371488532237));
#53719=CARTESIAN_POINT('Ctrl Pts',(-4.36201868849172,27.570103340577,-24.0303288758009));
#53720=CARTESIAN_POINT('Ctrl Pts',(-4.5,28.1300689255403,-24.4376807701152));
#53721=CARTESIAN_POINT('Ctrl Pts',(-4.5,29.0623192298848,-25.3699310744596));
#53722=CARTESIAN_POINT('Ctrl Pts',(-4.36201868849172,29.4696711241991,-25.929896659423));
#53723=CARTESIAN_POINT('Ctrl Pts',(-3.84102577827634,30.0628511467763,-27.0700258352893));
#53724=CARTESIAN_POINT('Ctrl Pts',(-3.4592693304692,30.2514047764218,-27.6493428393408));
#53725=CARTESIAN_POINT('Ctrl Pts',(-2.6011888924699,30.464858749013,-28.6493978597753));
#53726=CARTESIAN_POINT('Ctrl Pts',(-2.05916685178659,30.5004916773265,-29.1449502530038));
#53727=CARTESIAN_POINT('Ctrl Pts',(-1.1510614221383,30.4997450345785,-29.6908654782632));
#53728=CARTESIAN_POINT('Ctrl Pts',(-0.832103861684804,30.4919059041802,
-29.8400450302139));
#53729=CARTESIAN_POINT('Ctrl Pts',(-0.17559279968298,30.4779834454595,-30.0442457919164));
#53730=CARTESIAN_POINT('Ctrl Pts',(0.162147133960491,30.4723689370504,-30.098698874815));
#53731=CARTESIAN_POINT('Ctrl Pts',(0.500000000000003,30.4723689370504,-30.098698874815));
#53732=CARTESIAN_POINT('Ctrl Pts',(0.837852866039515,30.4723689370504,-30.098698874815));
#53733=CARTESIAN_POINT('Ctrl Pts',(1.17559279968299,30.4779834454595,-30.0442457919164));
#53734=CARTESIAN_POINT('Ctrl Pts',(1.83210386168481,30.4919059041802,-29.8400450302139));
#53735=CARTESIAN_POINT('Ctrl Pts',(2.15106142213831,30.4997450345785,-29.6908654782632));
#53736=CARTESIAN_POINT('Ctrl Pts',(3.05916685178659,30.5004916773265,-29.1449502530038));
#53737=CARTESIAN_POINT('Ctrl Pts',(3.6011888924699,30.464858749013,-28.6493978597753));
#53738=CARTESIAN_POINT('Ctrl Pts',(4.4592693304692,30.2514047764218,-27.6493428393408));
#53739=CARTESIAN_POINT('Ctrl Pts',(4.84102577827634,30.0628511467763,-27.0700258352893));
#53740=CARTESIAN_POINT('Ctrl Pts',(5.30317151084787,29.5366719786809,-26.0586765004412));
#53741=CARTESIAN_POINT('Ctrl Pts',(5.43322575640683,29.2422117893737,-25.6223621841961));
#53742=CARTESIAN_POINT('Ctrl Pts',(5.47974928497643,28.9030695832877,-25.2326930434478));
#53743=CARTESIAN_POINT('Ctrl Pts',(9.00000000000001,26.1794494717703,-23.3762756430421));
#53744=CARTESIAN_POINT('Ctrl Pts',(8.95705829231163,26.2681130022172,-23.4078312247981));
#53745=CARTESIAN_POINT('Ctrl Pts',(8.91168036869606,26.3551343885975,-23.4409704863788));
#53746=CARTESIAN_POINT('Ctrl Pts',(8.86390090675223,26.4405673266778,-23.4755804326099));
#53747=CARTESIAN_POINT('Ctrl Pts',(8.84001117578032,26.4832837957179,-23.4928854057254));
#53748=CARTESIAN_POINT('Ctrl Pts',(8.81552054185688,26.5256028638167,-23.5105582058587));
#53749=CARTESIAN_POINT('Ctrl Pts',(8.79043025746389,26.5675295920083,-23.528585446793));
#53750=CARTESIAN_POINT('Ctrl Pts',(8.7778851152674,26.5884929561041,-23.5375990672602));
#53751=CARTESIAN_POINT('Ctrl Pts',(8.76519002979884,26.609358216606,-23.5467012979276));
#53752=CARTESIAN_POINT('Ctrl Pts',(8.75234496374892,26.6301259112976,-23.5558905048174));
#53753=CARTESIAN_POINT('Ctrl Pts',(8.73949989769899,26.6508936059893,-23.5650797117071));
#53754=CARTESIAN_POINT('Ctrl Pts',(8.72649859393935,26.6715735006014,-23.5743603460415));
#53755=CARTESIAN_POINT('Ctrl Pts',(8.71336126912799,26.6921342492179,-23.5837162691274));
#53756=CARTESIAN_POINT('Ctrl Pts',(8.66081196988253,26.7743772436841,-23.6211399614708));
#53757=CARTESIAN_POINT('Ctrl Pts',(8.60632596649448,26.8543516336304,-23.6595986599364));
#53758=CARTESIAN_POINT('Ctrl Pts',(8.54996616236301,26.9321961195859,-23.6989459256624));
#53759=CARTESIAN_POINT('Ctrl Pts',(8.49360635823154,27.0100406055414,-23.7382931913885));
#53760=CARTESIAN_POINT('Ctrl Pts',(8.43537241023437,27.0857549441919,-23.778529024375));
#53761=CARTESIAN_POINT('Ctrl Pts',(8.3752944761572,27.1594450023802,-23.8195149862323));
#53762=CARTESIAN_POINT('Ctrl Pts',(8.31521654208003,27.2331350605686,-23.8605009480896));
#53763=CARTESIAN_POINT('Ctrl Pts',(8.25329445818045,27.30480070874,-23.9022370388178));
#53764=CARTESIAN_POINT('Ctrl Pts',(8.18952758291043,27.374520145879,-23.9445867313424));
#53765=CARTESIAN_POINT('Ctrl Pts',(8.1257607076404,27.4442395830179,-23.986936423867));
#53766=CARTESIAN_POINT('Ctrl Pts',(8.060149019676,27.5120127958191,-24.0298997181881));
#53767=CARTESIAN_POINT('Ctrl Pts',(7.99266073026277,27.5778933778524,-24.0733361102385));
#53768=CARTESIAN_POINT('Ctrl Pts',(7.92517244084954,27.6437739598858,-24.116772502289));
#53769=CARTESIAN_POINT('Ctrl Pts',(7.8558076658742,27.7077620280224,-24.1606819920687));
#53770=CARTESIAN_POINT('Ctrl Pts',(7.78450056732235,27.7698880650835,-24.2049132229263));
#53771=CARTESIAN_POINT('Ctrl Pts',(7.76667379268438,27.7854195743488,-24.2159710306407));
#53772=CARTESIAN_POINT('Ctrl Pts',(7.74873232686828,27.8008282864164,-24.22704452449));
#53773=CARTESIAN_POINT('Ctrl Pts',(7.73071339035289,27.8160832000095,-24.2381078488242));
#53774=CARTESIAN_POINT('Ctrl Pts',(7.71269445383749,27.8313381136026,-24.2491711731584));
#53775=CARTESIAN_POINT('Ctrl Pts',(7.69458755981618,27.8464484150864,-24.260230837196));
#53776=CARTESIAN_POINT('Ctrl Pts',(7.67639234498307,27.8614157598908,-24.2712842197217));
#53777=CARTESIAN_POINT('Ctrl Pts',(7.64000191531686,27.8913504494995,-24.2933909847731));
#53778=CARTESIAN_POINT('Ctrl Pts',(7.6032583061425,27.9207134511579,-24.315472623777));
#53779=CARTESIAN_POINT('Ctrl Pts',(7.5661573924812,27.9495162798162,-24.3375080087296));
#53780=CARTESIAN_POINT('Ctrl Pts',(7.49195556515859,28.0071219371326,-24.3815787786349));
#53781=CARTESIAN_POINT('Ctrl Pts',(7.41632621823999,28.0624890532935,-24.4254645323354));
#53782=CARTESIAN_POINT('Ctrl Pts',(7.33921485459175,28.1156845128685,-24.4689819138322));
#53783=CARTESIAN_POINT('Ctrl Pts',(7.26210349094351,28.1688799724435,-24.512499295329));
#53784=CARTESIAN_POINT('Ctrl Pts',(7.18351019104125,28.2199038792518,-24.555648304622));
#53785=CARTESIAN_POINT('Ctrl Pts',(7.10334918914321,28.2687905780663,-24.5982222579908));
#53786=CARTESIAN_POINT('Ctrl Pts',(7.02318818724517,28.3176772768808,-24.6407962113595));
#53787=CARTESIAN_POINT('Ctrl Pts',(6.94145966183726,28.3644270716961,-24.6827951088039));
#53788=CARTESIAN_POINT('Ctrl Pts',(6.85804161637582,28.4090406819896,-24.7239807093605));
#53789=CARTESIAN_POINT('Ctrl Pts',(6.77462357091438,28.4536542922832,-24.7651663099171));
#53790=CARTESIAN_POINT('Ctrl Pts',(6.68951653676254,28.4961321630524,-24.8055391316471));
#53791=CARTESIAN_POINT('Ctrl Pts',(6.60255363933461,28.536437830911,-24.8448166731826));
#53792=CARTESIAN_POINT('Ctrl Pts',(6.52294885299043,28.5733331526315,-24.88077086048));
#53793=CARTESIAN_POINT('Ctrl Pts',(6.44178967661408,28.6084080323174,-24.9158082171533));
#53794=CARTESIAN_POINT('Ctrl Pts',(6.35890495094121,28.6416023508446,-24.9496674442389));
#53795=CARTESIAN_POINT('Ctrl Pts',(6.35124366514855,28.6446706020678,-24.9527971549704));
#53796=CARTESIAN_POINT('Ctrl Pts',(6.34356763132479,28.6477227494887,-24.9559167999232));
#53797=CARTESIAN_POINT('Ctrl Pts',(6.33587671150817,28.6507587230625,-24.9590261727403));
#53798=CARTESIAN_POINT('Ctrl Pts',(6.31315265014489,28.6597289959861,-24.9682133155503));
#53799=CARTESIAN_POINT('Ctrl Pts',(6.29029836457671,28.6685582033252,-24.9773104490501));
#53800=CARTESIAN_POINT('Ctrl Pts',(6.26730968071364,28.6772445405875,-24.9863115407082));
#53801=CARTESIAN_POINT('Ctrl Pts',(6.24432099685057,28.6859308778499,-24.9953126323663));
#53802=CARTESIAN_POINT('Ctrl Pts',(6.22124816944649,28.6944552549752,-25.004197914353));
#53803=CARTESIAN_POINT('Ctrl Pts',(6.19810571453666,28.7028116039512,-25.0129560936244));
#53804=CARTESIAN_POINT('Ctrl Pts',(6.15182080471699,28.7195243019031,-25.0304724521673));
#53805=CARTESIAN_POINT('Ctrl Pts',(6.10523671422342,28.7355729176463,-25.0474882640567));
#53806=CARTESIAN_POINT('Ctrl Pts',(6.05834147324056,28.7509548359018,-25.0639622925458));
#53807=CARTESIAN_POINT('Ctrl Pts',(5.96455099127483,28.7817186724127,-25.0969103495238));
#53808=CARTESIAN_POINT('Ctrl Pts',(5.86951700719543,28.8098189622502,-25.1276912729003));
#53809=CARTESIAN_POINT('Ctrl Pts',(5.77312645725412,28.8351989642454,-25.1559407325179));
#53810=CARTESIAN_POINT('Ctrl Pts',(5.6767359073128,28.8605789662405,-25.1841901921354));
#53811=CARTESIAN_POINT('Ctrl Pts',(5.578988930962,28.8832391545062,-25.209908187994));
#53812=CARTESIAN_POINT('Ctrl Pts',(5.47974928497603,28.9030695832906,-25.2326930434511));
#53813=CARTESIAN_POINT('Ctrl Pts',(-0.479749284976029,24.449552064594,-35.9844354373545));
#53814=CARTESIAN_POINT('Ctrl Pts',(-0.433225756406109,24.9648995101448,
-35.9487074992219));
#53815=CARTESIAN_POINT('Ctrl Pts',(-0.303171510847291,25.4816351185375,
-35.848401484125));
#53816=CARTESIAN_POINT('Ctrl Pts',(0.158974221723663,26.5688319492351,-35.5053343691852));
#53817=CARTESIAN_POINT('Ctrl Pts',(0.540730669530803,27.1117984813963,-35.2290229373034));
#53818=CARTESIAN_POINT('Ctrl Pts',(1.3988111075301,27.9698789193956,-34.6728120022849));
#53819=CARTESIAN_POINT('Ctrl Pts',(1.9408331482134,28.3454836623247,-34.3475998298438));
#53820=CARTESIAN_POINT('Ctrl Pts',(2.84893857786169,28.7309760639084,-33.9610515159597));
#53821=CARTESIAN_POINT('Ctrl Pts',(3.16789613831519,28.8309188344438,-33.8500225408978));
#53822=CARTESIAN_POINT('Ctrl Pts',(3.82440720031702,28.965465912795,-33.6957861326022));
#53823=CARTESIAN_POINT('Ctrl Pts',(4.16214713396049,29.,-33.653311931459));
#53824=CARTESIAN_POINT('Ctrl Pts',(4.5,29.,-33.653311931459));
#53825=CARTESIAN_POINT('Ctrl Pts',(4.83785286603951,29.,-33.653311931459));
#53826=CARTESIAN_POINT('Ctrl Pts',(5.17559279968299,28.965465912795,-33.6957861326022));
#53827=CARTESIAN_POINT('Ctrl Pts',(5.83210386168481,28.8309188344438,-33.8500225408978));
#53828=CARTESIAN_POINT('Ctrl Pts',(6.15106142213831,28.7309760639084,-33.9610515159597));
#53829=CARTESIAN_POINT('Ctrl Pts',(7.05916685178659,28.3454836623247,-34.3475998298438));
#53830=CARTESIAN_POINT('Ctrl Pts',(7.6011888924699,27.9698789193956,-34.6728120022849));
#53831=CARTESIAN_POINT('Ctrl Pts',(8.40704600281352,27.164021809052,-35.1951715818606));
#53832=CARTESIAN_POINT('Ctrl Pts',(8.74715233812982,26.7015145589189,-35.4379200306866));
#53833=CARTESIAN_POINT('Ctrl Pts',(8.99999999999988,26.1794494717706,-35.6237243569579));
#53834=CARTESIAN_POINT('Origin',(4.5,24.,6.93889390390723E-15));
#53835=CARTESIAN_POINT('',(-0.4682273254511,23.4372236299906,-37.));
#53836=CARTESIAN_POINT('',(9.20487219075894,22.3076118445749,-37.));
#53837=CARTESIAN_POINT('Origin',(4.5,24.,-37.));
#53838=CARTESIAN_POINT('Ctrl Pts',(-0.468227325451101,23.4372236299906,
-37.));
#53839=CARTESIAN_POINT('Ctrl Pts',(-0.489596442334827,23.6258716189257,
-36.8053870417944));
#53840=CARTESIAN_POINT('Ctrl Pts',(-0.5,23.8141368149253,-36.6140664153501));
#53841=CARTESIAN_POINT('Ctrl Pts',(-0.5,24.1465968404519,-36.2816063898235));
#53842=CARTESIAN_POINT('Ctrl Pts',(-0.49353975798667,24.2967931218089,-36.1332972845454));
#53843=CARTESIAN_POINT('Ctrl Pts',(-0.479749284976031,24.449552064594,-35.9844354373545));
#53844=CARTESIAN_POINT('',(9.5,23.9999999737538,-35.9999999933889));
#53845=CARTESIAN_POINT('Ctrl Pts',(8.9999999999999,26.1794494717706,-35.6237243569579));
#53846=CARTESIAN_POINT('Ctrl Pts',(9.00499129300368,26.1691437423086,-35.6273921929549));
#53847=CARTESIAN_POINT('Ctrl Pts',(9.00995373459336,26.1588072269372,-35.6310416269391));
#53848=CARTESIAN_POINT('Ctrl Pts',(9.0148783576886,26.148458372271,-35.6346659517895));
#53849=CARTESIAN_POINT('Ctrl Pts',(9.01980298078383,26.1381095176048,-35.6382902766398));
#53850=CARTESIAN_POINT('Ctrl Pts',(9.02469199992633,26.1277437765558,-35.6418911200617));
#53851=CARTESIAN_POINT('Ctrl Pts',(9.02954542600208,26.117361124825,-35.6454683632644));
#53852=CARTESIAN_POINT('Ctrl Pts',(9.03782625969404,26.0996464195997,-35.6515717952679));
#53853=CARTESIAN_POINT('Ctrl Pts',(9.04600352023965,26.0818824635388,-35.6576065392216));
#53854=CARTESIAN_POINT('Ctrl Pts',(9.05407713254688,26.0640691586593,-35.6635718950109));
#53855=CARTESIAN_POINT('Ctrl Pts',(9.05546746601008,26.0610015808612,-35.6645991717067));
#53856=CARTESIAN_POINT('Ctrl Pts',(9.05685472633728,26.0579325366857,-35.665624391158));
#53857=CARTESIAN_POINT('Ctrl Pts',(9.05823891476301,26.0548620249938,-35.6666475507992));
#53858=CARTESIAN_POINT('Ctrl Pts',(9.07474419566317,26.018248759747,-35.6788478675838));
#53859=CARTESIAN_POINT('Ctrl Pts',(9.09081329757223,25.981425963608,-35.6907557840418));
#53860=CARTESIAN_POINT('Ctrl Pts',(9.10644398031607,25.9443956270176,-35.702364507792));
#53861=CARTESIAN_POINT('Ctrl Pts',(9.1086589941613,25.9391480821991,-35.7040095724545));
#53862=CARTESIAN_POINT('Ctrl Pts',(9.11086526354452,25.9338961913387,-35.7056486746972));
#53863=CARTESIAN_POINT('Ctrl Pts',(9.11306274833671,25.9286400605162,-35.7072817699926));
#53864=CARTESIAN_POINT('Ctrl Pts',(9.12802360671024,25.8928554083961,-35.7184001665852));
#53865=CARTESIAN_POINT('Ctrl Pts',(9.14258366284676,25.8568594685192,-35.7292449494624));
#53866=CARTESIAN_POINT('Ctrl Pts',(9.15672841971636,25.8206816235516,-35.7398011083539));
#53867=CARTESIAN_POINT('Ctrl Pts',(9.17322261740404,25.7784946469701,-35.752110642776));
#53868=CARTESIAN_POINT('Ctrl Pts',(9.1891563977555,25.7360515257514,-35.764030863753));
#53869=CARTESIAN_POINT('Ctrl Pts',(9.20453378247886,25.6933291108338,-35.7755585793107));
#53870=CARTESIAN_POINT('Ctrl Pts',(9.20718005181626,25.6859770793506,-35.7775423652899));
#53871=CARTESIAN_POINT('Ctrl Pts',(9.20980980902294,25.6786167048553,-35.7795145037213));
#53872=CARTESIAN_POINT('Ctrl Pts',(9.21242308500116,25.671247870195,-35.7814749876001));
#53873=CARTESIAN_POINT('Ctrl Pts',(9.23546015598842,25.6062886509707,-35.7987574356316));
#53874=CARTESIAN_POINT('Ctrl Pts',(9.2572083241211,25.5407013867059,-35.815128565412));
#53875=CARTESIAN_POINT('Ctrl Pts',(9.277647393158,25.4744769808417,-35.8305539170307));
#53876=CARTESIAN_POINT('Ctrl Pts',(9.28233239040935,25.4592971720703,-35.8340896812969));
#53877=CARTESIAN_POINT('Ctrl Pts',(9.28694852685422,25.4440836909435,-35.8375757061078));
#53878=CARTESIAN_POINT('Ctrl Pts',(9.29149540308989,25.42883609634,-35.8410114797098));
#53879=CARTESIAN_POINT('Ctrl Pts',(9.29365149253119,25.4216058186668,-35.8426406938784));
#53880=CARTESIAN_POINT('Ctrl Pts',(9.29579199751469,25.4143678777838,-35.84425859878));
#53881=CARTESIAN_POINT('Ctrl Pts',(9.29791690448527,25.4071222569905,-35.8458651628086));
#53882=CARTESIAN_POINT('Ctrl Pts',(9.31795789316064,25.3387854280019,-35.8610174174481));
#53883=CARTESIAN_POINT('Ctrl Pts',(9.33661353358467,25.269768592517,-35.8751629726986));
#53884=CARTESIAN_POINT('Ctrl Pts',(9.35385081458509,25.2000533307043,-35.888260097332));
#53885=CARTESIAN_POINT('Ctrl Pts',(9.35769303751339,25.1845136654066,-35.8911794714816));
#53886=CARTESIAN_POINT('Ctrl Pts',(9.36146465902595,25.1689391689937,-35.8940466623285));
#53887=CARTESIAN_POINT('Ctrl Pts',(9.36516507939256,25.1533294331882,-35.8968610404086));
#53888=CARTESIAN_POINT('Ctrl Pts',(9.36652977322614,25.1475726520426,-35.8978989669225));
#53889=CARTESIAN_POINT('Ctrl Pts',(9.36788477789201,25.1418110869741,-35.8989297055837));
#53890=CARTESIAN_POINT('Ctrl Pts',(9.36923008056749,25.1360447261538,-35.8999532391271));
#53891=CARTESIAN_POINT('Ctrl Pts',(9.3854250434066,25.0666283777718,-35.91227469511));
#53892=CARTESIAN_POINT('Ctrl Pts',(9.4002170109659,24.9965192841531,-35.9235542818067));
#53893=CARTESIAN_POINT('Ctrl Pts',(9.41356185655924,24.9256911858039,-35.9337460644235));
#53894=CARTESIAN_POINT('Ctrl Pts',(9.4170731352871,24.9070549870312,-35.9364277132482));
#53895=CARTESIAN_POINT('Ctrl Pts',(9.42048401358903,24.8883689383346,-35.9390338894768));
#53896=CARTESIAN_POINT('Ctrl Pts',(9.42379321375125,24.8696324419433,-35.9415633947187));
#53897=CARTESIAN_POINT('Ctrl Pts',(9.42449386001647,24.8656654240609,-35.942098958696));
#53898=CARTESIAN_POINT('Ctrl Pts',(9.42518994700153,24.8616961500279,-35.942631084413));
#53899=CARTESIAN_POINT('Ctrl Pts',(9.425881468401,24.8577246142275,-35.9431597654671));
#53900=CARTESIAN_POINT('Ctrl Pts',(9.42997413403971,24.8342196755289,-35.9462886849565));
#53901=CARTESIAN_POINT('Ctrl Pts',(9.43390864964311,24.8106232721573,-35.9492982524213));
#53902=CARTESIAN_POINT('Ctrl Pts',(9.43767033422769,24.7870207768946,-35.9521769341472));
#53903=CARTESIAN_POINT('Ctrl Pts',(9.44143201881227,24.763418281632,-35.9550556158731));
#53904=CARTESIAN_POINT('Ctrl Pts',(9.4450238707641,24.739793515833,-35.9578057016672));
#53905=CARTESIAN_POINT('Ctrl Pts',(9.44844616386937,24.7161465195238,-35.9604270560455));
#53906=CARTESIAN_POINT('Ctrl Pts',(9.45496209937026,24.6711234025667,-35.9654180300881));
#53907=CARTESIAN_POINT('Ctrl Pts',(9.46086375084294,24.6260198076498,-35.9699425212052));
#53908=CARTESIAN_POINT('Ctrl Pts',(9.46614854505997,24.5808346182974,-35.9739964724846));
#53909=CARTESIAN_POINT('Ctrl Pts',(9.46641509947409,24.5785555680298,-35.9742009456511));
#53910=CARTESIAN_POINT('Ctrl Pts',(9.46668008379669,24.576276311642,-35.9744042210618));
#53911=CARTESIAN_POINT('Ctrl Pts',(9.46694349854552,24.5739968483365,-35.9746062989503));
#53912=CARTESIAN_POINT('Ctrl Pts',(9.47560463179607,24.499047607582,-35.9812506631203));
#53913=CARTESIAN_POINT('Ctrl Pts',(9.48257224643251,24.4238758991093,-35.9866025262799));
#53914=CARTESIAN_POINT('Ctrl Pts',(9.48784091893968,24.3484791237477,-35.9906514402046));
#53915=CARTESIAN_POINT('Ctrl Pts',(9.48920116350454,24.3290134891398,-35.9916967724305));
#53916=CARTESIAN_POINT('Ctrl Pts',(9.4904479529791,24.3095328743889,-35.992655092703));
#53917=CARTESIAN_POINT('Ctrl Pts',(9.49158074820727,24.2900373108998,-35.9935258759464));
#53918=CARTESIAN_POINT('Ctrl Pts',(9.49161858693997,24.2893861010455,-35.9935549626988));
#53919=CARTESIAN_POINT('Ctrl Pts',(9.49165629872179,24.2887348743351,-35.9935839519911));
#53920=CARTESIAN_POINT('Ctrl Pts',(9.49169388354752,24.2880836307525,-35.9936128438172));
#53921=CARTESIAN_POINT('Ctrl Pts',(9.49444525199611,24.2404098419077,-35.9957278478682));
#53922=CARTESIAN_POINT('Ctrl Pts',(9.49651672032079,24.1926463019363,-35.9973208722724));
#53923=CARTESIAN_POINT('Ctrl Pts',(9.4979030806664,24.1447922723031,-35.9983871160602));
#53924=CARTESIAN_POINT('Ctrl Pts',(9.49790768768555,24.1446332484015,-35.9983906592989));
#53925=CARTESIAN_POINT('Ctrl Pts',(9.49791228713675,24.1444742234989,-35.9983941967189));
#53926=CARTESIAN_POINT('Ctrl Pts',(9.49791687901979,24.1443151975952,-35.9983977283201));
#53927=CARTESIAN_POINT('Ctrl Pts',(9.49860889038041,24.1203494887779,-35.998929951839));
#53928=CARTESIAN_POINT('Ctrl Pts',(9.49912904440715,24.0963610829959,-35.9993300507007));
#53929=CARTESIAN_POINT('Ctrl Pts',(9.49947652234889,24.072349866447,-35.9995973318569));
#53930=CARTESIAN_POINT('Ctrl Pts',(9.49947711854897,24.0723086681791,-35.9995977904559));
#53931=CARTESIAN_POINT('Ctrl Pts',(9.49947771424067,24.072267469844,-35.9995982486639));
#53932=CARTESIAN_POINT('Ctrl Pts',(9.49947830942397,24.0722262714417,-35.9995987064809));
#53933=CARTESIAN_POINT('Ctrl Pts',(9.49965176461951,24.060219756981,-35.9997321287929));
#53934=CARTESIAN_POINT('Ctrl Pts',(9.49978204199234,24.0482075968042,-35.9998323411043));
#53935=CARTESIAN_POINT('Ctrl Pts',(9.4998690295622,24.0361896019762,-35.9998992537352));
#53936=CARTESIAN_POINT('Ctrl Pts',(9.49986917252243,24.0361698509338,-35.9998993637031));
#53937=CARTESIAN_POINT('Ctrl Pts',(9.49986931536621,24.0361500999239,-35.9998994735815));
#53938=CARTESIAN_POINT('Ctrl Pts',(9.49986945809355,24.0361303489459,-35.9998995833703));
#53939=CARTESIAN_POINT('Ctrl Pts',(9.49991295239155,24.0301114956676,-35.9999330400806));
#53940=CARTESIAN_POINT('Ctrl Pts',(9.49994564654914,24.024091208166,-35.9999581449458));
#53941=CARTESIAN_POINT('Ctrl Pts',(9.49996740821826,24.0180694839239,-35.9999748847169));
#53942=CARTESIAN_POINT('Ctrl Pts',(9.49997828905281,24.0150586218028,-35.9999832546024));
#53943=CARTESIAN_POINT('Ctrl Pts',(9.49998644052914,24.0120474005484,-35.9999895333668));
#53944=CARTESIAN_POINT('Ctrl Pts',(9.49999186825306,24.0090358199681,-35.9999937197092));
#53945=CARTESIAN_POINT('Ctrl Pts',(9.49999458211502,24.0075300296779,-35.9999958128805));
#53946=CARTESIAN_POINT('Ctrl Pts',(9.49999661789029,24.0060222106567,-35.999997382956));
#53947=CARTESIAN_POINT('Ctrl Pts',(9.49999797235682,24.0045152712213,-35.9999984297334));
#53948=CARTESIAN_POINT('Ctrl Pts',(9.49999932682335,24.0030083317859,-35.9999994765107));
#53949=CARTESIAN_POINT('Ctrl Pts',(9.5,24.0015022719398,-36.));
#53950=CARTESIAN_POINT('Ctrl Pts',(9.5,24.,-36.));
#53951=CARTESIAN_POINT('Ctrl Pts',(9.5,23.9999999737538,-36.));
#53952=CARTESIAN_POINT('Ctrl Pts',(9.49999999993673,23.9879832282049,-35.999999999951));
#53953=CARTESIAN_POINT('Ctrl Pts',(9.49995667919472,23.9759763925916,-35.9999666761675));
#53954=CARTESIAN_POINT('Ctrl Pts',(9.4998702522827,23.9639797232321,-35.9999001945923));
#53955=CARTESIAN_POINT('Ctrl Pts',(9.49986975477033,23.9639106649817,-35.9998998118944));
#53956=CARTESIAN_POINT('Ctrl Pts',(9.49986925582743,23.9638416067762,-35.999899428096));
#53957=CARTESIAN_POINT('Ctrl Pts',(9.49986875545392,23.9637725486055,-35.9998990431972));
#53958=CARTESIAN_POINT('Ctrl Pts',(9.4997819986771,23.9517989644353,-35.9998323078902));
#53959=CARTESIAN_POINT('Ctrl Pts',(9.49965230110543,23.9398353051175,-35.999732542221));
#53960=CARTESIAN_POINT('Ctrl Pts',(9.49947986548288,23.9278815245469,-35.9995999050319));
#53961=CARTESIAN_POINT('Ctrl Pts',(9.49913150351934,23.9037319758056,-35.9993319455991));
#53962=CARTESIAN_POINT('Ctrl Pts',(9.49860871944609,23.8796227420958,-35.9989298298439));
#53963=CARTESIAN_POINT('Ctrl Pts',(9.4979130841039,23.8555534571282,-35.9983948168954));
#53964=CARTESIAN_POINT('Ctrl Pts',(9.49652417723533,23.8074966762467,-35.9973266090085));
#53965=CARTESIAN_POINT('Ctrl Pts',(9.49444633029436,23.7595991165855,-35.9957286757378));
#53966=CARTESIAN_POINT('Ctrl Pts',(9.49169052182656,23.7118581368826,-35.9936102643782));
#53967=CARTESIAN_POINT('Ctrl Pts',(9.49166437530495,23.7114051806732,-35.9935901653441));
#53968=CARTESIAN_POINT('Ctrl Pts',(9.49163816771039,23.7109522385841,-35.9935700194233));
#53969=CARTESIAN_POINT('Ctrl Pts',(9.49161189904947,23.7104993106094,-35.9935498266216));
#53970=CARTESIAN_POINT('Ctrl Pts',(9.48730051343738,23.6361617888405,-35.9902356510239));
#53971=CARTESIAN_POINT('Ctrl Pts',(9.48134411968866,23.5622032194035,-35.985658281014));
#53972=CARTESIAN_POINT('Ctrl Pts',(9.4737793415769,23.4886172124655,-35.9798518103728));
#53973=CARTESIAN_POINT('Ctrl Pts',(9.47168117086805,23.4682073601132,-35.9782413247193));
#53974=CARTESIAN_POINT('Ctrl Pts',(9.46945903056611,23.4478260956439,-35.9765361006218));
#53975=CARTESIAN_POINT('Ctrl Pts',(9.46711315648697,23.4274731548101,-35.9747364429526));
#53976=CARTESIAN_POINT('Ctrl Pts',(9.46682390991277,23.4249636346004,-35.9745145449317));
#53977=CARTESIAN_POINT('Ctrl Pts',(9.46653278205061,23.4224545465678,-35.9742912113484));
#53978=CARTESIAN_POINT('Ctrl Pts',(9.46623977303,23.4199458895996,-35.9740664425365));
#53979=CARTESIAN_POINT('Ctrl Pts',(9.45768749974971,23.3467238436917,-35.9675059472304));
#53980=CARTESIAN_POINT('Ctrl Pts',(9.44753564796578,23.2738705364315,-35.9597251325201));
#53981=CARTESIAN_POINT('Ctrl Pts',(9.43580765437234,23.2013794401489,-35.9507515376106));
#53982=CARTESIAN_POINT('Ctrl Pts',(9.43285767755637,23.1831455409151,-35.9484943828186));
#53983=CARTESIAN_POINT('Ctrl Pts',(9.42980777681206,23.1649345853686,-35.9461616054021));
#53984=CARTESIAN_POINT('Ctrl Pts',(9.4266579217613,23.1467465545623,-35.9437533337836));
#53985=CARTESIAN_POINT('Ctrl Pts',(9.42576245566971,23.1415759150893,-35.9430686909861));
#53986=CARTESIAN_POINT('Ctrl Pts',(9.42485891395591,23.1364071539974,-35.9423779507369));
#53987=CARTESIAN_POINT('Ctrl Pts',(9.42394729195393,23.1312402617232,-35.9416811131217));
#53988=CARTESIAN_POINT('Ctrl Pts',(9.41145567335541,23.0604402508758,-35.9321326054124));
#53989=CARTESIAN_POINT('Ctrl Pts',(9.3974493622803,22.989987995806,-35.9214411733268));
#53990=CARTESIAN_POINT('Ctrl Pts',(9.38193889031453,22.919878173417,-35.9096276267171));
#53991=CARTESIAN_POINT('Ctrl Pts',(9.37822780110102,22.9031034546204,-35.9068010766616));
#53992=CARTESIAN_POINT('Ctrl Pts',(9.37443043919327,22.8863484537643,-35.9039101676379));
#53993=CARTESIAN_POINT('Ctrl Pts',(9.37054664849344,22.869613341837,-35.9009549643899));
#53994=CARTESIAN_POINT('Ctrl Pts',(9.36883796974234,22.8622507076588,-35.8996548188916));
#53995=CARTESIAN_POINT('Ctrl Pts',(9.36711255863853,22.8548919158162,-35.8983422262096));
#53996=CARTESIAN_POINT('Ctrl Pts',(9.36537039239681,22.847536978434,-35.8970171856514));
#53997=CARTESIAN_POINT('Ctrl Pts',(9.3491022086485,22.7788572681249,-35.8846440821217));
#53998=CARTESIAN_POINT('Ctrl Pts',(9.33137622497279,22.7105113237437,-35.8711879248514));
#53999=CARTESIAN_POINT('Ctrl Pts',(9.31218977679271,22.6424941274949,-35.8566633015094));
#54000=CARTESIAN_POINT('Ctrl Pts',(9.3078168676122,22.6269918824146,-35.8533528993881));
#54001=CARTESIAN_POINT('Ctrl Pts',(9.30336798785164,22.61150688569,-35.8499869250491));
#54002=CARTESIAN_POINT('Ctrl Pts',(9.29884292932156,22.5960394019589,-35.8465654366677));
#54003=CARTESIAN_POINT('Ctrl Pts',(9.29649960113552,22.5880294744954,-35.8447935987767));
#54004=CARTESIAN_POINT('Ctrl Pts',(9.29413504811975,22.5800215351618,-35.8430062534732));
#54005=CARTESIAN_POINT('Ctrl Pts',(9.29175146133901,22.5720231168623,-35.841205088392));
#54006=CARTESIAN_POINT('Ctrl Pts',(9.29076497192281,22.5687128304224,-35.8404596444653));
#54007=CARTESIAN_POINT('Ctrl Pts',(9.28977522583305,22.5654041754969,-35.8397118364184));
#54008=CARTESIAN_POINT('Ctrl Pts',(9.28878238789472,22.5620976773719,-35.8389617909375));
#54009=CARTESIAN_POINT('Ctrl Pts',(9.28539062367664,22.5508019143933,-35.8363994619553));
#54010=CARTESIAN_POINT('Ctrl Pts',(9.28196280007465,22.5395313504075,-35.83381102518));
#54011=CARTESIAN_POINT('Ctrl Pts',(9.27849919458226,22.5282857541102,-35.8311967941509));
#54012=CARTESIAN_POINT('Ctrl Pts',(9.27157198359749,22.5057945615158,-35.8259683320927));
#54013=CARTESIAN_POINT('Ctrl Pts',(9.26450166607527,22.4834032284448,-35.8206367170279));
#54014=CARTESIAN_POINT('Ctrl Pts',(9.25729019799672,22.4611101419525,-35.8152042084262));
#54015=CARTESIAN_POINT('Ctrl Pts',(9.24286726183961,22.416523968968,-35.8043391912229));
#54016=CARTESIAN_POINT('Ctrl Pts',(9.22787987878537,22.3723306029726,-35.7930710047512));
#54017=CARTESIAN_POINT('Ctrl Pts',(9.21234040799164,22.328519572134,-35.7814132280349));
#54018=CARTESIAN_POINT('Ctrl Pts',(9.20984952418266,22.3214969271019,-35.7795445564658));
#54019=CARTESIAN_POINT('Ctrl Pts',(9.20734448156848,22.3144842554121,-35.777665909801));
#54020=CARTESIAN_POINT('Ctrl Pts',(9.20482529266609,22.3074814655873,-35.7757773219761));
#54021=CARTESIAN_POINT('Ctrl Pts',(9.18941669728238,22.2646489670536,-35.7642257921909));
#54022=CARTESIAN_POINT('Ctrl Pts',(9.17347821168039,22.2221793804084,-35.7523018030587));
#54023=CARTESIAN_POINT('Ctrl Pts',(9.15702114870064,22.1800673676922,-35.740019618893));
#54024=CARTESIAN_POINT('Ctrl Pts',(9.14259793406756,22.143159773744,-35.7292553301129));
#54025=CARTESIAN_POINT('Ctrl Pts',(9.12777686460726,22.1065281322112,-35.7182162688711));
#54026=CARTESIAN_POINT('Ctrl Pts',(9.11256256614464,22.0701639208216,-35.7069100481183));
#54027=CARTESIAN_POINT('Ctrl Pts',(9.11062517609986,22.0655332990874,-35.7054703130175));
#54028=CARTESIAN_POINT('Ctrl Pts',(9.10868143263058,22.0609070795274,-35.7040262625053));
#54029=CARTESIAN_POINT('Ctrl Pts',(9.10673134009715,22.056285242096,-35.7025779089919));
#54030=CARTESIAN_POINT('Ctrl Pts',(9.08972898401151,22.0159886282527,-35.6899500865939));
#54031=CARTESIAN_POINT('Ctrl Pts',(9.07224401686274,21.9760239385094,-35.6769951131352));
#54032=CARTESIAN_POINT('Ctrl Pts',(9.05428095101055,21.9363805796518,-35.6637224850983));
#54033=CARTESIAN_POINT('Ctrl Pts',(9.03664587444707,21.8974610725676,-35.6506922032102));
#54034=CARTESIAN_POINT('Ctrl Pts',(9.01854981494461,21.8588511000046,-35.6373556303559));
#54035=CARTESIAN_POINT('Ctrl Pts',(9.00000000000002,21.8205505282297,-35.6237243569579));
#54036=CARTESIAN_POINT('Origin',(4.5000000000009,23.9999999999992,-38.6923881554236));
#54037=CARTESIAN_POINT('Origin',(0.5,48.5249973351313,-4.97500266486866));
#54038=CARTESIAN_POINT('',(0.499999999643868,29.0827333318928,-17.3461988580058));
#54039=CARTESIAN_POINT('Origin',(0.39600932023275,31.6849458844993,-16.7453161466531));
#54040=CARTESIAN_POINT('',(0.500000000000045,27.0000000000001,-19.4289321881344));
#54041=CARTESIAN_POINT('',(0.500000000000001,44.9894634291986,-1.43946875893592));
#54042=CARTESIAN_POINT('Ctrl Pts',(0.500000000000087,27.0000000000001,-19.4289321881344));
#54043=CARTESIAN_POINT('Ctrl Pts',(0.630063764891852,27.1734183531891,-19.2555138349454));
#54044=CARTESIAN_POINT('Ctrl Pts',(0.773900537595572,27.3419476067783,-19.0939257507809));
#54045=CARTESIAN_POINT('Ctrl Pts',(1.0711763811429,27.6443407962334,-18.8281986778164));
#54046=CARTESIAN_POINT('Ctrl Pts',(1.23509725261859,27.7938951449731,-18.7069951671099));
#54047=CARTESIAN_POINT('Ctrl Pts',(1.59835434231765,28.0784412787328,-18.5182617650791));
#54048=CARTESIAN_POINT('Ctrl Pts',(1.79823937131942,28.2134034590434,-18.4517453020891));
#54049=CARTESIAN_POINT('Ctrl Pts',(2.13279052698853,28.4069534387743,-18.406567444179));
#54050=CARTESIAN_POINT('Ctrl Pts',(2.27824207369039,28.4822099736569,-18.4051451043186));
#54051=CARTESIAN_POINT('Ctrl Pts',(2.5740138256679,28.6170327901994,-18.4449321123119));
#54052=CARTESIAN_POINT('Ctrl Pts',(2.72431574730796,28.6766212956434,-18.4862020423829));
#54053=CARTESIAN_POINT('Ctrl Pts',(3.16223201946421,28.8276016861915,-18.6686564412896));
#54054=CARTESIAN_POINT('Ctrl Pts',(3.43743466557115,28.8911112631435,-18.8720368348926));
#54055=CARTESIAN_POINT('Ctrl Pts',(4.00248687235112,28.9871400474885,-19.4284741379288));
#54056=CARTESIAN_POINT('Ctrl Pts',(4.27125162606028,28.9999868518442,-19.8261269612256));
#54057=CARTESIAN_POINT('Ctrl Pts',(4.72816585783078,29.0000131311922,-20.6874933896537));
#54058=CARTESIAN_POINT('Ctrl Pts',(4.91347393380979,28.9851063276177,-21.1527100259297));
#54059=CARTESIAN_POINT('Ctrl Pts',(5.35782996082894,28.9348711666866,-22.6030865324071));
#54060=CARTESIAN_POINT('Ctrl Pts',(5.5,28.8989794855664,-23.6390951228936));
#54061=CARTESIAN_POINT('Ctrl Pts',(5.5,28.8989794855664,-24.8083397544018));
#54062=CARTESIAN_POINT('Ctrl Pts',(5.49353975798667,28.900313920569,-25.0194149375122));
#54063=CARTESIAN_POINT('Ctrl Pts',(5.47974928497603,28.9030695832906,-25.2326930434511));
#54064=CARTESIAN_POINT('',(-0.474937185533102,24.5,-22.0646561030811));
#54065=CARTESIAN_POINT('Origin',(0.500000000032158,24.5000000000003,-29.0000000001026));
#54066=CARTESIAN_POINT('Ctrl Pts',(-0.4749371855331,24.5,-22.0646561030811));
#54067=CARTESIAN_POINT('Ctrl Pts',(-0.430283424779195,24.944299309697,-21.6078023728738));
#54068=CARTESIAN_POINT('Ctrl Pts',(-0.32422833575544,25.394363859076,-21.1270657168025));
#54069=CARTESIAN_POINT('Ctrl Pts',(0.00642096108058736,26.2359626137404,
-20.2237995433534));
#54070=CARTESIAN_POINT('Ctrl Pts',(0.22196880373164,26.6292917383089,-19.7996404498256));
#54071=CARTESIAN_POINT('Ctrl Pts',(0.500000000000088,27.0000000000001,-19.4289321881344));
#54072=CARTESIAN_POINT('Ctrl Pts',(0.499999999661276,29.0827333318934,-17.3461988580053));
#54073=CARTESIAN_POINT('Ctrl Pts',(0.494640286720631,29.0825598614636,-17.3463723338252));
#54074=CARTESIAN_POINT('Ctrl Pts',(0.489278323252304,29.0824021998227,-17.346542198886));
#54075=CARTESIAN_POINT('Ctrl Pts',(0.483914104352405,29.0822603694729,-17.3467084484518));
#54076=CARTESIAN_POINT('Ctrl Pts',(0.47082609449057,29.0819143215112,-17.3471140761857));
#54077=CARTESIAN_POINT('Ctrl Pts',(0.457724658694381,29.081662489745,-17.3474981872329));
#54078=CARTESIAN_POINT('Ctrl Pts',(0.444609710549237,29.0815054764053,-17.347860648805));
#54079=CARTESIAN_POINT('Ctrl Pts',(0.438786451655717,29.0814357598256,-17.3480215878762));
#54080=CARTESIAN_POINT('Ctrl Pts',(0.432961830886728,29.0813847595728,-17.3481782214898));
#54081=CARTESIAN_POINT('Ctrl Pts',(0.427137031146438,29.081352531438,-17.3483305042711));
#54082=CARTESIAN_POINT('Ctrl Pts',(0.419843412498221,29.0813121764498,-17.3485211876565));
#54083=CARTESIAN_POINT('Ctrl Pts',(0.412554916938757,29.0813012192184,-17.3487049200745));
#54084=CARTESIAN_POINT('Ctrl Pts',(0.405272700896496,29.0813195495914,-17.3488816941982));
#54085=CARTESIAN_POINT('Ctrl Pts',(0.310866975848777,29.0815571822215,-17.3511733715135));
#54086=CARTESIAN_POINT('Ctrl Pts',(0.217320839007321,29.0867132990217,-17.3523038451532));
#54087=CARTESIAN_POINT('Ctrl Pts',(0.124594312162254,29.0965585511847,-17.3523322354303));
#54088=CARTESIAN_POINT('Ctrl Pts',(0.114401347256358,29.0976407906818,-17.352335356232));
#54089=CARTESIAN_POINT('Ctrl Pts',(0.104218288490283,29.0987797030209,-17.3523251576095));
#54090=CARTESIAN_POINT('Ctrl Pts',(0.0940450941988781,29.0999750546262,
-17.3523017088945));
#54091=CARTESIAN_POINT('Ctrl Pts',(0.0043183856975315,29.11051795413,-17.3520948932218));
#54092=CARTESIAN_POINT('Ctrl Pts',(-0.0846413778766092,29.1254494642378,
-17.3508590735705));
#54093=CARTESIAN_POINT('Ctrl Pts',(-0.172861973304381,29.1446114053705,
-17.3486408804781));
#54094=CARTESIAN_POINT('Ctrl Pts',(-0.185637033054331,29.147386210298,-17.348319668077));
#54095=CARTESIAN_POINT('Ctrl Pts',(-0.198396589790223,29.1502497370368,
-17.3479778528971));
#54096=CARTESIAN_POINT('Ctrl Pts',(-0.211140707083288,29.1532016314949,
-17.347615561321));
#54097=CARTESIAN_POINT('Ctrl Pts',(-0.296585498060996,29.1729930379266,
-17.3451865246695));
#54098=CARTESIAN_POINT('Ctrl Pts',(-0.381332734630402,29.1967542444877,
-17.3418385994444));
#54099=CARTESIAN_POINT('Ctrl Pts',(-0.465406902219237,29.2243801498567,
-17.3376101192265));
#54100=CARTESIAN_POINT('Ctrl Pts',(-0.480467616897809,29.2293289455502,
-17.3368526459632));
#54101=CARTESIAN_POINT('Ctrl Pts',(-0.495512841578221,29.2344040610324,
-17.3360665540002));
#54102=CARTESIAN_POINT('Ctrl Pts',(-0.510530623365413,29.2396007024458,
-17.3352527344234));
#54103=CARTESIAN_POINT('Ctrl Pts',(-0.519625874270915,29.2427479553617,
-17.334759859154));
#54104=CARTESIAN_POINT('Ctrl Pts',(-0.528715062171632,29.2459411878691,
-17.33425659577));
#54105=CARTESIAN_POINT('Ctrl Pts',(-0.537788620983005,29.2491769241415,
-17.333743521862));
#54106=CARTESIAN_POINT('Ctrl Pts',(-0.553369192460061,29.2547331365738,
-17.3328625020919));
#54107=CARTESIAN_POINT('Ctrl Pts',(-0.56887579523059,29.2604044022829,-17.3319542053377));
#54108=CARTESIAN_POINT('Ctrl Pts',(-0.584317019483223,29.2661908253089,
-17.3310189205406));
#54109=CARTESIAN_POINT('Ctrl Pts',(-0.592741616178843,29.269347847026,-17.3305086373479));
#54110=CARTESIAN_POINT('Ctrl Pts',(-0.601146149580129,29.2725389392175,
-17.3299903501898));
#54111=CARTESIAN_POINT('Ctrl Pts',(-0.609530854384228,29.2757637100109,
-17.3294641714673));
#54112=CARTESIAN_POINT('Ctrl Pts',(-0.625464084497629,29.2818916556352,
-17.3284642881247));
#54113=CARTESIAN_POINT('Ctrl Pts',(-0.641325740152662,29.2881411628421,
-17.3274359196832));
#54114=CARTESIAN_POINT('Ctrl Pts',(-0.657117305180762,29.2945097885707,
-17.3263797807976));
#54115=CARTESIAN_POINT('Ctrl Pts',(-0.688504756412231,29.3071681241512,
-17.3242805900141));
#54116=CARTESIAN_POINT('Ctrl Pts',(-0.719615331526967,29.3202969521538,
-17.3220717772427));
#54117=CARTESIAN_POINT('Ctrl Pts',(-0.750460137429674,29.3338774655774,
-17.3197586170282));
#54118=CARTESIAN_POINT('Ctrl Pts',(-0.766985401130791,29.3411532956225,
-17.3185193295239));
#54119=CARTESIAN_POINT('Ctrl Pts',(-0.783434470810792,29.3485585979443,
-17.317250129809));
#54120=CARTESIAN_POINT('Ctrl Pts',(-0.799808799112829,29.3560909668914,
-17.3159517170646));
#54121=CARTESIAN_POINT('Ctrl Pts',(-0.875661422642261,29.3909839979513,
-17.3099369351898));
#54122=CARTESIAN_POINT('Ctrl Pts',(-0.949912389395401,29.4286007159882,
-17.3032985351734));
#54123=CARTESIAN_POINT('Ctrl Pts',(-1.0227011139135,29.4687058692772,-17.2961057417184));
#54124=CARTESIAN_POINT('Ctrl Pts',(-1.03999534287283,29.4782346487416,-17.2943967707522));
#54125=CARTESIAN_POINT('Ctrl Pts',(-1.05720697183354,29.4879040019624,-17.2926564778399));
#54126=CARTESIAN_POINT('Ctrl Pts',(-1.07433751090772,29.497711457383,-17.290885634723));
#54127=CARTESIAN_POINT('Ctrl Pts',(-1.14527573158552,29.5383245072059,-17.2835525053174));
#54128=CARTESIAN_POINT('Ctrl Pts',(-1.21482462488908,29.5813034463345,-17.2756979414421));
#54129=CARTESIAN_POINT('Ctrl Pts',(-1.28308743240194,29.6264749237948,-17.2673765449636));
#54130=CARTESIAN_POINT('Ctrl Pts',(-1.30068964917242,29.6381228206082,-17.2652307934192));
#54131=CARTESIAN_POINT('Ctrl Pts',(-1.31820631057408,29.6499165781555,-17.2630539809597));
#54132=CARTESIAN_POINT('Ctrl Pts',(-1.33563885933988,29.6618538487408,-17.2608469041224));
#54133=CARTESIAN_POINT('Ctrl Pts',(-1.37815754441842,29.6909693301048,-17.255463755264));
#54134=CARTESIAN_POINT('Ctrl Pts',(-1.4201760084857,29.7209380445501,-17.2499011197985));
#54135=CARTESIAN_POINT('Ctrl Pts',(-1.46171476117621,29.7517257912023,-17.2441709839974));
#54136=CARTESIAN_POINT('Ctrl Pts',(-1.48248413752148,29.7671196645284,-17.2413059160968));
#54137=CARTESIAN_POINT('Ctrl Pts',(-1.50313358222067,29.7827183009981,-17.2383989778656));
#54138=CARTESIAN_POINT('Ctrl Pts',(-1.5236655210333,29.7985176702096,-17.2354514018751));
#54139=CARTESIAN_POINT('Ctrl Pts',(-1.52663299972461,29.8008011511755,-17.2350253890654));
#54140=CARTESIAN_POINT('Ctrl Pts',(-1.52959787132464,29.8030887060471,-17.2345985510579));
#54141=CARTESIAN_POINT('Ctrl Pts',(-1.53256022149386,29.8053803805644,-17.2341708817701));
#54142=CARTESIAN_POINT('Ctrl Pts',(-1.53984609864872,29.8110167361801,-17.2331190324899));
#54143=CARTESIAN_POINT('Ctrl Pts',(-1.54711863018462,29.8166796254338,-17.2320618519711));
#54144=CARTESIAN_POINT('Ctrl Pts',(-1.55437552343597,29.8223668935654,-17.2309997792847));
#54145=CARTESIAN_POINT('Ctrl Pts',(-1.56458298234939,29.830366536632,-17.2295058805964));
#54146=CARTESIAN_POINT('Ctrl Pts',(-1.57476243074193,29.8384167611187,-17.2280018638832));
#54147=CARTESIAN_POINT('Ctrl Pts',(-1.58489488875909,29.8465016671252,-17.2264907639462));
#54148=CARTESIAN_POINT('Ctrl Pts',(-1.58769371888662,29.8487349138331,-17.2260733615723));
#54149=CARTESIAN_POINT('Ctrl Pts',(-1.59048933583235,29.850971097859,-17.2256553663614));
#54150=CARTESIAN_POINT('Ctrl Pts',(-1.59328153837513,29.8532100410182,-17.2252368133482));
#54151=CARTESIAN_POINT('Ctrl Pts',(-1.61339119892336,29.8693350843224,-17.2222223618943));
#54152=CARTESIAN_POINT('Ctrl Pts',(-1.63333460185478,29.8856111808793,-17.2191774998543));
#54153=CARTESIAN_POINT('Ctrl Pts',(-1.65311698743174,29.9020332378137,-17.216103830654));
#54154=CARTESIAN_POINT('Ctrl Pts',(-1.69274299677892,29.9349281876693,-17.2099469774278));
#54155=CARTESIAN_POINT('Ctrl Pts',(-1.7317232430286,29.9684084814715,-17.2036746162589));
#54156=CARTESIAN_POINT('Ctrl Pts',(-1.77009588134444,30.0024371988237,-17.1972985702881));
#54157=CARTESIAN_POINT('Ctrl Pts',(-1.78694210817751,30.0173763720605,-17.1944993799943));
#54158=CARTESIAN_POINT('Ctrl Pts',(-1.80367137995709,30.0324210900912,-17.1916802447701));
#54159=CARTESIAN_POINT('Ctrl Pts',(-1.82028640118399,30.0475687611652,-17.188842026926));
#54160=CARTESIAN_POINT('Ctrl Pts',(-1.87958806677336,30.1016332195985,-17.1787119739361));
#54161=CARTESIAN_POINT('Ctrl Pts',(-1.93743845715215,30.1570108336236,-17.1683398926932));
#54162=CARTESIAN_POINT('Ctrl Pts',(-1.99396211476126,30.213591260895,-17.1577624007788));
#54163=CARTESIAN_POINT('Ctrl Pts',(-2.00985737737727,30.2295024879537,-17.154787858456));
#54164=CARTESIAN_POINT('Ctrl Pts',(-2.02564765372924,30.245508900131,-17.1517970533222));
#54165=CARTESIAN_POINT('Ctrl Pts',(-2.04133516140658,30.2616086006945,-17.1487906572123));
#54166=CARTESIAN_POINT('Ctrl Pts',(-2.09731775608623,30.3190621509747,-17.1380620023916));
#54167=CARTESIAN_POINT('Ctrl Pts',(-2.15199317849248,30.3777023875684,-17.1271371965694));
#54168=CARTESIAN_POINT('Ctrl Pts',(-2.20545904914118,30.4374432811992,-17.1160465937905));
#54169=CARTESIAN_POINT('Ctrl Pts',(-2.22025249087105,30.4539729555147,-17.1129779411347));
#54170=CARTESIAN_POINT('Ctrl Pts',(-2.23495328877808,30.4705869355724,-17.1098965827622));
#54171=CARTESIAN_POINT('Ctrl Pts',(-2.24956311487717,30.487283798179,-17.1068030622022));
#54172=CARTESIAN_POINT('Ctrl Pts',(-2.30276895690595,30.5480901779536,-17.095537126173));
#54173=CARTESIAN_POINT('Ctrl Pts',(-2.35476946268512,30.6099946764907,-17.0841119019788));
#54174=CARTESIAN_POINT('Ctrl Pts',(-2.40564340906758,30.6729284032563,-17.0725540010902));
#54175=CARTESIAN_POINT('Ctrl Pts',(-2.41922701910644,30.6897320377974,-17.0694679810406));
#54176=CARTESIAN_POINT('Ctrl Pts',(-2.43273028540881,30.7066090763658,-17.0663724934113));
#54177=CARTESIAN_POINT('Ctrl Pts',(-2.44615442796957,30.7235584904524,-17.063267977535));
#54178=CARTESIAN_POINT('Ctrl Pts',(-2.49700159070261,30.7877584654149,-17.0515088783408));
#54179=CARTESIAN_POINT('Ctrl Pts',(-2.54670382627324,30.8529820325238,-17.0396241050726));
#54180=CARTESIAN_POINT('Ctrl Pts',(-2.59535135150116,30.9192065689568,-17.0276321672655));
#54181=CARTESIAN_POINT('Ctrl Pts',(-2.60764898540964,30.9359475049242,-17.0246007188965));
#54182=CARTESIAN_POINT('Ctrl Pts',(-2.61988188181737,30.9527567274417,-17.0215616539119));
#54183=CARTESIAN_POINT('Ctrl Pts',(-2.63204242319319,30.969621047708,-17.0185175583762));
#54184=CARTESIAN_POINT('Ctrl Pts',(-2.64710886066503,30.9905152841523,-17.0147460424847));
#54185=CARTESIAN_POINT('Ctrl Pts',(-2.66205735353112,31.0114844768585,-17.0109685635766));
#54186=CARTESIAN_POINT('Ctrl Pts',(-2.67687815179317,31.03250984723,-17.0071889049466));
#54187=CARTESIAN_POINT('Ctrl Pts',(-2.68005872862648,31.0370219392735,-17.0063777816546));
#54188=CARTESIAN_POINT('Ctrl Pts',(-2.68323362145371,31.041536899362,-17.005566508625));
#54189=CARTESIAN_POINT('Ctrl Pts',(-2.68640262874064,31.0460543999021,-17.0047551487455));
#54190=CARTESIAN_POINT('Ctrl Pts',(-2.69800050813871,31.0625874721551,-17.0017857475485));
#54191=CARTESIAN_POINT('Ctrl Pts',(-2.70952411185291,31.07916060295,-16.9988140852021));
#54192=CARTESIAN_POINT('Ctrl Pts',(-2.72097236568739,31.0957696486511,-16.9958410668479));
#54193=CARTESIAN_POINT('Ctrl Pts',(-2.73902544468637,31.1219609279916,-16.9911528291488));
#54194=CARTESIAN_POINT('Ctrl Pts',(-2.75689333580946,31.1482446123294,-16.9864606814935));
#54195=CARTESIAN_POINT('Ctrl Pts',(-2.77458131746985,31.174618216052,-16.9817655560967));
#54196=CARTESIAN_POINT('Ctrl Pts',(-2.78545651842152,31.1908336467217,-16.9788788258205));
#54197=CARTESIAN_POINT('Ctrl Pts',(-2.79626404107529,31.2070828865657,-16.9759910156415));
#54198=CARTESIAN_POINT('Ctrl Pts',(-2.80700482713285,31.2233655128358,-16.9731023015609));
#54199=CARTESIAN_POINT('Ctrl Pts',(-2.863425124086,31.3088965535259,-16.9579281694845));
#54200=CARTESIAN_POINT('Ctrl Pts',(-2.91800594098433,31.3953483978114,-16.942731525384));
#54201=CARTESIAN_POINT('Ctrl Pts',(-2.970888038649,31.4826568738121,-16.9275498795692));
#54202=CARTESIAN_POINT('Ctrl Pts',(-3.01520349115017,31.5558217971419,-16.9148275872679));
#54203=CARTESIAN_POINT('Ctrl Pts',(-3.05832507044605,31.6295884628099,-16.9021146309357));
#54204=CARTESIAN_POINT('Ctrl Pts',(-3.10033004290332,31.7039199616385,-16.8894266815057));
#54205=CARTESIAN_POINT('Ctrl Pts',(-3.10845004786398,31.7182890256781,-16.8869739668321));
#54206=CARTESIAN_POINT('Ctrl Pts',(-3.11652825402692,31.732679235635,-16.884522173597));
#54207=CARTESIAN_POINT('Ctrl Pts',(-3.12456502627307,31.7470904300683,-16.8820713900921));
#54208=CARTESIAN_POINT('Ctrl Pts',(-3.17417620622964,31.8360510648259,-16.866942647137));
#54209=CARTESIAN_POINT('Ctrl Pts',(-3.22221018340241,31.9258110668167,-16.8518548517033));
#54210=CARTESIAN_POINT('Ctrl Pts',(-3.26875629613443,32.0163305079745,-16.83683855778));
#54211=CARTESIAN_POINT('Ctrl Pts',(-3.30936706167238,32.09530732442,-16.8237370729089));
#54212=CARTESIAN_POINT('Ctrl Pts',(-3.34884412638437,32.1748628249438,-16.8106877954571));
#54213=CARTESIAN_POINT('Ctrl Pts',(-3.38724441489668,32.2549704657586,-16.7977087994844));
#54214=CARTESIAN_POINT('Ctrl Pts',(-3.43686926623875,32.3584939006287,-16.7809359894178));
#54215=CARTESIAN_POINT('Ctrl Pts',(-3.48469413673384,32.4629403693864,-16.7642801974446));
#54216=CARTESIAN_POINT('Ctrl Pts',(-3.53079737027302,32.5682771939252,-16.7477759907028));
#54217=CARTESIAN_POINT('Ctrl Pts',(-3.56808998530252,32.6534834873756,-16.7344258418925));
#54218=CARTESIAN_POINT('Ctrl Pts',(-3.60425597317371,32.7392723139034,-16.7211747356865));
#54219=CARTESIAN_POINT('Ctrl Pts',(-3.63933555556943,32.8256258069973,-16.7080405816169));
#54220=CARTESIAN_POINT('Ctrl Pts',(-3.67862303088125,32.9223376403865,-16.6933309494459));
#54221=CARTESIAN_POINT('Ctrl Pts',(-3.71654441512108,33.0197596234453,-16.6787677314079));
#54222=CARTESIAN_POINT('Ctrl Pts',(-3.75313710541097,33.1178772474942,-16.6643748421233));
#54223=CARTESIAN_POINT('Ctrl Pts',(-3.75552008359739,33.1242668339378,-16.6634375527102));
#54224=CARTESIAN_POINT('Ctrl Pts',(-3.7578974238126,33.1306593722572,-16.6625009854662));
#54225=CARTESIAN_POINT('Ctrl Pts',(-3.76026913405428,33.1370548597423,-16.6615651469124));
#54226=CARTESIAN_POINT('Ctrl Pts',(-3.77612087232058,33.1798002136719,-16.6553103070276));
#54227=CARTESIAN_POINT('Ctrl Pts',(-3.79172111609674,33.2226772547136,-16.6490880829375));
#54228=CARTESIAN_POINT('Ctrl Pts',(-3.80707222536322,33.265685120324,-16.6429004381211));
#54229=CARTESIAN_POINT('Ctrl Pts',(-3.80898566072384,33.2710458254961,-16.6421291806057));
#54230=CARTESIAN_POINT('Ctrl Pts',(-3.81089522494559,33.2764085634821,-16.6413584603056));
#54231=CARTESIAN_POINT('Ctrl Pts',(-3.81280092196227,33.2817733329664,-16.6405882810111));
#54232=CARTESIAN_POINT('Ctrl Pts',(-3.81968664471756,33.3011574821736,-16.6378054456246));
#54233=CARTESIAN_POINT('Ctrl Pts',(-3.82652219626237,33.3205690601755,-16.6350295440705));
#54234=CARTESIAN_POINT('Ctrl Pts',(-3.83330686070246,33.3400054236625,-16.6322611252416));
#54235=CARTESIAN_POINT('Ctrl Pts',(-3.83499337862771,33.3448368749026,-16.6315729573859));
#54236=CARTESIAN_POINT('Ctrl Pts',(-3.83667686763365,33.3496701967109,-16.6308852041413));
#54237=CARTESIAN_POINT('Ctrl Pts',(-3.83835723509096,33.3545051076029,-16.6301979077439));
#54238=CARTESIAN_POINT('Ctrl Pts',(-3.8453096925068,33.3745093703251,-16.6273542446429));
#54239=CARTESIAN_POINT('Ctrl Pts',(-3.85221059805588,33.394546274598,-16.624517627869));
#54240=CARTESIAN_POINT('Ctrl Pts',(-3.85905346708592,33.4145963041088,-16.6216909852044));
#54241=CARTESIAN_POINT('Ctrl Pts',(-3.86051784694518,33.4188870276729,-16.6210860812425));
#54242=CARTESIAN_POINT('Ctrl Pts',(-3.86197953399095,33.4231782177245,-16.6204816524728));
#54243=CARTESIAN_POINT('Ctrl Pts',(-3.86343852387851,33.4274698499442,-16.6198777034043));
#54244=CARTESIAN_POINT('Ctrl Pts',(-3.89654521281925,33.5248534810153,-16.6061731848763));
#54245=CARTESIAN_POINT('Ctrl Pts',(-3.92827659709283,33.6225047869756,-16.5927095724306));
#54246=CARTESIAN_POINT('Ctrl Pts',(-3.9586750328472,33.7204187298343,-16.5795043418062));
#54247=CARTESIAN_POINT('Ctrl Pts',(-3.98912619588366,33.818502508277,-16.5662762061901));
#54248=CARTESIAN_POINT('Ctrl Pts',(-4.01823929067579,33.9168495280274,-16.5533063835685));
#54249=CARTESIAN_POINT('Ctrl Pts',(-4.04605562710238,34.0154538256492,-16.5406106331751));
#54250=CARTESIAN_POINT('Ctrl Pts',(-4.07377563355854,34.1137166495078,-16.527958849077));
#54251=CARTESIAN_POINT('Ctrl Pts',(-4.10020721787853,34.2122350952638,-16.5155791652252));
#54252=CARTESIAN_POINT('Ctrl Pts',(-4.12537067875558,34.3110072940172,-16.5034870911201));
#54253=CARTESIAN_POINT('Ctrl Pts',(-4.15177288597136,34.414641848556,-16.4907997486376));
#54254=CARTESIAN_POINT('Ctrl Pts',(-4.17677913217847,34.5185557899405,-16.4784293163084));
#54255=CARTESIAN_POINT('Ctrl Pts',(-4.2004125186538,34.622746628846,-16.466393709337));
#54256=CARTESIAN_POINT('Ctrl Pts',(-4.22190650430602,34.7175056427041,-16.4554476198365));
#54257=CARTESIAN_POINT('Ctrl Pts',(-4.24226468159238,34.8124937403118,-16.4447784266551));
#54258=CARTESIAN_POINT('Ctrl Pts',(-4.2614894046433,34.9077119948294,-16.4343999617148));
#54259=CARTESIAN_POINT('Ctrl Pts',(-4.28354054518552,35.0169292307288,-16.4224956555561));
#54260=CARTESIAN_POINT('Ctrl Pts',(-4.30410052030379,35.1264492980322,-16.410974115389));
#54261=CARTESIAN_POINT('Ctrl Pts',(-4.3231726349224,35.2362735924075,-16.3998563832951));
#54262=CARTESIAN_POINT('Ctrl Pts',(-4.33901061063775,35.327474518055,-16.3906239319161));
#54263=CARTESIAN_POINT('Ctrl Pts',(-4.35382253124448,35.4188852436833,-16.3816699084276));
#54264=CARTESIAN_POINT('Ctrl Pts',(-4.36759808576858,35.5105089644624,-16.3730069706139));
#54265=CARTESIAN_POINT('Ctrl Pts',(-4.38486272722525,35.6253392375675,-16.362149874803));
#54266=CARTESIAN_POINT('Ctrl Pts',(-4.40049956209613,35.7405040133384,-16.3517501661194));
#54267=CARTESIAN_POINT('Ctrl Pts',(-4.41448803991512,35.8560093809796,-16.3418329438277));
#54268=CARTESIAN_POINT('Ctrl Pts',(-4.42510172471939,35.9436484780428,-16.334308302984));
#54269=CARTESIAN_POINT('Ctrl Pts',(-4.43476662696607,36.0314836189183,-16.3270613908145));
#54270=CARTESIAN_POINT('Ctrl Pts',(-4.44346276114196,36.1195196258497,-16.320103932916));
#54271=CARTESIAN_POINT('Ctrl Pts',(-4.45536348826696,36.2399975847304,-16.3105825977734));
#54272=CARTESIAN_POINT('Ctrl Pts',(-4.46544989089848,36.3608515237431,-16.3016034223743));
#54273=CARTESIAN_POINT('Ctrl Pts',(-4.47367046250997,36.4820935950479,-16.2931966280678));
#54274=CARTESIAN_POINT('Ctrl Pts',(-4.47937382151229,36.5662102588901,-16.2873640694265));
#54275=CARTESIAN_POINT('Ctrl Pts',(-4.48417755850892,36.6505140455029,-16.2818071352268));
#54276=CARTESIAN_POINT('Ctrl Pts',(-4.4880564954921,36.7350105803116,-16.2765365518856));
#54277=CARTESIAN_POINT('Ctrl Pts',(-4.48901380998959,36.7558641693518,-16.2752357816322));
#54278=CARTESIAN_POINT('Ctrl Pts',(-4.4899147950835,36.7767294974198,-16.2739524535344));
#54279=CARTESIAN_POINT('Ctrl Pts',(-4.49075907137466,36.7976066463568,-16.2726867293248));
#54280=CARTESIAN_POINT('Ctrl Pts',(-4.49200271497388,36.828359295599,-16.2708222806506));
#54281=CARTESIAN_POINT('Ctrl Pts',(-4.49312325344046,36.8591376052184,-16.2689960335866));
#54282=CARTESIAN_POINT('Ctrl Pts',(-4.49411926046787,36.8899418787816,-16.267208522195));
#54283=CARTESIAN_POINT('Ctrl Pts',(-4.49483083024889,36.9119491433798,-16.2659314839267));
#54284=CARTESIAN_POINT('Ctrl Pts',(-4.49547886796317,36.9339707312023,-16.2646741560961));
#54285=CARTESIAN_POINT('Ctrl Pts',(-4.49606277160481,36.9560037243413,-16.2634368980414));
#54286=CARTESIAN_POINT('Ctrl Pts',(-4.49616494674342,36.959859196319,-16.2632203948306));
#54287=CARTESIAN_POINT('Ctrl Pts',(-4.49626515807568,36.9637152028417,-16.2630044973421));
#54288=CARTESIAN_POINT('Ctrl Pts',(-4.49636340186868,36.9675716494597,-16.2627892113485));
#54289=CARTESIAN_POINT('Ctrl Pts',(-4.4970230827126,36.9934666590264,-16.2613436233717));
#54290=CARTESIAN_POINT('Ctrl Pts',(-4.497594172852,37.0193857201734,-16.2599253456985));
#54291=CARTESIAN_POINT('Ctrl Pts',(-4.49807566203265,37.0453111639324,-16.2585356567974));
#54292=CARTESIAN_POINT('Ctrl Pts',(-4.49850557527374,37.0684595377707,-16.2572948279615));
#54293=CARTESIAN_POINT('Ctrl Pts',(-4.49886394922953,37.0916078702396,-16.2560770264095));
#54294=CARTESIAN_POINT('Ctrl Pts',(-4.49915002334757,37.1147399926744,-16.2548832910547));
#54295=CARTESIAN_POINT('Ctrl Pts',(-4.50014552494797,37.1952368410517,-16.2507292436199));
#54296=CARTESIAN_POINT('Ctrl Pts',(-4.50027046440707,37.2756130690668,-16.2468620241585));
#54297=CARTESIAN_POINT('Ctrl Pts',(-4.49951014118622,37.3558963157756,-16.2432842876556));
#54298=CARTESIAN_POINT('Ctrl Pts',(-4.4982747451551,37.4863429490343,-16.2374710738081));
#54299=CARTESIAN_POINT('Ctrl Pts',(-4.49470199172509,37.6165098660978,-16.232423759574));
#54300=CARTESIAN_POINT('Ctrl Pts',(-4.48872744871276,37.7463892347881,-16.2281599037842));
#54301=CARTESIAN_POINT('Ctrl Pts',(-4.48523462831247,37.8223189431529,-16.2256671804988));
#54302=CARTESIAN_POINT('Ctrl Pts',(-4.4809210796152,37.8981503907366,-16.2234422645953));
#54303=CARTESIAN_POINT('Ctrl Pts',(-4.47576652607971,37.9738810433624,-16.2214883404208));
#54304=CARTESIAN_POINT('Ctrl Pts',(-4.46671418296332,38.1068779842761,-16.2180568905526));
#54305=CARTESIAN_POINT('Ctrl Pts',(-4.45506810014391,38.2395642945037,-16.2154611869477));
#54306=CARTESIAN_POINT('Ctrl Pts',(-4.44071727209931,38.3719265373697,-16.213718742802));
#54307=CARTESIAN_POINT('Ctrl Pts',(-4.43291881054213,38.4438542240094,-16.2127718717474));
#54308=CARTESIAN_POINT('Ctrl Pts',(-4.42432191601837,38.5156862467986,-16.2120770179681));
#54309=CARTESIAN_POINT('Ctrl Pts',(-4.41490107380013,38.5874194528047,-16.2116365134872));
#54310=CARTESIAN_POINT('Ctrl Pts',(-4.39718579379342,38.7223090731529,-16.2108081735106));
#54311=CARTESIAN_POINT('Ctrl Pts',(-4.37655716797495,38.8568492198562,-16.2108791369079));
#54312=CARTESIAN_POINT('Ctrl Pts',(-4.35284372957258,38.9910192878985,-16.2118651687503));
#54313=CARTESIAN_POINT('Ctrl Pts',(-4.34074034128895,39.059499969696,-16.2123684414536));
#54314=CARTESIAN_POINT('Ctrl Pts',(-4.32783379023972,39.1278842987629,-16.2131101650123));
#54315=CARTESIAN_POINT('Ctrl Pts',(-4.31409242829866,39.1961684008776,-16.2140917574815));
#54316=CARTESIAN_POINT('Ctrl Pts',(-4.28670714269265,39.332252411093,-16.2160479820706));
#54317=CARTESIAN_POINT('Ctrl Pts',(-4.25600661265602,39.4679377608591,-16.2189567983645));
#54318=CARTESIAN_POINT('Ctrl Pts',(-4.22173771426279,39.603194020185,-16.2228296072566));
#54319=CARTESIAN_POINT('Ctrl Pts',(-4.20889439562926,39.6538854435208,-16.2242810609344));
#54320=CARTESIAN_POINT('Ctrl Pts',(-4.19554849436218,39.7045164220435,-16.2258678031695));
#54321=CARTESIAN_POINT('Ctrl Pts',(-4.18168367496839,39.7550849695418,-16.2275901874348));
#54322=CARTESIAN_POINT('Ctrl Pts',(-4.17761044096032,39.7699410972387,-16.2280961928839));
#54323=CARTESIAN_POINT('Ctrl Pts',(-4.17349241277035,39.7847918356752,-16.2286139046665));
#54324=CARTESIAN_POINT('Ctrl Pts',(-4.16932914922853,39.7996371310629,-16.2291433294851));
#54325=CARTESIAN_POINT('Ctrl Pts',(-4.1664106053186,39.8100440260407,-16.2295144685121));
#54326=CARTESIAN_POINT('Ctrl Pts',(-4.16346987059635,39.820448111608,-16.2298913542028));
#54327=CARTESIAN_POINT('Ctrl Pts',(-4.16050671816335,39.8308496295917,-16.230274002705));
#54328=CARTESIAN_POINT('Ctrl Pts',(-4.15634426034634,39.8454610546936,-16.2308115242418));
#54329=CARTESIAN_POINT('Ctrl Pts',(-4.15213657764192,39.8600706185222,-16.231360554189));
#54330=CARTESIAN_POINT('Ctrl Pts',(-4.1478866429035,39.8746669388683,-16.2319206454273));
#54331=CARTESIAN_POINT('Ctrl Pts',(-4.14479843005341,39.8852733473971,-16.232327635432));
#54332=CARTESIAN_POINT('Ctrl Pts',(-4.14168818815604,39.8958718046634,-16.2327404230012));
#54333=CARTESIAN_POINT('Ctrl Pts',(-4.13855697960968,39.9064582319492,-16.2331588413834));
#54334=CARTESIAN_POINT('Ctrl Pts',(-4.13431153697064,39.920811817515,-16.2337261530824));
#54335=CARTESIAN_POINT('Ctrl Pts',(-4.13002657740077,39.9351468985181,-16.2343039441294));
#54336=CARTESIAN_POINT('Ctrl Pts',(-4.1257014773501,39.9494648091859,-16.2348922103134));
#54337=CARTESIAN_POINT('Ctrl Pts',(-4.11067135817129,39.9992208613485,-16.2369364892322));
#54338=CARTESIAN_POINT('Ctrl Pts',(-4.09515994998905,40.0487579808328,-16.2391068321293));
#54339=CARTESIAN_POINT('Ctrl Pts',(-4.07915897210243,40.0980728016392,-16.2414006596024));
#54340=CARTESIAN_POINT('Ctrl Pts',(-4.06752785387619,40.1339197676915,-16.2430680438534));
#54341=CARTESIAN_POINT('Ctrl Pts',(-4.05563806503628,40.1696492375032,-16.244800674657));
#54342=CARTESIAN_POINT('Ctrl Pts',(-4.04348641224067,40.2052599000481,-16.2465975564644));
#54343=CARTESIAN_POINT('Ctrl Pts',(-4.02220390610394,40.2676287116735,-16.2497446302605));
#54344=CARTESIAN_POINT('Ctrl Pts',(-4.00011953136804,40.3296336871105,-16.2530891515926));
#54345=CARTESIAN_POINT('Ctrl Pts',(-3.97721133125741,40.391265705422,-16.2566245299766));
#54346=CARTESIAN_POINT('Ctrl Pts',(-3.9278482247377,40.5240717692003,-16.2642426430939));
#54347=CARTESIAN_POINT('Ctrl Pts',(-3.87466018715068,40.6551461600849,-16.2727469451434));
#54348=CARTESIAN_POINT('Ctrl Pts',(-3.81742461158264,40.7843965617411,-16.2820708005939));
#54349=CARTESIAN_POINT('Ctrl Pts',(-3.79120522380902,40.843605652718,-16.2863420214068));
#54350=CARTESIAN_POINT('Ctrl Pts',(-3.7641369473265,40.9024321914955,-16.2907853454144));
#54351=CARTESIAN_POINT('Ctrl Pts',(-3.73619027274348,40.9608637952424,-16.29539225053));
#54352=CARTESIAN_POINT('Ctrl Pts',(-3.69171385851549,41.0538561906178,-16.3027240216006));
#54353=CARTESIAN_POINT('Ctrl Pts',(-3.64501276311427,41.1458483760823,-16.3104700046038));
#54354=CARTESIAN_POINT('Ctrl Pts',(-3.5959667510252,41.236790012973,-16.3185954496022));
#54355=CARTESIAN_POINT('Ctrl Pts',(-3.57775919507526,41.2705506567305,-16.3216118924918));
#54356=CARTESIAN_POINT('Ctrl Pts',(-3.5592284199418,41.3041665597948,-16.3246806590239));
#54357=CARTESIAN_POINT('Ctrl Pts',(-3.54036821085535,41.3376351406411,-16.3277999436471));
#54358=CARTESIAN_POINT('Ctrl Pts',(-3.51504025644013,41.3825811264534,-16.331988926833));
#54359=CARTESIAN_POINT('Ctrl Pts',(-3.4891166942094,41.4272607781668,-16.3362686376718));
#54360=CARTESIAN_POINT('Ctrl Pts',(-3.46257912027332,41.471666391437,-16.3406338568241));
#54361=CARTESIAN_POINT('Ctrl Pts',(-3.45564724394915,41.4832655760509,-16.3417740951656));
#54362=CARTESIAN_POINT('Ctrl Pts',(-3.44867346629616,41.4948460598394,-16.3429201660408));
#54363=CARTESIAN_POINT('Ctrl Pts',(-3.44165743709138,41.5064076958658,-16.3440719709585));
#54364=CARTESIAN_POINT('Ctrl Pts',(-3.43525505324746,41.5169581125679,-16.3451230351689));
#54365=CARTESIAN_POINT('Ctrl Pts',(-3.42881677312205,41.5274940047084,-16.3461789887384));
#54366=CARTESIAN_POINT('Ctrl Pts',(-3.42234310591756,41.5380139649604,-16.3472396330566));
#54367=CARTESIAN_POINT('Ctrl Pts',(-3.41519765756377,41.5496255956313,-16.3484103418617));
#54368=CARTESIAN_POINT('Ctrl Pts',(-3.40801236578587,41.5612124098009,-16.3495862278856));
#54369=CARTESIAN_POINT('Ctrl Pts',(-3.40079121408887,41.5727677646131,-16.3507664882365));
#54370=CARTESIAN_POINT('Ctrl Pts',(-3.39430786372305,41.5831424828011,-16.3518261587292));
#54371=CARTESIAN_POINT('Ctrl Pts',(-3.38779445712395,41.593493696068,-16.3528895361063));
#54372=CARTESIAN_POINT('Ctrl Pts',(-3.38125307744712,41.6038178373831,-16.3539561696315));
#54373=CARTESIAN_POINT('Ctrl Pts',(-3.37390786261472,41.6154106571957,-16.3551538760448));
#54374=CARTESIAN_POINT('Ctrl Pts',(-3.36652564355628,41.6269722107526,-16.356355978957));
#54375=CARTESIAN_POINT('Ctrl Pts',(-3.35910628076637,41.638502435275,-16.357562339157));
#54376=CARTESIAN_POINT('Ctrl Pts',(-3.33105272891493,41.6820996767975,-16.3621237400994));
#54377=CARTESIAN_POINT('Ctrl Pts',(-3.30247105915328,41.7252445352261,-16.3667454697368));
#54378=CARTESIAN_POINT('Ctrl Pts',(-3.27335493473435,41.7679327857555,-16.3714194616471));
#54379=CARTESIAN_POINT('Ctrl Pts',(-3.25227576109997,41.7988377589625,-16.3748032872424));
#54380=CARTESIAN_POINT('Ctrl Pts',(-3.23091649151266,41.829503356823,-16.3782145096199));
#54381=CARTESIAN_POINT('Ctrl Pts',(-3.20927471543407,41.8599279650246,-16.3816500603677));
#54382=CARTESIAN_POINT('Ctrl Pts',(-3.17113002588739,41.9135528260441,-16.387705386706));
#54383=CARTESIAN_POINT('Ctrl Pts',(-3.13210933033934,41.9664304210326,-16.3938367176048));
#54384=CARTESIAN_POINT('Ctrl Pts',(-3.09219386076608,42.0185471540337,-16.4000257673312));
#54385=CARTESIAN_POINT('Ctrl Pts',(-3.0296319451254,42.1002328435254,-16.4097262371245));
#54386=CARTESIAN_POINT('Ctrl Pts',(-2.96487183583847,42.1800495345858,-16.4195685651031));
#54387=CARTESIAN_POINT('Ctrl Pts',(-2.89784096682193,42.2579443794122,-16.4294813804493));
#54388=CARTESIAN_POINT('Ctrl Pts',(-2.87481981995416,42.2846966607014,-16.4328858473958));
#54389=CARTESIAN_POINT('Ctrl Pts',(-2.85153079730427,42.3112222445507,-16.4362986700301));
#54390=CARTESIAN_POINT('Ctrl Pts',(-2.82797091137712,42.3375190282482,-16.4397169174014));
#54391=CARTESIAN_POINT('Ctrl Pts',(-2.78293127718922,42.3877908131675,-16.4462516099563));
#54392=CARTESIAN_POINT('Ctrl Pts',(-2.7369026014617,42.4372271471467,-16.4528063924184));
#54393=CARTESIAN_POINT('Ctrl Pts',(-2.68985294718769,42.4858039179662,-16.4593577681913));
#54394=CARTESIAN_POINT('Ctrl Pts',(-2.61819198095264,42.5597908236559,-16.4693361181984));
#54395=CARTESIAN_POINT('Ctrl Pts',(-2.54416287898252,42.6317832884634,-16.4793067723326));
#54396=CARTESIAN_POINT('Ctrl Pts',(-2.46765134397022,42.7016952483703,-16.4891862846922));
#54397=CARTESIAN_POINT('Ctrl Pts',(-2.44852346021716,42.719173238347,-16.4916561627821));
#54398=CARTESIAN_POINT('Ctrl Pts',(-2.42924039812022,42.7365212099537,-16.4941203413884));
#54399=CARTESIAN_POINT('Ctrl Pts',(-2.40980030866471,42.7537378771226,-16.4965774832717));
#54400=CARTESIAN_POINT('Ctrl Pts',(-2.40468220997069,42.7582706032685,-16.4972243884566));
#54401=CARTESIAN_POINT('Ctrl Pts',(-2.3995528142902,42.7627945886819,-16.4978708622516));
#54402=CARTESIAN_POINT('Ctrl Pts',(-2.39441238378145,42.7673095437809,-16.498516841502));
#54403=CARTESIAN_POINT('Ctrl Pts',(-2.38002790183651,42.7799437560311,-16.5003244871552));
#54404=CARTESIAN_POINT('Ctrl Pts',(-2.36555579501941,42.7925074952912,-16.5021282682303));
#54405=CARTESIAN_POINT('Ctrl Pts',(-2.35102884419466,42.8049721064802,-16.5039235120036));
#54406=CARTESIAN_POINT('Ctrl Pts',(-2.34615879630707,42.8091507709586,-16.504525353591));
#54407=CARTESIAN_POINT('Ctrl Pts',(-2.34128179329844,42.8133189729222,-16.5051263396681));
#54408=CARTESIAN_POINT('Ctrl Pts',(-2.33639885646367,42.8174758102531,-16.5057263203709));
#54409=CARTESIAN_POINT('Ctrl Pts',(-2.31696011386605,42.8340239847697,-16.5081148154179));
#54410=CARTESIAN_POINT('Ctrl Pts',(-2.29741214406742,42.8504055250415,-16.5104892997636));
#54411=CARTESIAN_POINT('Ctrl Pts',(-2.27775717372585,42.8666186333273,-16.5128481934888));
#54412=CARTESIAN_POINT('Ctrl Pts',(-2.26236860104002,42.8793124502593,-16.5146950549654));
#54413=CARTESIAN_POINT('Ctrl Pts',(-2.24691444825131,42.8919030377098,-16.5165323596086));
#54414=CARTESIAN_POINT('Ctrl Pts',(-2.2313957874581,42.9043895385496,-16.5183593566189));
#54415=CARTESIAN_POINT('Ctrl Pts',(-2.2073019676343,42.9237757153255,-16.5211958988547));
#54416=CARTESIAN_POINT('Ctrl Pts',(-2.18305057305376,42.9429126314443,-16.5240078954214));
#54417=CARTESIAN_POINT('Ctrl Pts',(-2.15864142271283,42.961800356319,-16.5267930988146));
#54418=CARTESIAN_POINT('Ctrl Pts',(-2.10135766986817,43.0061263467124,-16.5333294550816));
#54419=CARTESIAN_POINT('Ctrl Pts',(-2.04320552379719,43.0490806846287,-16.5397182747111));
#54420=CARTESIAN_POINT('Ctrl Pts',(-1.98417891498175,43.0906578349874,-16.5459303792842));
#54421=CARTESIAN_POINT('Ctrl Pts',(-1.9606171900974,43.1072542378282,-16.5484100727959));
#54422=CARTESIAN_POINT('Ctrl Pts',(-1.93691615197933,43.123631187596,-16.550861606755));
#54423=CARTESIAN_POINT('Ctrl Pts',(-1.91307539225617,43.1397883575922,-16.5532831180631));
#54424=CARTESIAN_POINT('Ctrl Pts',(-1.85174084432199,43.1813555194244,-16.5595128818426));
#54425=CARTESIAN_POINT('Ctrl Pts',(-1.78948388159612,43.221472033667,-16.5655442738707));
#54426=CARTESIAN_POINT('Ctrl Pts',(-1.72628822892224,43.2601164045817,-16.5713446579823));
#54427=CARTESIAN_POINT('Ctrl Pts',(-1.63852840447744,43.3137818556649,-16.5793996533785));
#54428=CARTESIAN_POINT('Ctrl Pts',(-1.54895857244756,43.3646081409297,-16.5870091768287));
#54429=CARTESIAN_POINT('Ctrl Pts',(-1.45753509356855,43.4125380051629,-16.5940846193997));
#54430=CARTESIAN_POINT('Ctrl Pts',(-1.43588830470891,43.4238865959609,-16.5957599069002));
#54431=CARTESIAN_POINT('Ctrl Pts',(-1.41413751963647,43.4350727363855,-16.5974053637665));
#54432=CARTESIAN_POINT('Ctrl Pts',(-1.39228215387348,43.4460956894796,-16.5990197793473));
#54433=CARTESIAN_POINT('Ctrl Pts',(-1.32183313291274,43.4816272958594,-16.6042237186599));
#54434=CARTESIAN_POINT('Ctrl Pts',(-1.25029501345785,43.5154590902996,-16.6091048720554));
#54435=CARTESIAN_POINT('Ctrl Pts',(-1.17763414652208,43.5475427918415,-16.6136202138518));
#54436=CARTESIAN_POINT('Ctrl Pts',(-1.15739410693042,43.5564798637048,-16.6148779843765));
#54437=CARTESIAN_POINT('Ctrl Pts',(-1.13706740551599,43.5652810566249,-16.6161073852453));
#54438=CARTESIAN_POINT('Ctrl Pts',(-1.11665204632759,43.5739458510516,-16.6173075683168));
#54439=CARTESIAN_POINT('Ctrl Pts',(-1.11306064109996,43.5754701342011,-16.6175187007155));
#54440=CARTESIAN_POINT('Ctrl Pts',(-1.10946637251239,43.5769902275687,-16.6177289324325));
#54441=CARTESIAN_POINT('Ctrl Pts',(-1.10586955611941,43.5785059994041,-16.6179382417103));
#54442=CARTESIAN_POINT('Ctrl Pts',(-1.09384808843183,43.5835720912337,-16.6186378061155));
#54443=CARTESIAN_POINT('Ctrl Pts',(-1.0817936254975,43.5885917864702,-16.6193273211788));
#54444=CARTESIAN_POINT('Ctrl Pts',(-1.06972876207832,43.5935556457637,-16.6200053966719));
#54445=CARTESIAN_POINT('Ctrl Pts',(-1.06188552091578,43.5967825986254,-16.6204462064377));
#54446=CARTESIAN_POINT('Ctrl Pts',(-1.05403471295521,43.5999873202319,-16.6208823173579));
#54447=CARTESIAN_POINT('Ctrl Pts',(-1.04617933152838,43.6031685148794,-16.6213135432057));
#54448=CARTESIAN_POINT('Ctrl Pts',(-1.04195117477803,43.6048807919659,-16.6215456503919));
#54449=CARTESIAN_POINT('Ctrl Pts',(-1.03772102067868,43.6065865438,-16.6217763829208));
#54450=CARTESIAN_POINT('Ctrl Pts',(-1.03348881978403,43.6082857884376,-16.6220057425198));
#54451=CARTESIAN_POINT('Ctrl Pts',(-1.01416402109236,43.6160447680716,-16.623053029307));
#54452=CARTESIAN_POINT('Ctrl Pts',(-0.994800665078688,43.6236663683118,
-16.6240715200906));
#54453=CARTESIAN_POINT('Ctrl Pts',(-0.975398838645345,43.6311509959951,
-16.6250607039036));
#54454=CARTESIAN_POINT('Ctrl Pts',(-0.946227439814781,43.6424044241195,
-16.6265479801467));
#54455=CARTESIAN_POINT('Ctrl Pts',(-0.916969087203641,43.6533482686037,
-16.6279690016024));
#54456=CARTESIAN_POINT('Ctrl Pts',(-0.887623971798692,43.6639834687485,
-16.6293220547001));
#54457=CARTESIAN_POINT('Ctrl Pts',(-0.869449089231215,43.6705703746455,
-16.6301600674602));
#54458=CARTESIAN_POINT('Ctrl Pts',(-0.851240929339034,43.6770388362738,
-16.6309720567335));
#54459=CARTESIAN_POINT('Ctrl Pts',(-0.832999523055785,43.6833890388058,
-16.6317576612342));
#54460=CARTESIAN_POINT('Ctrl Pts',(-0.753158275762128,43.7111833920948,
-16.6351961923561));
#54461=CARTESIAN_POINT('Ctrl Pts',(-0.672680496364904,43.7367139705469,
-16.6381292382759));
#54462=CARTESIAN_POINT('Ctrl Pts',(-0.591564904416325,43.759978410422,-16.6405269912691));
#54463=CARTESIAN_POINT('Ctrl Pts',(-0.576024848681799,43.7644353919173,
-16.6409863507369));
#54464=CARTESIAN_POINT('Ctrl Pts',(-0.560461385298049,43.7688091891839,
-16.6414260739135));
#54465=CARTESIAN_POINT('Ctrl Pts',(-0.54487449675861,43.7730997914147,-16.6418459474937));
#54466=CARTESIAN_POINT('Ctrl Pts',(-0.460512928369039,43.7963219972201,
-16.6441184468226));
#54467=CARTESIAN_POINT('Ctrl Pts',(-0.375465187199559,43.8171072363759,
-16.6458095771723));
#54468=CARTESIAN_POINT('Ctrl Pts',(-0.289722449806869,43.8354260792837,
-16.6468857729884));
#54469=CARTESIAN_POINT('Ctrl Pts',(-0.277274221907169,43.8380856296819,
-16.6470420163181));
#54470=CARTESIAN_POINT('Ctrl Pts',(-0.264811340139473,43.8406931831398,
-16.6471853089574));
#54471=CARTESIAN_POINT('Ctrl Pts',(-0.252333773908635,43.8432486511893,
-16.6473155453024));
#54472=CARTESIAN_POINT('Ctrl Pts',(-0.213899223809915,43.8511202395231,
-16.6477167113019));
#54473=CARTESIAN_POINT('Ctrl Pts',(-0.175325354404486,43.8584976721331,
-16.6479940080683));
#54474=CARTESIAN_POINT('Ctrl Pts',(-0.136610688709363,43.8653757031155,
-16.6481443294018));
#54475=CARTESIAN_POINT('Ctrl Pts',(-0.0917379150289355,43.8733477809341,
-16.6483185614416));
#54476=CARTESIAN_POINT('Ctrl Pts',(-0.0466760171364662,43.8806488794434,
-16.6483222800481));
#54477=CARTESIAN_POINT('Ctrl Pts',(-0.00142252104673145,43.8872706258809,
-16.6481507404151));
#54478=CARTESIAN_POINT('Ctrl Pts',(0.00504226410894038,43.8882165896577,
-16.6481262347533));
#54479=CARTESIAN_POINT('Ctrl Pts',(0.0115023831731756,43.8891474722818,
-16.6480981942689));
#54480=CARTESIAN_POINT('Ctrl Pts',(0.017983572713365,43.8900669127708,-16.6480664654997));
#54481=CARTESIAN_POINT('Ctrl Pts',(0.0268684009855446,43.8913273404748,
-16.6480229696778));
#54482=CARTESIAN_POINT('Ctrl Pts',(0.0357560300500095,43.892560944674,-16.6479727334698));
#54483=CARTESIAN_POINT('Ctrl Pts',(0.0446464265659024,43.8937677392893,
-16.6479157416917));
#54484=CARTESIAN_POINT('Ctrl Pts',(0.0946198190147424,43.9005511961139,
-16.6475953878708));
#54485=CARTESIAN_POINT('Ctrl Pts',(0.144680824104186,43.9064867836914,-16.647061551913));
#54486=CARTESIAN_POINT('Ctrl Pts',(0.194824381188862,43.9115730116413,-16.6463116348634));
#54487=CARTESIAN_POINT('Ctrl Pts',(0.219976230483605,43.9141242474592,-16.6459354788483));
#54488=CARTESIAN_POINT('Ctrl Pts',(0.245148857175417,43.9164617506663,-16.6455049604648));
#54489=CARTESIAN_POINT('Ctrl Pts',(0.270341668442436,43.9185851214958,-16.6450197727132));
#54490=CARTESIAN_POINT('Ctrl Pts',(0.282958869797485,43.9196485596735,-16.644776778333));
#54491=CARTESIAN_POINT('Ctrl Pts',(0.29558113442138,43.920658285667,-16.6445200715934));
#54492=CARTESIAN_POINT('Ctrl Pts',(0.308208390846211,43.92161423551,-16.6442496152386));
#54493=CARTESIAN_POINT('Ctrl Pts',(0.315530705182528,43.9221685732857,-16.6440927825603));
#54494=CARTESIAN_POINT('Ctrl Pts',(0.322859901802196,43.9227051771392,-16.6439312040685));
#54495=CARTESIAN_POINT('Ctrl Pts',(0.330186921934994,43.9232234261787,-16.6437650852288));
#54496=CARTESIAN_POINT('Ctrl Pts',(0.335506964409879,43.9235997192492,-16.6436444687617));
#54497=CARTESIAN_POINT('Ctrl Pts',(0.340827324348622,43.9239664363589,-16.6435214329505));
#54498=CARTESIAN_POINT('Ctrl Pts',(0.346147593727981,43.9243235322772,-16.6433959637249));
#54499=CARTESIAN_POINT('Origin',(4.5,24.,-35.));
#54500=CARTESIAN_POINT('',(5.56574965699116,22.3076118445749,-37.));
#54501=CARTESIAN_POINT('',(6.5,24.,-37.));
#54502=CARTESIAN_POINT('Origin',(4.5,24.,-37.));
#54503=CARTESIAN_POINT('',(3.43425034300884,22.3076118445749,-37.));
#54504=CARTESIAN_POINT('Origin',(4.5,23.9999999999985,-38.6923881554236));
#54505=CARTESIAN_POINT('Origin',(4.5,24.,-37.));
#54506=CARTESIAN_POINT('',(6.5,24.,-35.));
#54507=CARTESIAN_POINT('',(6.5,24.,-35.));
#54508=CARTESIAN_POINT('Origin',(4.5,24.,-35.));
#54509=CARTESIAN_POINT('Origin',(-31.5,50.9282032302755,96.1658609549528));
#54510=CARTESIAN_POINT('',(-29.2705,50.9282032302755,-24.5));
#54511=CARTESIAN_POINT('Origin',(-31.5,50.9282032302755,-24.5));
#54512=CARTESIAN_POINT('',(-29.2705,50.9282032302755,-17.));
#54513=CARTESIAN_POINT('',(-29.2705,50.9282032302755,96.1658609549528));
#54514=CARTESIAN_POINT('Origin',(-31.5,50.9282032302755,-17.));
#54515=CARTESIAN_POINT('Origin',(3.49012810839377E-15,57.,-2.60208521396521E-14));
#54516=CARTESIAN_POINT('',(2.14313189850786E-15,-8.88178419700125E-15,17.5));
#54517=CARTESIAN_POINT('Origin',(-1.54074395550979E-30,-1.38777878078145E-14,
5.20417042793043E-15));
#54518=CARTESIAN_POINT('',(2.84458618865033E-15,11.4559962546824,17.5));
#54519=CARTESIAN_POINT('',(5.63326000690164E-15,57.,17.5));
#54520=CARTESIAN_POINT('Origin',(7.01454290142472E-16,11.4559962546824,
-1.07150924902746E-15));
#54521=CARTESIAN_POINT('Origin',(-49.5,46.2097438724404,-22.5588698729115));
#54522=CARTESIAN_POINT('',(-49.8535533905933,46.3993237581462,-22.2604415449401));
#54523=CARTESIAN_POINT('',(-50.,46.2097438724404,-22.5588698729115));
#54524=CARTESIAN_POINT('Origin',(-49.5,46.2097438724404,-22.5588698729115));
#54525=CARTESIAN_POINT('',(-49.5,45.787702483627,-22.2907634273934));
#54526=CARTESIAN_POINT('Origin',(-49.5,46.2097438724404,-22.5588698729115));
#54527=CARTESIAN_POINT('Origin',(-49.5,46.2097438724404,-22.5588698729115));
#54528=CARTESIAN_POINT('Origin',(-50.,41.3460650567048,-35.8098521656684));
#54529=CARTESIAN_POINT('',(-6.5,41.7681064455182,-36.0779586111866));
#54530=CARTESIAN_POINT('',(-6.5,41.0779586111866,-36.2318935544818));
#54531=CARTESIAN_POINT('Origin',(-6.5,41.3460650567048,-35.8098521656684));
#54532=CARTESIAN_POINT('',(-45.2928932188134,41.0779586111866,-36.2318935544818));
#54533=CARTESIAN_POINT('',(-50.,41.0779586111866,-36.2318935544818));
#54534=CARTESIAN_POINT('',(-45.2928932188134,41.7681064455182,-36.0779586111866));
#54535=CARTESIAN_POINT('Origin',(-45.2928932188134,41.3460650567048,-35.8098521656684));
#54536=CARTESIAN_POINT('',(-50.,41.7681064455182,-36.0779586111866));
#54537=CARTESIAN_POINT('Origin',(-47.3964466094067,42.4740175017242,-34.0342789768499));
#54538=CARTESIAN_POINT('',(-45.6464466094067,41.156485170999,-36.1082804936397));
#54539=CARTESIAN_POINT('Origin',(-45.2928932188135,41.3460650567048,-35.8098521656684));
#54540=CARTESIAN_POINT('',(-49.8535533905933,43.412390061038,-32.5571341160028));
#54541=CARTESIAN_POINT('',(-45.5,41.0779586111866,-36.2318935544818));
#54542=CARTESIAN_POINT('',(-49.5,44.0240113355571,-32.5268122335495));
#54543=CARTESIAN_POINT('Origin',(-49.5,43.6019699467437,-32.2587057880314));
#54544=CARTESIAN_POINT('',(-49.6464466094067,44.1025378953696,-32.4031991727075));
#54545=CARTESIAN_POINT('Origin',(-49.5,43.6019699467437,-32.2587057880314));
#54546=CARTESIAN_POINT('',(-50.,43.6019699467437,-32.2587057880314));
#54547=CARTESIAN_POINT('Origin',(-49.5,43.6019699467437,-32.2587057880314));
#54548=CARTESIAN_POINT('Origin',(-49.5,43.6019699467437,-32.2587057880314));
#54549=CARTESIAN_POINT('Origin',(-45.2221315177632,42.835413406597,-27.8705926603572));
#54550=CARTESIAN_POINT('',(-49.5,42.4133720177836,-27.602486214839));
#54551=CARTESIAN_POINT('',(-50.,43.1035198521152,-27.4485512715437));
#54552=CARTESIAN_POINT('Origin',(-49.5000000000041,42.8354134065986,-27.8705926603528));
#54553=CARTESIAN_POINT('',(-50.,42.4133720177836,-27.602486214839));
#54554=CARTESIAN_POINT('',(-45.2221315177632,43.1035198521152,-27.4485512715437));
#54555=CARTESIAN_POINT('Origin',(-6.5,41.3460650567048,-35.8098521656684));
#54556=CARTESIAN_POINT('',(-6.,41.3460650567048,-35.8098521656684));
#54557=CARTESIAN_POINT('Origin',(-6.5,41.3460650567048,-35.8098521656684));
#54558=CARTESIAN_POINT('Origin',(-6.5,41.3460650567048,-35.8098521656684));
#54559=CARTESIAN_POINT('Origin',(-27.5,24.,-29.5));
#54560=CARTESIAN_POINT('',(-17.5,27.3235,-29.5));
#54561=CARTESIAN_POINT('Origin',(-17.5,24.,-29.5));
#54562=CARTESIAN_POINT('',(-27.5,27.3235,-29.5));
#54563=CARTESIAN_POINT('',(-27.5,27.3235,-29.5));
#54564=CARTESIAN_POINT('Origin',(-27.5,24.,-29.5));
#54565=CARTESIAN_POINT('Origin',(-29.,21.,1.));
#54566=CARTESIAN_POINT('',(-16.9705627484772,21.5,1.));
#54567=CARTESIAN_POINT('',(-17.0000000870233,21.0000000000022,0.499999252982979));
#54568=CARTESIAN_POINT('Ctrl Pts',(-16.9705627484772,21.5,1.));
#54569=CARTESIAN_POINT('Ctrl Pts',(-16.9730813739591,21.5,0.97862875046525));
#54570=CARTESIAN_POINT('Ctrl Pts',(-16.9754128387929,21.49863561053,0.957471138975276));
#54571=CARTESIAN_POINT('Ctrl Pts',(-16.977567566868,21.4959539436567,0.936520192097311));
#54572=CARTESIAN_POINT('Ctrl Pts',(-16.9797222949432,21.4932722767835,0.915569245219347));
#54573=CARTESIAN_POINT('Ctrl Pts',(-16.9817002334104,21.4892732994039,0.894824944327382));
#54574=CARTESIAN_POINT('Ctrl Pts',(-16.9835103667152,21.4839393536879,0.874291199214557));
#54575=CARTESIAN_POINT('Ctrl Pts',(-16.9844154333676,21.4812723808299,0.864024326658143));
#54576=CARTESIAN_POINT('Ctrl Pts',(-16.9852785330442,21.4782708106201,0.853810226313161));
#54577=CARTESIAN_POINT('Ctrl Pts',(-16.9861007130495,21.4749261233953,0.843650463575198));
#54578=CARTESIAN_POINT('Ctrl Pts',(-16.9865118030522,21.4732537797829,0.838570582206216));
#54579=CARTESIAN_POINT('Ctrl Pts',(-16.9869133178517,21.4714922243147,0.833495564598339));
#54580=CARTESIAN_POINT('Ctrl Pts',(-16.987302317957,21.4696553181118,0.828466093560954));
#54581=CARTESIAN_POINT('Ctrl Pts',(-16.9876913180624,21.4678184119089,0.82343662252357));
#54582=CARTESIAN_POINT('Ctrl Pts',(-16.9880681393362,21.4659051003747,0.818448723733261));
#54583=CARTESIAN_POINT('Ctrl Pts',(-16.9884333019219,21.4639163929689,0.813501795185541));
#54584=CARTESIAN_POINT('Ctrl Pts',(-16.989893952265,21.4559615633459,0.793714080994655));
#54585=CARTESIAN_POINT('Ctrl Pts',(-16.9911680656929,21.4468050031027,0.774580106115942));
#54586=CARTESIAN_POINT('Ctrl Pts',(-16.9922828276023,21.4364710184893,0.756088025810979));
#54587=CARTESIAN_POINT('Ctrl Pts',(-16.9933975895117,21.4261370338759,0.737595945506016));
#54588=CARTESIAN_POINT('Ctrl Pts',(-16.9943528877412,21.4146260902305,0.719745496340949));
#54589=CARTESIAN_POINT('Ctrl Pts',(-16.9951723491632,21.4019047888025,0.702556657651023));
#54590=CARTESIAN_POINT('Ctrl Pts',(-16.9953772145187,21.3987244634455,0.698259447978542));
#54591=CARTESIAN_POINT('Ctrl Pts',(-16.9955735792695,21.3954682517381,0.69400371178678));
#54592=CARTESIAN_POINT('Ctrl Pts',(-16.9957617899228,21.3921349753008,0.689790133583646));
#54593=CARTESIAN_POINT('Ctrl Pts',(-16.9959500005762,21.3888016988636,0.685576555380513));
#54594=CARTESIAN_POINT('Ctrl Pts',(-16.9961295493961,21.3853997705542,0.681416137771084));
#54595=CARTESIAN_POINT('Ctrl Pts',(-16.9963002484149,21.381944233318,0.677325857685364));
#54596=CARTESIAN_POINT('Ctrl Pts',(-16.9966416464526,21.3750331588455,0.669145297513925));
#54597=CARTESIAN_POINT('Ctrl Pts',(-16.9969485933011,21.3678906232202,0.661223354235855));
#54598=CARTESIAN_POINT('Ctrl Pts',(-16.9972257305589,21.360521338635,0.65355467291949));
#54599=CARTESIAN_POINT('Ctrl Pts',(-16.9977800050746,21.3457827694648,0.638217310286761));
#54600=CARTESIAN_POINT('Ctrl Pts',(-16.9982150450431,21.3301402535137,0.623890202235327));
#54601=CARTESIAN_POINT('Ctrl Pts',(-16.9985616334457,21.3135980989733,0.61056934740525));
#54602=CARTESIAN_POINT('Ctrl Pts',(-16.9987349276469,21.3053270217032,0.603908919990211));
#54603=CARTESIAN_POINT('Ctrl Pts',(-16.9988860174545,21.2968304471392,0.597500710279847));
#54604=CARTESIAN_POINT('Ctrl Pts',(-16.9990182484227,21.2881047011117,0.591348949103243));
#54605=CARTESIAN_POINT('Ctrl Pts',(-16.9990843639068,21.2837418280979,0.588273068514941));
#54606=CARTESIAN_POINT('Ctrl Pts',(-16.9991457654173,21.2793216399187,0.585261334334855));
#54607=CARTESIAN_POINT('Ctrl Pts',(-16.9992028412883,21.2748433907653,0.58231457937545));
#54608=CARTESIAN_POINT('Ctrl Pts',(-16.9992599171592,21.2703651416119,0.579367824416043));
#54609=CARTESIAN_POINT('Ctrl Pts',(-16.9993127537119,21.2658204194787,0.576481010796243));
#54610=CARTESIAN_POINT('Ctrl Pts',(-16.9993614043243,21.2612406847754,0.573674650246304));
#54611=CARTESIAN_POINT('Ctrl Pts',(-16.9995560067739,21.2429217459622,0.562449208046549));
#54612=CARTESIAN_POINT('Ctrl Pts',(-16.9996844419683,21.2240702465873,0.552514693415452));
#54613=CARTESIAN_POINT('Ctrl Pts',(-16.9997740428036,21.204705397676,0.543824923165798));
#54614=CARTESIAN_POINT('Ctrl Pts',(-16.9998636436388,21.1853405487646,0.535135152916144));
#54615=CARTESIAN_POINT('Ctrl Pts',(-16.9999142934875,21.1654623146662,0.527690138120709));
#54616=CARTESIAN_POINT('Ctrl Pts',(-16.9999455849911,21.1450641098525,0.52150610826049));
#54617=CARTESIAN_POINT('Ctrl Pts',(-16.999961230743,21.1348650074456,0.518414093330381));
#54618=CARTESIAN_POINT('Ctrl Pts',(-16.9999719363109,21.1245355567772,0.515638162273462));
#54619=CARTESIAN_POINT('Ctrl Pts',(-16.9999795432265,21.114072442886,0.513186403367121));
#54620=CARTESIAN_POINT('Ctrl Pts',(-16.9999833466843,21.1088408859405,0.511960523913951));
#54621=CARTESIAN_POINT('Ctrl Pts',(-16.9999863636806,21.1035820426627,0.510817546177565));
#54622=CARTESIAN_POINT('Ctrl Pts',(-16.9999887849483,21.0983273296019,0.509763591729921));
#54623=CARTESIAN_POINT('Ctrl Pts',(-16.999991206216,21.093072616541,0.508709637282276));
#54624=CARTESIAN_POINT('Ctrl Pts',(-16.9999930072076,21.0878132493178,0.507742627816665));
#54625=CARTESIAN_POINT('Ctrl Pts',(-16.9999944360759,21.08254922085,0.506861453386952));
#54626=CARTESIAN_POINT('Ctrl Pts',(-17.0000001515491,21.0614931069787,0.5033367556681));
#54627=CARTESIAN_POINT('Ctrl Pts',(-16.9999999151385,21.0403633334935,0.501180364269346));
#54628=CARTESIAN_POINT('Ctrl Pts',(-16.999999983465,21.0191612004193,0.500367286323289));
#54629=CARTESIAN_POINT('Ctrl Pts',(-17.000000004027,21.0127807046791,0.500122601491195));
#54630=CARTESIAN_POINT('Ctrl Pts',(-17.0000000526406,21.0063936586163,0.499999543843031));
#54631=CARTESIAN_POINT('Ctrl Pts',(-17.0000000862986,21.0000000000001,0.499999252164641));
#54632=CARTESIAN_POINT('',(-16.9996439954592,20.7720018726588,0.555009152983013));
#54633=CARTESIAN_POINT('Ctrl Pts',(-17.0000000877479,21.,0.499999253801316));
#54634=CARTESIAN_POINT('Ctrl Pts',(-17.0000001651403,20.9851477858762,0.49999856840262));
#54635=CARTESIAN_POINT('Ctrl Pts',(-17.0000001594763,20.9702598890947,0.500660382574086));
#54636=CARTESIAN_POINT('Ctrl Pts',(-16.9999993047839,20.9499982803608,0.502477594919463));
#54637=CARTESIAN_POINT('Ctrl Pts',(-16.9999989597664,20.9446478701007,0.503044245481599));
#54638=CARTESIAN_POINT('Ctrl Pts',(-16.9999978251355,20.9339792642195,0.504348769112458));
#54639=CARTESIAN_POINT('Ctrl Pts',(-16.9999954462377,20.9180500526981,0.506558461151423));
#54640=CARTESIAN_POINT('Ctrl Pts',(-16.9999899689093,20.9023385597306,0.509515289748651));
#54641=CARTESIAN_POINT('Ctrl Pts',(-16.9999708157118,20.8712004350647,0.516406468513256));
#54642=CARTESIAN_POINT('Ctrl Pts',(-16.9999475802786,20.8508203671619,0.522300064017838));
#54643=CARTESIAN_POINT('Ctrl Pts',(-16.9998727181797,20.8208178771162,0.533088108138553));
#54644=CARTESIAN_POINT('Ctrl Pts',(-16.9998251170355,20.805958960354,0.538970501410492));
#54645=CARTESIAN_POINT('Ctrl Pts',(-16.9997329714124,20.7864371314905,0.54780774482637));
#54646=CARTESIAN_POINT('Ctrl Pts',(-16.9996756422965,20.7767738128281,0.552564173654396));
#54647=CARTESIAN_POINT('Ctrl Pts',(-16.9996439954592,20.7720018726588,0.555009152983013));
#54648=CARTESIAN_POINT('Ctrl Pts',(-16.9996439954592,20.7720018726588,0.555009152983015));
#54649=CARTESIAN_POINT('Ctrl Pts',(-16.9995764019144,20.7618096266294,0.560231312098567));
#54650=CARTESIAN_POINT('Ctrl Pts',(-16.999744036059,20.7518188801895,0.565791848329536));
#54651=CARTESIAN_POINT('Ctrl Pts',(-17.0001141476166,20.7420298241553,0.571687744309563));
#54652=CARTESIAN_POINT('Ctrl Pts',(-17.0004874229058,20.7321570907942,0.577634038694984));
#54653=CARTESIAN_POINT('Ctrl Pts',(-17.0010693506212,20.7224661626916,0.583939604181921));
#54654=CARTESIAN_POINT('Ctrl Pts',(-17.0018149866956,20.7130824637923,0.590514557747761));
#54655=CARTESIAN_POINT('Ctrl Pts',(-17.0033122137324,20.694240124774,0.603716974560899));
#54656=CARTESIAN_POINT('Ctrl Pts',(-17.0054671735487,20.6765333488168,0.618051718651848));
#54657=CARTESIAN_POINT('Ctrl Pts',(-17.0079791771995,20.6598958538764,0.633490559753894));
#54658=CARTESIAN_POINT('Ctrl Pts',(-17.0104973975899,20.6432171842449,0.648967609102669));
#54659=CARTESIAN_POINT('Ctrl Pts',(-17.0133771603985,20.6276123165059,0.665555354806171));
#54660=CARTESIAN_POINT('Ctrl Pts',(-17.0163366248286,20.6130881199025,0.683299515252358));
#54661=CARTESIAN_POINT('Ctrl Pts',(-17.0170769637466,20.6094547503342,0.687738390209771));
#54662=CARTESIAN_POINT('Ctrl Pts',(-17.0178235541468,20.6058834717914,0.692257774069122));
#54663=CARTESIAN_POINT('Ctrl Pts',(-17.018567812662,20.6023942721301,0.696833898390537));
#54664=CARTESIAN_POINT('Ctrl Pts',(-17.019312023868,20.5989052942621,0.701409731827615));
#54665=CARTESIAN_POINT('Ctrl Pts',(-17.020052498857,20.595504625966,0.706033510702339));
#54666=CARTESIAN_POINT('Ctrl Pts',(-17.0207848923251,20.5921907419765,0.710704979181601));
#54667=CARTESIAN_POINT('Ctrl Pts',(-17.02224911219,20.5855655398429,0.720044299155679));
#54668=CARTESIAN_POINT('Ctrl Pts',(-17.0236809280861,20.5792868927269,0.729573973065133));
#54669=CARTESIAN_POINT('Ctrl Pts',(-17.0250473303692,20.5733474924981,0.739293962781099));
#54670=CARTESIAN_POINT('Ctrl Pts',(-17.0277720965537,20.5615036328232,0.75867676067364));
#54671=CARTESIAN_POINT('Ctrl Pts',(-17.0302364268958,20.5510032860685,0.778813429678428));
#54672=CARTESIAN_POINT('Ctrl Pts',(-17.0321922520697,20.5418565839912,0.799738644735398));
#54673=CARTESIAN_POINT('Ctrl Pts',(-17.0331698308387,20.5372847941006,0.810197680773625));
#54674=CARTESIAN_POINT('Ctrl Pts',(-17.0340205434215,20.5330525151684,0.820854418209816));
#54675=CARTESIAN_POINT('Ctrl Pts',(-17.0347134066204,20.52916974434,0.831717884603113));
#54676=CARTESIAN_POINT('Ctrl Pts',(-17.0350598382199,20.5272283589258,0.837149617799762));
#54677=CARTESIAN_POINT('Ctrl Pts',(-17.0353668002234,20.5253734731873,0.842637732950806));
#54678=CARTESIAN_POINT('Ctrl Pts',(-17.0356284233313,20.5236226585739,0.84812956651519));
#54679=CARTESIAN_POINT('Ctrl Pts',(-17.0358900464393,20.5218718439606,0.853621400079574));
#54680=CARTESIAN_POINT('Ctrl Pts',(-17.0361071634375,20.5202207447736,0.859128525898787));
#54681=CARTESIAN_POINT('Ctrl Pts',(-17.0362776979317,20.5186679181996,0.864650722093725));
#54682=CARTESIAN_POINT('Ctrl Pts',(-17.0369593616,20.512460930786,0.886724147967845));
#54683=CARTESIAN_POINT('Ctrl Pts',(-17.0368937799335,20.5078176119001,0.909036478152388));
#54684=CARTESIAN_POINT('Ctrl Pts',(-17.0359746831307,20.5047035481734,0.931579061625702));
#54685=CARTESIAN_POINT('Ctrl Pts',(-17.0350543072948,20.5015851508547,0.954153015799173));
#54686=CARTESIAN_POINT('Ctrl Pts',(-17.0332780282032,20.5,0.976957807069396));
#54687=CARTESIAN_POINT('Ctrl Pts',(-17.0305720504421,20.5,1.));
#54688=CARTESIAN_POINT('',(-28.5,20.5,1.));
#54689=CARTESIAN_POINT('',(-29.,20.5,1.));
#54690=CARTESIAN_POINT('',(-28.5,21.5,1.));
#54691=CARTESIAN_POINT('Origin',(-28.5,21.,1.));
#54692=CARTESIAN_POINT('',(-29.,21.5,1.));
#54693=CARTESIAN_POINT('Origin',(-28.5,21.,0.));
#54694=CARTESIAN_POINT('Origin',(-28.5,21.,1.));
#54695=CARTESIAN_POINT('',(-28.5,20.5,4.01452801010865));
#54696=CARTESIAN_POINT('',(-28.5,20.5,1.));
#54697=CARTESIAN_POINT('',(-28.9999999990691,21.0000000000002,3.86712647556469));
#54698=CARTESIAN_POINT('Ctrl Pts',(-28.5,20.5,4.01452801010866));
#54699=CARTESIAN_POINT('Ctrl Pts',(-28.5164513514331,20.5,4.01507018860936));
#54700=CARTESIAN_POINT('Ctrl Pts',(-28.5328300075924,20.5008099557645,4.0150659425191));
#54701=CARTESIAN_POINT('Ctrl Pts',(-28.5491369527492,20.5024202979677,4.01452953611992));
#54702=CARTESIAN_POINT('Ctrl Pts',(-28.5495960158313,20.5024656313302,4.01451443553716));
#54703=CARTESIAN_POINT('Ctrl Pts',(-28.5500550220854,20.502511600136,4.01449891327935));
#54704=CARTESIAN_POINT('Ctrl Pts',(-28.550513971537,20.5025582045811,4.01448296968854));
#54705=CARTESIAN_POINT('Ctrl Pts',(-28.5582710692767,20.5033459062212,4.01421349340558));
#54706=CARTESIAN_POINT('Ctrl Pts',(-28.566010072344,20.5043149278755,4.01382377207131));
#54707=CARTESIAN_POINT('Ctrl Pts',(-28.5737362162412,20.5054669167645,4.01331514715339));
#54708=CARTESIAN_POINT('Ctrl Pts',(-28.5743575582699,20.5055595605364,4.01327424317302));
#54709=CARTESIAN_POINT('Ctrl Pts',(-28.5749787684162,20.5056533859706,4.01323257019164));
#54710=CARTESIAN_POINT('Ctrl Pts',(-28.5755997697761,20.5057483782164,4.0131901369871));
#54711=CARTESIAN_POINT('Ctrl Pts',(-28.5790836390542,20.5062812926157,4.01295208318048));
#54712=CARTESIAN_POINT('Ctrl Pts',(-28.5825594001091,20.5068506858238,4.01269019751249));
#54713=CARTESIAN_POINT('Ctrl Pts',(-28.5860143380244,20.5074540288925,4.01240599961348));
#54714=CARTESIAN_POINT('Ctrl Pts',(-28.5900946138146,20.5081665760285,4.01207036237905));
#54715=CARTESIAN_POINT('Ctrl Pts',(-28.5941521350908,20.5089273704629,4.01170321587125));
#54716=CARTESIAN_POINT('Ctrl Pts',(-28.598189247445,20.5097359163816,4.01130545373038));
#54717=CARTESIAN_POINT('Ctrl Pts',(-28.5989198489116,20.5098822399867,4.01123347019909));
#54718=CARTESIAN_POINT('Ctrl Pts',(-28.5996497830969,20.5100301241402,4.01116048399731));
#54719=CARTESIAN_POINT('Ctrl Pts',(-28.6003790631507,20.5101795680466,4.01108649976395));
#54720=CARTESIAN_POINT('Ctrl Pts',(-28.6158373800123,20.5133472828995,4.00951827954991));
#54721=CARTESIAN_POINT('Ctrl Pts',(-28.6309836846376,20.51721179935,4.00750372591642));
#54722=CARTESIAN_POINT('Ctrl Pts',(-28.6458381311819,20.5217414512072,4.00509762013458));
#54723=CARTESIAN_POINT('Ctrl Pts',(-28.6466878656163,20.5220005656176,4.00495998115022));
#54724=CARTESIAN_POINT('Ctrl Pts',(-28.6475366445442,20.5222618577133,4.00482105955225));
#54725=CARTESIAN_POINT('Ctrl Pts',(-28.6483844703545,20.522525325589,4.00468086503783));
#54726=CARTESIAN_POINT('Ctrl Pts',(-28.6631564601653,20.5271158260522,4.00223820297968));
#54727=CARTESIAN_POINT('Ctrl Pts',(-28.6776392202979,20.5323666655798,3.99940952546827));
#54728=CARTESIAN_POINT('Ctrl Pts',(-28.6918445815767,20.5382688482248,3.99624486790792));
#54729=CARTESIAN_POINT('Ctrl Pts',(-28.6927070946931,20.5386272136227,3.99605271801456));
#54730=CARTESIAN_POINT('Ctrl Pts',(-28.6935685850001,20.5389879805298,3.99585932819182));
#54731=CARTESIAN_POINT('Ctrl Pts',(-28.69442905358,20.539351151545,3.99566470942585));
#54732=CARTESIAN_POINT('Ctrl Pts',(-28.7019451320231,20.5425234019941,3.99396474042557));
#54733=CARTESIAN_POINT('Ctrl Pts',(-28.7093832773834,20.5458790798609,3.99217104269849));
#54734=CARTESIAN_POINT('Ctrl Pts',(-28.7167440887879,20.5494199410241,3.99029080026248));
#54735=CARTESIAN_POINT('Ctrl Pts',(-28.7232979155013,20.5525726084686,3.98861669364193));
#54736=CARTESIAN_POINT('Ctrl Pts',(-28.7297897873453,20.5558717313291,3.98687415899974));
#54737=CARTESIAN_POINT('Ctrl Pts',(-28.736222233402,20.5593197798329,3.98506764460692));
#54738=CARTESIAN_POINT('Ctrl Pts',(-28.7370142722704,20.5597443443626,3.98484520517987));
#54739=CARTESIAN_POINT('Ctrl Pts',(-28.7378049045635,20.560170909351,3.98462193461541));
#54740=CARTESIAN_POINT('Ctrl Pts',(-28.738594101696,20.560599450483,3.98439785654188));
#54741=CARTESIAN_POINT('Ctrl Pts',(-28.7450528664492,20.564106617761,3.98256400856681));
#54742=CARTESIAN_POINT('Ctrl Pts',(-28.7514055277704,20.5677406151965,3.98067895641415));
#54743=CARTESIAN_POINT('Ctrl Pts',(-28.7576397468618,20.5714889023174,3.97875498379703));
#54744=CARTESIAN_POINT('Ctrl Pts',(-28.7646594833789,20.5757094771148,3.97658858883395));
#54745=CARTESIAN_POINT('Ctrl Pts',(-28.7715387445494,20.5800801099293,3.97437012159623));
#54746=CARTESIAN_POINT('Ctrl Pts',(-28.7782883626914,20.5846018931307,3.9721074341771));
#54747=CARTESIAN_POINT('Ctrl Pts',(-28.7789062759519,20.5850158528159,3.97190028993112));
#54748=CARTESIAN_POINT('Ctrl Pts',(-28.7795231038942,20.5854310777311,3.97169277505919));
#54749=CARTESIAN_POINT('Ctrl Pts',(-28.7801388532259,20.5858475706905,3.97148489500656));
#54750=CARTESIAN_POINT('Ctrl Pts',(-28.7930138998851,20.5945562545815,3.96713821488955));
#54751=CARTESIAN_POINT('Ctrl Pts',(-28.8054045352405,20.6038101537282,3.96263694559618));
#54752=CARTESIAN_POINT('Ctrl Pts',(-28.8173345884296,20.6136080241694,3.95804337703345));
#54753=CARTESIAN_POINT('Ctrl Pts',(-28.8177423111309,20.6139428771781,3.95788638677082));
#54754=CARTESIAN_POINT('Ctrl Pts',(-28.8181494955581,20.6142783658853,3.95772928820928));
#54755=CARTESIAN_POINT('Ctrl Pts',(-28.8185561420664,20.6146144909891,3.95757208373558));
#54756=CARTESIAN_POINT('Ctrl Pts',(-28.8306505221365,20.6246114408557,3.95289654708411));
#54757=CARTESIAN_POINT('Ctrl Pts',(-28.8422694642204,20.6351711425685,3.9481277290909));
#54758=CARTESIAN_POINT('Ctrl Pts',(-28.8534199982048,20.6463132673266,3.94332838466393));
#54759=CARTESIAN_POINT('Ctrl Pts',(-28.8536143750091,20.6465074975408,3.94324472219236));
#54760=CARTESIAN_POINT('Ctrl Pts',(-28.8538086101574,20.6467019063127,3.94316104994417));
#54761=CARTESIAN_POINT('Ctrl Pts',(-28.8540027035162,20.6468964937161,3.94307736830263));
#54762=CARTESIAN_POINT('Ctrl Pts',(-28.8595679483428,20.6524759042999,3.9406779620294));
#54763=CARTESIAN_POINT('Ctrl Pts',(-28.8650165644509,20.6582020618217,3.93827087234596));
#54764=CARTESIAN_POINT('Ctrl Pts',(-28.8703459030302,20.6640775206855,3.93586485412722));
#54765=CARTESIAN_POINT('Ctrl Pts',(-28.8704406479323,20.664181974506,3.93582207997102));
#54766=CARTESIAN_POINT('Ctrl Pts',(-28.8705353426575,20.6642864617524,3.93577931180518));
#54767=CARTESIAN_POINT('Ctrl Pts',(-28.8706299872311,20.6643909824247,3.93573654967076));
#54768=CARTESIAN_POINT('Ctrl Pts',(-28.8760419628682,20.6703676941454,3.93329132094817));
#54769=CARTESIAN_POINT('Ctrl Pts',(-28.8812917390082,20.6764556221647,3.93086501555022));
#54770=CARTESIAN_POINT('Ctrl Pts',(-28.8863833106843,20.6826548610351,3.92846553582844));
#54771=CARTESIAN_POINT('Ctrl Pts',(-28.8863892980072,20.6826621508951,3.92846271421248));
#54772=CARTESIAN_POINT('Ctrl Pts',(-28.8863952851119,20.682669440909,3.92845989263359));
#54773=CARTESIAN_POINT('Ctrl Pts',(-28.8864012719985,20.6826767310768,3.92845707109178));
#54774=CARTESIAN_POINT('Ctrl Pts',(-28.8965956469561,20.695090312607,3.9236525946728));
#54775=CARTESIAN_POINT('Ctrl Pts',(-28.906157067648,20.7079490685553,3.91895575780338));
#54776=CARTESIAN_POINT('Ctrl Pts',(-28.9150984275965,20.7212648273691,3.91442809948265));
#54777=CARTESIAN_POINT('Ctrl Pts',(-28.9152182750854,20.7214433080774,3.91436741201639));
#54778=CARTESIAN_POINT('Ctrl Pts',(-28.9153380111198,20.7216218709325,3.91430675503477));
#54779=CARTESIAN_POINT('Ctrl Pts',(-28.9154576357267,20.7218005159667,3.91424612868925));
#54780=CARTESIAN_POINT('Ctrl Pts',(-28.9242627426992,20.7349498894741,3.90978365669779));
#54781=CARTESIAN_POINT('Ctrl Pts',(-28.9324644748558,20.7485442462784,3.90548665876825));
#54782=CARTESIAN_POINT('Ctrl Pts',(-28.9400523922733,20.7626102463437,3.90141604958038));
#54783=CARTESIAN_POINT('Ctrl Pts',(-28.9402293321847,20.7629382463295,3.90132112851187));
#54784=CARTESIAN_POINT('Ctrl Pts',(-28.9404059381619,20.7632665029513,3.90122633069731));
#54785=CARTESIAN_POINT('Ctrl Pts',(-28.9405822100495,20.7635950165753,3.90113165692879));
#54786=CARTESIAN_POINT('Ctrl Pts',(-28.9442369224986,20.7704062151575,3.89916874948485));
#54787=CARTESIAN_POINT('Ctrl Pts',(-28.9477477566326,20.7773280603452,3.89725914981838));
#54788=CARTESIAN_POINT('Ctrl Pts',(-28.9511114770745,20.7843650393795,3.89541021586002));
#54789=CARTESIAN_POINT('Ctrl Pts',(-28.9512925263593,20.7847437985669,3.89531069862113));
#54790=CARTESIAN_POINT('Ctrl Pts',(-28.9514731291436,20.7851228489911,3.89521136826826));
#54791=CARTESIAN_POINT('Ctrl Pts',(-28.9516532891227,20.7855021994876,3.89511222369121));
#54792=CARTESIAN_POINT('Ctrl Pts',(-28.9532274481634,20.7888167980831,3.89424594177283));
#54793=CARTESIAN_POINT('Ctrl Pts',(-28.954769491257,20.7921584950771,3.89339288708423));
#54794=CARTESIAN_POINT('Ctrl Pts',(-28.9562782863987,20.7955254042893,3.89255427234121));
#54795=CARTESIAN_POINT('Ctrl Pts',(-28.9579597607261,20.7992776508642,3.89161967948501));
#54796=CARTESIAN_POINT('Ctrl Pts',(-28.9596006031374,20.8030630949436,3.89070263223272));
#54797=CARTESIAN_POINT('Ctrl Pts',(-28.9611903084036,20.8068588900011,3.88980980999067));
#54798=CARTESIAN_POINT('Ctrl Pts',(-28.9613600382809,20.8072641599861,3.88971448501893));
#54799=CARTESIAN_POINT('Ctrl Pts',(-28.9615292133495,20.8076696119071,3.88961942017834));
#54800=CARTESIAN_POINT('Ctrl Pts',(-28.9616978272843,20.8080752327577,3.88952461997149));
#54801=CARTESIAN_POINT('Ctrl Pts',(-28.9678462263432,20.8228659370924,3.88606779119053));
#54802=CARTESIAN_POINT('Ctrl Pts',(-28.9732630364474,20.83789669793,3.88295611032183));
#54803=CARTESIAN_POINT('Ctrl Pts',(-28.9779549539186,20.8531699429438,3.88022807675177));
#54804=CARTESIAN_POINT('Ctrl Pts',(-28.9780746227798,20.8535594919608,3.88015849737982));
#54805=CARTESIAN_POINT('Ctrl Pts',(-28.9781938201495,20.8539491990382,3.88008916763081));
#54806=CARTESIAN_POINT('Ctrl Pts',(-28.9783125461397,20.8543390642437,3.88002008814799));
#54807=CARTESIAN_POINT('Ctrl Pts',(-28.9829764275231,20.8696540350547,3.87730645726259));
#54808=CARTESIAN_POINT('Ctrl Pts',(-28.986912984661,20.88521298573,3.87497871048076));
#54809=CARTESIAN_POINT('Ctrl Pts',(-28.9901062452497,20.9010259115082,3.87307658812189));
#54810=CARTESIAN_POINT('Ctrl Pts',(-28.9901641270832,20.901312540523,3.87304210978022));
#54811=CARTESIAN_POINT('Ctrl Pts',(-28.9902217646508,20.9015992530081,3.87300777139739));
#54812=CARTESIAN_POINT('Ctrl Pts',(-28.9902791578525,20.9018860490275,3.87297357321668));
#54813=CARTESIAN_POINT('Ctrl Pts',(-28.9934686710319,20.9178241681235,3.87107307725357));
#54814=CARTESIAN_POINT('Ctrl Pts',(-28.9959038918218,20.9340201547597,3.86960522446342));
#54815=CARTESIAN_POINT('Ctrl Pts',(-28.9975428631309,20.9504914199225,3.86861479762559));
#54816=CARTESIAN_POINT('Ctrl Pts',(-28.9975508466297,20.9505716521533,3.86860997321448));
#54817=CARTESIAN_POINT('Ctrl Pts',(-28.9975588112477,20.9506518910969,3.8686051601259));
#54818=CARTESIAN_POINT('Ctrl Pts',(-28.9975667569751,20.9507321367091,3.86860035836809));
#54819=CARTESIAN_POINT('Ctrl Pts',(-28.9979739536847,20.9548445039341,3.86835428146862));
#54820=CARTESIAN_POINT('Ctrl Pts',(-28.9983312836708,20.9589758111358,3.86813805483529));
#54821=CARTESIAN_POINT('Ctrl Pts',(-28.9986360973411,20.9630941410715,3.86795347229001));
#54822=CARTESIAN_POINT('Ctrl Pts',(-28.9986369825427,20.9631061010088,3.86795293624854));
#54823=CARTESIAN_POINT('Ctrl Pts',(-28.9986378673028,20.9631180608498,3.86795240047308));
#54824=CARTESIAN_POINT('Ctrl Pts',(-28.9986387516214,20.9631300205938,3.86795186496367));
#54825=CARTESIAN_POINT('Ctrl Pts',(-28.9989442640887,20.9672618470215,3.86776685833533));
#54826=CARTESIAN_POINT('Ctrl Pts',(-28.9991977435996,20.9713882018456,3.86761320323202));
#54827=CARTESIAN_POINT('Ctrl Pts',(-28.9993998330421,20.9755090474354,3.86749064815707));
#54828=CARTESIAN_POINT('Ctrl Pts',(-28.9994025151862,20.975563739564,3.86748902159821));
#54829=CARTESIAN_POINT('Ctrl Pts',(-28.9994051882825,20.9756184307224,3.86748740051734));
#54830=CARTESIAN_POINT('Ctrl Pts',(-28.9994078523321,20.9756731209105,3.86748578491389));
#54831=CARTESIAN_POINT('Ctrl Pts',(-28.9998038844389,20.9838032512471,3.86724561264447));
#54832=CARTESIAN_POINT('Ctrl Pts',(-29.0000000019467,20.9919120710539,3.86712648199996));
#54833=CARTESIAN_POINT('Ctrl Pts',(-29.0000000000226,21.0000000000002,3.86712647556469));
#54834=CARTESIAN_POINT('',(-28.5,21.5,4.01452801010865));
#54835=CARTESIAN_POINT('Ctrl Pts',(-29.0000000000226,21.0000000000002,3.86712647556469));
#54836=CARTESIAN_POINT('Ctrl Pts',(-29.0000000000077,21.0000628081229,3.86712647551472));
#54837=CARTESIAN_POINT('Ctrl Pts',(-28.9999999881654,21.0001256149852,3.86712648264873));
#54838=CARTESIAN_POINT('Ctrl Pts',(-28.9999999644977,21.0001884205867,3.86712649696792));
#54839=CARTESIAN_POINT('Ctrl Pts',(-28.9999998965082,21.0003688399577,3.86712653810216));
#54840=CARTESIAN_POINT('Ctrl Pts',(-28.9999997311066,21.0005492489388,3.86712663852461));
#54841=CARTESIAN_POINT('Ctrl Pts',(-28.9999994683105,21.0007296475219,3.86712679826507));
#54842=CARTESIAN_POINT('Ctrl Pts',(-28.9999757916729,21.0169826794255,3.86714119010008));
#54843=CARTESIAN_POINT('Ctrl Pts',(-28.9991615791828,21.0331513380247,3.86763657203004));
#54844=CARTESIAN_POINT('Ctrl Pts',(-28.9975697782028,21.0492373417148,3.86859853229563));
#54845=CARTESIAN_POINT('Ctrl Pts',(-28.9975299458722,21.0496398688054,3.86862260384717));
#54846=CARTESIAN_POINT('Ctrl Pts',(-28.9974896266431,21.0500423441396,3.86864696760125));
#54847=CARTESIAN_POINT('Ctrl Pts',(-28.9974488203613,21.0504447677163,3.86867162334182));
#54848=CARTESIAN_POINT('Ctrl Pts',(-28.9958374348699,21.0663359365465,3.86964524556126));
#54849=CARTESIAN_POINT('Ctrl Pts',(-28.9934664417955,21.0821470065985,3.87107424571494));
#54850=CARTESIAN_POINT('Ctrl Pts',(-28.9903267115591,21.0978760232723,3.87294518199751));
#54851=CARTESIAN_POINT('Ctrl Pts',(-28.9902095243118,21.0984630928699,3.87301501279706));
#54852=CARTESIAN_POINT('Ctrl Pts',(-28.9900912606925,21.0990500622799,3.8730854613775));
#54853=CARTESIAN_POINT('Ctrl Pts',(-28.9899719201338,21.099636928186,3.873156526561));
#54854=CARTESIAN_POINT('Ctrl Pts',(-28.9891427293275,21.1037145344837,3.87365029496153));
#54855=CARTESIAN_POINT('Ctrl Pts',(-28.9882616492729,21.1077866910186,3.8741737758945));
#54856=CARTESIAN_POINT('Ctrl Pts',(-28.9873282487272,21.1118533764022,3.87472671536206));
#54857=CARTESIAN_POINT('Ctrl Pts',(-28.9865480123162,21.115252748754,3.87518892154743));
#54858=CARTESIAN_POINT('Ctrl Pts',(-28.9857308794749,21.1186496307155,3.8756719108919));
#54859=CARTESIAN_POINT('Ctrl Pts',(-28.984877571924,21.1220399125086,3.87617496320682));
#54860=CARTESIAN_POINT('Ctrl Pts',(-28.9847100635754,21.1227054410203,3.87627371477936));
#54861=CARTESIAN_POINT('Ctrl Pts',(-28.9845412792207,21.1233702543533,3.87637316979248));
#54862=CARTESIAN_POINT('Ctrl Pts',(-28.9843712295124,21.1240343283173,3.87647331953722));
#54863=CARTESIAN_POINT('Ctrl Pts',(-28.9824842924156,21.1314031489441,3.87758461970075));
#54864=CARTESIAN_POINT('Ctrl Pts',(-28.9804413090385,21.1386820012024,3.8787816368253));
#54865=CARTESIAN_POINT('Ctrl Pts',(-28.9782473821909,21.1458747456812,3.88005797372067));
#54866=CARTESIAN_POINT('Ctrl Pts',(-28.9780315058454,21.1465824918825,3.88018356174789));
#54867=CARTESIAN_POINT('Ctrl Pts',(-28.977814170689,21.1472894055721,3.88030991766809));
#54868=CARTESIAN_POINT('Ctrl Pts',(-28.9775953797715,21.1479954896081,3.88043703577741));
#54869=CARTESIAN_POINT('Ctrl Pts',(-28.9729390160451,21.1630225489193,3.88314239558005));
#54870=CARTESIAN_POINT('Ctrl Pts',(-28.9676236436874,21.1776738449045,3.88619297247208));
#54871=CARTESIAN_POINT('Ctrl Pts',(-28.9616771780539,21.1919744338817,3.88953620066551));
#54872=CARTESIAN_POINT('Ctrl Pts',(-28.9613856085175,21.1926756262127,3.88970012719846));
#54873=CARTESIAN_POINT('Ctrl Pts',(-28.9610925208102,21.1933759749083,3.88986475847562));
#54874=CARTESIAN_POINT('Ctrl Pts',(-28.960797915745,21.1940754818056,3.89003008861958));
#54875=CARTESIAN_POINT('Ctrl Pts',(-28.9547604581748,21.208410752005,3.89341826433982));
#54876=CARTESIAN_POINT('Ctrl Pts',(-28.9480857142471,21.2223930775751,3.89709988405803));
#54877=CARTESIAN_POINT('Ctrl Pts',(-28.9407802200781,21.2360355854272,3.90102529736883));
#54878=CARTESIAN_POINT('Ctrl Pts',(-28.9404589312627,21.2366355701902,3.90119793338271));
#54879=CARTESIAN_POINT('Ctrl Pts',(-28.9401364145058,21.2372349093322,3.90137104572976));
#54880=CARTESIAN_POINT('Ctrl Pts',(-28.939812669612,21.2378336017067,3.90154462963897));
#54881=CARTESIAN_POINT('Ctrl Pts',(-28.9359701268155,21.2449395085967,3.90360490491386));
#54882=CARTESIAN_POINT('Ctrl Pts',(-28.9319553000605,21.2519530849821,3.90573124712142));
#54883=CARTESIAN_POINT('Ctrl Pts',(-28.9277662154186,21.2588750987062,3.90791660649015));
#54884=CARTESIAN_POINT('Ctrl Pts',(-28.9238452263219,21.2653541132546,3.90996210592255));
#54885=CARTESIAN_POINT('Ctrl Pts',(-28.9197699102247,21.2717553746919,3.91206015529359));
#54886=CARTESIAN_POINT('Ctrl Pts',(-28.915543176381,21.2780716968035,3.91420268904662));
#54887=CARTESIAN_POINT('Ctrl Pts',(-28.9152541757013,21.2785035719702,3.91434918365304));
#54888=CARTESIAN_POINT('Ctrl Pts',(-28.9149646115042,21.2789348366557,3.91449581247848));
#54889=CARTESIAN_POINT('Ctrl Pts',(-28.9146744857417,21.2793654904408,3.91464257259226));
#54890=CARTESIAN_POINT('Ctrl Pts',(-28.9057700776902,21.2925829206963,3.91914686730788));
#54891=CARTESIAN_POINT('Ctrl Pts',(-28.8963265621576,21.30524079736,3.92377989260965));
#54892=CARTESIAN_POINT('Ctrl Pts',(-28.8863569087761,21.3173772818602,3.92847795723015));
#54893=CARTESIAN_POINT('Ctrl Pts',(-28.8861752815226,21.3175983844665,3.92856354662239));
#54894=CARTESIAN_POINT('Ctrl Pts',(-28.8859934794983,21.3178193138715,3.92864915773935));
#54895=CARTESIAN_POINT('Ctrl Pts',(-28.8858115026676,21.3180400701975,3.92873479020661));
#54896=CARTESIAN_POINT('Ctrl Pts',(-28.8756595580032,21.3303554072503,3.9335119701669));
#54897=CARTESIAN_POINT('Ctrl Pts',(-28.8649638851134,21.3421324339506,3.93835551745067));
#54898=CARTESIAN_POINT('Ctrl Pts',(-28.8537165289396,21.3533901769361,3.94320069869318));
#54899=CARTESIAN_POINT('Ctrl Pts',(-28.8536956182929,21.3534111068935,3.94320970666551));
#54900=CARTESIAN_POINT('Ctrl Pts',(-28.8536747057384,21.3534320350552,3.94321871464462));
#54901=CARTESIAN_POINT('Ctrl Pts',(-28.853653791276,21.353452961421,3.94322772263006));
#54902=CARTESIAN_POINT('Ctrl Pts',(-28.8423834682513,21.3647296988866,3.94808191890573));
#54903=CARTESIAN_POINT('Ctrl Pts',(-28.8305594631821,21.3754852655172,3.95293799265001));
#54904=CARTESIAN_POINT('Ctrl Pts',(-28.8181518421502,21.3857193365208,3.95772816499657));
#54905=CARTESIAN_POINT('Ctrl Pts',(-28.8179754092975,21.3858648621084,3.957796279889));
#54906=CARTESIAN_POINT('Ctrl Pts',(-28.817798858339,21.3860102822034,3.95786438143738));
#54907=CARTESIAN_POINT('Ctrl Pts',(-28.817622189181,21.3861555967999,3.95793246944758));
#54908=CARTESIAN_POINT('Ctrl Pts',(-28.8146927985446,21.3885650904719,3.95906145190157));
#54909=CARTESIAN_POINT('Ctrl Pts',(-28.8117308312189,21.3909455061188,3.96018669192006));
#54910=CARTESIAN_POINT('Ctrl Pts',(-28.8087356960771,21.3932966693065,3.96130724892932));
#54911=CARTESIAN_POINT('Ctrl Pts',(-28.8085068196737,21.3934763359154,3.96139287747226));
#54912=CARTESIAN_POINT('Ctrl Pts',(-28.8082777512694,21.3936558303765,3.96147847800928));
#54913=CARTESIAN_POINT('Ctrl Pts',(-28.808048490278,21.3938351528717,3.96156405023994));
#54914=CARTESIAN_POINT('Ctrl Pts',(-28.8050966456304,21.3961440155534,3.96266583353729));
#54915=CARTESIAN_POINT('Ctrl Pts',(-28.802109551168,21.3984267656514,3.96376410259036));
#54916=CARTESIAN_POINT('Ctrl Pts',(-28.7991010675383,21.4006726193195,3.96485276880369));
#54917=CARTESIAN_POINT('Ctrl Pts',(-28.7988201115451,21.4008823548959,3.96495443706415));
#54918=CARTESIAN_POINT('Ctrl Pts',(-28.7985389685179,21.4010917689656,3.96505602171734));
#54919=CARTESIAN_POINT('Ctrl Pts',(-28.7982576504616,21.4013008521561,3.9651575175244));
#54920=CARTESIAN_POINT('Ctrl Pts',(-28.7920463251258,21.4059172771921,3.96739848095954));
#54921=CARTESIAN_POINT('Ctrl Pts',(-28.7857412868542,21.410379634955,3.96959946571781));
#54922=CARTESIAN_POINT('Ctrl Pts',(-28.779342978021,21.4146896451178,3.97175302079555));
#54923=CARTESIAN_POINT('Ctrl Pts',(-28.778966071058,21.4149435360886,3.97187988086517));
#54924=CARTESIAN_POINT('Ctrl Pts',(-28.7785888389221,21.4151968994391,3.97200657683767));
#54925=CARTESIAN_POINT('Ctrl Pts',(-28.7782112814686,21.4154497356643,3.97213310725282));
#54926=CARTESIAN_POINT('Ctrl Pts',(-28.7651895622522,21.4241698981271,3.97649706172807));
#54927=CARTESIAN_POINT('Ctrl Pts',(-28.7517817007072,21.4322645500552,3.98066442474707));
#54928=CARTESIAN_POINT('Ctrl Pts',(-28.7379728369994,21.4397373496941,3.98457399470782));
#54929=CARTESIAN_POINT('Ctrl Pts',(-28.7374403638241,21.440025502683,3.98472474868548));
#54930=CARTESIAN_POINT('Ctrl Pts',(-28.7369072941828,21.4403127306051,3.98487511891608));
#54931=CARTESIAN_POINT('Ctrl Pts',(-28.7363736271155,21.4405990335943,3.9850251018032));
#54932=CARTESIAN_POINT('Ctrl Pts',(-28.7226661907559,21.4479528319546,3.98887746783095));
#54933=CARTESIAN_POINT('Ctrl Pts',(-28.708564846762,21.4546967924008,3.99247483292586));
#54934=CARTESIAN_POINT('Ctrl Pts',(-28.6940418379805,21.4608120817006,3.99575219618881));
#54935=CARTESIAN_POINT('Ctrl Pts',(-28.6934296259969,21.4610698694256,3.99589035220693));
#54936=CARTESIAN_POINT('Ctrl Pts',(-28.6928166640662,21.4613265394595,3.99602793885868));
#54937=CARTESIAN_POINT('Ctrl Pts',(-28.6922029499329,21.4615820902473,3.99616495113051));
#54938=CARTESIAN_POINT('Ctrl Pts',(-28.6852539391292,21.4644756608685,3.9977163244909));
#54939=CARTESIAN_POINT('Ctrl Pts',(-28.6782083508407,21.4672254747693,3.99919404072758));
#54940=CARTESIAN_POINT('Ctrl Pts',(-28.6710619027125,21.4698274446379,4.00059030840056));
#54941=CARTESIAN_POINT('Ctrl Pts',(-28.6704499885629,21.4700502381363,4.00070986372797));
#54942=CARTESIAN_POINT('Ctrl Pts',(-28.6698373005598,21.4702719599817,4.00082882902828));
#54943=CARTESIAN_POINT('Ctrl Pts',(-28.6692238485867,21.4704926025662,4.00094719650824));
#54944=CARTESIAN_POINT('Ctrl Pts',(-28.6620401551094,21.4730763886888,4.00233331266908));
#54945=CARTESIAN_POINT('Ctrl Pts',(-28.6547457476138,21.4755124549176,4.00363754090848));
#54946=CARTESIAN_POINT('Ctrl Pts',(-28.6474356860117,21.4777684558703,4.00483716666479));
#54947=CARTESIAN_POINT('Ctrl Pts',(-28.6468600465228,21.4779461073466,4.00493163262073));
#54948=CARTESIAN_POINT('Ctrl Pts',(-28.6462842497821,21.4781226628457,4.00502546186105));
#54949=CARTESIAN_POINT('Ctrl Pts',(-28.6457083335891,21.4782981094701,4.00511864492646));
#54950=CARTESIAN_POINT('Ctrl Pts',(-28.6304080123218,21.4829591864661,4.00759423226838));
#54951=CARTESIAN_POINT('Ctrl Pts',(-28.6149415475987,21.4868701345595,4.00963042415946));
#54952=CARTESIAN_POINT('Ctrl Pts',(-28.5993223066573,21.4900357985373,4.01119295353938));
#54953=CARTESIAN_POINT('Ctrl Pts',(-28.5988756076155,21.4901263342471,4.0112376407543));
#54954=CARTESIAN_POINT('Ctrl Pts',(-28.5984287796622,21.4902162615444,4.01128194112185));
#54955=CARTESIAN_POINT('Ctrl Pts',(-28.5979818227772,21.4903055806385,4.01132585388403));
#54956=CARTESIAN_POINT('Ctrl Pts',(-28.5822122630561,21.4934569422931,4.01287518660258));
#54957=CARTESIAN_POINT('Ctrl Pts',(-28.566282210323,21.4958512063425,4.01394216943519));
#54958=CARTESIAN_POINT('Ctrl Pts',(-28.5501870504247,21.497474885185,4.01449425451777));
#54959=CARTESIAN_POINT('Ctrl Pts',(-28.5499299179448,21.4975008246954,4.01450307449889));
#54960=CARTESIAN_POINT('Ctrl Pts',(-28.5496727433489,21.497526567513,4.01451176304298));
#54961=CARTESIAN_POINT('Ctrl Pts',(-28.5494155266162,21.4975521135813,4.0145203200153));
#54962=CARTESIAN_POINT('Ctrl Pts',(-28.5331159748128,21.4991709408639,4.0150625662842));
#54963=CARTESIAN_POINT('Ctrl Pts',(-28.5166471370518,21.5,4.01507664076422));
#54964=CARTESIAN_POINT('Ctrl Pts',(-28.5,21.5,4.01452801010865));
#54965=CARTESIAN_POINT('',(-28.5,21.5,4.40714435599954));
#54966=CARTESIAN_POINT('Origin',(-174.463204856321,34.9999999945948,6.54993637452805E-10));
#54967=CARTESIAN_POINT('',(33.,30.9999999945948,6.54994127311525E-10));
#54968=CARTESIAN_POINT('Origin',(33.,34.9999999945948,6.54993637452805E-10));
#54969=CARTESIAN_POINT('',(-174.463204856321,30.9999999945948,6.54994127311525E-10));
#54970=CARTESIAN_POINT('Origin',(-174.463204856321,34.9999999945948,6.54993637452805E-10));
#54971=CARTESIAN_POINT('',(-39.,30.9999999945948,6.54994127311525E-10));
#54972=CARTESIAN_POINT('',(-174.463204856321,30.9999999945948,6.54994127311525E-10));
#54973=CARTESIAN_POINT('Origin',(-39.,34.9999999945948,6.54993637452805E-10));
#54974=CARTESIAN_POINT('Origin',(6.61363325216158E-15,57.,-24.));
#54975=CARTESIAN_POINT('',(-4.19913133791448,57.,-27.5520833333334));
#54976=CARTESIAN_POINT('',(-4.19913133791448,57.,-27.5520833333334));
#54977=CARTESIAN_POINT('',(4.1991313379145,57.,-27.5520833333334));
#54978=CARTESIAN_POINT('Origin',(6.61363325216158E-15,57.,-24.));
#54979=CARTESIAN_POINT('',(4.1991313379145,57.,-27.5520833333334));
#54980=CARTESIAN_POINT('Origin',(6.61363325216158E-15,69.8123087321227,
-24.));
#54981=CARTESIAN_POINT('',(6.91979495194842E-15,52.,-21.5));
#54982=CARTESIAN_POINT('Origin',(6.61363325216158E-15,52.,-24.));
#54983=CARTESIAN_POINT('',(6.91979495194842E-15,57.,-21.5));
#54984=CARTESIAN_POINT('',(6.91979495194842E-15,69.8123087321227,-21.5));
#54985=CARTESIAN_POINT('Origin',(6.61363325216158E-15,57.,-24.));
#54986=CARTESIAN_POINT('Origin',(33.,25.2727793885888,2.53685745363396));
#54987=CARTESIAN_POINT('',(16.5015526417024,25.4697390379769,2.99642996887271));
#54988=CARTESIAN_POINT('Ctrl Pts',(17.3583590725823,24.8843482494656,2.85169179564682));
#54989=CARTESIAN_POINT('Ctrl Pts',(17.3427646761208,24.8904421031615,2.85921017028675));
#54990=CARTESIAN_POINT('Ctrl Pts',(17.3271931898089,24.8967466727953,2.86654362190466));
#54991=CARTESIAN_POINT('Ctrl Pts',(17.1751346754118,24.9602776965675,2.93623867167078));
#54992=CARTESIAN_POINT('Ctrl Pts',(17.0358151286748,25.0347314689897,2.98601836429146));
#54993=CARTESIAN_POINT('Ctrl Pts',(16.8292928010538,25.1726430909796,3.0295764232713));
#54994=CARTESIAN_POINT('Ctrl Pts',(16.7546033612845,25.2287590875601,3.03852282224654));
#54995=CARTESIAN_POINT('Ctrl Pts',(16.6187499796368,25.3457029504125,3.03477909002088));
#54996=CARTESIAN_POINT('Ctrl Pts',(16.5558465481405,25.4073521349368,3.02316721276094));
#54997=CARTESIAN_POINT('Ctrl Pts',(16.5015526417035,25.4697390378793,2.99642996864261));
#54998=CARTESIAN_POINT('',(33.,25.4697390378784,2.99642996864299));
#54999=CARTESIAN_POINT('',(16.1963226914819,25.4697390378784,2.99642996864299));
#55000=CARTESIAN_POINT('Origin',(33.,25.2727793885888,2.53685745363396));
#55001=CARTESIAN_POINT('Origin',(33.,21.,6.));
#55002=CARTESIAN_POINT('',(23.,21.,8.067));
#55003=CARTESIAN_POINT('Origin',(23.,21.,6.));
#55004=CARTESIAN_POINT('',(33.,21.,8.067));
#55005=CARTESIAN_POINT('',(33.,21.,8.067));
#55006=CARTESIAN_POINT('Origin',(33.,21.,6.));
#55007=CARTESIAN_POINT('Origin',(1.25791587597333E-15,20.5440037453175,
-6.93889390390723E-15));
#55008=CARTESIAN_POINT('',(-6.64306116621187E-16,18.7883865373756,14.8183541121548));
#55009=CARTESIAN_POINT('Origin',(-1.13014538236401E-15,20.5440037453175,
19.5));
#55010=CARTESIAN_POINT('Origin',(1.15041887658705E-15,18.7883865373756,
-5.08824700431546E-15));
#55011=CARTESIAN_POINT('Origin',(7.22953690019729E-16,11.8071196962708,
-1.26385727337141E-15));
#55012=CARTESIAN_POINT('',(-1.41238078159923E-15,11.8071196962708,17.4363291775691));
#55013=CARTESIAN_POINT('',(-1.41238078159923E-15,11.8071196962708,17.4363291775691));
#55014=CARTESIAN_POINT('Origin',(7.22953690019729E-16,11.8071196962708,
-1.26385727337141E-15));
#55015=CARTESIAN_POINT('Origin',(7.01454290142472E-16,11.4559962546824,
-3.46944695195362E-15));
#55016=CARTESIAN_POINT('Origin',(-1.31921292845066E-15,11.4559962546824,
16.5));
#55017=CARTESIAN_POINT('Origin',(6.61363325216158E-15,88.645101838174,24.));
#55018=CARTESIAN_POINT('',(6.91979495194842E-15,52.,26.5));
#55019=CARTESIAN_POINT('Origin',(6.61363325216158E-15,52.,24.));
#55020=CARTESIAN_POINT('',(6.91979495194842E-15,57.,26.5));
#55021=CARTESIAN_POINT('',(6.91979495194842E-15,88.645101838174,26.5));
#55022=CARTESIAN_POINT('Origin',(6.61363325216158E-15,57.,24.));
#55023=CARTESIAN_POINT('Origin',(0.5,20.8180194846606,-32.6819805153395));
#55024=CARTESIAN_POINT('',(0.5,17.9895923599144,-32.6819805153395));
#55025=CARTESIAN_POINT('Origin',(0.5,19.4038059222875,-34.0961940777126));
#55026=CARTESIAN_POINT('',(0.5,19.4038059222875,-31.2677669529664));
#55027=CARTESIAN_POINT('',(0.5,19.4038059222875,-31.2677669529664));
#55028=CARTESIAN_POINT('Origin',(0.5,20.8180194846606,-32.6819805153395));
#55029=CARTESIAN_POINT('Origin',(4.5,24.,-35.));
#55030=CARTESIAN_POINT('Origin',(0.5,20.8180194846606,-32.6819805153395));
#55031=CARTESIAN_POINT('Origin',(23.,21.,6.));
#55032=CARTESIAN_POINT('Origin',(33.,26.9685342791486,5.07400811733573));
#55033=CARTESIAN_POINT('',(15.9496310351764,26.7715746300098,4.6144356021428));
#55034=CARTESIAN_POINT('Ctrl Pts',(16.6650252178836,27.3912430012986,4.80695505852849));
#55035=CARTESIAN_POINT('Ctrl Pts',(16.6630100761954,27.3903535292942,4.80554714514958));
#55036=CARTESIAN_POINT('Ctrl Pts',(16.6610051967559,27.3894616239388,4.80415074255901));
#55037=CARTESIAN_POINT('Ctrl Pts',(16.6589687547288,27.388548553701,4.80273701829963));
#55038=CARTESIAN_POINT('Ctrl Pts',(16.6569323127016,27.3876354834631,4.80132329404023));
#55039=CARTESIAN_POINT('Ctrl Pts',(16.6548961566558,27.3867154046794,4.79991437939278));
#55040=CARTESIAN_POINT('Ctrl Pts',(16.6528602685867,27.385788334266,4.79851028887233));
#55041=CARTESIAN_POINT('Ctrl Pts',(16.6487884924487,27.3839341934393,4.79570210783142));
#55042=CARTESIAN_POINT('Ctrl Pts',(16.6447177882178,27.3820520875034,4.79291322229783));
#55043=CARTESIAN_POINT('Ctrl Pts',(16.6406480126451,27.3801421344537,4.79014375984945));
#55044=CARTESIAN_POINT('Ctrl Pts',(16.6325084614997,27.3763222283545,4.78460483495268));
#55045=CARTESIAN_POINT('Ctrl Pts',(16.6243726249869,27.372390956667,4.7791435868405));
#55046=CARTESIAN_POINT('Ctrl Pts',(16.6162393697714,27.368348990199,4.7737612242166));
#55047=CARTESIAN_POINT('Ctrl Pts',(16.6081061145559,27.364307023731,4.7683788615927));
#55048=CARTESIAN_POINT('Ctrl Pts',(16.5999754406376,27.3601543628628,4.76307538424318));
#55049=CARTESIAN_POINT('Ctrl Pts',(16.5918462155288,27.3558913214684,4.75785226689918));
#55050=CARTESIAN_POINT('Ctrl Pts',(16.5837169904199,27.351628280074,4.75262914955517));
#55051=CARTESIAN_POINT('Ctrl Pts',(16.5755828927852,27.3472513208491,4.7474824908028));
#55052=CARTESIAN_POINT('Ctrl Pts',(16.5674672015749,27.34277402452,4.74242914788145));
#55053=CARTESIAN_POINT('Ctrl Pts',(16.5408797860593,27.3281061749427,4.72587414048764));
#55054=CARTESIAN_POINT('Ctrl Pts',(16.5144995283404,27.3123723786464,4.71032264739845));
#55055=CARTESIAN_POINT('Ctrl Pts',(16.4882866689286,27.2955991018421,4.69581689353952));
#55056=CARTESIAN_POINT('Ctrl Pts',(16.4824940898877,27.2918925038652,4.69261137809167));
#55057=CARTESIAN_POINT('Ctrl Pts',(16.4767096854409,27.2881350164069,4.68945708527442));
#55058=CARTESIAN_POINT('Ctrl Pts',(16.4709330265328,27.2843267278126,4.68635475495276));
#55059=CARTESIAN_POINT('Ctrl Pts',(16.4464825909653,27.2682076672312,4.67322375157423));
#55060=CARTESIAN_POINT('Ctrl Pts',(16.4221714637226,27.251181209635,4.6610210419516));
#55061=CARTESIAN_POINT('Ctrl Pts',(16.3979687202308,27.2332322814993,4.64982069702305));
#55062=CARTESIAN_POINT('Ctrl Pts',(16.3905773239509,27.2277507690131,4.64640016794677));
#55063=CARTESIAN_POINT('Ctrl Pts',(16.3831960361998,27.222183128309,4.6430734765975));
#55064=CARTESIAN_POINT('Ctrl Pts',(16.375823976153,27.2165287627257,4.63984370594838));
#55065=CARTESIAN_POINT('Ctrl Pts',(16.3679461041414,27.2104864396722,4.63639233419622));
#55066=CARTESIAN_POINT('Ctrl Pts',(16.3600787695375,27.2043448876271,4.63305150714274));
#55067=CARTESIAN_POINT('Ctrl Pts',(16.352220780091,27.1981025685342,4.62982527152944));
#55068=CARTESIAN_POINT('Ctrl Pts',(16.3443627906444,27.1918602494413,4.62659903591615));
#55069=CARTESIAN_POINT('Ctrl Pts',(16.336507501934,27.1855117252021,4.62348488529172));
#55070=CARTESIAN_POINT('Ctrl Pts',(16.3286750968802,27.179072825651,4.62049569144569));
#55071=CARTESIAN_POINT('Ctrl Pts',(16.3130102867726,27.1661950265487,4.61451730375362));
#55072=CARTESIAN_POINT('Ctrl Pts',(16.2975164416325,27.1530220764324,4.60906778525686));
#55073=CARTESIAN_POINT('Ctrl Pts',(16.2821841177728,27.139559361384,4.60416727061593));
#55074=CARTESIAN_POINT('Ctrl Pts',(16.2605485852015,27.1205620448264,4.59725212552117));
#55075=CARTESIAN_POINT('Ctrl Pts',(16.2392344529781,27.1009901681504,4.59142869627441));
#55076=CARTESIAN_POINT('Ctrl Pts',(16.2182190259903,27.0808433725107,4.58678469061224));
#55077=CARTESIAN_POINT('Ctrl Pts',(16.2094486983112,27.0724355490796,4.5848466166714));
#55078=CARTESIAN_POINT('Ctrl Pts',(16.200730393949,27.0639276706392,4.58311455657391));
#55079=CARTESIAN_POINT('Ctrl Pts',(16.1920624633548,27.0553203598125,4.58159754047634));
#55080=CARTESIAN_POINT('Ctrl Pts',(16.1773434663233,27.0407043010969,4.57902149822564));
#55081=CARTESIAN_POINT('Ctrl Pts',(16.162769897045,27.0257998208095,4.57706420508458));
#55082=CARTESIAN_POINT('Ctrl Pts',(16.1483338722369,27.0106028593833,4.57578102598377));
#55083=CARTESIAN_POINT('Ctrl Pts',(16.1411158598328,27.0030043786702,4.57513943643336));
#55084=CARTESIAN_POINT('Ctrl Pts',(16.1339322335463,26.9953327615401,4.57466662768078));
#55085=CARTESIAN_POINT('Ctrl Pts',(16.1267819344675,26.9875871364787,4.57437126058119));
#55086=CARTESIAN_POINT('Ctrl Pts',(16.1196316353886,26.9798415114174,4.5740758934816));
#55087=CARTESIAN_POINT('Ctrl Pts',(16.112507031152,26.9720133755952,4.57395805152907));
#55088=CARTESIAN_POINT('Ctrl Pts',(16.1054312238926,26.964128732385,4.57402752655474));
#55089=CARTESIAN_POINT('Ctrl Pts',(16.0871593099881,26.9437681549098,4.5742069324714));
#55090=CARTESIAN_POINT('Ctrl Pts',(16.0694041230973,26.9232488322717,4.57562785316267));
#55091=CARTESIAN_POINT('Ctrl Pts',(16.0521364611193,26.9026061632371,4.57837369204593));
#55092=CARTESIAN_POINT('Ctrl Pts',(16.0426564821845,26.8912732990742,4.57988116276228));
#55093=CARTESIAN_POINT('Ctrl Pts',(16.0333234447536,26.8799036284063,4.58178874960394));
#55094=CARTESIAN_POINT('Ctrl Pts',(16.0241325167303,26.8685069912516,4.58411573968941));
#55095=CARTESIAN_POINT('Ctrl Pts',(16.0111664730231,26.8524292573071,4.58739852626739));
#55096=CARTESIAN_POINT('Ctrl Pts',(15.9984836522186,26.8362950343224,4.59151528406382));
#55097=CARTESIAN_POINT('Ctrl Pts',(15.9860712395022,26.8201300060185,4.59653961395909));
#55098=CARTESIAN_POINT('Ctrl Pts',(15.9736588267857,26.8039649777146,4.60156394385436));
#55099=CARTESIAN_POINT('Ctrl Pts',(15.9615168221573,26.7877689169305,4.60749519358178));
#55100=CARTESIAN_POINT('Ctrl Pts',(15.9496310354892,26.771574629859,4.61443560232671));
#55101=CARTESIAN_POINT('',(33.,26.771574629859,4.6144356023267));
#55102=CARTESIAN_POINT('',(15.8907046022141,26.771574629859,4.6144356023267));
#55103=CARTESIAN_POINT('Origin',(33.,26.9685342791486,5.07400811733573));
#55104=CARTESIAN_POINT('Origin',(33.,25.7867763834111,2.31657302728156));
#55105=CARTESIAN_POINT('',(16.4143885868334,25.9837360327007,2.77614554229059));
#55106=CARTESIAN_POINT('',(33.,25.9837360327007,2.77614554229058));
#55107=CARTESIAN_POINT('',(33.,25.9837360327007,2.77614554229058));
#55108=CARTESIAN_POINT('Ctrl Pts',(16.4143885868334,25.9837360327007,2.77614554229059));
#55109=CARTESIAN_POINT('Ctrl Pts',(16.4633974984172,26.0470957947593,2.74899135855118));
#55110=CARTESIAN_POINT('Ctrl Pts',(16.5255478930996,26.1033294237433,2.70947695324141));
#55111=CARTESIAN_POINT('Ctrl Pts',(16.6761004083686,26.1963150747648,2.61126695343904));
#55112=CARTESIAN_POINT('Ctrl Pts',(16.7580192832196,26.2291178133552,2.55689292095467));
#55113=CARTESIAN_POINT('Ctrl Pts',(17.014944149898,26.2965251314195,2.38873820449799));
#55114=CARTESIAN_POINT('Ctrl Pts',(17.1872180079846,26.2925712666988,2.2799008816023));
#55115=CARTESIAN_POINT('Ctrl Pts',(17.3257575088157,26.2722073998847,2.19674998526149));
#55116=CARTESIAN_POINT('Ctrl Pts',(17.3277958722061,26.2719052005207,2.19553219265278));
#55117=CARTESIAN_POINT('Ctrl Pts',(17.3292733299329,26.2716827465251,2.19464747699608));
#55118=CARTESIAN_POINT('Origin',(33.,25.7867763834111,2.31657302728156));
#55119=CARTESIAN_POINT('Origin',(16.0330469265826,57.,-13.5625));
#55120=CARTESIAN_POINT('',(16.0330469265826,57.,-13.5625));
#55121=CARTESIAN_POINT('',(16.0330469265826,53.,-13.5625));
#55122=CARTESIAN_POINT('',(16.0330469265826,57.,-13.5625));
#55123=CARTESIAN_POINT('',(16.0330469265826,53.,-13.5625));
#55124=CARTESIAN_POINT('',(16.0330469265826,57.,-13.5625));
#55125=CARTESIAN_POINT('Origin',(6.61287431064084E-15,57.,0.));
#55126=CARTESIAN_POINT('',(16.0330469265826,57.,13.5625));
#55127=CARTESIAN_POINT('',(16.0330469265826,53.,13.5625));
#55128=CARTESIAN_POINT('',(16.0330469265826,57.,13.5625));
#55129=CARTESIAN_POINT('Origin',(6.61287431064084E-15,53.,0.));
#55130=CARTESIAN_POINT('Origin',(6.61287431064084E-15,57.,0.));
#55131=CARTESIAN_POINT('Origin',(6.61363325216158E-15,57.,24.));
#55132=CARTESIAN_POINT('',(4.1991313379145,57.,27.5520833333334));
#55133=CARTESIAN_POINT('',(-4.19913133791448,57.,27.5520833333334));
#55134=CARTESIAN_POINT('Origin',(6.61363325216158E-15,57.,24.));
#55135=CARTESIAN_POINT('',(4.1991313379145,57.,27.5520833333334));
#55136=CARTESIAN_POINT('',(-16.0330469265826,57.,-13.5625));
#55137=CARTESIAN_POINT('',(-4.19913133791448,57.,-27.5520833333334));
#55138=CARTESIAN_POINT('',(-16.0330469265826,57.,13.5625));
#55139=CARTESIAN_POINT('Origin',(6.61287431064084E-15,57.,0.));
#55140=CARTESIAN_POINT('',(-4.19913133791448,57.,27.5520833333334));
#55141=CARTESIAN_POINT('Origin',(4.1991313379145,57.,27.5520833333334));
#55142=CARTESIAN_POINT('',(4.1991313379145,53.,27.5520833333334));
#55143=CARTESIAN_POINT('',(4.1991313379145,57.,27.5520833333334));
#55144=CARTESIAN_POINT('',(4.1991313379145,53.,27.5520833333334));
#55145=CARTESIAN_POINT('Origin',(6.61363325216158E-15,57.,24.));
#55146=CARTESIAN_POINT('',(-4.19913133791448,53.,27.5520833333334));
#55147=CARTESIAN_POINT('',(-4.19913133791448,57.,27.5520833333334));
#55148=CARTESIAN_POINT('Origin',(6.61363325216158E-15,53.,24.));
#55149=CARTESIAN_POINT('Origin',(-4.19913133791448,57.,27.5520833333334));
#55150=CARTESIAN_POINT('',(-16.0330469265826,53.,13.5625));
#55151=CARTESIAN_POINT('',(-16.0330469265826,57.,13.5625));
#55152=CARTESIAN_POINT('',(-4.19913133791448,53.,27.5520833333334));
#55153=CARTESIAN_POINT('Origin',(6.61287431064084E-15,57.,0.));
#55154=CARTESIAN_POINT('',(-16.0330469265826,53.,-13.5625));
#55155=CARTESIAN_POINT('',(-16.0330469265826,57.,-13.5625));
#55156=CARTESIAN_POINT('Origin',(6.61287431064084E-15,53.,0.));
#55157=CARTESIAN_POINT('Origin',(-38.,21.,7.));
#55158=CARTESIAN_POINT('',(-38.,23.6912516952905,7.08464226247173));
#55159=CARTESIAN_POINT('Ctrl Pts',(-16.5433923268431,19.8911992509365,0.971393813304918));
#55160=CARTESIAN_POINT('Ctrl Pts',(-16.407897387297,20.5,0.963437830432189));
#55161=CARTESIAN_POINT('Ctrl Pts',(-17.0305720504421,20.5,1.));
#55162=CARTESIAN_POINT('Ctrl Pts',(-16.5460230165557,19.891199259935,0.926591628387505));
#55163=CARTESIAN_POINT('Ctrl Pts',(-16.4084072798099,20.5016889125451,0.948330479285953));
#55164=CARTESIAN_POINT('Ctrl Pts',(-17.0332802188509,20.5,0.976939153062529));
#55165=CARTESIAN_POINT('Ctrl Pts',(-16.5475841116722,19.8950096166727,0.882278171409564));
#55166=CARTESIAN_POINT('Ctrl Pts',(-16.4096816508543,20.5038083386403,0.933858336274406));
#55167=CARTESIAN_POINT('Ctrl Pts',(-17.0350550463224,20.5015876519666,0.954134911206445));
#55168=CARTESIAN_POINT('Ctrl Pts',(-16.5487479801528,19.909965914742,0.794606678521227));
#55169=CARTESIAN_POINT('Ctrl Pts',(-16.4137261112856,20.5090429824563,0.904356864073263));
#55170=CARTESIAN_POINT('Ctrl Pts',(-17.0368945748498,20.5078194436758,0.909023217144905));
#55171=CARTESIAN_POINT('Ctrl Pts',(-16.5483503357205,19.9211125982883,0.751247887293482));
#55172=CARTESIAN_POINT('Ctrl Pts',(-16.4164789427531,20.5121455900044,0.889404076489988));
#55173=CARTESIAN_POINT('Ctrl Pts',(-17.0369589041897,20.5124638957006,0.88671544260711));
#55174=CARTESIAN_POINT('Ctrl Pts',(-16.5467905191782,19.9397158472753,0.697663995679634));
#55175=CARTESIAN_POINT('Ctrl Pts',(-16.4206834264394,20.5171906160361,0.869517502731721));
#55176=CARTESIAN_POINT('Ctrl Pts',(-17.0361078121662,20.5202152482318,0.859147613733574));
#55177=CARTESIAN_POINT('Ctrl Pts',(-16.5464256319663,19.9436710140189,0.686978084831627));
#55178=CARTESIAN_POINT('Ctrl Pts',(-16.4215581463202,20.5182547550123,0.865499434449415));
#55179=CARTESIAN_POINT('Ctrl Pts',(-17.0358911926661,20.5218632349471,0.853649964743502));
#55180=CARTESIAN_POINT('Ctrl Pts',(-16.545594966273,19.9520567304156,0.665669029571539));
#55181=CARTESIAN_POINT('Ctrl Pts',(-16.4233747022659,20.5205189452442,0.857341577641165));
#55182=CARTESIAN_POINT('Ctrl Pts',(-17.0353693593641,20.5253572827868,0.842686968399742));
#55183=CARTESIAN_POINT('Ctrl Pts',(-16.5451281146306,19.9564966696759,0.655025666938477));
#55184=CARTESIAN_POINT('Ctrl Pts',(-16.4243180509428,20.5217209530893,0.853195047255348));
#55185=CARTESIAN_POINT('Ctrl Pts',(-17.0350633970533,20.5272072572878,0.837211219553851));
#55186=CARTESIAN_POINT('Ctrl Pts',(-16.5435950680448,19.9704461060348,0.623402194616967));
#55187=CARTESIAN_POINT('Ctrl Pts',(-16.4272156936075,20.5255308654207,0.840655045305963));
#55188=CARTESIAN_POINT('Ctrl Pts',(-17.0340268420252,20.5330195239982,0.820941647960808));
#55189=CARTESIAN_POINT('Ctrl Pts',(-16.5423960960644,19.9805919436888,0.602698030449193));
#55190=CARTESIAN_POINT('Ctrl Pts',(-16.4292443604542,20.5283496476911,0.832125812433268));
#55191=CARTESIAN_POINT('Ctrl Pts',(-17.0331776130024,20.5372469546676,0.810289716104096));
#55192=CARTESIAN_POINT('Ctrl Pts',(-16.5383740427822,20.0135045500505,0.541688220646475));
#55193=CARTESIAN_POINT('Ctrl Pts',(-16.4355081831529,20.5378206889875,0.806060489096857));
#55194=CARTESIAN_POINT('Ctrl Pts',(-17.0302461821317,20.5509605425891,0.778900346429098));
#55195=CARTESIAN_POINT('Ctrl Pts',(-16.5351244462826,20.0387346852731,0.502480294969622));
#55196=CARTESIAN_POINT('Ctrl Pts',(-16.4399382995849,20.5455007368547,0.78792924810244));
#55197=CARTESIAN_POINT('Ctrl Pts',(-17.0277791213822,20.5614730977609,0.758726732122362));
#55198=CARTESIAN_POINT('Ctrl Pts',(-16.5298329930104,20.0814825069704,0.445834797421413));
#55199=CARTESIAN_POINT('Ctrl Pts',(-16.4467056213962,20.5599852183674,0.759646126498156));
#55200=CARTESIAN_POINT('Ctrl Pts',(-17.0236814376451,20.5792846899537,0.729577577968062));
#55201=CARTESIAN_POINT('Ctrl Pts',(-16.5279999224092,20.0965518409253,0.427315285485088));
#55202=CARTESIAN_POINT('Ctrl Pts',(-16.4489689372401,20.5652690924714,0.750102567161397));
#55203=CARTESIAN_POINT('Ctrl Pts',(-17.0222495454306,20.585563579545,0.72004706252039));
#55204=CARTESIAN_POINT('Ctrl Pts',(-16.5252050045946,20.1204096270575,0.400087134515338));
#55205=CARTESIAN_POINT('Ctrl Pts',(-16.4523742507172,20.5740318567946,0.735583389128628));
#55206=CARTESIAN_POINT('Ctrl Pts',(-17.0200525657724,20.5955043231922,0.706033937512207));
#55207=CARTESIAN_POINT('Ctrl Pts',(-16.5242658526117,20.1285713796292,0.391103018058698));
#55208=CARTESIAN_POINT('Ctrl Pts',(-16.4535078916128,20.5770823745325,0.730724230937434));
#55209=CARTESIAN_POINT('Ctrl Pts',(-17.0193120752144,20.5989050538913,0.701410047075698));
#55210=CARTESIAN_POINT('Ctrl Pts',(-16.5223828507085,20.1453196286114,0.373320964386736));
#55211=CARTESIAN_POINT('Ctrl Pts',(-16.4557745374995,20.5834720397517,0.720959701653889));
#55212=CARTESIAN_POINT('Ctrl Pts',(-17.0178235516284,20.6058834904285,0.692257749627275));
#55213=CARTESIAN_POINT('Ctrl Pts',(-16.5214408462345,20.1538906455271,0.364540612191054));
#55214=CARTESIAN_POINT('Ctrl Pts',(-16.4569053132703,20.5868043886051,0.716064040471107));
#55215=CARTESIAN_POINT('Ctrl Pts',(-17.0170769643931,20.6094547473659,0.687738393835301));
#55216=CARTESIAN_POINT('Ctrl Pts',(-16.5167801741158,20.1974911117525,0.321422255422651));
#55217=CARTESIAN_POINT('Ctrl Pts',(-16.4624823349259,20.6039933346536,0.691819606845547));
#55218=CARTESIAN_POINT('Ctrl Pts',(-17.0133752701266,20.6276216101941,0.665544000743011));
#55219=CARTESIAN_POINT('Ctrl Pts',(-16.5131856715377,20.2349569684753,0.289196318408042));
#55220=CARTESIAN_POINT('Ctrl Pts',(-16.4668466775319,20.6198679793505,0.672490019195905));
#55221=CARTESIAN_POINT('Ctrl Pts',(-17.0104951031623,20.6432323821084,0.648953506162977));
#55222=CARTESIAN_POINT('Ctrl Pts',(-16.5069251772217,20.3149416326476,0.229133699455863));
#55223=CARTESIAN_POINT('Ctrl Pts',(-16.475404952459,20.6561212773607,0.63516338539478));
#55224=CARTESIAN_POINT('Ctrl Pts',(-17.0054632578451,20.6765593259124,0.618027613096065));
#55225=CARTESIAN_POINT('Ctrl Pts',(-16.5042566734341,20.3574602973108,0.201297028703423));
#55226=CARTESIAN_POINT('Ctrl Pts',(-16.4796079694452,20.676460019731,0.617125809267408));
#55227=CARTESIAN_POINT('Ctrl Pts',(-17.0033094070265,20.6942754368156,0.603692232152243));
#55228=CARTESIAN_POINT('Ctrl Pts',(-16.5014702539652,20.4251655989665,0.162918760220545));
#55229=CARTESIAN_POINT('Ctrl Pts',(-16.4859952506699,20.7105903622794,0.591789565823027));
#55230=CARTESIAN_POINT('Ctrl Pts',(-17.0010678009979,20.7224859779327,0.583925720088675));
#55231=CARTESIAN_POINT('Ctrl Pts',(-16.5007448950925,20.4484653982754,0.150660370006624));
#55232=CARTESIAN_POINT('Ctrl Pts',(-16.488138164386,20.7225596194786,0.583636449987115));
#55233=CARTESIAN_POINT('Ctrl Pts',(-17.0004860701606,20.732194227621,0.577611671372152));
#55234=CARTESIAN_POINT('Ctrl Pts',(-16.4998065086035,20.4956762612484,0.127659535369717));
#55235=CARTESIAN_POINT('Ctrl Pts',(-16.4924238463118,20.7472907980385,0.568298316995553));
#55236=CARTESIAN_POINT('Ctrl Pts',(-16.9997422762988,20.7518654214002,0.565763816818942));
#55237=CARTESIAN_POINT('Ctrl Pts',(-16.4995891679361,20.5196569119538,0.116872129943027));
#55238=CARTESIAN_POINT('Ctrl Pts',(-16.4945751007252,20.7600913803133,0.561073592164906));
#55239=CARTESIAN_POINT('Ctrl Pts',(-16.9995767220622,20.7618573347902,0.560206868064739));
#55240=CARTESIAN_POINT('Ctrl Pts',(-16.499654466181,20.5440037453176,0.106782473437618));
#55241=CARTESIAN_POINT('Ctrl Pts',(-16.4967580121734,20.7733226724976,0.554332420210066));
#55242=CARTESIAN_POINT('Ctrl Pts',(-16.9996439954592,20.7720018726588,0.555009152983015));
#55243=CARTESIAN_POINT('Origin',(-16.9996439954592,20.5440037453176,0.110018305966033));
#55244=CARTESIAN_POINT('Ctrl Pts',(-16.5433923268431,19.8911992509365,0.971393813304911));
#55245=CARTESIAN_POINT('Ctrl Pts',(-16.5460324658657,19.8911992599673,0.926430701110204));
#55246=CARTESIAN_POINT('Ctrl Pts',(-16.5475861334947,19.895035620538,0.882125735271342));
#55247=CARTESIAN_POINT('Ctrl Pts',(-16.5481658959472,19.9024884294234,0.83844251359447));
#55248=CARTESIAN_POINT('Ctrl Pts',(-16.5482102764594,19.9030589380404,0.835098585852582));
#55249=CARTESIAN_POINT('Ctrl Pts',(-16.5482489443743,19.9036506508715,0.831758298116806));
#55250=CARTESIAN_POINT('Ctrl Pts',(-16.5482819658505,19.9042635663159,0.828421646010209));
#55251=CARTESIAN_POINT('Ctrl Pts',(-16.5485141637358,19.9085734181441,0.804959231555224));
#55252=CARTESIAN_POINT('Ctrl Pts',(-16.5484668356028,19.9139332687769,0.781677203367974));
#55253=CARTESIAN_POINT('Ctrl Pts',(-16.548163843894,19.9203370163541,0.758574853429922));
#55254=CARTESIAN_POINT('Ctrl Pts',(-16.5480123480396,19.9235388901426,0.747023678460895));
#55255=CARTESIAN_POINT('Ctrl Pts',(-16.5477968713962,19.9270019786639,0.735517459337272));
#55256=CARTESIAN_POINT('Ctrl Pts',(-16.5475200008255,19.930727105518,0.724056384611012));
#55257=CARTESIAN_POINT('Ctrl Pts',(-16.5473935804081,19.9324280161282,0.718823203468597));
#55258=CARTESIAN_POINT('Ctrl Pts',(-16.5472542508089,19.934184833772,0.713595822387411));
#55259=CARTESIAN_POINT('Ctrl Pts',(-16.5471024601299,19.9359952994074,0.708380803007421));
#55260=CARTESIAN_POINT('Ctrl Pts',(-16.5469218173869,19.9381498946732,0.702174523336911));
#55261=CARTESIAN_POINT('Ctrl Pts',(-16.5467235931023,19.9403808422703,0.695985801536031));
#55262=CARTESIAN_POINT('Ctrl Pts',(-16.5465088555626,19.9426837122906,0.689825608166473));
#55263=CARTESIAN_POINT('Ctrl Pts',(-16.5463513980074,19.9443723051828,0.685308610400069));
#55264=CARTESIAN_POINT('Ctrl Pts',(-16.5461851308859,19.9460989058903,0.68080855796723));
#55265=CARTESIAN_POINT('Ctrl Pts',(-16.5460102979366,19.9478638776901,0.676323558973994));
#55266=CARTESIAN_POINT('Ctrl Pts',(-16.5457463457432,19.9505285251712,0.669552379246432));
#55267=CARTESIAN_POINT('Ctrl Pts',(-16.5454624471804,19.953284362771,0.662807405302023));
#55268=CARTESIAN_POINT('Ctrl Pts',(-16.5451605304242,19.9561229704575,0.656105186271793));
#55269=CARTESIAN_POINT('Ctrl Pts',(-16.5449852593692,19.9577708609899,0.652214362140303));
#55270=CARTESIAN_POINT('Ctrl Pts',(-16.544803981033,19.9594459793856,0.648339654550236));
#55271=CARTESIAN_POINT('Ctrl Pts',(-16.5446170815428,19.9611465644699,0.644484539592544));
#55272=CARTESIAN_POINT('Ctrl Pts',(-16.5442687863734,19.964315677287,0.637300368487396));
#55273=CARTESIAN_POINT('Ctrl Pts',(-16.5439009460353,19.9675739823819,0.630180634746881));
#55274=CARTESIAN_POINT('Ctrl Pts',(-16.5435149788688,19.9709216245128,0.623118586715854));
#55275=CARTESIAN_POINT('Ctrl Pts',(-16.5427600892517,19.9774690733777,0.609306358121234));
#55276=CARTESIAN_POINT('Ctrl Pts',(-16.5419362971708,19.9843543605266,0.595724100296492));
#55277=CARTESIAN_POINT('Ctrl Pts',(-16.5410553222413,19.9915632524549,0.582361623576685));
#55278=CARTESIAN_POINT('Ctrl Pts',(-16.5405520145231,19.9956817475735,0.574727538381498));
#55279=CARTESIAN_POINT('Ctrl Pts',(-16.5400299818145,19.9999054727865,0.567165025052416));
#55280=CARTESIAN_POINT('Ctrl Pts',(-16.53949136959,20.0042328969111,0.559672683798894));
#55281=CARTESIAN_POINT('Ctrl Pts',(-16.5371210098482,20.0232773067176,0.52669990065196));
#55282=CARTESIAN_POINT('Ctrl Pts',(-16.5344328843906,20.0443209958337,0.495080232313346));
#55283=CARTESIAN_POINT('Ctrl Pts',(-16.5315967308495,20.0672336806369,0.464716909039771));
#55284=CARTESIAN_POINT('Ctrl Pts',(-16.530887911956,20.0729600786099,0.457128428058937));
#55285=CARTESIAN_POINT('Ctrl Pts',(-16.5301697840599,20.078803778894,0.449618679050732));
#55286=CARTESIAN_POINT('Ctrl Pts',(-16.5294449711324,20.0847640692831,0.4421867484608));
#55287=CARTESIAN_POINT('Ctrl Pts',(-16.5283543136099,20.093732777349,0.431003599406807));
#55288=CARTESIAN_POINT('Ctrl Pts',(-16.5272486400087,20.1029648268381,0.419996611718037));
#55289=CARTESIAN_POINT('Ctrl Pts',(-16.5261366293535,20.1124571205592,0.409163249025999));
#55290=CARTESIAN_POINT('Ctrl Pts',(-16.5254006736455,20.1187393515012,0.401993466009371));
#55291=CARTESIAN_POINT('Ctrl Pts',(-16.5246619587109,20.125135694536,0.394899784876159));
#55292=CARTESIAN_POINT('Ctrl Pts',(-16.5239230422738,20.1316458538301,0.38788173218008));
#55293=CARTESIAN_POINT('Ctrl Pts',(-16.5237234984912,20.1334039170503,0.385986512759983));
#55294=CARTESIAN_POINT('Ctrl Pts',(-16.523523911521,20.1351705286926,0.384096538884203));
#55295=CARTESIAN_POINT('Ctrl Pts',(-16.5233243509668,20.1369455085955,0.382211994691331));
#55296=CARTESIAN_POINT('Ctrl Pts',(-16.5225961332083,20.1434225996812,0.375335091819148));
#55297=CARTESIAN_POINT('Ctrl Pts',(-16.5218693863997,20.1500018836066,0.368541134605226));
#55298=CARTESIAN_POINT('Ctrl Pts',(-16.5211497942102,20.1566507251102,0.361858850291119));
#55299=CARTESIAN_POINT('Ctrl Pts',(-16.5209355163636,20.1586305957379,0.359869021170887));
#55300=CARTESIAN_POINT('Ctrl Pts',(-16.5207217743018,20.1606175258447,0.35788820461828));
#55301=CARTESIAN_POINT('Ctrl Pts',(-16.5205086998133,20.1626108208916,0.355917009055417));
#55302=CARTESIAN_POINT('Ctrl Pts',(-16.5198101338809,20.1691458501336,0.349454433098762));
#55303=CARTESIAN_POINT('Ctrl Pts',(-16.5191179110668,20.1757563528476,0.343086927086753));
#55304=CARTESIAN_POINT('Ctrl Pts',(-16.5184344300571,20.1824373565126,0.336815925899807));
#55305=CARTESIAN_POINT('Ctrl Pts',(-16.5154181393187,20.2119214960751,0.309141180687308));
#55306=CARTESIAN_POINT('Ctrl Pts',(-16.5125720762524,20.2427958934596,0.283311277070422));
#55307=CARTESIAN_POINT('Ctrl Pts',(-16.510055328672,20.2749501941091,0.259165979639789));
#55308=CARTESIAN_POINT('Ctrl Pts',(-16.5095951431617,20.2808295851809,0.254751029127042));
#55309=CARTESIAN_POINT('Ctrl Pts',(-16.5091458580602,20.2867518129195,0.2503924601709));
#55310=CARTESIAN_POINT('Ctrl Pts',(-16.5087084339304,20.29271673787,0.246089778989223));
#55311=CARTESIAN_POINT('Ctrl Pts',(-16.5061295101034,20.3278841784264,0.220722438084665));
#55312=CARTESIAN_POINT('Ctrl Pts',(-16.5039651443336,20.3645429559342,0.197285361633269));
#55313=CARTESIAN_POINT('Ctrl Pts',(-16.5023990236787,20.4025977542277,0.17571235928992));
#55314=CARTESIAN_POINT('Ctrl Pts',(-16.5022467391559,20.4062980801142,0.173614670099621));
#55315=CARTESIAN_POINT('Ctrl Pts',(-16.502100105633,20.4100136575059,0.17153383559746));
#55316=CARTESIAN_POINT('Ctrl Pts',(-16.5019593154156,20.4137424636006,0.169470743535446));
#55317=CARTESIAN_POINT('Ctrl Pts',(-16.5015621400589,20.4242615885576,0.163650670662964));
#55318=CARTESIAN_POINT('Ctrl Pts',(-16.501210954272,20.4348995025215,0.157964972318453));
#55319=CARTESIAN_POINT('Ctrl Pts',(-16.5009103026471,20.4456137584343,0.152432928451714));
#55320=CARTESIAN_POINT('Ctrl Pts',(-16.5006642210316,20.454383314908,0.147904982554238));
#55321=CARTESIAN_POINT('Ctrl Pts',(-16.5004519129355,20.463205509022,0.143479117894903));
#55322=CARTESIAN_POINT('Ctrl Pts',(-16.5002757006572,20.4720708611006,0.139160004757658));
#55323=CARTESIAN_POINT('Ctrl Pts',(-16.500236624574,20.4740368037643,0.138202216650574));
#55324=CARTESIAN_POINT('Ctrl Pts',(-16.5001992951787,20.4760053545502,0.137249370747565));
#55325=CARTESIAN_POINT('Ctrl Pts',(-16.5001637279027,20.4779766555572,0.136301387950723));
#55326=CARTESIAN_POINT('Ctrl Pts',(-16.499771814489,20.4996982882644,0.12585562951363));
#55327=CARTESIAN_POINT('Ctrl Pts',(-16.4995946736473,20.5217097527716,0.11602140670495));
#55328=CARTESIAN_POINT('Ctrl Pts',(-16.499654466181,20.5440037453176,0.106782473437692));
#55329=CARTESIAN_POINT('Ctrl Pts',(-28.4921884404488,20.1587841073205,4.48858136870839));
#55330=CARTESIAN_POINT('Ctrl Pts',(-28.4940712295089,20.5,4.37432217737224));
#55331=CARTESIAN_POINT('Ctrl Pts',(-28.5000000000009,20.5,4.01452801010852));
#55332=CARTESIAN_POINT('Ctrl Pts',(-24.4459493854662,20.1555956263289,4.42297449836793));
#55333=CARTESIAN_POINT('Ctrl Pts',(-24.43798817446,20.5,4.31004373441984));
#55334=CARTESIAN_POINT('Ctrl Pts',(-24.4537608788502,20.5,3.94785315837506));
#55335=CARTESIAN_POINT('Ctrl Pts',(-20.3997065615446,20.152598599004,4.35749244459499));
#55336=CARTESIAN_POINT('Ctrl Pts',(-20.392720406832,20.5,4.24601800956522));
#55337=CARTESIAN_POINT('Ctrl Pts',(-20.4075180616586,20.5,3.8814026561495));
#55338=CARTESIAN_POINT('Ctrl Pts',(-16.353460662545,20.1497621460669,4.29211722911022));
#55339=CARTESIAN_POINT('Ctrl Pts',(-16.3552611303492,20.5,4.18217914609945));
#55340=CARTESIAN_POINT('Ctrl Pts',(-16.3612722214407,20.5,3.81513685304315));
#55341=CARTESIAN_POINT('Ctrl Pts',(-16.6268429955203,20.5,3.81948640102502));
#55342=CARTESIAN_POINT('Ctrl Pts',(-20.5845651132323,20.5,3.88431036677466));
#55343=CARTESIAN_POINT('Ctrl Pts',(-24.5422843246593,20.5,3.94931186830211));
#55344=CARTESIAN_POINT('Ctrl Pts',(-28.5,20.5,4.01452801010866));
#55345=CARTESIAN_POINT('Ctrl Pts',(-17.2867685703854,20.1504190344619,4.30719696626493));
#55346=CARTESIAN_POINT('Ctrl Pts',(-17.2686590325533,20.1588563948581,4.30423831313666));
#55347=CARTESIAN_POINT('Ctrl Pts',(-17.2506684453864,20.1671804561454,4.30107402084104));
#55348=CARTESIAN_POINT('Ctrl Pts',(-17.1042449506796,20.2339840890514,4.27363942811962));
#55349=CARTESIAN_POINT('Ctrl Pts',(-16.9731490285154,20.2896863690097,4.23809161586893));
#55350=CARTESIAN_POINT('Ctrl Pts',(-16.6906483986079,20.399246275303,4.13270660898505));
#55351=CARTESIAN_POINT('Ctrl Pts',(-16.5477523533627,20.4474978177044,4.05836797170915));
#55352=CARTESIAN_POINT('Ctrl Pts',(-16.431123175528,20.4751899387349,3.97184757185369));
#55353=CARTESIAN_POINT('Origin',(-28.5,20.,4.01452801010857));
#55354=CARTESIAN_POINT('Ctrl Pts',(-28.4921884534997,21.8412135273285,4.48858057664302));
#55355=CARTESIAN_POINT('Ctrl Pts',(-28.4940712607011,21.5,4.37432028438836));
#55356=CARTESIAN_POINT('Ctrl Pts',(-28.5,21.5,4.01452801010865));
#55357=CARTESIAN_POINT('Ctrl Pts',(-28.5254209870357,21.8411873349216,4.48911941663496));
#55358=CARTESIAN_POINT('Ctrl Pts',(-28.5146908680549,21.5001969822507,4.37470508095403));
#55359=CARTESIAN_POINT('Ctrl Pts',(-28.5166162662214,21.5,4.01507562146144));
#55360=CARTESIAN_POINT('Ctrl Pts',(-28.5583612383751,21.8397714826907,4.48918675379326));
#55361=CARTESIAN_POINT('Ctrl Pts',(-28.535159969218,21.499164542665,4.37488527730213));
#55362=CARTESIAN_POINT('Ctrl Pts',(-28.5330863925031,21.4991738788987,4.01506355035577));
#55363=CARTESIAN_POINT('Ctrl Pts',(-28.6236777750892,21.8342637186865,4.48842670530818));
#55364=CARTESIAN_POINT('Ctrl Pts',(-28.5755649619896,21.4947581941247,4.37486259947081));
#55365=CARTESIAN_POINT('Ctrl Pts',(-28.5657446607293,21.495930348264,4.01397708967205));
#55366=CARTESIAN_POINT('Ctrl Pts',(-28.6560542665336,21.8301715190968,4.48759926621887));
#55367=CARTESIAN_POINT('Ctrl Pts',(-28.5955312938426,21.4913781502374,4.37465937506852));
#55368=CARTESIAN_POINT('Ctrl Pts',(-28.5819329064879,21.4935127684286,4.01290263291554));
#55369=CARTESIAN_POINT('Ctrl Pts',(-28.7202499315746,21.8193320805794,4.48509841768535));
#55370=CARTESIAN_POINT('Ctrl Pts',(-28.6347751662465,21.4823684641649,4.37391749566476));
#55371=CARTESIAN_POINT('Ctrl Pts',(-28.6140307390665,21.4870983928484,4.00974907485253));
#55372=CARTESIAN_POINT('Ctrl Pts',(-28.7520691233355,21.8125849450047,4.48342495569087));
#55373=CARTESIAN_POINT('Ctrl Pts',(-28.6540799499148,21.47672616809,4.37337748925145));
#55374=CARTESIAN_POINT('Ctrl Pts',(-28.6299403346358,21.4831016592162,4.00766990484807));
#55375=CARTESIAN_POINT('Ctrl Pts',(-28.7993731038122,21.8004300668428,4.4803184744276));
#55376=CARTESIAN_POINT('Ctrl Pts',(-28.6823709564734,21.4666385444995,4.37236633380816));
#55377=CARTESIAN_POINT('Ctrl Pts',(-28.6535923252973,21.4758963369637,4.00384291003086));
#55378=CARTESIAN_POINT('Ctrl Pts',(-28.8151137135972,21.7960246635793,4.47917993735541));
#55379=CARTESIAN_POINT('Ctrl Pts',(-28.6917346273236,21.4629852312693,4.37199383821505));
#55380=CARTESIAN_POINT('Ctrl Pts',(-28.6614626302949,21.4732841092092,4.00244472483011));
#55381=CARTESIAN_POINT('Ctrl Pts',(-28.8461585861444,21.7866115397394,4.47673486071072));
#55382=CARTESIAN_POINT('Ctrl Pts',(-28.7100601376562,21.4552142843188,4.37119916143592));
#55383=CARTESIAN_POINT('Ctrl Pts',(-28.6769850660762,21.4677010962118,3.99944965879431));
#55384=CARTESIAN_POINT('Ctrl Pts',(-28.8614762447451,21.7816027460074,4.47542812825129));
#55385=CARTESIAN_POINT('Ctrl Pts',(-28.7190324938991,21.4510933302668,4.37077668089638));
#55386=CARTESIAN_POINT('Ctrl Pts',(-28.6846438958177,21.4647296831086,3.99785250652423));
#55387=CARTESIAN_POINT('Ctrl Pts',(-28.9068305655355,21.7656885765681,4.47127862320908));
#55388=CARTESIAN_POINT('Ctrl Pts',(-28.7454005836816,21.4380588957433,4.36945208065789));
#55389=CARTESIAN_POINT('Ctrl Pts',(-28.7073210556279,21.4552869055806,3.99278981369038));
#55390=CARTESIAN_POINT('Ctrl Pts',(-28.9362700223319,21.7538976633587,4.46820672183587));
#55391=CARTESIAN_POINT('Ctrl Pts',(-28.7621839351622,21.4284950526857,4.36849519695348));
#55392=CARTESIAN_POINT('Ctrl Pts',(-28.7220407844993,21.4482883513904,3.9890532279118));
#55393=CARTESIAN_POINT('Ctrl Pts',(-28.9936013918011,21.7279957199606,4.46156954348255));
#55394=CARTESIAN_POINT('Ctrl Pts',(-28.7941394198094,21.4078545566988,4.36653621615206));
#55395=CARTESIAN_POINT('Ctrl Pts',(-28.7507064690675,21.4329097161546,3.98099696960699));
#55396=CARTESIAN_POINT('Ctrl Pts',(-29.0214932534172,21.7138846523769,4.45800409484777));
#55397=CARTESIAN_POINT('Ctrl Pts',(-28.809316572376,21.3967577837743,4.36553299161296));
#55398=CARTESIAN_POINT('Ctrl Pts',(-28.7646523995967,21.4245296160374,3.9766770804571));
#55399=CARTESIAN_POINT('Ctrl Pts',(-29.062169897947,21.6909554930138,4.45237100283138));
#55400=CARTESIAN_POINT('Ctrl Pts',(-28.8307957370868,21.3791608345931,4.36406993139224));
#55401=CARTESIAN_POINT('Ctrl Pts',(-28.7849907224046,21.4109097954778,3.96986112065059));
#55402=CARTESIAN_POINT('Ctrl Pts',(-29.075534899249,21.6830181207054,4.45044580430147));
#55403=CARTESIAN_POINT('Ctrl Pts',(-28.8377611399515,21.3731163751088,4.36358768640991));
#55404=CARTESIAN_POINT('Ctrl Pts',(-28.7916732225539,21.4061945771178,3.96753309139709));
#55405=CARTESIAN_POINT('Ctrl Pts',(-29.0952881820098,21.6706624712522,4.44749745570096));
#55406=CARTESIAN_POINT('Ctrl Pts',(-28.8478828377938,21.3638285391936,4.36288328557115));
#55407=CARTESIAN_POINT('Ctrl Pts',(-28.8015498644154,21.3988539896752,3.96396973058805));
#55408=CARTESIAN_POINT('Ctrl Pts',(-29.1018282853599,21.6664655673196,4.44650380913622));
#55409=CARTESIAN_POINT('Ctrl Pts',(-28.8512095441988,21.3606882699083,4.36265113339823));
#55410=CARTESIAN_POINT('Ctrl Pts',(-28.8048199161347,21.3963604667832,3.9627691229626));
#55411=CARTESIAN_POINT('Ctrl Pts',(-29.1147425825927,21.6579651097018,4.44450864515904));
#55412=CARTESIAN_POINT('Ctrl Pts',(-28.8577231856397,21.3543668875625,4.3621966351092));
#55413=CARTESIAN_POINT('Ctrl Pts',(-28.8112770643419,21.3913098390223,3.96035897683085));
#55414=CARTESIAN_POINT('Ctrl Pts',(-29.1211247277383,21.6536567486803,4.44350596775694));
#55415=CARTESIAN_POINT('Ctrl Pts',(-28.8609140856392,21.351181922773,4.36197401207208));
#55416=CARTESIAN_POINT('Ctrl Pts',(-28.8144681372952,21.3887498797035,3.95914803253197));
#55417=CARTESIAN_POINT('Ctrl Pts',(-29.1526652448549,21.631827005439,4.43847235110778));
#55418=CARTESIAN_POINT('Ctrl Pts',(-28.8765929641311,21.3350979442923,4.36088339644741));
#55419=CARTESIAN_POINT('Ctrl Pts',(-28.8302383949739,21.3757784666252,3.95307020188013));
#55420=CARTESIAN_POINT('Ctrl Pts',(-29.1767159566876,21.6134440801678,4.43438108172183));
#55421=CARTESIAN_POINT('Ctrl Pts',(-28.8880537416351,21.3219144059112,4.3600980840368));
#55422=CARTESIAN_POINT('Ctrl Pts',(-28.8422637517799,21.3648535306115,3.94813437198529));
#55423=CARTESIAN_POINT('Ctrl Pts',(-29.2225270660648,21.574871526052,4.4261971800743));
#55424=CARTESIAN_POINT('Ctrl Pts',(-28.9090374964588,21.2951002599166,4.358748713827));
#55425=CARTESIAN_POINT('Ctrl Pts',(-28.8651693060966,21.3419268232634,3.9382670253751));
#55426=CARTESIAN_POINT('Ctrl Pts',(-29.2442873168817,21.5546818289773,4.4221043148659));
#55427=CARTESIAN_POINT('Ctrl Pts',(-28.9185449045375,21.2814642482843,4.35818647001453));
#55428=CARTESIAN_POINT('Ctrl Pts',(-28.8760494312548,21.3299250141018,3.93333521783471));
#55429=CARTESIAN_POINT('Ctrl Pts',(-29.2855172252132,21.5124704374293,4.4140388236016));
#55430=CARTESIAN_POINT('Ctrl Pts',(-28.9357479492706,21.2539523862257,4.35731088088201));
#55431=CARTESIAN_POINT('Ctrl Pts',(-28.8966643862929,21.3048295496241,3.92362069657755));
#55432=CARTESIAN_POINT('Ctrl Pts',(-29.3049871100764,21.4904489712157,4.410065963496));
#55433=CARTESIAN_POINT('Ctrl Pts',(-28.9434266252406,21.240076656282,4.35699977222348));
#55434=CARTESIAN_POINT('Ctrl Pts',(-28.9063993271011,21.2917360294249,3.91883768812767));
#55435=CARTESIAN_POINT('Ctrl Pts',(-29.3415625002293,21.4444902677988,4.402363670954));
#55436=CARTESIAN_POINT('Ctrl Pts',(-28.9571107238047,21.2122497699259,4.35662455375813));
#55437=CARTESIAN_POINT('Ctrl Pts',(-28.924687024552,21.2644073658392,3.90956767582023));
#55438=CARTESIAN_POINT('Ctrl Pts',(-29.3583797183681,21.4209125841129,4.39869552597858));
#55439=CARTESIAN_POINT('Ctrl Pts',(-28.9629914489214,21.1985271478654,4.35656529392032));
#55440=CARTESIAN_POINT('Ctrl Pts',(-28.9330956328352,21.250386023388,3.90515441115447));
#55441=CARTESIAN_POINT('Ctrl Pts',(-29.3891180653537,21.3726539763336,4.39183005163618));
#55442=CARTESIAN_POINT('Ctrl Pts',(-28.973161148024,21.1715660793365,4.35664406229473));
#55443=CARTESIAN_POINT('Ctrl Pts',(-28.9484648055261,21.2216851508184,3.89689615360288));
#55444=CARTESIAN_POINT('Ctrl Pts',(-29.4030479090076,21.3479616794509,4.38863064158663));
#55445=CARTESIAN_POINT('Ctrl Pts',(-28.9774363028591,21.1583373942717,4.35678323811578));
#55446=CARTESIAN_POINT('Ctrl Pts',(-28.9554297274226,21.2069988583241,3.89304864813538));
#55447=CARTESIAN_POINT('Ctrl Pts',(-29.4280377101348,21.2974429815817,4.38278815283631));
#55448=CARTESIAN_POINT('Ctrl Pts',(-28.9846847835139,21.132352936126,4.35718155517005));
#55449=CARTESIAN_POINT('Ctrl Pts',(-28.9679246286489,21.1769500095266,3.88602375231856));
#55450=CARTESIAN_POINT('Ctrl Pts',(-29.4390978280929,21.2716166629097,4.38014489699121));
#55451=CARTESIAN_POINT('Ctrl Pts',(-28.9876452414535,21.1196164947342,4.35744097622522));
#55452=CARTESIAN_POINT('Ctrl Pts',(-28.9734546861524,21.1615875015985,3.88284613948955));
#55453=CARTESIAN_POINT('Ctrl Pts',(-29.4534759095429,21.2319956842511,4.37666552971888));
#55454=CARTESIAN_POINT('Ctrl Pts',(-28.9912930054326,21.100819367134,4.35785159131797));
#55455=CARTESIAN_POINT('Ctrl Pts',(-28.9806437285937,21.1380183730222,3.87866382554668));
#55456=CARTESIAN_POINT('Ctrl Pts',(-29.4578992249067,21.2186415082209,4.37558668943266));
#55457=CARTESIAN_POINT('Ctrl Pts',(-28.9923770229233,21.0945950001855,4.35799224521163));
#55458=CARTESIAN_POINT('Ctrl Pts',(-28.9828553849103,21.1300742769095,3.87736710403448));
#55459=CARTESIAN_POINT('Ctrl Pts',(-29.465987969714,21.191630150372,4.37360293094838));
#55460=CARTESIAN_POINT('Ctrl Pts',(-28.9943073102353,21.0822177995094,4.35826908963608));
#55461=CARTESIAN_POINT('Ctrl Pts',(-28.9868997589003,21.1140055482561,3.87498282025292));
#55462=CARTESIAN_POINT('Ctrl Pts',(-29.4696192822395,21.1780858893991,4.37270640575372));
#55463=CARTESIAN_POINT('Ctrl Pts',(-28.9951445909393,21.0761195371597,4.35840399173927));
#55464=CARTESIAN_POINT('Ctrl Pts',(-28.9887154148245,21.1059480903675,3.87390533985094));
#55465=CARTESIAN_POINT('Ctrl Pts',(-29.4792870650363,21.13738000291,4.37030959268363));
#55466=CARTESIAN_POINT('Ctrl Pts',(-28.9973268947821,21.0580347058315,4.35878246091283));
#55467=CARTESIAN_POINT('Ctrl Pts',(-28.993549304859,21.0817318899304,3.87102485145596));
#55468=CARTESIAN_POINT('Ctrl Pts',(-29.4841057550382,21.1101273328488,4.36910072638058));
#55469=CARTESIAN_POINT('Ctrl Pts',(-28.9983395250804,21.0463040140866,4.35899767552963));
#55470=CARTESIAN_POINT('Ctrl Pts',(-28.9959586508823,21.0655186484503,3.86957217090424));
#55471=CARTESIAN_POINT('Ctrl Pts',(-29.490550264767,21.0553939291526,4.3674802440335));
#55472=CARTESIAN_POINT('Ctrl Pts',(-28.9996760790639,21.0230971570783,4.3592939950583));
#55473=CARTESIAN_POINT('Ctrl Pts',(-28.9991809055205,21.0329560350085,3.86762489270201));
#55474=CARTESIAN_POINT('Ctrl Pts',(-29.4921760097455,21.0279131927772,4.36706858867408));
#55475=CARTESIAN_POINT('Ctrl Pts',(-28.9999974971213,21.0116434845654,4.35937439790459));
#55476=CARTESIAN_POINT('Ctrl Pts',(-28.9999937774283,21.0166066609195,3.86713024612489));
#55477=CARTESIAN_POINT('Ctrl Pts',(-29.4921945688699,20.9865184618008,4.36706389944914));
#55478=CARTESIAN_POINT('Ctrl Pts',(-29.0000012300241,20.9943763875203,4.35937529589598));
#55479=CARTESIAN_POINT('Ctrl Pts',(-29.0000030580324,20.9919793004215,3.86712461212284));
#55480=CARTESIAN_POINT('Ctrl Pts',(-29.491796693937,20.9726912328558,4.36716447751106));
#55481=CARTESIAN_POINT('Ctrl Pts',(-28.9999215676363,20.988610264623,4.3593559292573));
#55482=CARTESIAN_POINT('Ctrl Pts',(-28.9998041196641,20.9837529354893,3.86724546797549));
#55483=CARTESIAN_POINT('Ctrl Pts',(-29.4905838324028,20.9519061373972,4.36747053318267));
#55484=CARTESIAN_POINT('Ctrl Pts',(-28.999675702201,20.9799035943349,4.35929796339857));
#55485=CARTESIAN_POINT('Ctrl Pts',(-28.9991976897288,20.9713871033612,3.86761323505766));
#55486=CARTESIAN_POINT('Ctrl Pts',(-29.4900768240666,20.9449703938439,4.36759841750078));
#55487=CARTESIAN_POINT('Ctrl Pts',(-28.9995726548501,20.9769928752733,4.35927385175331));
#55488=CARTESIAN_POINT('Ctrl Pts',(-28.9989441849534,20.9672607767751,3.86776690539778));
#55489=CARTESIAN_POINT('Ctrl Pts',(-29.4888550894157,20.9310839796645,4.36790625998637));
#55490=CARTESIAN_POINT('Ctrl Pts',(-28.9993226236041,20.9711468188149,4.35921639130902));
#55491=CARTESIAN_POINT('Ctrl Pts',(-28.998333318288,20.958999264393,3.86813682365838));
#55492=CARTESIAN_POINT('Ctrl Pts',(-29.4881390288598,20.9241230577317,4.36808655417366));
#55493=CARTESIAN_POINT('Ctrl Pts',(-28.9991753960847,20.9682075011393,4.359182987778));
#55494=CARTESIAN_POINT('Ctrl Pts',(-28.9979752880381,20.954857979854,3.86835347509526));
#55495=CARTESIAN_POINT('Ctrl Pts',(-29.4840537217879,20.8894481005333,4.36911380624685));
#55496=CARTESIAN_POINT('Ctrl Pts',(-28.9983287272948,20.9535160550957,4.35899529685436));
#55497=CARTESIAN_POINT('Ctrl Pts',(-28.9959326327119,20.9342287640144,3.86958788758089));
#55498=CARTESIAN_POINT('Ctrl Pts',(-29.4791760262202,20.8620847319681,4.3703372687358));
#55499=CARTESIAN_POINT('Ctrl Pts',(-28.9973025839744,20.9417309609864,4.35877783659216));
#55500=CARTESIAN_POINT('Ctrl Pts',(-28.99349378694,20.9179496726881,3.87105811205627));
#55501=CARTESIAN_POINT('Ctrl Pts',(-29.4663175094312,20.8080808536016,4.37352482341733));
#55502=CARTESIAN_POINT('Ctrl Pts',(-28.994401313152,20.9177541238724,4.35827550035249));
#55503=CARTESIAN_POINT('Ctrl Pts',(-28.9870645273859,20.8858224184757,3.87488891416135));
#55504=CARTESIAN_POINT('Ctrl Pts',(-29.4583363712703,20.781440422373,4.3754890345634));
#55505=CARTESIAN_POINT('Ctrl Pts',(-28.9925312984857,20.9055848597636,4.35799165813907));
#55506=CARTESIAN_POINT('Ctrl Pts',(-28.9830739586739,20.8699743012662,3.87724964182235));
#55507=CARTESIAN_POINT('Ctrl Pts',(-29.4392907133724,20.7288730680683,4.38009852314833));
#55508=CARTESIAN_POINT('Ctrl Pts',(-28.9876955597396,20.8806200036176,4.35744597641831));
#55509=CARTESIAN_POINT('Ctrl Pts',(-28.9735511301478,20.838703815867,3.88279039442718));
#55510=CARTESIAN_POINT('Ctrl Pts',(-29.4282263471482,20.7029461219291,4.38274392128853));
#55511=CARTESIAN_POINT('Ctrl Pts',(-28.9847392481334,20.8678470649529,4.35718476315632));
#55512=CARTESIAN_POINT('Ctrl Pts',(-28.9680189458604,20.8232814341429,3.88597056971191));
#55513=CARTESIAN_POINT('Ctrl Pts',(-29.4092629849526,20.6645986868852,4.38717765262327));
#55514=CARTESIAN_POINT('Ctrl Pts',(-28.9792302173559,20.8480911023819,4.35688171049857));
#55515=CARTESIAN_POINT('Ctrl Pts',(-28.9585372662084,20.8004721277644,3.89130160193992));
#55516=CARTESIAN_POINT('Ctrl Pts',(-29.4025397457092,20.6518998355629,4.38873461288905));
#55517=CARTESIAN_POINT('Ctrl Pts',(-28.9772187361615,20.841423256124,4.35679578954984));
#55518=CARTESIAN_POINT('Ctrl Pts',(-28.9551756466686,20.792918985876,3.89317381761125));
#55519=CARTESIAN_POINT('Ctrl Pts',(-29.3884503169696,20.6269598359164,4.39195827974487));
#55520=CARTESIAN_POINT('Ctrl Pts',(-28.9728478403863,20.8280481355966,4.3566663867452));
#55521=CARTESIAN_POINT('Ctrl Pts',(-28.9481309311711,20.7780854122449,3.89705062175834));
#55522=CARTESIAN_POINT('Ctrl Pts',(-29.3810676023746,20.6146832373181,4.39362888709889));
#55523=CARTESIAN_POINT('Ctrl Pts',(-28.9704856627442,20.8213250082211,4.35662245897598));
#55524=CARTESIAN_POINT('Ctrl Pts',(-28.9444395747976,20.7707838933009,3.89905990688947));
#55525=CARTESIAN_POINT('Ctrl Pts',(-29.3579234151702,20.5784203361143,4.39879588786272));
#55526=CARTESIAN_POINT('Ctrl Pts',(-28.962834961066,20.8010908203,4.35656590199818));
#55527=CARTESIAN_POINT('Ctrl Pts',(-28.9328674801151,20.7492172623072,3.90527514970604));
#55528=CARTESIAN_POINT('Ctrl Pts',(-29.3411684295824,20.554999545547,4.40244744076628));
#55529=CARTESIAN_POINT('Ctrl Pts',(-28.9569650458199,20.7874431803912,4.35662793190136));
#55530=CARTESIAN_POINT('Ctrl Pts',(-28.9244899880314,20.7352892524624,3.90966848618537));
#55531=CARTESIAN_POINT('Ctrl Pts',(-29.3050389928751,20.509631383246,4.41005424644623));
#55532=CARTESIAN_POINT('Ctrl Pts',(-28.9434428600321,20.7599671800727,4.35699994410375));
#55533=CARTESIAN_POINT('Ctrl Pts',(-28.9064252696976,20.7083117589753,3.91882359624169));
#55534=CARTESIAN_POINT('Ctrl Pts',(-29.2856645850222,20.4876840236708,4.41400971484573));
#55535=CARTESIAN_POINT('Ctrl Pts',(-28.9358090310734,20.7461480282885,4.35730790601429));
#55536=CARTESIAN_POINT('Ctrl Pts',(-28.8967380651115,20.6952622835462,3.92358563950055));
#55537=CARTESIAN_POINT('Ctrl Pts',(-29.2546003141753,20.4558748807086,4.42008700257675));
#55538=CARTESIAN_POINT('Ctrl Pts',(-28.922820708895,20.7253724543198,4.35796877663784));
#55539=CARTESIAN_POINT('Ctrl Pts',(-28.8812059306627,20.6763511463606,3.93090545440959));
#55540=CARTESIAN_POINT('Ctrl Pts',(-29.2439108547355,20.4454572265231,4.42213679870052));
#55541=CARTESIAN_POINT('Ctrl Pts',(-28.9182525509865,20.7184631598855,4.35822084476127));
#55542=CARTESIAN_POINT('Ctrl Pts',(-28.8758612003024,20.6701579942265,3.93337488161505));
#55543=CARTESIAN_POINT('Ctrl Pts',(-29.2218496639032,20.4249998034319,4.42626941644993));
#55544=CARTESIAN_POINT('Ctrl Pts',(-28.9085864424628,20.704673758766,4.35878899591022));
#55545=CARTESIAN_POINT('Ctrl Pts',(-28.8648306055172,20.6579970468792,3.93835482427701));
#55546=CARTESIAN_POINT('Ctrl Pts',(-29.2105624521793,20.4150385371535,4.42833633785348));
#55547=CARTESIAN_POINT('Ctrl Pts',(-28.9035275473896,20.6978463189018,4.35910263212055));
#55548=CARTESIAN_POINT('Ctrl Pts',(-28.8591869996611,20.652075919572,3.9408461871511));
#55549=CARTESIAN_POINT('Ctrl Pts',(-29.17596044531,20.3859527127987,4.43451242027464));
#55550=CARTESIAN_POINT('Ctrl Pts',(-28.8877003840881,20.6776599163682,4.36012163656125));
#55551=CARTESIAN_POINT('Ctrl Pts',(-28.8418859952628,20.6347879628064,3.94829277941604));
#55552=CARTESIAN_POINT('Ctrl Pts',(-29.1518999346225,20.3676173671137,4.43859827357297));
#55553=CARTESIAN_POINT('Ctrl Pts',(-28.8762195965627,20.6644978369657,4.3609092118001));
#55554=CARTESIAN_POINT('Ctrl Pts',(-28.8298557406079,20.623891349496,3.95322218460065));
#55555=CARTESIAN_POINT('Ctrl Pts',(-29.1018152722641,20.3330053854538,4.44658373092187));
#55556=CARTESIAN_POINT('Ctrl Pts',(-28.8513847136705,20.6390640139852,4.36263702917292));
#55557=CARTESIAN_POINT('Ctrl Pts',(-28.8048134093357,20.6033246767378,3.96286433535749));
#55558=CARTESIAN_POINT('Ctrl Pts',(-29.0757911091889,20.3167288114029,4.45048354811133));
#55559=CARTESIAN_POINT('Ctrl Pts',(-28.8380400572134,20.6267792408873,4.36357636390023));
#55560=CARTESIAN_POINT('Ctrl Pts',(-28.7918013274224,20.5936546558004,3.96757734921668));
#55561=CARTESIAN_POINT('Ctrl Pts',(-29.0352521593023,20.2938681210549,4.45609925522955));
#55562=CARTESIAN_POINT('Ctrl Pts',(-28.8165561798406,20.6091707900662,4.3650399217219));
#55563=CARTESIAN_POINT('Ctrl Pts',(-28.7715318531124,20.5800754935647,3.97437224143204));
#55564=CARTESIAN_POINT('Ctrl Pts',(-29.0214882535223,20.2865074155593,4.45793211239332));
#55565=CARTESIAN_POINT('Ctrl Pts',(-28.8091714143158,20.6034513832319,4.36553535860525));
#55566=CARTESIAN_POINT('Ctrl Pts',(-28.7646498997047,20.5757037147109,3.97659139070366));
#55567=CARTESIAN_POINT('Ctrl Pts',(-28.9934475912048,20.2723129927531,4.46150315485745));
#55568=CARTESIAN_POINT('Ctrl Pts',(-28.7939226308694,20.5923278305027,4.36653127887413));
#55569=CARTESIAN_POINT('Ctrl Pts',(-28.7506295691592,20.5672740749771,3.98091835755158));
#55570=CARTESIAN_POINT('Ctrl Pts',(-28.9791516290983,20.2654706309964,4.46324356194687));
#55571=CARTESIAN_POINT('Ctrl Pts',(-28.7860480544218,20.5869145754601,4.36703250165608));
#55572=CARTESIAN_POINT('Ctrl Pts',(-28.7434815880803,20.5632110844206,3.9830288783974));
#55573=CARTESIAN_POINT('Ctrl Pts',(-28.9355954945563,20.2458084368345,4.46828239715749));
#55574=CARTESIAN_POINT('Ctrl Pts',(-28.7618066384647,20.5712704270414,4.36851780691574));
#55575=CARTESIAN_POINT('Ctrl Pts',(-28.7217035199663,20.5515371684708,3.98914513962966));
#55576=CARTESIAN_POINT('Ctrl Pts',(-28.9060067033566,20.2339995629551,4.47135989471833));
#55577=CARTESIAN_POINT('Ctrl Pts',(-28.744926685415,20.561687181048,4.36947765667699));
#55578=CARTESIAN_POINT('Ctrl Pts',(-28.7069091250645,20.5445280122945,3.99288879390593));
#55579=CARTESIAN_POINT('Ctrl Pts',(-28.8457485283665,20.2129019554985,4.47686103269499));
#55580=CARTESIAN_POINT('Ctrl Pts',(-28.7099310450066,20.5444276147742,4.37123208934274));
#55581=CARTESIAN_POINT('Ctrl Pts',(-28.6767800372973,20.5320096838262,3.99960093357708));
#55582=CARTESIAN_POINT('Ctrl Pts',(-28.8150790711961,20.2036134333842,4.47928478552995));
#55583=CARTESIAN_POINT('Ctrl Pts',(-28.6918007935838,20.5367306237201,4.37202848226936));
#55584=CARTESIAN_POINT('Ctrl Pts',(-28.661445308714,20.5265006375016,4.00256956422312));
#55585=CARTESIAN_POINT('Ctrl Pts',(-28.7526503432492,20.1875566536874,4.48338903627318));
#55586=CARTESIAN_POINT('Ctrl Pts',(-28.6544284801008,20.5233913850482,4.3733658398148));
#55587=CARTESIAN_POINT('Ctrl Pts',(-28.630230945009,20.5169822622779,4.00762555943285));
#55588=CARTESIAN_POINT('Ctrl Pts',(-28.7208911539916,20.1807882220752,4.48506965036132));
#55589=CARTESIAN_POINT('Ctrl Pts',(-28.6351661922031,20.5177318547895,4.3739085857297));
#55590=CARTESIAN_POINT('Ctrl Pts',(-28.6143513499902,20.5129728344691,4.00971307048814));
#55591=CARTESIAN_POINT('Ctrl Pts',(-28.6804858960801,20.1739508495855,4.48664840826309));
#55592=CARTESIAN_POINT('Ctrl Pts',(-28.6104428872724,20.5120427346769,4.37437784801154));
#55593=CARTESIAN_POINT('Ctrl Pts',(-28.5941487213541,20.5089266867687,4.01170353994373));
#55594=CARTESIAN_POINT('Ctrl Pts',(-28.6723694509432,20.1726647303069,4.48693804895347));
#55595=CARTESIAN_POINT('Ctrl Pts',(-28.6054711836597,20.5109751096991,4.37446121623121));
#55596=CARTESIAN_POINT('Ctrl Pts',(-28.5900904986563,20.5081658573795,4.01207067678645));
#55597=CARTESIAN_POINT('Ctrl Pts',(-28.6560648033424,20.1702572399895,4.4874636130762));
#55598=CARTESIAN_POINT('Ctrl Pts',(-28.5954663925238,20.5089814406573,4.37460598400524));
#55599=CARTESIAN_POINT('Ctrl Pts',(-28.5819381749868,20.5067421999854,4.01274126216542));
#55600=CARTESIAN_POINT('Ctrl Pts',(-28.64786409799,20.1691343513156,4.48769983367621));
#55601=CARTESIAN_POINT('Ctrl Pts',(-28.5904251656171,20.5080539749396,4.37466747173636));
#55602=CARTESIAN_POINT('Ctrl Pts',(-28.5778378222945,20.5060784772816,4.01304510036563));
#55603=CARTESIAN_POINT('Ctrl Pts',(-28.6232544580252,20.1660288494912,4.48832318516655));
#55604=CARTESIAN_POINT('Ctrl Pts',(-28.5752783730565,20.5054996163594,4.37481674441907));
#55605=CARTESIAN_POINT('Ctrl Pts',(-28.565533002164,20.5042437954364,4.01385517953166));
#55606=CARTESIAN_POINT('Ctrl Pts',(-28.606854980142,20.1643100524113,4.4886249903596));
#55607=CARTESIAN_POINT('Ctrl Pts',(-28.565150180646,20.5040992890267,4.37486951557626));
#55608=CARTESIAN_POINT('Ctrl Pts',(-28.5573332633662,20.5032296994079,4.01425992288297));
#55609=CARTESIAN_POINT('Ctrl Pts',(-28.5576771166509,20.1601865473193,4.48918952635597));
#55610=CARTESIAN_POINT('Ctrl Pts',(-28.5347358984571,20.5008030232128,4.3748833203254));
#55611=CARTESIAN_POINT('Ctrl Pts',(-28.5327443314856,20.5008014950845,4.01506876078307));
#55612=CARTESIAN_POINT('Ctrl Pts',(-28.5249192895454,20.1588122643254,4.48911128378351));
#55613=CARTESIAN_POINT('Ctrl Pts',(-28.5143793401766,20.4998059891208,4.37469926808766));
#55614=CARTESIAN_POINT('Ctrl Pts',(-28.5163654189693,20.5,4.01506735657853));
#55615=CARTESIAN_POINT('Ctrl Pts',(-28.4921884534997,20.1587864726715,4.48858057664303));
#55616=CARTESIAN_POINT('Ctrl Pts',(-28.4940712607011,20.5,4.37432028438837));
#55617=CARTESIAN_POINT('Ctrl Pts',(-28.5,20.5,4.01452801010866));
#55618=CARTESIAN_POINT('Origin',(-28.5,22.,4.01452801010865));
#55619=CARTESIAN_POINT('Ctrl Pts',(-17.1604382594737,21.8496676025271,4.3051562369529));
#55620=CARTESIAN_POINT('Ctrl Pts',(-17.1622439953065,21.5,4.19493778427511));
#55621=CARTESIAN_POINT('Ctrl Pts',(-17.168249805974,21.5,3.82835528266346));
#55622=CARTESIAN_POINT('Ctrl Pts',(-20.9376911771606,21.8469996121483,4.36619869326066));
#55623=CARTESIAN_POINT('Ctrl Pts',(-20.9317890321398,21.5,4.25454850865233));
#55624=CARTESIAN_POINT('Ctrl Pts',(-20.9455027250583,21.5,3.89023893993915));
#55625=CARTESIAN_POINT('Ctrl Pts',(-24.7149414253597,21.8441900241541,4.42733523082889));
#55626=CARTESIAN_POINT('Ctrl Pts',(-24.7082452246339,21.5,4.3143246996786));
#55627=CARTESIAN_POINT('Ctrl Pts',(-24.7227529733574,21.5,3.9522856706513));
#55628=CARTESIAN_POINT('Ctrl Pts',(-28.4921884534997,21.8412135273285,4.48858057664302));
#55629=CARTESIAN_POINT('Ctrl Pts',(-28.4940712607011,21.5,4.37432028438836));
#55630=CARTESIAN_POINT('Ctrl Pts',(-28.5,21.5,4.01452801010865));
#55631=CARTESIAN_POINT('',(-17.1682498059738,21.5,3.82835528266346));
#55632=CARTESIAN_POINT('Origin',(-17.1682498059739,22.,3.82835528266346));
#55633=CARTESIAN_POINT('Ctrl Pts',(-28.5,21.5,4.01452801010865));
#55634=CARTESIAN_POINT('Ctrl Pts',(-24.7227529733574,21.5,3.9522856706513));
#55635=CARTESIAN_POINT('Ctrl Pts',(-20.9455027250583,21.5,3.89023893993915));
#55636=CARTESIAN_POINT('Ctrl Pts',(-17.168249805974,21.5,3.82835528266346));
#55637=CARTESIAN_POINT('Ctrl Pts',(-16.2025936105234,22.0000000000015,3.11864718944382));
#55638=CARTESIAN_POINT('Ctrl Pts',(-16.2025936105219,21.5,3.11864718944354));
#55639=CARTESIAN_POINT('Ctrl Pts',(-16.6935812956895,21.5,3.21315164973649));
#55640=CARTESIAN_POINT('Ctrl Pts',(-16.1958052905938,21.9952325252242,3.15391517021521));
#55641=CARTESIAN_POINT('Ctrl Pts',(-16.2004968595706,21.5,3.15464482315937));
#55642=CARTESIAN_POINT('Ctrl Pts',(-16.6900632709881,21.5,3.23142922671518));
#55643=CARTESIAN_POINT('Ctrl Pts',(-16.1909736753984,21.9904410335953,3.18921042980328));
#55644=CARTESIAN_POINT('Ctrl Pts',(-16.2003114121254,21.5,3.1903398755215));
#55645=CARTESIAN_POINT('Ctrl Pts',(-16.6875219293389,21.5,3.24972861619305));
#55646=CARTESIAN_POINT('Ctrl Pts',(-16.1850775609935,21.9808091032242,3.25984918716021));
#55647=CARTESIAN_POINT('Ctrl Pts',(-16.2035534038268,21.5,3.26082216812292));
#55648=CARTESIAN_POINT('Ctrl Pts',(-16.6843194194186,21.5,3.28636833461055));
#55649=CARTESIAN_POINT('Ctrl Pts',(-16.184013429373,21.9759686124482,3.29519304000078));
#55650=CARTESIAN_POINT('Ctrl Pts',(-16.2069478202362,21.5,3.2956192570052));
#55651=CARTESIAN_POINT('Ctrl Pts',(-16.683658429449,21.5,3.30470884710496));
#55652=CARTESIAN_POINT('Ctrl Pts',(-16.1856383299933,21.9662403165847,3.36592917468473));
#55653=CARTESIAN_POINT('Ctrl Pts',(-16.2171931046112,21.5,3.36436828037402));
#55654=CARTESIAN_POINT('Ctrl Pts',(-16.6842095997079,21.5,3.34143101656532));
#55655=CARTESIAN_POINT('Ctrl Pts',(-16.1883270541929,21.9613524899569,3.40132143910138));
#55656=CARTESIAN_POINT('Ctrl Pts',(-16.2240124021103,21.5,3.39832915993044));
#55657=CARTESIAN_POINT('Ctrl Pts',(-16.6854215969232,21.5,3.35981266995062));
#55658=CARTESIAN_POINT('Ctrl Pts',(-16.1952611487782,21.9539890215863,3.45444862229374));
#55659=CARTESIAN_POINT('Ctrl Pts',(-16.2368456377949,21.5,3.44879630945697));
#55660=CARTESIAN_POINT('Ctrl Pts',(-16.688687584381,21.5,3.38741695572715));
#55661=CARTESIAN_POINT('Ctrl Pts',(-16.1980673520651,21.9515228743596,3.47221008447614));
#55662=CARTESIAN_POINT('Ctrl Pts',(-16.2415532166551,21.5,3.46552752665128));
#55663=CARTESIAN_POINT('Ctrl Pts',(-16.690023065315,21.5,3.39664756592707));
#55664=CARTESIAN_POINT('Ctrl Pts',(-16.2046004673532,21.9466330695926,3.50737333745249));
#55665=CARTESIAN_POINT('Ctrl Pts',(-16.2517211449691,21.5,3.49845354955799));
#55666=CARTESIAN_POINT('Ctrl Pts',(-16.6931549914451,21.5,3.41492555061629));
#55667=CARTESIAN_POINT('Ctrl Pts',(-16.2083287551219,21.9442051915696,3.52480572265553));
#55668=CARTESIAN_POINT('Ctrl Pts',(-16.2571835066352,21.5,3.51468075299862));
#55669=CARTESIAN_POINT('Ctrl Pts',(-16.6949520176578,21.5,3.42398881019779));
#55670=CARTESIAN_POINT('Ctrl Pts',(-16.2208770992767,21.9369742070162,3.57666299693395));
#55671=CARTESIAN_POINT('Ctrl Pts',(-16.2746405337289,21.5,3.56257355900406));
#55672=CARTESIAN_POINT('Ctrl Pts',(-16.7010254780178,21.5,3.45095493296853));
#55673=CARTESIAN_POINT('Ctrl Pts',(-16.2310567694075,21.9322234484231,3.61064917902866));
#55674=CARTESIAN_POINT('Ctrl Pts',(-16.2877614275171,21.5,3.59367857500056));
#55675=CARTESIAN_POINT('Ctrl Pts',(-16.7059823717865,21.5,3.46863477016759));
#55676=CARTESIAN_POINT('Ctrl Pts',(-16.2550248020928,21.9228769565563,3.67746306648168));
#55677=CARTESIAN_POINT('Ctrl Pts',(-16.3168653669915,21.5,3.65418392042109));
#55678=CARTESIAN_POINT('Ctrl Pts',(-16.7177028394155,21.5,3.50340229096279));
#55679=CARTESIAN_POINT('Ctrl Pts',(-16.2688128936766,21.9182811628345,3.71029083551438));
#55680=CARTESIAN_POINT('Ctrl Pts',(-16.332830368222,21.5,3.68360921264127));
#55681=CARTESIAN_POINT('Ctrl Pts',(-16.7244662683933,21.5,3.5204900220454));
#55682=CARTESIAN_POINT('Ctrl Pts',(-16.2922824275864,21.9115226184388,3.75864368771028));
#55683=CARTESIAN_POINT('Ctrl Pts',(-16.3589982628845,21.5,3.72661747700725));
#55684=CARTESIAN_POINT('Ctrl Pts',(-16.736007563454,21.5,3.54566401900879));
#55685=CARTESIAN_POINT('Ctrl Pts',(-16.3005711842475,21.9092923779025,3.77461286058377));
#55686=CARTESIAN_POINT('Ctrl Pts',(-16.3680638057343,21.5,3.74072812126781));
#55687=CARTESIAN_POINT('Ctrl Pts',(-16.7400878524955,21.5,3.55397892124875));
#55688=CARTESIAN_POINT('Ctrl Pts',(-16.3137228907241,21.9059841503794,3.79833842758307));
#55689=CARTESIAN_POINT('Ctrl Pts',(-16.3822304023763,21.5,3.76161740284943));
#55690=CARTESIAN_POINT('Ctrl Pts',(-16.7465683117126,21.5,3.56633327337009));
#55691=CARTESIAN_POINT('Ctrl Pts',(-16.3182212166037,21.9048890818084,3.80619831559438));
#55692=CARTESIAN_POINT('Ctrl Pts',(-16.3870345783552,21.5,3.76851593328029));
#55693=CARTESIAN_POINT('Ctrl Pts',(-16.7487858382735,21.5,3.57042620530286));
#55694=CARTESIAN_POINT('Ctrl Pts',(-16.3274032276077,21.9027249657743,3.82174713590922));
#55695=CARTESIAN_POINT('Ctrl Pts',(-16.3967694053034,21.5,3.78213337204833));
#55696=CARTESIAN_POINT('Ctrl Pts',(-16.7533142130753,21.5,3.57852323401373));
#55697=CARTESIAN_POINT('Ctrl Pts',(-16.3320928677396,21.9016544021241,3.82944691852646));
#55698=CARTESIAN_POINT('Ctrl Pts',(-16.4017064266611,21.5,3.78886237761036));
#55699=CARTESIAN_POINT('Ctrl Pts',(-16.7556279975421,21.5,3.58253297968588));
#55700=CARTESIAN_POINT('Ctrl Pts',(-16.3560302683597,21.8963596025904,3.86757608216625));
#55701=CARTESIAN_POINT('Ctrl Pts',(-16.4266703272049,21.5,3.82202712471223));
#55702=CARTESIAN_POINT('Ctrl Pts',(-16.7674429297045,21.5,3.60238940882647));
#55703=CARTESIAN_POINT('Ctrl Pts',(-16.3767412732872,21.8923088287891,3.89689945605709));
#55704=CARTESIAN_POINT('Ctrl Pts',(-16.4477938851887,21.5,3.8473985141041));
#55705=CARTESIAN_POINT('Ctrl Pts',(-16.7776799493915,21.5,3.61766088108806));
#55706=CARTESIAN_POINT('Ctrl Pts',(-16.4212547011672,21.8846000679653,3.95321952314127));
#55707=CARTESIAN_POINT('Ctrl Pts',(-16.4922230549556,21.5,3.89577853632942));
#55708=CARTESIAN_POINT('Ctrl Pts',(-16.7997098422747,21.5,3.64698765705913));
#55709=CARTESIAN_POINT('Ctrl Pts',(-16.4450569830293,21.8809420124786,3.98021630120148));
#55710=CARTESIAN_POINT('Ctrl Pts',(-16.5155303766581,21.5,3.91881887619101));
#55711=CARTESIAN_POINT('Ctrl Pts',(-16.8115026386653,21.5,3.66104302080526));
#55712=CARTESIAN_POINT('Ctrl Pts',(-16.4831394704891,21.8757778117398,4.01892896400379));
#55713=CARTESIAN_POINT('Ctrl Pts',(-16.5522429195535,21.5,3.9517142788955));
#55714=CARTESIAN_POINT('Ctrl Pts',(-16.8303901405096,21.5,3.6811893820933));
#55715=CARTESIAN_POINT('Ctrl Pts',(-16.4962310185836,21.87411034819,4.03153544455166));
#55716=CARTESIAN_POINT('Ctrl Pts',(-16.5647486534221,21.5,3.96238401751056));
#55717=CARTESIAN_POINT('Ctrl Pts',(-16.8368861257833,21.5,3.68774838298534));
#55718=CARTESIAN_POINT('Ctrl Pts',(-16.5232304690003,21.8708896855758,4.05613814359352));
#55719=CARTESIAN_POINT('Ctrl Pts',(-16.590350960388,21.5,3.98315775527099));
#55720=CARTESIAN_POINT('Ctrl Pts',(-16.8502894580342,21.5,3.70054483446619));
#55721=CARTESIAN_POINT('Ctrl Pts',(-16.5371840523959,21.8693320923327,4.06816930064024));
#55722=CARTESIAN_POINT('Ctrl Pts',(-16.6034911562703,21.5,3.99329469932326));
#55723=CARTESIAN_POINT('Ctrl Pts',(-16.857219503229,21.5,3.7068004456941));
#55724=CARTESIAN_POINT('Ctrl Pts',(-16.5798092654162,21.8648926734758,4.10291746959841));
#55725=CARTESIAN_POINT('Ctrl Pts',(-16.6433246202798,21.5,4.02248194760078));
#55726=CARTESIAN_POINT('Ctrl Pts',(-16.8783985705853,21.5,3.72486007985719));
#55727=CARTESIAN_POINT('Ctrl Pts',(-16.6093180269739,21.8622318314065,4.12437979135235));
#55728=CARTESIAN_POINT('Ctrl Pts',(-16.6706091197525,21.5,4.04047712969076));
#55729=CARTESIAN_POINT('Ctrl Pts',(-16.8930725009553,21.5,3.73600407557229));
#55730=CARTESIAN_POINT('Ctrl Pts',(-16.6704766461075,21.8575203303899,4.16397285607147));
#55731=CARTESIAN_POINT('Ctrl Pts',(-16.7265858290891,21.5,4.07360970878173));
#55732=CARTESIAN_POINT('Ctrl Pts',(-16.9235088870901,21.5,3.75653378697986));
#55733=CARTESIAN_POINT('Ctrl Pts',(-16.7021265340692,21.8554696437867,4.18210353848355));
#55734=CARTESIAN_POINT('Ctrl Pts',(-16.7553000207359,21.5,4.08877356617264));
#55735=CARTESIAN_POINT('Ctrl Pts',(-16.939271358146,21.5,3.76591947797279));
#55736=CARTESIAN_POINT('Ctrl Pts',(-16.7512338740401,21.8528738488001,4.20676429215578));
#55737=CARTESIAN_POINT('Ctrl Pts',(-16.7995480615473,21.5,4.10943149659409));
#55738=CARTESIAN_POINT('Ctrl Pts',(-16.9637457752419,21.5,3.77865617925544));
#55739=CARTESIAN_POINT('Ctrl Pts',(-16.7678756736467,21.8520887609395,4.21456104764755));
#55740=CARTESIAN_POINT('Ctrl Pts',(-16.8144838835962,21.5,4.11596590227308));
#55741=CARTESIAN_POINT('Ctrl Pts',(-16.9720426664911,21.5,3.78267762181121));
#55742=CARTESIAN_POINT('Ctrl Pts',(-16.7932565263885,21.851035571477,4.22560727704492));
#55743=CARTESIAN_POINT('Ctrl Pts',(-16.8372007595605,21.5,4.12524195165351));
#55744=CARTESIAN_POINT('Ctrl Pts',(-16.9847008585882,21.5,3.78836596354519));
#55745=CARTESIAN_POINT('Ctrl Pts',(-16.801786542946,21.8507052596251,4.22918113595141));
#55746=CARTESIAN_POINT('Ctrl Pts',(-16.844822832901,21.5,4.12824551873968));
#55747=CARTESIAN_POINT('Ctrl Pts',(-16.988955749425,21.5,3.79020474534342));
#55748=CARTESIAN_POINT('Ctrl Pts',(-16.8189881015471,21.8500869595188,4.23610930375404));
#55749=CARTESIAN_POINT('Ctrl Pts',(-16.8601732377462,21.5,4.13407543455927));
#55750=CARTESIAN_POINT('Ctrl Pts',(-16.9975375853533,21.5,3.79376592069795));
#55751=CARTESIAN_POINT('Ctrl Pts',(-16.8276738712233,21.8497985841018,4.23946862537602));
#55752=CARTESIAN_POINT('Ctrl Pts',(-16.867914670736,21.5,4.1369063079806));
#55753=CARTESIAN_POINT('Ctrl Pts',(-17.0018716295893,21.5,3.79549088840137));
#55754=CARTESIAN_POINT('Ctrl Pts',(-16.8711939657873,21.8484725442454,4.25561007104468));
#55755=CARTESIAN_POINT('Ctrl Pts',(-16.9066342732154,21.5,4.15052253339453));
#55756=CARTESIAN_POINT('Ctrl Pts',(-17.0235910074471,21.5,3.80377002509308));
#55757=CARTESIAN_POINT('Ctrl Pts',(-16.9064159264563,21.8477761420408,4.26648696465632));
#55758=CARTESIAN_POINT('Ctrl Pts',(-16.9378678496199,21.5,4.15978704982608));
#55759=CARTESIAN_POINT('Ctrl Pts',(-17.0411805852199,21.5,3.80931813715357));
#55760=CARTESIAN_POINT('Ctrl Pts',(-16.9776436707534,21.8470943053695,4.2843084329609));
#55761=CARTESIAN_POINT('Ctrl Pts',(-17.000858079899,21.5,4.17518084553056));
#55762=CARTESIAN_POINT('Ctrl Pts',(-17.0767734998278,21.5,3.81833625027318));
#55763=CARTESIAN_POINT('Ctrl Pts',(-17.01364953131,21.8471089197294,4.29125260718064));
#55764=CARTESIAN_POINT('Ctrl Pts',(-17.0326487818633,21.5,4.1813198113202));
#55765=CARTESIAN_POINT('Ctrl Pts',(-17.0947768799094,21.5,3.82180603412564));
#55766=CARTESIAN_POINT('Ctrl Pts',(-17.0864469048579,21.8478497977723,4.30119943960749));
#55767=CARTESIAN_POINT('Ctrl Pts',(-17.0968888854338,21.5,4.1904875213887));
#55768=CARTESIAN_POINT('Ctrl Pts',(-17.1311983375874,21.5,3.82666277743901));
#55769=CARTESIAN_POINT('Ctrl Pts',(-17.1232387598336,21.848576004873,4.30420261445776));
#55770=CARTESIAN_POINT('Ctrl Pts',(-17.1293741316385,21.5,4.19351989656681));
#55771=CARTESIAN_POINT('Ctrl Pts',(-17.1496165974329,21.5,3.8280499971787));
#55772=CARTESIAN_POINT('Ctrl Pts',(-17.1604382594748,21.8496676025273,4.3051562369486));
#55773=CARTESIAN_POINT('Ctrl Pts',(-17.1622439953075,21.5,4.19493778427092));
#55774=CARTESIAN_POINT('Ctrl Pts',(-17.1682498059746,21.5,3.82835528265908));
#55775=CARTESIAN_POINT('',(-16.6935812956895,21.5,3.21315164973691));
#55776=CARTESIAN_POINT('Origin',(-16.6935812956894,22.,3.21315164973691));
#55777=CARTESIAN_POINT('Ctrl Pts',(-17.1682498059738,21.5,3.82835528266346));
#55778=CARTESIAN_POINT('Ctrl Pts',(-17.1496163615266,21.5,3.82805000639156));
#55779=CARTESIAN_POINT('Ctrl Pts',(-17.1311983124107,21.5,3.82666291100431));
#55780=CARTESIAN_POINT('Ctrl Pts',(-17.1129875977713,21.5,3.82423447272218));
#55781=CARTESIAN_POINT('Ctrl Pts',(-17.0947768831318,21.5,3.82180603444003));
#55782=CARTESIAN_POINT('Ctrl Pts',(-17.0767734953455,21.5,3.81833624928029));
#55783=CARTESIAN_POINT('Ctrl Pts',(-17.0589770387714,21.5,3.81382719380588));
#55784=CARTESIAN_POINT('Ctrl Pts',(-17.0411805821973,21.5,3.8093181383315));
#55785=CARTESIAN_POINT('Ctrl Pts',(-17.0235910065198,21.5,3.80377002473762));
#55786=CARTESIAN_POINT('Ctrl Pts',(-17.0062155047223,21.5,3.79714671688814));
#55787=CARTESIAN_POINT('Ctrl Pts',(-17.001871629273,21.5,3.79549088992577));
#55788=CARTESIAN_POINT('Ctrl Pts',(-16.9975375843724,21.5,3.79376592229798));
#55789=CARTESIAN_POINT('Ctrl Pts',(-16.9932466670332,21.5,3.79198533387674));
#55790=CARTESIAN_POINT('Ctrl Pts',(-16.9889557496941,21.5,3.79020474545551));
#55791=CARTESIAN_POINT('Ctrl Pts',(-16.9847008623217,21.5,3.7883659651211));
#55792=CARTESIAN_POINT('Ctrl Pts',(-16.9804814700195,21.5,3.78646985358707));
#55793=CARTESIAN_POINT('Ctrl Pts',(-16.9720426854152,21.5,3.78267763051893));
#55794=CARTESIAN_POINT('Ctrl Pts',(-16.9637458137767,21.5,3.7786561987763));
#55795=CARTESIAN_POINT('Ctrl Pts',(-16.9555876582206,21.5,3.77441062361576));
#55796=CARTESIAN_POINT('Ctrl Pts',(-16.9392713471094,21.5,3.76591947329292));
#55797=CARTESIAN_POINT('Ctrl Pts',(-16.9235088867934,21.5,3.75653378679473));
#55798=CARTESIAN_POINT('Ctrl Pts',(-16.9082906937124,21.5,3.74626893113479));
#55799=CARTESIAN_POINT('Ctrl Pts',(-16.8930725006315,21.5,3.73600407547485));
#55800=CARTESIAN_POINT('Ctrl Pts',(-16.8783985701434,21.5,3.72486007947304));
#55801=CARTESIAN_POINT('Ctrl Pts',(-16.8642791914462,21.5,3.71282032480514));
#55802=CARTESIAN_POINT('Ctrl Pts',(-16.8572195020976,21.5,3.70680044747119));
#55803=CARTESIAN_POINT('Ctrl Pts',(-16.8502894552196,21.5,3.70054483670679));
#55804=CARTESIAN_POINT('Ctrl Pts',(-16.8435877906765,21.5,3.69414661001588));
#55805=CARTESIAN_POINT('Ctrl Pts',(-16.8368861261335,21.5,3.68774838332496));
#55806=CARTESIAN_POINT('Ctrl Pts',(-16.8303901666861,21.5,3.68118940941518));
#55807=CARTESIAN_POINT('Ctrl Pts',(-16.8240943181697,21.5,3.67447394733714));
#55808=CARTESIAN_POINT('Ctrl Pts',(-16.8115026211382,21.5,3.66104302317998));
#55809=CARTESIAN_POINT('Ctrl Pts',(-16.7997097982202,21.5,3.6469876915202));
#55810=CARTESIAN_POINT('Ctrl Pts',(-16.7886948737312,21.5,3.63232428633634));
#55811=CARTESIAN_POINT('Ctrl Pts',(-16.7776799492422,21.5,3.61766088115248));
#55812=CARTESIAN_POINT('Ctrl Pts',(-16.767442929528,21.5,3.60238940852384));
#55813=CARTESIAN_POINT('Ctrl Pts',(-16.7579909834741,21.5,3.58650426581163));
#55814=CARTESIAN_POINT('Ctrl Pts',(-16.7556279969606,21.5,3.58253298013358));
#55815=CARTESIAN_POINT('Ctrl Pts',(-16.7533142130046,21.5,3.57852323388594));
#55816=CARTESIAN_POINT('Ctrl Pts',(-16.7510500252507,21.5,3.57447471989511));
#55817=CARTESIAN_POINT('Ctrl Pts',(-16.7487858374968,21.5,3.57042620590428));
#55818=CARTESIAN_POINT('Ctrl Pts',(-16.7465683099919,21.5,3.56633327394474));
#55819=CARTESIAN_POINT('Ctrl Pts',(-16.744408157582,21.5,3.56221515655127));
#55820=CARTESIAN_POINT('Ctrl Pts',(-16.7400878527623,21.5,3.55397892176433));
#55821=CARTESIAN_POINT('Ctrl Pts',(-16.7360075823247,21.5,3.54566405902614));
#55822=CARTESIAN_POINT('Ctrl Pts',(-16.7321604686133,21.5,3.53727271349726));
#55823=CARTESIAN_POINT('Ctrl Pts',(-16.7244662411923,21.5,3.52049002243889));
#55824=CARTESIAN_POINT('Ctrl Pts',(-16.71770275581,21.5,3.50340231839282));
#55825=CARTESIAN_POINT('Ctrl Pts',(-16.7118425636876,21.5,3.4860185443094));
#55826=CARTESIAN_POINT('Ctrl Pts',(-16.7059823715651,21.5,3.46863477022598));
#55827=CARTESIAN_POINT('Ctrl Pts',(-16.7010254779788,21.5,3.45095493277599));
#55828=CARTESIAN_POINT('Ctrl Pts',(-16.6969765036837,21.5,3.43297751795946));
#55829=CARTESIAN_POINT('Ctrl Pts',(-16.6949520165362,21.5,3.4239888105512));
#55830=CARTESIAN_POINT('Ctrl Pts',(-16.6931549913987,21.5,3.41492555032882));
#55831=CARTESIAN_POINT('Ctrl Pts',(-16.6915890273506,21.5,3.40578655844823));
#55832=CARTESIAN_POINT('Ctrl Pts',(-16.6900230633025,21.5,3.39664756656763));
#55833=CARTESIAN_POINT('Ctrl Pts',(-16.6886875818764,21.5,3.38741695570003));
#55834=CARTESIAN_POINT('Ctrl Pts',(-16.6875989202476,21.5,3.37821552733009));
#55835=CARTESIAN_POINT('Ctrl Pts',(-16.6854215969899,21.5,3.3598126705902));
#55836=CARTESIAN_POINT('Ctrl Pts',(-16.6842095211892,21.5,3.341431016089));
#55837=CARTESIAN_POINT('Ctrl Pts',(-16.6839339752301,21.5,3.3230699323332));
#55838=CARTESIAN_POINT('Ctrl Pts',(-16.6836584292711,21.5,3.3047088485774));
#55839=CARTESIAN_POINT('Ctrl Pts',(-16.6843194198805,21.5,3.28636832755855));
#55840=CARTESIAN_POINT('Ctrl Pts',(-16.6859206734574,21.5,3.26804847058621));
#55841=CARTESIAN_POINT('Ctrl Pts',(-16.6875219270342,21.5,3.24972861361384));
#55842=CARTESIAN_POINT('Ctrl Pts',(-16.690063224909,21.5,3.23142940534175));
#55843=CARTESIAN_POINT('Ctrl Pts',(-16.6935812956894,21.5,3.2131516497369));
#55844=CARTESIAN_POINT('Ctrl Pts',(-16.202593610521,22.0000000000008,3.11864718945664));
#55845=CARTESIAN_POINT('Ctrl Pts',(-16.1957184589487,21.9951715430978,3.15436629462203));
#55846=CARTESIAN_POINT('Ctrl Pts',(-16.1859815099194,21.9854654363101,3.2258598790665));
#55847=CARTESIAN_POINT('Ctrl Pts',(-16.1829665819188,21.9707542512648,3.33325881028339));
#55848=CARTESIAN_POINT('Ctrl Pts',(-16.1886594487158,21.9608489185629,3.40496390278775));
#55849=CARTESIAN_POINT('Ctrl Pts',(-16.1947028831469,21.9546309218519,3.44981433014988));
#55850=CARTESIAN_POINT('Ctrl Pts',(-16.1960370051889,21.953385286737,3.45879111255802));
#55851=CARTESIAN_POINT('Ctrl Pts',(-16.198954525102,21.9508943481814,3.47672737206541));
#55852=CARTESIAN_POINT('Ctrl Pts',(-16.2036886600536,21.9471719103735,3.50350885086792));
#55853=CARTESIAN_POINT('Ctrl Pts',(-16.2094820387957,21.943491629387,3.52992662971199));
#55854=CARTESIAN_POINT('Ctrl Pts',(-16.2224555305134,21.9361888154331,3.58228639799885));
#55855=CARTESIAN_POINT('Ctrl Pts',(-16.243443740362,21.926605150889,3.65083327008112));
#55856=CARTESIAN_POINT('Ctrl Pts',(-16.2717387445229,21.9173594545968,3.71687788011058));
#55857=CARTESIAN_POINT('Ctrl Pts',(-16.2917644766302,21.9117030148381,3.7573558784022));
#55858=CARTESIAN_POINT('Ctrl Pts',(-16.2958870189328,21.9105778618014,3.76541137344736));
#55859=CARTESIAN_POINT('Ctrl Pts',(-16.3043697052139,21.9083403604339,3.78144124856931));
#55860=CARTESIAN_POINT('Ctrl Pts',(-16.3087328107494,21.9072272829545,3.78942086022403));
#55861=CARTESIAN_POINT('Ctrl Pts',(-16.322164701551,21.9039128024683,3.81320292616586));
#55862=CARTESIAN_POINT('Ctrl Pts',(-16.3502131607211,21.897428434432,3.85981308323516));
#55863=CARTESIAN_POINT('Ctrl Pts',(-16.4027322179389,21.8873501734346,3.93285235362841));
#55864=CARTESIAN_POINT('Ctrl Pts',(-16.4507908256363,21.8801055090351,3.98642820570205));
#55865=CARTESIAN_POINT('Ctrl Pts',(-16.489139535366,21.8750052615153,4.02476122756083));
#55866=CARTESIAN_POINT('Ctrl Pts',(-16.5023073928949,21.8733608411019,4.03723009232507));
#55867=CARTESIAN_POINT('Ctrl Pts',(-16.5226493863467,21.8709822151684,4.05546028919251));
#55868=CARTESIAN_POINT('Ctrl Pts',(-16.5295361102566,21.8702031867554,4.06146456476965));
#55869=CARTESIAN_POINT('Ctrl Pts',(-16.543474562978,21.8686791236909,4.07328378046564));
#55870=CARTESIAN_POINT('Ctrl Pts',(-16.5786505469972,21.8649629318275,4.10228849368512));
#55871=CARTESIAN_POINT('Ctrl Pts',(-16.6448850977027,21.8591153975305,4.14969206171699));
#55872=CARTESIAN_POINT('Ctrl Pts',(-16.7078023052139,21.8551318036597,4.18517776427292));
#55873=CARTESIAN_POINT('Ctrl Pts',(-16.7565201517863,21.8526184966066,4.20927636685549));
#55874=CARTESIAN_POINT('Ctrl Pts',(-16.7812623913296,21.8514806347264,4.2206953758905));
#55875=CARTESIAN_POINT('Ctrl Pts',(-16.8065901477069,21.8505264209456,4.23115186259816));
#55876=CARTESIAN_POINT('Ctrl Pts',(-16.823607193619,21.849931839782,4.23790608915463));
#55877=CARTESIAN_POINT('Ctrl Pts',(-16.832186504007,21.8496552608978,4.24117617269013));
#55878=CARTESIAN_POINT('Ctrl Pts',(-16.8751402484291,21.8483856367268,4.25688013740921));
#55879=CARTESIAN_POINT('Ctrl Pts',(-16.9446525228319,21.8470617787459,4.27805545503759));
#55880=CARTESIAN_POINT('Ctrl Pts',(-17.051203088172,21.847149288382,4.29835081221195));
#55881=CARTESIAN_POINT('Ctrl Pts',(-17.1237622003836,21.8485913694647,4.30421603447309));
#55882=CARTESIAN_POINT('Ctrl Pts',(-17.1604382594737,21.8496676025262,4.30515623695262));
#55883=CARTESIAN_POINT('Origin',(6.61363325216158E-15,22.,8.67361737988404E-16));
#55884=CARTESIAN_POINT('Origin',(-16.9705627484772,22.,1.));
#55885=CARTESIAN_POINT('Origin',(6.61363325216158E-15,21.5,8.67361737988404E-16));
#55886=CARTESIAN_POINT('Ctrl Pts',(-16.9705627484772,21.5,1.));
#55887=CARTESIAN_POINT('Ctrl Pts',(-16.4714285499925,21.5,0.970588235294119));
#55888=CARTESIAN_POINT('Ctrl Pts',(-16.4714285499925,22.,0.970588235294118));
#55889=CARTESIAN_POINT('Ctrl Pts',(-16.9730924147114,21.5,0.978535066559706));
#55890=CARTESIAN_POINT('Ctrl Pts',(-16.4726248688848,21.4987357550958,0.950286027904117));
#55891=CARTESIAN_POINT('Ctrl Pts',(-16.4738838149159,21.9999999929056,0.928921007848723));
#55892=CARTESIAN_POINT('Ctrl Pts',(-16.9754317317103,21.4986236405249,0.957298789971464));
#55893=CARTESIAN_POINT('Ctrl Pts',(-16.473800294324,21.4962631113247,0.930413747061852));
#55894=CARTESIAN_POINT('Ctrl Pts',(-16.4761543280373,21.9972472802644,0.887697651229367));
#55895=CARTESIAN_POINT('Ctrl Pts',(-16.9797520531917,21.4932235672925,0.915268418547053));
#55896=CARTESIAN_POINT('Ctrl Pts',(-16.4761285834595,21.4890472146769,0.89129077147285));
#55897=CARTESIAN_POINT('Ctrl Pts',(-16.4803475808381,21.9864471353705,0.806109282953636));
#55898=CARTESIAN_POINT('Ctrl Pts',(-16.9817330388163,21.4891995296268,0.894474005556199));
#55899=CARTESIAN_POINT('Ctrl Pts',(-16.477280626014,21.4843014926403,0.872053955068109));
#55900=CARTESIAN_POINT('Ctrl Pts',(-16.4822703025775,21.9783990610965,0.765743657386917));
#55901=CARTESIAN_POINT('Ctrl Pts',(-16.9844503569915,21.4811576965197,0.863617266846394));
#55902=CARTESIAN_POINT('Ctrl Pts',(-16.478997614542,21.4754624026359,0.843578987364932));
#55903=CARTESIAN_POINT('Ctrl Pts',(-16.4849076993345,21.962315392118,0.705845282930559));
#55904=CARTESIAN_POINT('Ctrl Pts',(-16.9853137502372,21.4781418015439,0.853387668521146));
#55905=CARTESIAN_POINT('Ctrl Pts',(-16.4795681715045,21.4722267570588,0.834149063173336));
#55906=CARTESIAN_POINT('Ctrl Pts',(-16.4857456988577,21.9562836046578,0.685987826630035));
#55907=CARTESIAN_POINT('Ctrl Pts',(-16.9865469689091,21.4731031270861,0.83812930879024));
#55908=CARTESIAN_POINT('Ctrl Pts',(-16.4804215368506,21.4669273082589,0.820090807417157));
#55909=CARTESIAN_POINT('Ctrl Pts',(-16.4869426462451,21.9462062533871,0.656368658489502));
#55910=CARTESIAN_POINT('Ctrl Pts',(-16.9869483441066,21.4713344879556,0.833049325850491));
#55911=CARTESIAN_POINT('Ctrl Pts',(-16.4807060704638,21.4650828708149,0.81541110466952));
#55912=CARTESIAN_POINT('Ctrl Pts',(-16.4873322164795,21.9426689751386,0.646507515166357));
#55913=CARTESIAN_POINT('Ctrl Pts',(-16.9877257789808,21.4676473220122,0.822983872627081));
#55914=CARTESIAN_POINT('Ctrl Pts',(-16.4812706985101,21.4612671112103,0.806139057202684));
#55915=CARTESIAN_POINT('Ctrl Pts',(-16.4880867853405,21.935294644797,0.626968693643048));
#55916=CARTESIAN_POINT('Ctrl Pts',(-16.9881022884415,21.4657273940252,0.817993215794496));
#55917=CARTESIAN_POINT('Ctrl Pts',(-16.4815510701315,21.4592943080115,0.801542122223246));
#55918=CARTESIAN_POINT('Ctrl Pts',(-16.4884522212722,21.9314547874519,0.617280948546226));
#55919=CARTESIAN_POINT('Ctrl Pts',(-16.9899262296916,21.4557510501466,0.793247536974804));
#55920=CARTESIAN_POINT('Ctrl Pts',(-16.4829437859584,21.4491049656455,0.778740039448324));
#55921=CARTESIAN_POINT('Ctrl Pts',(-16.4902225165023,21.9115021026871,0.569245217876393));
#55922=CARTESIAN_POINT('Ctrl Pts',(-16.9911982217854,21.4465691378748,0.774112785120951));
#55923=CARTESIAN_POINT('Ctrl Pts',(-16.4840273309326,21.4399290909792,0.761105698710872));
#55924=CARTESIAN_POINT('Ctrl Pts',(-16.4914570981261,21.8931382758739,0.532101288712044));
#55925=CARTESIAN_POINT('Ctrl Pts',(-16.9934231069503,21.4258556925665,0.737138900069214));
#55926=CARTESIAN_POINT('Ctrl Pts',(-16.4861354093574,21.4194806578111,0.726913881060247));
#55927=CARTESIAN_POINT('Ctrl Pts',(-16.4936165444703,21.8517113850087,0.46032845312769));
#55928=CARTESIAN_POINT('Ctrl Pts',(-16.9943758591795,21.414324206792,0.71929973894501));
#55929=CARTESIAN_POINT('Ctrl Pts',(-16.4871593711862,21.408212854135,0.710365087012568));
#55930=CARTESIAN_POINT('Ctrl Pts',(-16.4945412755648,21.8286484158979,0.42569949159161));
#55931=CARTESIAN_POINT('Ctrl Pts',(-16.9953970848308,21.3984014616618,0.697833076923672));
#55932=CARTESIAN_POINT('Ctrl Pts',(-16.4883990487207,21.3927164742621,0.690342539314858));
#55933=CARTESIAN_POINT('Ctrl Pts',(-16.495532464569,21.796802922745,0.384028914441952));
#55934=CARTESIAN_POINT('Ctrl Pts',(-16.9955928310526,21.3951412010012,0.693581520762139));
#55935=CARTESIAN_POINT('Ctrl Pts',(-16.4886448954113,21.389547103093,0.686372439009793));
#55936=CARTESIAN_POINT('Ctrl Pts',(-16.4957224537866,21.7902824027076,0.375775892704089));
#55937=CARTESIAN_POINT('Ctrl Pts',(-16.9959680297371,21.3884670399167,0.685163197758813));
#55938=CARTESIAN_POINT('Ctrl Pts',(-16.4891323578279,21.3830633781607,0.678500451067321));
#55939=CARTESIAN_POINT('Ctrl Pts',(-16.4960866169799,21.7769340791281,0.359434443248347));
#55940=CARTESIAN_POINT('Ctrl Pts',(-16.9961468750295,21.3850634632371,0.681009770694884));
#55941=CARTESIAN_POINT('Ctrl Pts',(-16.4893731970484,21.3797591439209,0.674611100232451));
#55942=CARTESIAN_POINT('Ctrl Pts',(-16.4962602024104,21.7701269259005,0.351371908294615));
#55943=CARTESIAN_POINT('Ctrl Pts',(-16.9966570591121,21.3746901264464,0.668757101822919));
#55944=CARTESIAN_POINT('Ctrl Pts',(-16.4900845285808,21.3696931424689,0.663121500578075));
#55945=CARTESIAN_POINT('Ctrl Pts',(-16.4967553805512,21.7493802540404,0.327587314353041));
#55946=CARTESIAN_POINT('Ctrl Pts',(-16.9969628806611,21.367543746169,0.660847276778648));
#55947=CARTESIAN_POINT('Ctrl Pts',(-16.4905449680627,21.3627634611966,0.655681319541789));
#55948=CARTESIAN_POINT('Ctrl Pts',(-16.4970522080279,21.7350874917574,0.312232949589363));
#55949=CARTESIAN_POINT('Ctrl Pts',(-16.9977909492914,21.3454263958916,0.637877776038412));
#55950=CARTESIAN_POINT('Ctrl Pts',(-16.4918845932564,21.3413163750418,0.634012177598984));
#55951=CARTESIAN_POINT('Ctrl Pts',(-16.4978559207164,21.6908527929444,0.267645093565885));
#55952=CARTESIAN_POINT('Ctrl Pts',(-16.9982241467675,21.3297798973633,0.623575071775558));
#55953=CARTESIAN_POINT('Ctrl Pts',(-16.4927226159692,21.3261385831506,0.620424702005762));
#55954=CARTESIAN_POINT('Ctrl Pts',(-16.4982763783124,21.6595597954117,0.239881020862232));
#55955=CARTESIAN_POINT('Ctrl Pts',(-16.9987417316421,21.3049641718212,0.603629616735995));
#55956=CARTESIAN_POINT('Ctrl Pts',(-16.4938942111891,21.3019902595213,0.601351128009065));
#55957=CARTESIAN_POINT('Ctrl Pts',(-16.4987787392512,21.6099283432998,0.201163374073859));
#55958=CARTESIAN_POINT('Ctrl Pts',(-16.9988921266689,21.2964672601923,0.597233320088741));
#55959=CARTESIAN_POINT('Ctrl Pts',(-16.4942703351611,21.2937134410915,0.59521430533367));
#55960=CARTESIAN_POINT('Ctrl Pts',(-16.4989247114421,21.5929345210954,0.188747032136024));
#55961=CARTESIAN_POINT('Ctrl Pts',(-16.9990895438383,21.2833789662798,0.588023277146211));
#55962=CARTESIAN_POINT('Ctrl Pts',(-16.4948124151445,21.2809410864574,0.58634835836836));
#55963=CARTESIAN_POINT('Ctrl Pts',(-16.499116321829,21.5667579322043,0.170868714949001));
#55964=CARTESIAN_POINT('Ctrl Pts',(-16.9991506486861,21.278959003145,0.585017379496349));
#55965=CARTESIAN_POINT('Ctrl Pts',(-16.4949893919106,21.2766248913159,0.583450140483979));
#55966=CARTESIAN_POINT('Ctrl Pts',(-16.4991756297338,21.5579180067263,0.165033736025826));
#55967=CARTESIAN_POINT('Ctrl Pts',(-16.9992642464521,21.2700032207303,0.579135459380374));
#55968=CARTESIAN_POINT('Ctrl Pts',(-16.4953358105115,21.2678716432874,0.577769744216801));
#55969=CARTESIAN_POINT('Ctrl Pts',(-16.4992858861356,21.5400064410244,0.153615892381932));
#55970=CARTESIAN_POINT('Ctrl Pts',(-16.9993168223211,21.2654589507784,0.576254390691533));
#55971=CARTESIAN_POINT('Ctrl Pts',(-16.495505551458,21.2634263453468,0.574982645018446));
#55972=CARTESIAN_POINT('Ctrl Pts',(-16.4993369159319,21.5309179011113,0.148023229697779));
#55973=CARTESIAN_POINT('Ctrl Pts',(-16.9995587890305,21.2425697250579,0.562255024254108));
#55974=CARTESIAN_POINT('Ctrl Pts',(-16.4963302414363,21.2410229373867,0.561423225150239));
#55975=CARTESIAN_POINT('Ctrl Pts',(-16.4995717652251,21.4851394518979,0.120847985424646));
#55976=CARTESIAN_POINT('Ctrl Pts',(-16.9996864974581,21.2237270718151,0.552343930390703));
#55977=CARTESIAN_POINT('Ctrl Pts',(-16.4969149739077,21.2225074098179,0.551748630561899));
#55978=CARTESIAN_POINT('Ctrl Pts',(-16.4996957185789,21.4474541433703,0.101608806618414));
#55979=CARTESIAN_POINT('Ctrl Pts',(-16.9998646648994,21.1850170081964,0.535007025860517));
#55980=CARTESIAN_POINT('Ctrl Pts',(-16.497937467953,21.1843269944478,0.534747006217183));
#55981=CARTESIAN_POINT('Ctrl Pts',(-16.4998686448857,21.3700340166527,0.0679548143398367));
#55982=CARTESIAN_POINT('Ctrl Pts',(-16.9999149747695,21.1651494999123,0.527581453344155));
#55983=CARTESIAN_POINT('Ctrl Pts',(-16.4983754282979,21.1646605210359,0.527417269072898));
#55984=CARTESIAN_POINT('Ctrl Pts',(-16.4999174758386,21.3302990004269,0.0535404663248945));
#55985=CARTESIAN_POINT('Ctrl Pts',(-16.9999615835097,21.1345695782299,0.518331609142281));
#55986=CARTESIAN_POINT('Ctrl Pts',(-16.4989206599236,21.1342942076196,0.518256449450954));
#55987=CARTESIAN_POINT('Ctrl Pts',(-16.499962713243,21.2691391561586,0.03558488930072));
#55988=CARTESIAN_POINT('Ctrl Pts',(-16.9999722038594,21.1242461095535,0.515564014231725));
#55989=CARTESIAN_POINT('Ctrl Pts',(-16.4990837274006,21.1240294091075,0.515509487574471));
#55990=CARTESIAN_POINT('Ctrl Pts',(-16.4999730215237,21.2484922195051,0.0302124965614095));
#55991=CARTESIAN_POINT('Ctrl Pts',(-16.9999835208626,21.1085607133984,0.511898164807746));
#55992=CARTESIAN_POINT('Ctrl Pts',(-16.4992996622756,21.1084131980924,0.511865629153836));
#55993=CARTESIAN_POINT('Ctrl Pts',(-16.4999840054778,21.2171214265978,0.0230964383945357));
#55994=CARTESIAN_POINT('Ctrl Pts',(-16.9999865105534,21.103306350935,0.510759293490706));
#55995=CARTESIAN_POINT('Ctrl Pts',(-16.4993667326936,21.1031791513432,0.510732629817123));
#55996=CARTESIAN_POINT('Ctrl Pts',(-16.4999869073623,21.2066127017183,0.0208856881011679));
#55997=CARTESIAN_POINT('Ctrl Pts',(-16.9999913085683,21.0928052333294,0.508659120654602));
#55998=CARTESIAN_POINT('Ctrl Pts',(-16.4994903974202,21.0927131482552,0.508641928307854));
#55999=CARTESIAN_POINT('Ctrl Pts',(-16.4999915641382,21.1856104668105,0.0168088805338418));
#56000=CARTESIAN_POINT('Ctrl Pts',(-16.9999931228912,21.0875500018386,0.507695791798136));
#56001=CARTESIAN_POINT('Ctrl Pts',(-16.4995471133876,21.0874726632328,0.507682173326117));
#56002=CARTESIAN_POINT('Ctrl Pts',(-16.4999933252095,21.1751000035788,0.0149388905328434));
#56003=CARTESIAN_POINT('Ctrl Pts',(-17.0000001629822,21.0612507660885,0.503307616912964));
#56004=CARTESIAN_POINT('Ctrl Pts',(-16.4998053929721,21.0612395973646,0.503308608999867));
#56005=CARTESIAN_POINT('Ctrl Pts',(-16.5000001579872,21.1225015325702,0.00642066583814521));
#56006=CARTESIAN_POINT('Ctrl Pts',(-16.9999999168185,21.0401378114417,0.501162938454188));
#56007=CARTESIAN_POINT('Ctrl Pts',(-16.4999315871971,21.0401353257552,0.501162809927001));
#56008=CARTESIAN_POINT('Ctrl Pts',(-16.4999999193109,21.080275622896,0.00225746843716186));
#56009=CARTESIAN_POINT('Ctrl Pts',(-17.0000000528006,20.9977674399885,0.499555723826538));
#56010=CARTESIAN_POINT('Ctrl Pts',(-16.500026133197,20.9977703241831,0.499555867466912));
#56011=CARTESIAN_POINT('Ctrl Pts',(-16.5000000512018,20.9955348799642,-0.000862418127516337));
#56012=CARTESIAN_POINT('Ctrl Pts',(-17.0000004327897,20.9765100308675,0.500093051759841));
#56013=CARTESIAN_POINT('Ctrl Pts',(-16.4999945261161,20.9765031360088,0.500094127563245));
#56014=CARTESIAN_POINT('Ctrl Pts',(-16.5000004199499,20.9530200614576,0.000180626893516891));
#56015=CARTESIAN_POINT('Ctrl Pts',(-16.9999992958654,20.949845179443,0.502493050353376));
#56016=CARTESIAN_POINT('Ctrl Pts',(-16.4998533288364,20.9498593753611,0.50249165881252));
#56017=CARTESIAN_POINT('Ctrl Pts',(-16.4999993166029,20.8996903589554,0.00483945143427439));
#56018=CARTESIAN_POINT('Ctrl Pts',(-16.9999989479835,20.9444988945152,0.503060911828994));
#56019=CARTESIAN_POINT('Ctrl Pts',(-16.4998199145986,20.9445181653914,0.50305883795362));
#56020=CARTESIAN_POINT('Ctrl Pts',(-16.4999989788889,20.888997789137,0.00594177086414229));
#56021=CARTESIAN_POINT('Ctrl Pts',(-16.9999978061467,20.9338399384988,0.504367397839467));
#56022=CARTESIAN_POINT('Ctrl Pts',(-16.4997430304164,20.9338730534644,0.50436305067304));
#56023=CARTESIAN_POINT('Ctrl Pts',(-16.4999978707081,20.8676798768911,0.00847788908051538));
#56024=CARTESIAN_POINT('Ctrl Pts',(-16.9999970135041,20.9285349696757,0.505104749276568));
#56025=CARTESIAN_POINT('Ctrl Pts',(-16.4996996337999,20.9285767396921,0.505098840478412));
#56026=CARTESIAN_POINT('Ctrl Pts',(-16.4999971012969,20.8570699394581,0.00990921985109947));
#56027=CARTESIAN_POINT('Ctrl Pts',(-16.9999935826483,20.9126925582127,0.507565588529774));
#56028=CARTESIAN_POINT('Ctrl Pts',(-16.4995547778939,20.9127662249117,0.507552986668588));
#56029=CARTESIAN_POINT('Ctrl Pts',(-16.4999937714846,20.8253851162119,0.0146861411058046));
#56030=CARTESIAN_POINT('Ctrl Pts',(-16.9999899191601,20.9022275356819,0.509537601288132));
#56031=CARTESIAN_POINT('Ctrl Pts',(-16.4994386694513,20.9023313755917,0.509517878518783));
#56032=CARTESIAN_POINT('Ctrl Pts',(-16.4999902155292,20.8044550715146,0.018514167866819));
#56033=CARTESIAN_POINT('Ctrl Pts',(-16.9999707269349,20.8711168396759,0.516429520854516));
#56034=CARTESIAN_POINT('Ctrl Pts',(-16.4990327235418,20.8713427933764,0.516372901480069));
#56035=CARTESIAN_POINT('Ctrl Pts',(-16.4999715881597,20.7422336790502,0.0318925979849346));
#56036=CARTESIAN_POINT('Ctrl Pts',(-16.9999474621371,20.8507544093414,0.52232143473415));
#56037=CARTESIAN_POINT('Ctrl Pts',(-16.498685458987,20.8511091143981,0.522220449062311));
#56038=CARTESIAN_POINT('Ctrl Pts',(-16.4999490069737,20.7015088182385,0.0433298426955125));
#56039=CARTESIAN_POINT('Ctrl Pts',(-16.999872593906,20.8207774110138,0.533103835838787));
#56040=CARTESIAN_POINT('Ctrl Pts',(-16.49804985819,20.8214264933554,0.532857061552179));
#56041=CARTESIAN_POINT('Ctrl Pts',(-16.4998763413414,20.6415548222497,0.0642603878165643));
#56042=CARTESIAN_POINT('Ctrl Pts',(-16.9998408653516,20.8108798020863,0.537023027180669));
#56043=CARTESIAN_POINT('Ctrl Pts',(-16.4978187255782,20.811640257904,0.536715854407526));
#56044=CARTESIAN_POINT('Ctrl Pts',(-16.4998455455476,20.6217596036359,0.0718682280307113));
#56045=CARTESIAN_POINT('Ctrl Pts',(-16.9997583144814,20.7912774765208,0.545523339639611));
#56046=CARTESIAN_POINT('Ctrl Pts',(-16.4973174053915,20.7922932250178,0.545060273323437));
#56047=CARTESIAN_POINT('Ctrl Pts',(-16.4997654231138,20.5825549535782,0.088368836973362));
#56048=CARTESIAN_POINT('Ctrl Pts',(-16.9997073352247,20.7815527714696,0.550115598300045));
#56049=CARTESIAN_POINT('Ctrl Pts',(-16.4970465330306,20.7827124914974,0.549557176956291));
#56050=CARTESIAN_POINT('Ctrl Pts',(-16.4997159433886,20.5631055157649,0.0972832302481202));
#56051=CARTESIAN_POINT('Ctrl Pts',(-16.9996439954592,20.7720018726588,0.555009152983024));
#56052=CARTESIAN_POINT('Ctrl Pts',(-16.4967580121734,20.7733226724976,0.554332420210074));
#56053=CARTESIAN_POINT('Ctrl Pts',(-16.499654466181,20.5440037453175,0.106782473437634));
#56054=CARTESIAN_POINT('Origin',(-28.5,21.,1.));
#56055=CARTESIAN_POINT('Origin',(-17.5,24.,-29.5));
#56056=CARTESIAN_POINT('Origin',(6.61287431064084E-15,53.,0.));
#56057=CARTESIAN_POINT('',(-15.2695685015073,52.,12.9166666666667));
#56058=CARTESIAN_POINT('Origin',(-15.2695685015073,53.,12.9166666666667));
#56059=CARTESIAN_POINT('',(-15.2695685015073,52.,-12.9166666666666));
#56060=CARTESIAN_POINT('Origin',(-15.2695685015073,53.,-12.9166666666667));
#56061=CARTESIAN_POINT('Origin',(6.61287431064084E-15,52.,0.));
#56062=CARTESIAN_POINT('Origin',(-45.2928932188135,48.4656487624794,-19.0077234952746));
#56063=CARTESIAN_POINT('',(-45.2928932188135,48.0436073736659,-18.7396170497563));
#56064=CARTESIAN_POINT('',(-45.2928932188135,48.7337552079976,-18.5856821064611));
#56065=CARTESIAN_POINT('Origin',(-45.2928932188135,48.4656487624794,-19.0077234952746));
#56066=CARTESIAN_POINT('',(-45.6464466094067,48.6552286481851,-18.7092951673032));
#56067=CARTESIAN_POINT('Origin',(-45.2928932188135,48.4656487624794,-19.0077234952746));
#56068=CARTESIAN_POINT('Origin',(-45.2928932188135,48.4656487624794,-19.0077234952746));
#56069=CARTESIAN_POINT('Origin',(-50.,48.4656487624794,-19.0077234952746));
#56070=CARTESIAN_POINT('',(-50.,48.7337552079976,-18.5856821064611));
#56071=CARTESIAN_POINT('',(-50.,48.0436073736659,-18.7396170497563));
#56072=CARTESIAN_POINT('Origin',(-45.2928932188135,51.4199384841736,-20.884468613902));
#56073=CARTESIAN_POINT('',(-45.2928932188135,51.2660035408783,-20.1943207795704));
#56074=CARTESIAN_POINT('',(-45.6464466094067,51.1874769810659,-20.3179338404124));
#56075=CARTESIAN_POINT('Origin',(-45.2928932188135,50.9978970953601,-20.6163621683838));
#56076=CARTESIAN_POINT('',(-45.6464466094067,51.6095183698793,-20.5860402859306));
#56077=CARTESIAN_POINT('',(-45.2928932188135,48.3117138191841,-18.3175756609429));
#56078=CARTESIAN_POINT('Origin',(-36.5,53.9282032302755,-24.));
#56079=CARTESIAN_POINT('',(-37.,53.9282032302755,-24.));
#56080=CARTESIAN_POINT('',(-36.5,54.4282032302755,-24.));
#56081=CARTESIAN_POINT('Origin',(-36.5,53.9282032302755,-24.));
#56082=CARTESIAN_POINT('',(-36.5,53.9282032302755,-24.5));
#56083=CARTESIAN_POINT('Origin',(-36.5,53.9282032302755,-24.));
#56084=CARTESIAN_POINT('Origin',(-36.5,53.9282032302755,-24.));
#56085=CARTESIAN_POINT('Origin',(-36.5,53.9282032302755,0.));
#56086=CARTESIAN_POINT('',(-37.,53.9282032302755,-17.5));
#56087=CARTESIAN_POINT('',(-36.5,54.4282032302755,-17.5));
#56088=CARTESIAN_POINT('Origin',(-36.5,53.9282032302755,-17.5));
#56089=CARTESIAN_POINT('',(-36.5,54.4282032302755,-17.));
#56090=CARTESIAN_POINT('',(-37.,53.9282032302755,-24.5));
#56091=CARTESIAN_POINT('Origin',(-37.,53.9282032302755,-24.));
#56092=CARTESIAN_POINT('',(-6.78091634720693,53.9282032302755,-24.5));
#56093=CARTESIAN_POINT('',(-7.20387088797839,54.4282032302755,-24.));
#56094=CARTESIAN_POINT('Origin',(-7.20387088797737,53.9282032302767,-24.0000000000012));
#56095=CARTESIAN_POINT('',(-37.,53.9282032302755,-24.5));
#56096=CARTESIAN_POINT('',(-37.,54.4282032302755,-24.));
#56097=CARTESIAN_POINT('Origin',(-36.5,53.9282032302755,-17.5));
#56098=CARTESIAN_POINT('',(-36.5,53.9282032302755,-17.));
#56099=CARTESIAN_POINT('Origin',(-36.5,53.9282032302755,-17.5));
#56100=CARTESIAN_POINT('Origin',(-36.5,53.9282032302755,-17.5));
#56101=CARTESIAN_POINT('Origin',(-36.5,3.36766747301154E-16,-17.5));
#56102=CARTESIAN_POINT('',(-37.,45.4641016151378,-17.5));
#56103=CARTESIAN_POINT('',(-36.5,45.4641016151378,-17.));
#56104=CARTESIAN_POINT('Origin',(-36.5,45.4641016151378,-17.5));
#56105=CARTESIAN_POINT('',(-36.5,44.9641016151378,-17.));
#56106=CARTESIAN_POINT('',(-37.,54.4282032302755,-17.5));
#56107=CARTESIAN_POINT('Origin',(-37.,53.9282032302755,-17.5));
#56108=CARTESIAN_POINT('',(-12.7022799180074,54.4282032302755,-17.5));
#56109=CARTESIAN_POINT('',(-13.1252344587788,53.9282032302755,-17.));
#56110=CARTESIAN_POINT('Origin',(-12.702279918008,53.9282032302763,-17.4999999999992));
#56111=CARTESIAN_POINT('',(-37.,54.4282032302755,-17.5));
#56112=CARTESIAN_POINT('',(-37.,53.9282032302755,-17.));
#56113=CARTESIAN_POINT('Origin',(-36.5,45.4641016151378,-17.5));
#56114=CARTESIAN_POINT('',(-36.5,44.9641016151378,-17.5));
#56115=CARTESIAN_POINT('Origin',(-36.5,45.4641016151378,-17.5));
#56116=CARTESIAN_POINT('Origin',(-36.5,45.4641016151378,-17.5));
#56117=CARTESIAN_POINT('Origin',(-36.5,45.4641016151375,6.30941155087793E-13));
#56118=CARTESIAN_POINT('',(-36.5,44.9641016151378,-23.5872397343813));
#56119=CARTESIAN_POINT('',(-37.,45.4641016151378,-22.800161699018));
#56120=CARTESIAN_POINT('Origin',(-36.5000000000005,45.4641016151372,-22.8001616990189));
#56121=CARTESIAN_POINT('',(-36.5,44.9641016151378,-23.5872397343815));
#56122=CARTESIAN_POINT('',(-37.,45.4641016151378,-17.));
#56123=CARTESIAN_POINT('Origin',(-6.5,41.0779586111866,-36.2318935544818));
#56124=CARTESIAN_POINT('',(-6.5,49.1231323076242,-24.5));
#56125=CARTESIAN_POINT('',(-6.5,41.5,-36.5));
#56126=CARTESIAN_POINT('',(-6.,48.8484038560691,-24.));
#56127=CARTESIAN_POINT('Origin',(-6.49999999999975,48.8484038560692,-24.0000000000003));
#56128=CARTESIAN_POINT('',(-6.,45.6658960598572,-29.0097639675421));
#56129=CARTESIAN_POINT('Origin',(-6.5,38.813816723824,-34.2012134925591));
#56130=CARTESIAN_POINT('',(-6.,38.813816723824,-34.2012134925591));
#56131=CARTESIAN_POINT('',(-6.5,38.5457102783057,-34.6232548813726));
#56132=CARTESIAN_POINT('Origin',(-6.5,38.813816723824,-34.2012134925591));
#56133=CARTESIAN_POINT('',(-6.5,38.3917753350105,-33.9331070470409));
#56134=CARTESIAN_POINT('Origin',(-6.5,38.813816723824,-34.2012134925591));
#56135=CARTESIAN_POINT('Origin',(-6.5,38.813816723824,-34.2012134925591));
#56136=CARTESIAN_POINT('Origin',(-6.5,41.7681064455182,-36.0779586111866));
#56137=CARTESIAN_POINT('',(-6.5,41.5,-36.5));
#56138=CARTESIAN_POINT('',(-6.,-4.31983100315249,-6.80008819812621));
#56139=CARTESIAN_POINT('Origin',(-45.2928932188134,41.7681064455182,-36.0779586111866));
#56140=CARTESIAN_POINT('',(-45.2928932188134,38.5457102783057,-34.6232548813726));
#56141=CARTESIAN_POINT('',(-45.6464466094067,38.6242368381183,-34.4996418205305));
#56142=CARTESIAN_POINT('Origin',(-45.2928932188135,38.813816723824,-34.2012134925591));
#56143=CARTESIAN_POINT('',(-45.6464466094067,38.2021954493047,-34.2315353750123));
#56144=CARTESIAN_POINT('Origin',(-45.2928932188134,41.3460650567048,-35.8098521656684));
#56145=CARTESIAN_POINT('',(-45.2928932188134,41.5,-36.5));
#56146=CARTESIAN_POINT('Origin',(-45.2928932188135,38.813816723824,-34.2012134925591));
#56147=CARTESIAN_POINT('',(-45.2928932188135,38.3917753350105,-33.9331070470409));
#56148=CARTESIAN_POINT('Origin',(-45.2928932188134,38.813816723824,-34.2012134925591));
#56149=CARTESIAN_POINT('Origin',(-45.2928932188135,38.813816723824,-34.2012134925591));
#56150=CARTESIAN_POINT('Origin',(-50.,38.813816723824,-34.2012134925591));
#56151=CARTESIAN_POINT('',(-50.,38.3917753350105,-33.9331070470409));
#56152=CARTESIAN_POINT('',(-50.,38.5457102783057,-34.6232548813726));
#56153=CARTESIAN_POINT('Origin',(-47.3964466094067,39.9417691688435,-32.4256403037406));
#56154=CARTESIAN_POINT('',(-49.5,40.6476802250494,-30.3819606694039));
#56155=CARTESIAN_POINT('',(-45.1464466094067,38.313248775198,-34.056720107883));
#56156=CARTESIAN_POINT('',(-49.8535533905933,40.8801417281571,-30.9484954428935));
#56157=CARTESIAN_POINT('Origin',(-49.5,41.0697216138629,-30.6500671149221));
#56158=CARTESIAN_POINT('',(-50.,40.9586682879697,-30.8248823820514));
#56159=CARTESIAN_POINT('Origin',(-49.5,-2.06392611311356,-3.24894182048922));
#56160=CARTESIAN_POINT('',(-50.,41.0697216138629,-30.6500671149221));
#56161=CARTESIAN_POINT('Origin',(-49.5,41.0697216138629,-30.6500671149221));
#56162=CARTESIAN_POINT('',(-50.,-2.06392611311356,-3.24894182048923));
#56163=CARTESIAN_POINT('',(-49.8535533905933,-2.2535059988193,-3.54737014846061));
#56164=CARTESIAN_POINT('Origin',(-49.5,41.0697216138629,-30.6500671149221));
#56165=CARTESIAN_POINT('Origin',(-49.5,41.0697216138629,-30.6500671149221));
#56166=CARTESIAN_POINT('Origin',(-49.5,43.1336477269765,-27.4011252944329));
#56167=CARTESIAN_POINT('',(-50.,43.1035198521152,-27.4485512715437));
#56168=CARTESIAN_POINT('',(-49.5,40.5366268991562,-30.5567759365332));
#56169=CARTESIAN_POINT('Origin',(-6.5,38.5457102783057,-34.6232548813726));
#56170=CARTESIAN_POINT('',(-6.,40.2323075626015,-31.9682875274271));
#56171=CARTESIAN_POINT('',(-6.,43.1336477269765,-27.4011252944329));
#56172=CARTESIAN_POINT('',(-6.5,39.7323075626015,-31.8229001029736));
#56173=CARTESIAN_POINT('Origin',(-6.5000000000006,40.2323075626021,-31.9682875274273));
#56174=CARTESIAN_POINT('',(-6.5,38.1236688894923,-34.3551484358543));
#56175=CARTESIAN_POINT('Origin',(-45.2928932188135,41.3460650567048,-35.8098521656684));
#56176=CARTESIAN_POINT('Origin',(-49.5,45.6658960598572,-29.0097639675421));
#56177=CARTESIAN_POINT('',(-50.,48.7419922053212,-24.1675085460208));
#56178=CARTESIAN_POINT('',(-50.,46.7081939670689,-27.3690243893992));
#56179=CARTESIAN_POINT('',(-49.5,49.1640335941347,-24.435614991539));
#56180=CARTESIAN_POINT('Origin',(-49.5,48.7419922053212,-24.1675085460208));
#56181=CARTESIAN_POINT('',(-49.5,49.275086920028,-24.2607997244097));
#56182=CARTESIAN_POINT('Origin',(-49.5,48.7419922053212,-24.1675085460208));
#56183=CARTESIAN_POINT('',(-49.8535533905933,48.931572091027,-23.8690802180494));
#56184=CARTESIAN_POINT('Origin',(-49.5,48.7419922053212,-24.1675085460208));
#56185=CARTESIAN_POINT('Origin',(-49.5,48.7419922053212,-24.1675085460208));
#56186=CARTESIAN_POINT('Origin',(-56.8964466094067,44.7759221854948,-30.4107217446581));
#56187=CARTESIAN_POINT('',(-45.2928932188135,51.4199384841736,-20.884468613902));
#56188=CARTESIAN_POINT('Origin',(-45.2928932188135,50.9978970953601,-20.6163621683838));
#56189=CARTESIAN_POINT('',(-45.1464466094067,51.4984650439861,-20.7608555530599));
#56190=CARTESIAN_POINT('',(-50.,48.8530455312145,-23.9926932788915));
#56191=CARTESIAN_POINT('Origin',(-56.8964466094067,42.243673852614,-28.8020830715488));
#56192=CARTESIAN_POINT('',(-45.5,48.7337552079976,-18.5856821064611));
#56193=CARTESIAN_POINT('',(-49.6464466094067,45.7091759238145,-22.4143764882355));
#56194=CARTESIAN_POINT('Origin',(-49.5,3.07609614546394,4.8422554215213));
#56195=CARTESIAN_POINT('',(-50.,3.07609614546394,4.84225542152131));
#56196=CARTESIAN_POINT('',(-49.8535533905933,3.26567603116969,5.14068374949269));
#56197=CARTESIAN_POINT('Origin',(-49.5,43.1336477269765,-27.4011252944329));
#56198=CARTESIAN_POINT('',(-50.,44.1759456341881,-25.7603857162899));
#56199=CARTESIAN_POINT('',(-50.,46.3207971983337,-22.3840546057823));
#56200=CARTESIAN_POINT('',(-49.5,44.0220106908928,-25.0702378819582));
#56201=CARTESIAN_POINT('Origin',(-49.5000000000009,44.444052079705,-25.3383443274766));
#56202=CARTESIAN_POINT('',(-49.5,43.7539042453746,-25.4922792707717));
#56203=CARTESIAN_POINT('Origin',(-37.,54.4282032302755,-17.));
#56204=CARTESIAN_POINT('',(-4.19913133791448,54.4282032302755,-27.5520833333334));
#56205=CARTESIAN_POINT('Origin',(-37.,3.67381906146713E-16,0.));
#56206=CARTESIAN_POINT('',(-37.,51.5341099863965,-19.7722793907569));
#56207=CARTESIAN_POINT('',(-37.,5.86821392653928,9.23748457678522));
#56208=CARTESIAN_POINT('',(-37.,38.1236688894923,-34.3551484358543));
#56209=CARTESIAN_POINT('',(-37.,50.0331217848147,-24.));
#56210=CARTESIAN_POINT('',(-37.,49.1231323076242,-24.));
#56211=CARTESIAN_POINT('',(-37.,51.8419798729871,-21.1525750594202));
#56212=CARTESIAN_POINT('',(-37.,46.5099788374842,-29.5459768585786));
#56213=CARTESIAN_POINT('Origin',(-37.,50.9978970953601,-20.6163621683838));
#56214=CARTESIAN_POINT('Origin',(-37.,44.9641016151378,-24.5));
#56215=CARTESIAN_POINT('',(-10.,44.9641016151378,-23.5872397343813));
#56216=CARTESIAN_POINT('',(-10.,44.9641016151378,-17.5));
#56217=CARTESIAN_POINT('',(-10.,44.9641016151375,6.24002261183886E-13));
#56218=CARTESIAN_POINT('',(-37.,44.9641016151378,-17.5));
#56219=CARTESIAN_POINT('',(-50.,44.9641016151378,-23.5872397343813));
#56220=CARTESIAN_POINT('Origin',(-37.,44.9641016151378,-17.));
#56221=CARTESIAN_POINT('',(-10.,45.4641016151378,-17.));
#56222=CARTESIAN_POINT('',(-10.,51.,-17.));
#56223=CARTESIAN_POINT('',(-10.,3.67381906146713E-16,-17.));
#56224=CARTESIAN_POINT('',(-11.,52.,-17.));
#56225=CARTESIAN_POINT('Origin',(-11.,51.,-17.));
#56226=CARTESIAN_POINT('',(-11.8154397518737,52.,-17.));
#56227=CARTESIAN_POINT('',(6.61363325216158E-15,52.,-17.));
#56228=CARTESIAN_POINT('',(-13.1252344587788,53.,-17.));
#56229=CARTESIAN_POINT('Origin',(-11.8154397518729,53.0000000000004,-17.));
#56230=CARTESIAN_POINT('',(-13.1252344587788,57.,-17.));
#56231=CARTESIAN_POINT('',(-37.,45.4641016151378,-17.));
#56232=CARTESIAN_POINT('Origin',(33.,25.8967919448979,4.98934246731003));
#56233=CARTESIAN_POINT('',(15.863798335516,26.6272203612273,4.67630172554642));
#56234=CARTESIAN_POINT('Origin',(16.7453756123118,26.2781107809041,4.82592044071226));
#56235=CARTESIAN_POINT('',(16.0339930597927,26.2575776988747,4.83472006237606));
#56236=CARTESIAN_POINT('Origin',(16.8887635278285,26.8426106081843,4.58399492666055));
#56237=CARTESIAN_POINT('',(33.,26.2575776350368,4.83472002867911));
#56238=CARTESIAN_POINT('',(33.,26.2575776350368,4.83472002867911));
#56239=CARTESIAN_POINT('',(33.,25.8967919448979,4.98934246731003));
#56240=CARTESIAN_POINT('Origin',(0.5,48.5249973351313,-4.97500266486866));
#56241=CARTESIAN_POINT('',(5.4811647369232,19.0972134699726,-33.7896016253977));
#56242=CARTESIAN_POINT('Ctrl Pts',(5.47974928497604,19.0969304167095,-33.767306956549));
#56243=CARTESIAN_POINT('Ctrl Pts',(5.48022993085033,19.0970264611248,-33.7747404391871));
#56244=CARTESIAN_POINT('Ctrl Pts',(5.48070183516169,19.097120832269,-33.7821735628567));
#56245=CARTESIAN_POINT('Ctrl Pts',(5.4811647369232,19.0972134699726,-33.7896016253977));
#56246=CARTESIAN_POINT('Origin',(0.5,19.4038059222875,-34.0961940777126));
#56247=CARTESIAN_POINT('Origin',(-27.5,24.,-29.5));
#56248=CARTESIAN_POINT('',(-27.5,23.5,-23.));
#56249=CARTESIAN_POINT('',(-27.5,23.5,-29.5));
#56250=CARTESIAN_POINT('',(-27.5,24.5,-23.));
#56251=CARTESIAN_POINT('',(-27.5,23.5,-23.));
#56252=CARTESIAN_POINT('',(-27.5,24.5,-29.5));
#56253=CARTESIAN_POINT('Origin',(4.5,24.,-37.));
#56254=CARTESIAN_POINT('',(0.5,22.3076118445749,-37.));
#56255=CARTESIAN_POINT('',(-2.35233629352793,22.3076118445749,-37.));
#56256=CARTESIAN_POINT('',(0.5,22.3076118445749,-37.));
#56257=CARTESIAN_POINT('Origin',(0.499999999976273,16.5000000000764,-36.9999999999998));
#56258=CARTESIAN_POINT('Origin',(4.5,24.,6.93889390390723E-15));
#56259=CARTESIAN_POINT('Origin',(4.49999999937185,24.0000000020693,-38.6923881574814));
#56260=CARTESIAN_POINT('Origin',(0.5,19.4038059222875,-34.0961940777126));
#56261=CARTESIAN_POINT('Origin',(0.5,19.4038059222875,-34.0961940777126));
#56262=CARTESIAN_POINT('Origin',(9.,24.,-29.5));
#56263=CARTESIAN_POINT('',(9.5,21.9882004875966,-35.152668637192));
#56264=CARTESIAN_POINT('Origin',(9.,21.9882004875966,-35.152668637192));
#56265=CARTESIAN_POINT('',(9.5,21.9882004875966,-23.847331362808));
#56266=CARTESIAN_POINT('Origin',(9.5,24.,-29.5));
#56267=CARTESIAN_POINT('Origin',(9.,21.9882004875966,-23.847331362808));
#56268=CARTESIAN_POINT('Ctrl Pts',(9.5,26.0117995124037,-35.1526686371919));
#56269=CARTESIAN_POINT('Ctrl Pts',(9.50000000000001,26.1794494717706,-35.623724356958));
#56270=CARTESIAN_POINT('Ctrl Pts',(8.99999999999989,26.1794494717706,-35.6237243569579));
#56271=CARTESIAN_POINT('Ctrl Pts',(9.5,25.969126524566,-35.1678560713817));
#56272=CARTESIAN_POINT('Ctrl Pts',(9.50000000000001,26.1363858923875,-35.6200054618018));
#56273=CARTESIAN_POINT('Ctrl Pts',(9.01826917526509,26.1417283486801,-35.6371494030576));
#56274=CARTESIAN_POINT('Ctrl Pts',(9.5,25.9266618092262,-35.1837246773205));
#56275=CARTESIAN_POINT('Ctrl Pts',(9.49999999999997,26.0919477789377,-35.6183024929583));
#56276=CARTESIAN_POINT('Ctrl Pts',(9.03631589192574,26.1032568243223,-35.6504486521462));
#56277=CARTESIAN_POINT('Ctrl Pts',(9.5,25.8420590117766,-35.21653092188));
#56278=CARTESIAN_POINT('Ctrl Pts',(9.50000000000005,26.0025448380055,-35.6183771479464));
#56279=CARTESIAN_POINT('Ctrl Pts',(9.07183836849202,26.0248814931803,-35.6766951383499));
#56280=CARTESIAN_POINT('Ctrl Pts',(9.5,25.7999211590539,-35.2334691645038));
#56281=CARTESIAN_POINT('Ctrl Pts',(9.50000000000001,25.9574863153535,-35.6200467193352));
#56282=CARTESIAN_POINT('Ctrl Pts',(9.08931415962551,25.9849775488743,-35.6896423865758));
#56283=CARTESIAN_POINT('Ctrl Pts',(9.5,25.7158975753409,-35.2681705887087));
#56284=CARTESIAN_POINT('Ctrl Pts',(9.49999999999999,25.8671165675929,-35.6260854809282));
#56285=CARTESIAN_POINT('Ctrl Pts',(9.1235736889288,25.9038137144825,-35.7150866515789));
#56286=CARTESIAN_POINT('Ctrl Pts',(9.5,25.6740028719298,-35.2859382131717));
#56287=CARTESIAN_POINT('Ctrl Pts',(9.5,25.8216976115558,-35.6303888638396));
#56288=CARTESIAN_POINT('Ctrl Pts',(9.14036084384017,25.8625443955667,-35.7275862152158));
#56289=CARTESIAN_POINT('Ctrl Pts',(9.5,25.5904820429837,-35.322051972562));
#56290=CARTESIAN_POINT('Ctrl Pts',(9.5,25.7308556139648,-35.6410699898064));
#56291=CARTESIAN_POINT('Ctrl Pts',(9.17309573545697,25.7788188856162,-35.7520160803084));
#56292=CARTESIAN_POINT('Ctrl Pts',(9.5,25.54884683225,-35.3404019499814));
#56293=CARTESIAN_POINT('Ctrl Pts',(9.50000000000001,25.6853264252681,-35.6474086022825));
#56294=CARTESIAN_POINT('Ctrl Pts',(9.18904735031175,25.7363542059438,-35.7639492338914));
#56295=CARTESIAN_POINT('Ctrl Pts',(9.5,25.4242015033402,-35.3960612434519));
#56296=CARTESIAN_POINT('Ctrl Pts',(9.50000000000001,25.5502828319477,-35.6685604400058));
#56297=CARTESIAN_POINT('Ctrl Pts',(9.23550610480808,25.607279019684,-35.7987774920106));
#56298=CARTESIAN_POINT('Ctrl Pts',(9.5,25.3414487728041,-35.433973095274));
#56299=CARTESIAN_POINT('Ctrl Pts',(9.50000000000009,25.4588206457325,-35.685861865764));
#56300=CARTESIAN_POINT('Ctrl Pts',(9.2646135723705,25.5189820341969,-35.8206987330504));
#56301=CARTESIAN_POINT('Ctrl Pts',(9.5,25.176109276692,-35.5101853172836));
#56302=CARTESIAN_POINT('Ctrl Pts',(9.49999999999992,25.2766858194012,-35.7237734257663));
#56303=CARTESIAN_POINT('Ctrl Pts',(9.31837705316277,25.3386902127447,-35.8613243440875));
#56304=CARTESIAN_POINT('Ctrl Pts',(9.5,25.0935237034198,-35.5484884786143));
#56305=CARTESIAN_POINT('Ctrl Pts',(9.49999999999992,25.1853323050273,-35.7444076007431));
#56306=CARTESIAN_POINT('Ctrl Pts',(9.34303153817123,25.2466967857052,-35.8800272698057));
#56307=CARTESIAN_POINT('Ctrl Pts',(9.5,24.9280807136363,-35.6244584254345));
#56308=CARTESIAN_POINT('Ctrl Pts',(9.50000000000008,25.0033399898978,-35.7867586891882));
#56309=CARTESIAN_POINT('Ctrl Pts',(9.38729861344404,25.0599620838701,-35.9136948179777));
#56310=CARTESIAN_POINT('Ctrl Pts',(9.5,24.8452239160408,-35.6621266597857));
#56311=CARTESIAN_POINT('Ctrl Pts',(9.5,24.9120763623833,-35.8085867314734));
#56312=CARTESIAN_POINT('Ctrl Pts',(9.40691008519286,24.9652233257944,-35.9286583428068));
#56313=CARTESIAN_POINT('Ctrl Pts',(9.5,24.6788556331735,-35.7359305267538));
#56314=CARTESIAN_POINT('Ctrl Pts',(9.5,24.7301341256831,-35.8516195729549));
#56315=CARTESIAN_POINT('Ctrl Pts',(9.44067629739234,24.7740415871847,-35.9544685122108));
#56316=CARTESIAN_POINT('Ctrl Pts',(9.5,24.5953445434688,-35.7720670853785));
#56317=CARTESIAN_POINT('Ctrl Pts',(9.5,24.6388718622012,-35.8729686489815));
#56318=CARTESIAN_POINT('Ctrl Pts',(9.45483075696681,24.6776017522002,-35.9653147728946));
#56319=CARTESIAN_POINT('Ctrl Pts',(9.5,24.4273258947367,-35.8420075016043));
#56320=CARTESIAN_POINT('Ctrl Pts',(9.5,24.4567995163812,-35.913676588705));
#56321=CARTESIAN_POINT('Ctrl Pts',(9.47746628181506,24.4840675352485,-35.9826782942412));
#56322=CARTESIAN_POINT('Ctrl Pts',(9.5,24.3428186889365,-35.875812186098));
#56323=CARTESIAN_POINT('Ctrl Pts',(9.50000000000009,24.365437407906,-35.9331791082525));
#56324=CARTESIAN_POINT('Ctrl Pts',(9.48594808355023,24.3869762064944,-35.9891960450384));
#56325=CARTESIAN_POINT('Ctrl Pts',(9.5,24.2150771332136,-35.9242233171871));
#56326=CARTESIAN_POINT('Ctrl Pts',(9.49999999999996,24.2284532489845,-35.9601253781755));
#56327=CARTESIAN_POINT('Ctrl Pts',(9.49439707925568,24.2415678655432,-35.9956907978406));
#56328=CARTESIAN_POINT('Ctrl Pts',(9.5,24.1723333665474,-35.939978202615));
#56329=CARTESIAN_POINT('Ctrl Pts',(9.50000000000017,24.1827991755656,-35.9687288907579));
#56330=CARTESIAN_POINT('Ctrl Pts',(9.49650254697548,24.1931355198232,-35.9973099740758));
#56331=CARTESIAN_POINT('Ctrl Pts',(9.5,24.1079451005327,-35.9629723458731));
#56332=CARTESIAN_POINT('Ctrl Pts',(9.49999999999993,24.11429879057,-35.9809702182257));
#56333=CARTESIAN_POINT('Ctrl Pts',(9.49860334653214,24.1206206521294,-35.998925697095));
#56334=CARTESIAN_POINT('Ctrl Pts',(9.5,24.0864369182992,-35.9705307174653));
#56335=CARTESIAN_POINT('Ctrl Pts',(9.49999999999993,24.0914619868762,-35.9849404193503));
#56336=CARTESIAN_POINT('Ctrl Pts',(9.49912745052014,24.0964712112024,-35.9993288281094));
#56337=CARTESIAN_POINT('Ctrl Pts',(9.5,24.0541030972586,-35.9817007841272));
#56338=CARTESIAN_POINT('Ctrl Pts',(9.50000000000002,24.0571981105742,-35.9907188498919));
#56339=CARTESIAN_POINT('Ctrl Pts',(9.49965105814884,24.0602891948851,-35.9997315860922));
#56340=CARTESIAN_POINT('Ctrl Pts',(9.5,24.0433132330065,-35.9853962262216));
#56341=CARTESIAN_POINT('Ctrl Pts',(9.49999999999965,24.0457753673003,-35.9926155427435));
#56342=CARTESIAN_POINT('Ctrl Pts',(9.49978183973438,24.0482355396307,-35.9998321856301));
#56343=CARTESIAN_POINT('Ctrl Pts',(9.5,24.021709091742,-35.9927299609635));
#56344=CARTESIAN_POINT('Ctrl Pts',(9.50000000000013,24.0229268751936,-35.9963480615538));
#56345=CARTESIAN_POINT('Ctrl Pts',(9.49995621937517,24.0241436645304,-35.9999663224548));
#56346=CARTESIAN_POINT('Ctrl Pts',(9.5,24.0109082581165,-35.9963507604577));
#56347=CARTESIAN_POINT('Ctrl Pts',(9.5,24.0115165090366,-35.998175025983));
#56348=CARTESIAN_POINT('Ctrl Pts',(9.5,24.0121234081387,-36.0000000002211));
#56349=CARTESIAN_POINT('Ctrl Pts',(9.5,24.,-36.));
#56350=CARTESIAN_POINT('Ctrl Pts',(9.5,24.,-36.));
#56351=CARTESIAN_POINT('Ctrl Pts',(9.5,24.,-36.));
#56352=CARTESIAN_POINT('Ctrl Pts',(9.5,24.,-36.));
#56353=CARTESIAN_POINT('Ctrl Pts',(9.5,24.0054150064504,-35.9981884682733));
#56354=CARTESIAN_POINT('Ctrl Pts',(9.49999999999458,24.0108043085154,-35.9963861629621));
#56355=CARTESIAN_POINT('Ctrl Pts',(9.49999999999452,24.0161950807351,-35.994574350307));
#56356=CARTESIAN_POINT('Ctrl Pts',(9.49999999999445,24.0215858529548,-35.9927625376518));
#56357=CARTESIAN_POINT('Ctrl Pts',(9.5,24.0269887853828,-35.9909375873191));
#56358=CARTESIAN_POINT('Ctrl Pts',(9.5,24.0323884057965,-35.9891047955571));
#56359=CARTESIAN_POINT('Ctrl Pts',(9.5,24.0431876466238,-35.9854392120329));
#56360=CARTESIAN_POINT('Ctrl Pts',(9.5,24.0539746311336,-35.9817449034163));
#56361=CARTESIAN_POINT('Ctrl Pts',(9.5,24.0647497302229,-35.9780227911426));
#56362=CARTESIAN_POINT('Ctrl Pts',(9.5,24.0862999284017,-35.9705785665953));
#56363=CARTESIAN_POINT('Ctrl Pts',(9.5,24.1078024533637,-35.9630227406302));
#56364=CARTESIAN_POINT('Ctrl Pts',(9.5,24.1292595640221,-35.9553606016205));
#56365=CARTESIAN_POINT('Ctrl Pts',(9.5,24.1721737853388,-35.9400363236011));
#56366=CARTESIAN_POINT('Ctrl Pts',(9.5,24.214906343328,-35.9242867765023));
#56367=CARTESIAN_POINT('Ctrl Pts',(9.5,24.2574757167881,-35.9081552208262));
#56368=CARTESIAN_POINT('Ctrl Pts',(9.5,24.3426144637084,-35.8758921094742));
#56369=CARTESIAN_POINT('Ctrl Pts',(9.5,24.4270996255911,-35.8420989822636));
#56370=CARTESIAN_POINT('Ctrl Pts',(9.5,24.511087024606,-35.8071406043763));
#56371=CARTESIAN_POINT('Ctrl Pts',(9.5,24.5950744236209,-35.7721822264891));
#56372=CARTESIAN_POINT('Ctrl Pts',(9.5,24.6785636988575,-35.7360577521598));
#56373=CARTESIAN_POINT('Ctrl Pts',(9.5,24.7617259798232,-35.6991678002813));
#56374=CARTESIAN_POINT('Ctrl Pts',(9.5,24.8448882607888,-35.6622778484028));
#56375=CARTESIAN_POINT('Ctrl Pts',(9.5,24.927723145438,-35.6246214737663));
#56376=CARTESIAN_POINT('Ctrl Pts',(9.5,25.0104224970507,-35.586647819507));
#56377=CARTESIAN_POINT('Ctrl Pts',(9.5,25.0931218486634,-35.5486741652478));
#56378=CARTESIAN_POINT('Ctrl Pts',(9.5,25.1756850333398,-35.510381750864));
#56379=CARTESIAN_POINT('Ctrl Pts',(9.5,25.2583319332265,-35.4722853085716));
#56380=CARTESIAN_POINT('Ctrl Pts',(9.5,25.3409788331131,-35.4341888662792));
#56381=CARTESIAN_POINT('Ctrl Pts',(9.5,25.4237082318775,-35.396285553944));
#56382=CARTESIAN_POINT('Ctrl Pts',(9.5,25.5067810211281,-35.359186104854));
#56383=CARTESIAN_POINT('Ctrl Pts',(9.5,25.5483174157534,-35.3406363803091));
#56384=CARTESIAN_POINT('Ctrl Pts',(9.5,25.5899403696571,-35.322289289189));
#56385=CARTESIAN_POINT('Ctrl Pts',(9.5,25.631688289108,-35.3042347373429));
#56386=CARTESIAN_POINT('Ctrl Pts',(9.5,25.673436208559,-35.2861801854968));
#56387=CARTESIAN_POINT('Ctrl Pts',(9.5,25.7153114927794,-35.2684168699898));
#56388=CARTESIAN_POINT('Ctrl Pts',(9.5,25.7573416172799,-35.2510543894317));
#56389=CARTESIAN_POINT('Ctrl Pts',(9.5,25.7993717417804,-35.2336919088736));
#56390=CARTESIAN_POINT('Ctrl Pts',(9.5,25.8415589341829,-35.2167287338712));
#56391=CARTESIAN_POINT('Ctrl Pts',(9.5,25.8839510568005,-35.2002865579818));
#56392=CARTESIAN_POINT('Ctrl Pts',(9.5,25.9263431794182,-35.1838443820923));
#56393=CARTESIAN_POINT('Ctrl Pts',(9.5,25.9689399542761,-35.167922472263));
#56394=CARTESIAN_POINT('Ctrl Pts',(9.5,26.0117995124036,-35.1526686371919));
#56395=CARTESIAN_POINT('Origin',(33.,25.1089533477396,3.15105240727392));
#56396=CARTESIAN_POINT('',(16.3099522017294,25.8138525767018,2.84895274151619));
#56397=CARTESIAN_POINT('Origin',(17.2842114798612,26.0363332260021,2.7536033866521));
#56398=CARTESIAN_POINT('Ctrl Pts',(16.3099522026769,25.8138525749482,2.84895273847024));
#56399=CARTESIAN_POINT('Ctrl Pts',(16.3240895307231,25.8437370215131,2.83614511851386));
#56400=CARTESIAN_POINT('Ctrl Pts',(16.3399187528226,25.8729217068007,2.82363739624781));
#56401=CARTESIAN_POINT('Ctrl Pts',(16.3748080290301,25.9296601647623,2.79932091426426));
#56402=CARTESIAN_POINT('Ctrl Pts',(16.3938455706131,25.9571775849078,2.78752773420181));
#56403=CARTESIAN_POINT('Ctrl Pts',(16.4143885868334,25.9837360327007,2.77614554229059));
#56404=CARTESIAN_POINT('',(33.,25.1089533477396,3.15105240727392));
#56405=CARTESIAN_POINT('Origin',(6.61325378140121E-15,20.5440037453176,
8.67361737988404E-16));
#56406=CARTESIAN_POINT('Ctrl Pts',(-16.385691310591,19.4906335657927,3.17789716423393));
#56407=CARTESIAN_POINT('Ctrl Pts',(-16.3838865721657,19.4947404992376,3.17911372502469));
#56408=CARTESIAN_POINT('Ctrl Pts',(-16.3820956441718,19.4988402929659,3.1803255757144));
#56409=CARTESIAN_POINT('Ctrl Pts',(-16.3802955079033,19.5029802288914,3.18155987450784));
#56410=CARTESIAN_POINT('Ctrl Pts',(-16.3784953716348,19.5071201648169,3.18279417330128));
#56411=CARTESIAN_POINT('Ctrl Pts',(-16.3767037318314,19.5112616232316,3.18403510677131));
#56412=CARTESIAN_POINT('Ctrl Pts',(-16.3749204594914,19.5154048469311,3.18528271336203));
#56413=CARTESIAN_POINT('Ctrl Pts',(-16.3713539148114,19.5236912943301,3.18777792654347));
#56414=CARTESIAN_POINT('Ctrl Pts',(-16.3678208473976,19.5319848056864,3.19029983360368));
#56415=CARTESIAN_POINT('Ctrl Pts',(-16.3643220920495,19.540282957292,3.19284739442709));
#56416=CARTESIAN_POINT('Ctrl Pts',(-16.3573245813534,19.5568792605033,3.19794251607391));
#56417=CARTESIAN_POINT('Ctrl Pts',(-16.3504642791346,19.573494110083,3.20314024696002));
#56418=CARTESIAN_POINT('Ctrl Pts',(-16.3437394425506,19.5901276480582,3.20843815327197));
#56419=CARTESIAN_POINT('Ctrl Pts',(-16.3333325527163,19.6158685556778,3.216636824965));
#56420=CARTESIAN_POINT('Ctrl Pts',(-16.3232499873013,19.6416542601259,3.22507559721058));
#56421=CARTESIAN_POINT('Ctrl Pts',(-16.3134863331361,19.6674851436201,3.23374592772394));
#56422=CARTESIAN_POINT('Ctrl Pts',(-16.3106316200911,19.6750376192432,3.23628097302589));
#56423=CARTESIAN_POINT('Ctrl Pts',(-16.3078041721284,19.6825939649084,3.23883583254844));
#56424=CARTESIAN_POINT('Ctrl Pts',(-16.3050038513243,19.6901542140904,3.24141036122125));
#56425=CARTESIAN_POINT('Ctrl Pts',(-16.2988148796738,19.7068630739431,3.2471003110821));
#56426=CARTESIAN_POINT('Ctrl Pts',(-16.2927584396821,19.7235909289062,3.2528861111911));
#56427=CARTESIAN_POINT('Ctrl Pts',(-16.2868332639472,19.7403379264866,3.25876585540606));
#56428=CARTESIAN_POINT('Ctrl Pts',(-16.2809080882122,19.7570849240671,3.26464559962101));
#56429=CARTESIAN_POINT('Ctrl Pts',(-16.2751116707373,19.7738586442461,3.27062203393933));
#56430=CARTESIAN_POINT('Ctrl Pts',(-16.2694535638472,19.7906272310772,3.27668164700856));
#56431=CARTESIAN_POINT('Ctrl Pts',(-16.2581373500668,19.8241644047395,3.28880087314701));
#56432=CARTESIAN_POINT('Ctrl Pts',(-16.2473713706875,19.8576872094414,3.30125446802705));
#56433=CARTESIAN_POINT('Ctrl Pts',(-16.2371394993118,19.891199479047,3.31402457021168));
#56434=CARTESIAN_POINT('Ctrl Pts',(0.214931209580442,20.543989890264,-16.4986005940977));
#56435=CARTESIAN_POINT('Ctrl Pts',(0.248500277094282,20.5181273342308,-16.4981634012918));
#56436=CARTESIAN_POINT('Ctrl Pts',(0.281612583091536,20.493053464206,-16.4979577166671));
#56437=CARTESIAN_POINT('Ctrl Pts',(0.5671966423497,20.2806701732619,-16.4978943536735));
#56438=CARTESIAN_POINT('Ctrl Pts',(0.831304673132399,20.1086229690508,-16.5088512065424));
#56439=CARTESIAN_POINT('Ctrl Pts',(1.41340912589609,19.7774389533295,-16.5366009814182));
#56440=CARTESIAN_POINT('Ctrl Pts',(1.73506034135079,19.6224000490625,-16.5541218518306));
#56441=CARTESIAN_POINT('Ctrl Pts',(2.06506260776274,19.4906334205533,-16.5627719180497));
#56442=CARTESIAN_POINT('Origin',(-39.,35.,5.80048162279745E-15));
#56443=CARTESIAN_POINT('Origin',(33.,35.,5.81688018065629E-15));
#56444=CARTESIAN_POINT('Origin',(33.,26.4545372843263,5.29429254368814));
#56445=CARTESIAN_POINT('Origin',(-37.5,50.9978970953601,-20.6163621683838));
#56446=CARTESIAN_POINT('',(-37.5,51.4199384841736,-20.884468613902));
#56447=CARTESIAN_POINT('Origin',(-37.5,51.8419798729871,-21.1525750594202));
#56448=CARTESIAN_POINT('',(-37.5,51.2660035408783,-20.1943207795704));
#56449=CARTESIAN_POINT('Origin',(-37.5,50.9978970953601,-20.6163621683838));
#56450=CARTESIAN_POINT('Origin',(-37.5,51.5341099863965,-19.7722793907569));
#56451=CARTESIAN_POINT('Origin',(-50.,50.9978970953601,-20.6163621683838));
#56452=CARTESIAN_POINT('',(-50.,51.4199384841736,-20.884468613902));
#56453=CARTESIAN_POINT('Origin',(-45.2928932188135,50.9978970953601,-20.6163621683838));
#56454=CARTESIAN_POINT('',(-50.,51.2660035408783,-20.1943207795704));
#56455=CARTESIAN_POINT('Origin',(-37.5,51.95615137521,-20.0403858362751));
#56456=CARTESIAN_POINT('',(-37.5,51.6880449296918,-20.4624272250886));
#56457=CARTESIAN_POINT('Origin',(-45.2928932188135,50.9978970953601,-20.6163621683838));
#56458=CARTESIAN_POINT('Origin',(-45.2221315177632,41.5560116976042,-24.0960437966388));
#56459=CARTESIAN_POINT('',(-50.,44.1759456341881,-25.7603857162899));
#56460=CARTESIAN_POINT('',(-50.,41.5560116976042,-24.0960437966388));
#56461=CARTESIAN_POINT('Origin',(-50.,3.18714947135723,5.01707068865061));
#56462=CARTESIAN_POINT('Origin',(-49.5,45.6658960598572,-29.0097639675421));
#56463=CARTESIAN_POINT('',(-50.,45.635768184996,-29.057189944653));
#56464=CARTESIAN_POINT('',(-50.,43.4909166208504,-32.4335210551606));
#56465=CARTESIAN_POINT('',(-49.5,45.7897031282913,-29.7473377789847));
#56466=CARTESIAN_POINT('Origin',(-49.5,45.3676617394779,-29.4792313334666));
#56467=CARTESIAN_POINT('',(-49.5,46.0578095738095,-29.3252963901712));
#56468=CARTESIAN_POINT('Origin',(-50.,45.3676617394778,-29.4792313334664));
#56469=CARTESIAN_POINT('',(-50.,45.635768184996,-29.057189944653));
#56470=CARTESIAN_POINT('',(-45.2221315177632,45.7897031282913,-29.7473377789847));
#56471=CARTESIAN_POINT('Origin',(9.5,24.,-29.5));
#56472=CARTESIAN_POINT('',(9.5,24.0000000040242,-23.000000001077));
#56473=CARTESIAN_POINT('Ctrl Pts',(9.5,26.0117995124034,-23.847331362808));
#56474=CARTESIAN_POINT('Ctrl Pts',(9.5,25.9689096319939,-23.8320667357437));
#56475=CARTESIAN_POINT('Ctrl Pts',(9.5,25.9262879467264,-23.8161349281401));
#56476=CARTESIAN_POINT('Ctrl Pts',(9.5,25.883874978838,-23.7996839392245));
#56477=CARTESIAN_POINT('Ctrl Pts',(9.5,25.8414587998583,-23.7832317048023));
#56478=CARTESIAN_POINT('Ctrl Pts',(9.5,25.7992516394778,-23.7662594986502));
#56479=CARTESIAN_POINT('Ctrl Pts',(9.5,25.7572045884039,-23.7488890070158));
#56480=CARTESIAN_POINT('Ctrl Pts',(9.5,25.7151550358237,-23.7315174819583));
#56481=CARTESIAN_POINT('Ctrl Pts',(9.5,25.6732659998802,-23.7137472811973));
#56482=CARTESIAN_POINT('Ctrl Pts',(9.5,25.6314953697901,-23.6956818329298));
#56483=CARTESIAN_POINT('Ctrl Pts',(9.5,25.5897299794738,-23.6776186508207));
#56484=CARTESIAN_POINT('Ctrl Pts',(9.5,25.5480846709542,-23.6592606571989));
#56485=CARTESIAN_POINT('Ctrl Pts',(9.5,25.5065351970736,-23.640704126495));
#56486=CARTESIAN_POINT('Ctrl Pts',(9.50000000000001,25.4234324751939,-23.6035893795174));
#56487=CARTESIAN_POINT('Ctrl Pts',(9.5,25.340692297494,-23.5656796578226));
#56488=CARTESIAN_POINT('Ctrl Pts',(9.5,25.2580389063772,-23.5275796334702));
#56489=CARTESIAN_POINT('Ctrl Pts',(9.5,25.1753855152603,-23.4894796091178));
#56490=CARTESIAN_POINT('Ctrl Pts',(9.5,25.0928202181361,-23.4511864152134));
#56491=CARTESIAN_POINT('Ctrl Pts',(9.5,25.0101108671149,-23.4132090978422));
#56492=CARTESIAN_POINT('Ctrl Pts',(9.5,24.9274015160936,-23.3752317804711));
#56493=CARTESIAN_POINT('Ctrl Pts',(9.5,24.8445483055857,-23.337568859186));
#56494=CARTESIAN_POINT('Ctrl Pts',(9.5,24.7613805795409,-23.3006789941698));
#56495=CARTESIAN_POINT('Ctrl Pts',(9.5,24.6781802428869,-23.2637746643964));
#56496=CARTESIAN_POINT('Ctrl Pts',(9.5,24.5946613246052,-23.2276411758559));
#56497=CARTESIAN_POINT('Ctrl Pts',(9.5,24.5106576117287,-23.1926806714327));
#56498=CARTESIAN_POINT('Ctrl Pts',(9.5,24.4267197498417,-23.1577475727482));
#56499=CARTESIAN_POINT('Ctrl Pts',(9.5,24.3422981983971,-23.1239848109111));
#56500=CARTESIAN_POINT('Ctrl Pts',(9.5,24.2572425017914,-23.0917564080366));
#56501=CARTESIAN_POINT('Ctrl Pts',(9.5,24.2146979715,-23.0756358856371));
#56502=CARTESIAN_POINT('Ctrl Pts',(9.5,24.1719949918743,-23.0598987437645));
#56503=CARTESIAN_POINT('Ctrl Pts',(9.5,24.1291157581348,-23.0445880627847));
#56504=CARTESIAN_POINT('Ctrl Pts',(9.5,24.1076774470549,-23.0369331885468));
#56505=CARTESIAN_POINT('Ctrl Pts',(9.5,24.0861944286833,-23.0293846978839));
#56506=CARTESIAN_POINT('Ctrl Pts',(9.5,24.0646742539635,-23.0219511396643));
#56507=CARTESIAN_POINT('Ctrl Pts',(9.5,24.0539125104744,-23.0182337884897));
#56508=CARTESIAN_POINT('Ctrl Pts',(9.5,24.0431409392655,-23.0145449829623));
#56509=CARTESIAN_POINT('Ctrl Pts',(9.5,24.032359320533,-23.0108853638909));
#56510=CARTESIAN_POINT('Ctrl Pts',(9.5,24.0269687018538,-23.0090556190804));
#56511=CARTESIAN_POINT('Ctrl Pts',(9.49999999999461,24.0215753227308,-23.0072339008906));
#56512=CARTESIAN_POINT('Ctrl Pts',(9.49999999999462,24.0161787253986,-23.0054201450326));
#56513=CARTESIAN_POINT('Ctrl Pts',(9.49999999999464,24.0107824390184,-23.0036064936833));
#56514=CARTESIAN_POINT('Ctrl Pts',(9.5,24.0053865342605,-23.0018020066657));
#56515=CARTESIAN_POINT('Ctrl Pts',(9.5,24.0000000128774,-23.000000004308));
#56516=CARTESIAN_POINT('Ctrl Pts',(9.5,24.,-23.));
#56517=CARTESIAN_POINT('Ctrl Pts',(9.5,23.9945849935496,-23.0018115317267));
#56518=CARTESIAN_POINT('Ctrl Pts',(9.49999999999458,23.9891956914846,-23.0036138370378));
#56519=CARTESIAN_POINT('Ctrl Pts',(9.49999999999452,23.9838049192649,-23.005425649693));
#56520=CARTESIAN_POINT('Ctrl Pts',(9.49999999999445,23.9784141470452,-23.0072374623481));
#56521=CARTESIAN_POINT('Ctrl Pts',(9.5,23.9730112146172,-23.0090624126808));
#56522=CARTESIAN_POINT('Ctrl Pts',(9.5,23.9676115942036,-23.0108952044431));
#56523=CARTESIAN_POINT('Ctrl Pts',(9.5,23.9568123533764,-23.0145607879675));
#56524=CARTESIAN_POINT('Ctrl Pts',(9.5,23.9460253688664,-23.0182550965837));
#56525=CARTESIAN_POINT('Ctrl Pts',(9.5,23.9352502697771,-23.0219772088574));
#56526=CARTESIAN_POINT('Ctrl Pts',(9.5,23.9137000715983,-23.0294214334047));
#56527=CARTESIAN_POINT('Ctrl Pts',(9.5,23.8921975466363,-23.0369772593698));
#56528=CARTESIAN_POINT('Ctrl Pts',(9.5,23.8707404359779,-23.0446393983796));
#56529=CARTESIAN_POINT('Ctrl Pts',(9.5,23.8278262146613,-23.059963676399));
#56530=CARTESIAN_POINT('Ctrl Pts',(9.5,23.7850936566721,-23.0757132234977));
#56531=CARTESIAN_POINT('Ctrl Pts',(9.5,23.742524283212,-23.0918447791738));
#56532=CARTESIAN_POINT('Ctrl Pts',(9.5,23.6573855362917,-23.1241078905259));
#56533=CARTESIAN_POINT('Ctrl Pts',(9.5,23.572900374409,-23.1579010177367));
#56534=CARTESIAN_POINT('Ctrl Pts',(9.5,23.488912975394,-23.1928593956236));
#56535=CARTESIAN_POINT('Ctrl Pts',(9.5,23.404925576379,-23.2278177735106));
#56536=CARTESIAN_POINT('Ctrl Pts',(9.5,23.3214363011426,-23.2639422478401));
#56537=CARTESIAN_POINT('Ctrl Pts',(9.5,23.2382740201769,-23.3008321997186));
#56538=CARTESIAN_POINT('Ctrl Pts',(9.5,23.1551117392113,-23.3377221515971));
#56539=CARTESIAN_POINT('Ctrl Pts',(9.5,23.0722768545621,-23.3753785262336));
#56540=CARTESIAN_POINT('Ctrl Pts',(9.5,22.9895775029495,-23.4133521804931));
#56541=CARTESIAN_POINT('Ctrl Pts',(9.5,22.9068781513369,-23.4513258347525));
#56542=CARTESIAN_POINT('Ctrl Pts',(9.5,22.8243149666603,-23.4896182491358));
#56543=CARTESIAN_POINT('Ctrl Pts',(9.5,22.7416680667737,-23.5277146914284));
#56544=CARTESIAN_POINT('Ctrl Pts',(9.5,22.6590211668871,-23.5658111337209));
#56545=CARTESIAN_POINT('Ctrl Pts',(9.5,22.5762917681227,-23.603714446056));
#56546=CARTESIAN_POINT('Ctrl Pts',(9.5,22.493218978872,-23.6408138951459));
#56547=CARTESIAN_POINT('Ctrl Pts',(9.5,22.4516825842467,-23.6593636196908));
#56548=CARTESIAN_POINT('Ctrl Pts',(9.5,22.4100596303431,-23.677710710811));
#56549=CARTESIAN_POINT('Ctrl Pts',(9.5,22.3683117108922,-23.695765262657));
#56550=CARTESIAN_POINT('Ctrl Pts',(9.5,22.3265637914412,-23.713819814503));
#56551=CARTESIAN_POINT('Ctrl Pts',(9.5,22.2846885072208,-23.7315831300102));
#56552=CARTESIAN_POINT('Ctrl Pts',(9.5,22.2426583827203,-23.7489456105683));
#56553=CARTESIAN_POINT('Ctrl Pts',(9.5,22.2006282582199,-23.7663080911264));
#56554=CARTESIAN_POINT('Ctrl Pts',(9.5,22.1584410658174,-23.7832712661287));
#56555=CARTESIAN_POINT('Ctrl Pts',(9.5,22.1160489431998,-23.7997134420182));
#56556=CARTESIAN_POINT('Ctrl Pts',(9.50000000000001,22.0736568205821,-23.8161556179077));
#56557=CARTESIAN_POINT('Ctrl Pts',(9.5,22.031060045724,-23.8320775277365));
#56558=CARTESIAN_POINT('Ctrl Pts',(9.5,21.9882004875966,-23.847331362808));
#56559=CARTESIAN_POINT('Ctrl Pts',(9.5,21.9882004875966,-35.152668637192));
#56560=CARTESIAN_POINT('Ctrl Pts',(9.5,22.0310903680061,-35.1679332642564));
#56561=CARTESIAN_POINT('Ctrl Pts',(9.5,22.0737120532736,-35.1838650718599));
#56562=CARTESIAN_POINT('Ctrl Pts',(9.5,22.116125021162,-35.2003160607755));
#56563=CARTESIAN_POINT('Ctrl Pts',(9.5,22.1585412001417,-35.2167682951977));
#56564=CARTESIAN_POINT('Ctrl Pts',(9.5,22.2007483605221,-35.23374050135));
#56565=CARTESIAN_POINT('Ctrl Pts',(9.5,22.242795411596,-35.2511109929843));
#56566=CARTESIAN_POINT('Ctrl Pts',(9.5,22.2848449641762,-35.2684825180418));
#56567=CARTESIAN_POINT('Ctrl Pts',(9.5,22.3267340001198,-35.2862527188033));
#56568=CARTESIAN_POINT('Ctrl Pts',(9.5,22.3685046302098,-35.3043181670704));
#56569=CARTESIAN_POINT('Ctrl Pts',(9.5,22.410270020526,-35.3223813491792));
#56570=CARTESIAN_POINT('Ctrl Pts',(9.5,22.4519153290457,-35.3407393428013));
#56571=CARTESIAN_POINT('Ctrl Pts',(9.5,22.4934648029264,-35.3592958735051));
#56572=CARTESIAN_POINT('Ctrl Pts',(9.5,22.5765675248061,-35.3964106204826));
#56573=CARTESIAN_POINT('Ctrl Pts',(9.5,22.659307702506,-35.4343203421775));
#56574=CARTESIAN_POINT('Ctrl Pts',(9.5,22.7419610936227,-35.4724203665301));
#56575=CARTESIAN_POINT('Ctrl Pts',(9.5,22.8246144847395,-35.5105203908827));
#56576=CARTESIAN_POINT('Ctrl Pts',(9.5,22.9071797818639,-35.5488135847866));
#56577=CARTESIAN_POINT('Ctrl Pts',(9.5,22.9898891328852,-35.5867909021576));
#56578=CARTESIAN_POINT('Ctrl Pts',(9.5,23.0725984839066,-35.6247682195286));
#56579=CARTESIAN_POINT('Ctrl Pts',(9.5,23.1554516944143,-35.662431140814));
#56580=CARTESIAN_POINT('Ctrl Pts',(9.5,23.2386194204592,-35.6993210058301));
#56581=CARTESIAN_POINT('Ctrl Pts',(9.5,23.3217871465041,-35.7362108708462));
#56582=CARTESIAN_POINT('Ctrl Pts',(9.50000000000004,23.4052731920914,-35.7723305361407));
#56583=CARTESIAN_POINT('Ctrl Pts',(9.49999999999995,23.4892435227574,-35.8072784366652));
#56584=CARTESIAN_POINT('Ctrl Pts',(9.49999999999985,23.5732138534233,-35.8422263371897));
#56585=CARTESIAN_POINT('Ctrl Pts',(9.5,23.6576684376259,-35.8760025471646));
#56586=CARTESIAN_POINT('Ctrl Pts',(9.5,23.7427574982086,-35.9082435919634));
#56587=CARTESIAN_POINT('Ctrl Pts',(9.5,23.7853020285,-35.9243641143629));
#56588=CARTESIAN_POINT('Ctrl Pts',(9.5,23.8280050081257,-35.9401012562356));
#56589=CARTESIAN_POINT('Ctrl Pts',(9.5,23.8708842418652,-35.9554119372154));
#56590=CARTESIAN_POINT('Ctrl Pts',(9.5,23.8923225529451,-35.9630668114532));
#56591=CARTESIAN_POINT('Ctrl Pts',(9.5,23.9138055713167,-35.9706153021161));
#56592=CARTESIAN_POINT('Ctrl Pts',(9.5,23.9353257460365,-35.9780488603358));
#56593=CARTESIAN_POINT('Ctrl Pts',(9.5,23.9460874895256,-35.9817662115104));
#56594=CARTESIAN_POINT('Ctrl Pts',(9.5,23.9568590607345,-35.9854550170376));
#56595=CARTESIAN_POINT('Ctrl Pts',(9.5,23.9676406794671,-35.989114636109));
#56596=CARTESIAN_POINT('Ctrl Pts',(9.5,23.9730312981462,-35.9909443809195));
#56597=CARTESIAN_POINT('Ctrl Pts',(9.49999999999524,23.9784247177933,-35.9927659777918));
#56598=CARTESIAN_POINT('Ctrl Pts',(9.49999999999624,23.983819858151,-35.9945789780646));
#56599=CARTESIAN_POINT('Ctrl Pts',(9.49999999999724,23.9892146876407,-35.9963918738723));
#56600=CARTESIAN_POINT('Ctrl Pts',(9.5,23.9946073268916,-35.9981959396455));
#56601=CARTESIAN_POINT('Ctrl Pts',(9.5,23.9999999209526,-35.9999999735555));
#56602=CARTESIAN_POINT('Ctrl Pts',(9.5,21.9882004875966,-23.847331362808));
#56603=CARTESIAN_POINT('Ctrl Pts',(9.5,21.8205505282296,-23.376275643042));
#56604=CARTESIAN_POINT('Ctrl Pts',(9.,21.8205505282296,-23.376275643042));
#56605=CARTESIAN_POINT('Ctrl Pts',(9.5,22.0308734754341,-23.8321439286178));
#56606=CARTESIAN_POINT('Ctrl Pts',(9.49999999999997,21.8636141076127,-23.3799945381981));
#56607=CARTESIAN_POINT('Ctrl Pts',(9.01826917526517,21.8582716513203,-23.3628505969422));
#56608=CARTESIAN_POINT('Ctrl Pts',(9.5,22.0733381907741,-23.8162753226795));
#56609=CARTESIAN_POINT('Ctrl Pts',(9.50000000000008,21.9080522210625,-23.3816975070418));
#56610=CARTESIAN_POINT('Ctrl Pts',(9.03631589192582,21.8967431756777,-23.3495513478538));
#56611=CARTESIAN_POINT('Ctrl Pts',(9.5,22.1579409882236,-23.7834690781199));
#56612=CARTESIAN_POINT('Ctrl Pts',(9.49999999999993,21.9974551619948,-23.3816228520534));
#56613=CARTESIAN_POINT('Ctrl Pts',(9.07183836849214,21.9751185068201,-23.32330486165));
#56614=CARTESIAN_POINT('Ctrl Pts',(9.5,22.2000788409464,-23.7665308354962));
#56615=CARTESIAN_POINT('Ctrl Pts',(9.49999999999999,22.0425136846468,-23.3799532806648));
#56616=CARTESIAN_POINT('Ctrl Pts',(9.08931415962565,22.015022451126,-23.3103576134241));
#56617=CARTESIAN_POINT('Ctrl Pts',(9.5,22.2841024246593,-23.7318294112912));
#56618=CARTESIAN_POINT('Ctrl Pts',(9.5,22.1328834324073,-23.3739145190718));
#56619=CARTESIAN_POINT('Ctrl Pts',(9.12357368892884,22.0961862855176,-23.284913348421));
#56620=CARTESIAN_POINT('Ctrl Pts',(9.5,22.3259971280704,-23.7140617868281));
#56621=CARTESIAN_POINT('Ctrl Pts',(9.49999999999999,22.1783023884446,-23.3696111361603));
#56622=CARTESIAN_POINT('Ctrl Pts',(9.14036084384036,22.1374556044338,-23.2724137847841));
#56623=CARTESIAN_POINT('Ctrl Pts',(9.5,22.4095179570165,-23.677948027438));
#56624=CARTESIAN_POINT('Ctrl Pts',(9.5,22.2691443860353,-23.3589300101936));
#56625=CARTESIAN_POINT('Ctrl Pts',(9.17309573545695,22.2211811143838,-23.2479839196916));
#56626=CARTESIAN_POINT('Ctrl Pts',(9.5,22.4511531677501,-23.6595980500185));
#56627=CARTESIAN_POINT('Ctrl Pts',(9.50000000000004,22.3146735747321,-23.3525913977176));
#56628=CARTESIAN_POINT('Ctrl Pts',(9.18904735031177,22.2636457940565,-23.2360507661085));
#56629=CARTESIAN_POINT('Ctrl Pts',(9.5,22.5757984966601,-23.603938756548));
#56630=CARTESIAN_POINT('Ctrl Pts',(9.49999999999992,22.4497171680525,-23.3314395599938));
#56631=CARTESIAN_POINT('Ctrl Pts',(9.23550610480825,22.3927209803161,-23.2012225079895));
#56632=CARTESIAN_POINT('Ctrl Pts',(9.5,22.6585512271961,-23.5660269047261));
#56633=CARTESIAN_POINT('Ctrl Pts',(9.50000000000001,22.5411793542677,-23.3141381342362));
#56634=CARTESIAN_POINT('Ctrl Pts',(9.26461357237069,22.4810179658032,-23.1793012669497));
#56635=CARTESIAN_POINT('Ctrl Pts',(9.5,22.8238907233082,-23.4898146827162));
#56636=CARTESIAN_POINT('Ctrl Pts',(9.5,22.723314180599,-23.2762265742333));
#56637=CARTESIAN_POINT('Ctrl Pts',(9.31837705316271,22.6613097872554,-23.1386756559123));
#56638=CARTESIAN_POINT('Ctrl Pts',(9.5,22.9064762965803,-23.4515115213861));
#56639=CARTESIAN_POINT('Ctrl Pts',(9.50000000000008,22.8146676949729,-23.2555923992572));
#56640=CARTESIAN_POINT('Ctrl Pts',(9.34303153817126,22.7533032142948,-23.1199727301944));
#56641=CARTESIAN_POINT('Ctrl Pts',(9.5,23.0719192863638,-23.375541574565));
#56642=CARTESIAN_POINT('Ctrl Pts',(9.49999999999992,22.9966600101024,-23.2132413108115));
#56643=CARTESIAN_POINT('Ctrl Pts',(9.38729861344406,22.9400379161302,-23.0863051820222));
#56644=CARTESIAN_POINT('Ctrl Pts',(9.5,23.1547760839593,-23.3378733402142));
#56645=CARTESIAN_POINT('Ctrl Pts',(9.5,23.0879236376168,-23.1914132685269));
#56646=CARTESIAN_POINT('Ctrl Pts',(9.40691008519306,23.0347766742058,-23.0713416571934));
#56647=CARTESIAN_POINT('Ctrl Pts',(9.5,23.3211443668266,-23.2640694732462));
#56648=CARTESIAN_POINT('Ctrl Pts',(9.5,23.269865874317,-23.1483804270448));
#56649=CARTESIAN_POINT('Ctrl Pts',(9.44067629739217,23.2259584128153,-23.0455314877889));
#56650=CARTESIAN_POINT('Ctrl Pts',(9.5,23.4046554565311,-23.2279329146211));
#56651=CARTESIAN_POINT('Ctrl Pts',(9.49999999999991,23.3611281377987,-23.1270313510183));
#56652=CARTESIAN_POINT('Ctrl Pts',(9.45483075696682,23.3223982477998,-23.0346852271054));
#56653=CARTESIAN_POINT('Ctrl Pts',(9.5,23.5726741052635,-23.1579924983959));
#56654=CARTESIAN_POINT('Ctrl Pts',(9.50000000000008,23.543200483619,-23.0863234112952));
#56655=CARTESIAN_POINT('Ctrl Pts',(9.47746628181507,23.5159324647517,-23.0173217057587));
#56656=CARTESIAN_POINT('Ctrl Pts',(9.5,23.6571813110635,-23.1241878139021));
#56657=CARTESIAN_POINT('Ctrl Pts',(9.50000000000015,23.6345625920942,-23.0668208917478));
#56658=CARTESIAN_POINT('Ctrl Pts',(9.48594808355026,23.613023793506,-23.0108039549616));
#56659=CARTESIAN_POINT('Ctrl Pts',(9.5,23.7849228667865,-23.0757766828128));
#56660=CARTESIAN_POINT('Ctrl Pts',(9.49999999999992,23.7715467510155,-23.0398746218244));
#56661=CARTESIAN_POINT('Ctrl Pts',(9.49439707925567,23.7584321344567,-23.0043092021594));
#56662=CARTESIAN_POINT('Ctrl Pts',(9.5,23.8276666334525,-23.0600217973851));
#56663=CARTESIAN_POINT('Ctrl Pts',(9.49999999999982,23.8172008244345,-23.0312711092426));
#56664=CARTESIAN_POINT('Ctrl Pts',(9.49650254697548,23.8068644801768,-23.0026900259242));
#56665=CARTESIAN_POINT('Ctrl Pts',(9.5,23.8920548994674,-23.0370276541268));
#56666=CARTESIAN_POINT('Ctrl Pts',(9.50000000000011,23.8857012094299,-23.019029781774));
#56667=CARTESIAN_POINT('Ctrl Pts',(9.49860334653214,23.8793793478707,-23.001074302905));
#56668=CARTESIAN_POINT('Ctrl Pts',(9.5,23.9135630817008,-23.0294692825348));
#56669=CARTESIAN_POINT('Ctrl Pts',(9.50000000000052,23.9085380131238,-23.0150595806498));
#56670=CARTESIAN_POINT('Ctrl Pts',(9.49912745052014,23.9035287887977,-23.0006711718907));
#56671=CARTESIAN_POINT('Ctrl Pts',(9.5,23.9458969027414,-23.0182992158728));
#56672=CARTESIAN_POINT('Ctrl Pts',(9.49999999999972,23.9428018894257,-23.0092811501081));
#56673=CARTESIAN_POINT('Ctrl Pts',(9.49965105814884,23.9397108051149,-23.0002684139077));
#56674=CARTESIAN_POINT('Ctrl Pts',(9.5,23.9566867669937,-23.0146037737788));
#56675=CARTESIAN_POINT('Ctrl Pts',(9.5000000000002,23.9542246326999,-23.0073844572567));
#56676=CARTESIAN_POINT('Ctrl Pts',(9.49978183973438,23.9517644603695,-23.0001678143699));
#56677=CARTESIAN_POINT('Ctrl Pts',(9.5,23.9782909082579,-23.0072700390361));
#56678=CARTESIAN_POINT('Ctrl Pts',(9.49999999999955,23.9770731248063,-23.003651938446));
#56679=CARTESIAN_POINT('Ctrl Pts',(9.49995621937517,23.9758563354694,-23.0000336775452));
#56680=CARTESIAN_POINT('Ctrl Pts',(9.5,23.9890917418835,-23.0036492395423));
#56681=CARTESIAN_POINT('Ctrl Pts',(9.5,23.9884834909635,-23.0018249740171));
#56682=CARTESIAN_POINT('Ctrl Pts',(9.5,23.9878765918614,-22.999999999779));
#56683=CARTESIAN_POINT('Ctrl Pts',(9.5,24.,-23.));
#56684=CARTESIAN_POINT('Ctrl Pts',(9.5,24.,-23.));
#56685=CARTESIAN_POINT('Ctrl Pts',(9.5,24.,-23.));
#56686=CARTESIAN_POINT('Ctrl Pts',(9.00000000000003,21.8205505282297,-23.376275643042));
#56687=CARTESIAN_POINT('Ctrl Pts',(9.00499129300375,21.8308562576916,-23.372607807045));
#56688=CARTESIAN_POINT('Ctrl Pts',(9.00995373459346,21.841192773063,-23.3689583730607));
#56689=CARTESIAN_POINT('Ctrl Pts',(9.0148783576887,21.8515416277292,-23.3653340482104));
#56690=CARTESIAN_POINT('Ctrl Pts',(9.01980298078395,21.8618904823954,-23.3617097233601));
#56691=CARTESIAN_POINT('Ctrl Pts',(9.02469199992643,21.8722562234444,-23.3581088799382));
#56692=CARTESIAN_POINT('Ctrl Pts',(9.02954542600218,21.8826388751752,-23.3545316367355));
#56693=CARTESIAN_POINT('Ctrl Pts',(9.03782625969413,21.9003535804005,-23.348428204732));
#56694=CARTESIAN_POINT('Ctrl Pts',(9.04600352023976,21.9181175364614,-23.3423934607784));
#56695=CARTESIAN_POINT('Ctrl Pts',(9.05407713254697,21.9359308413409,-23.3364281049891));
#56696=CARTESIAN_POINT('Ctrl Pts',(9.05546746601018,21.938998419139,-23.3354008282933));
#56697=CARTESIAN_POINT('Ctrl Pts',(9.05685472633738,21.9420674633145,-23.3343756088419));
#56698=CARTESIAN_POINT('Ctrl Pts',(9.0582389147631,21.9451379750064,-23.3333524492007));
#56699=CARTESIAN_POINT('Ctrl Pts',(9.07474419566322,21.9817512402532,-23.3211521324161));
#56700=CARTESIAN_POINT('Ctrl Pts',(9.09081329757236,22.0185740363922,-23.3092442159581));
#56701=CARTESIAN_POINT('Ctrl Pts',(9.10644398031617,22.0556043729826,-23.2976354922079));
#56702=CARTESIAN_POINT('Ctrl Pts',(9.10865899416138,22.060851917801,-23.2959904275454));
#56703=CARTESIAN_POINT('Ctrl Pts',(9.11086526354459,22.0661038086614,-23.2943513253027));
#56704=CARTESIAN_POINT('Ctrl Pts',(9.11306274833677,22.0713599394839,-23.2927182300073));
#56705=CARTESIAN_POINT('Ctrl Pts',(9.12802360671032,22.1071445916041,-23.2815998334148));
#56706=CARTESIAN_POINT('Ctrl Pts',(9.14258366284695,22.1431405314812,-23.2707550505375));
#56707=CARTESIAN_POINT('Ctrl Pts',(9.15672841971646,22.1793183764486,-23.2601988916461));
#56708=CARTESIAN_POINT('Ctrl Pts',(9.173222617404,22.2215053530299,-23.247889357224));
#56709=CARTESIAN_POINT('Ctrl Pts',(9.18915639775547,22.2639484742488,-23.2359691362469));
#56710=CARTESIAN_POINT('Ctrl Pts',(9.20453378247886,22.3066708891664,-23.2244414206892));
#56711=CARTESIAN_POINT('Ctrl Pts',(9.20718005181625,22.3140229206496,-23.2224576347101));
#56712=CARTESIAN_POINT('Ctrl Pts',(9.20980980902293,22.3213832951449,-23.2204854962787));
#56713=CARTESIAN_POINT('Ctrl Pts',(9.21242308500115,22.3287521298052,-23.2185250123999));
#56714=CARTESIAN_POINT('Ctrl Pts',(9.23546015599538,22.393711349049,-23.2012425643632));
#56715=CARTESIAN_POINT('Ctrl Pts',(9.25720832413433,22.4592986133338,-23.1848714345782));
#56716=CARTESIAN_POINT('Ctrl Pts',(9.27764739317659,22.5255230192183,-23.1694460829554));
#56717=CARTESIAN_POINT('Ctrl Pts',(9.2823323904216,22.5407028279698,-23.165910318694));
#56718=CARTESIAN_POINT('Ctrl Pts',(9.28694852686031,22.5559163090766,-23.1624242938876));
#56719=CARTESIAN_POINT('Ctrl Pts',(9.29149540308999,22.5711639036601,-23.1589885202901));
#56720=CARTESIAN_POINT('Ctrl Pts',(9.29365149253128,22.5783941813333,-23.1573593061216));
#56721=CARTESIAN_POINT('Ctrl Pts',(9.29579199751476,22.5856321222163,-23.15574140122));
#56722=CARTESIAN_POINT('Ctrl Pts',(9.29791690448533,22.5928777430096,-23.1541348371914));
#56723=CARTESIAN_POINT('Ctrl Pts',(9.31795789315131,22.6612145719663,-23.1389825825589));
#56724=CARTESIAN_POINT('Ctrl Pts',(9.33661353356725,22.7302314074187,-23.1248370273146));
#56725=CARTESIAN_POINT('Ctrl Pts',(9.35385081456094,22.7999466691982,-23.1117399026863));
#56726=CARTESIAN_POINT('Ctrl Pts',(9.35769303749758,22.8154863345283,-23.1088205285304));
#56727=CARTESIAN_POINT('Ctrl Pts',(9.36146465901819,22.8310608309738,-23.1059533376774));
#56728=CARTESIAN_POINT('Ctrl Pts',(9.36516507939254,22.8466705668119,-23.1031389595914));
#56729=CARTESIAN_POINT('Ctrl Pts',(9.36652977322612,22.8524273479576,-23.1021010330775));
#56730=CARTESIAN_POINT('Ctrl Pts',(9.36788477789199,22.8581889130261,-23.1010702944162));
#56731=CARTESIAN_POINT('Ctrl Pts',(9.36923008056748,22.8639552738464,-23.1000467608728));
#56732=CARTESIAN_POINT('Ctrl Pts',(9.38542504339938,22.9333716221974,-23.0877253048954));
#56733=CARTESIAN_POINT('Ctrl Pts',(9.40021701095275,23.0034807157845,-23.0764457182034));
#56734=CARTESIAN_POINT('Ctrl Pts',(9.41356185654141,23.0743088141014,-23.0662539355901));
#56735=CARTESIAN_POINT('Ctrl Pts',(9.41707313527556,23.0929450129055,-23.0635722867606));
#56736=CARTESIAN_POINT('Ctrl Pts',(9.42048401358343,23.1116310616337,-23.0609661105274));
#56737=CARTESIAN_POINT('Ctrl Pts',(9.42379321375124,23.1303675580568,-23.0584366052813));
#56738=CARTESIAN_POINT('Ctrl Pts',(9.42449386001645,23.1343345759392,-23.0579010413039));
#56739=CARTESIAN_POINT('Ctrl Pts',(9.4251899470015,23.1383038499722,-23.0573689155869));
#56740=CARTESIAN_POINT('Ctrl Pts',(9.42588146840096,23.1422753857726,-23.0568402345328));
#56741=CARTESIAN_POINT('Ctrl Pts',(9.42997413403966,23.1657803244711,-23.0537113150433));
#56742=CARTESIAN_POINT('Ctrl Pts',(9.43390864964305,23.1893767278427,-23.0507017475785));
#56743=CARTESIAN_POINT('Ctrl Pts',(9.43767033422762,23.2129792231054,-23.0478230658526));
#56744=CARTESIAN_POINT('Ctrl Pts',(9.4414320188122,23.2365817183681,-23.0449443841267));
#56745=CARTESIAN_POINT('Ctrl Pts',(9.44502387076404,23.2602064841671,-23.0421942983327));
#56746=CARTESIAN_POINT('Ctrl Pts',(9.44844616386932,23.2838534804762,-23.0395729439543));
#56747=CARTESIAN_POINT('Ctrl Pts',(9.45496209937024,23.3288765974333,-23.0345819699118));
#56748=CARTESIAN_POINT('Ctrl Pts',(9.46086375084296,23.3739801923503,-23.0300574787948));
#56749=CARTESIAN_POINT('Ctrl Pts',(9.46614854505998,23.4191653817027,-23.0260035275154));
#56750=CARTESIAN_POINT('Ctrl Pts',(9.4664150994741,23.4214444319703,-23.0257990543489));
#56751=CARTESIAN_POINT('Ctrl Pts',(9.4666800837967,23.4237236883581,-23.0255957789381));
#56752=CARTESIAN_POINT('Ctrl Pts',(9.46694349854553,23.4260031516636,-23.0253937010497));
#56753=CARTESIAN_POINT('Ctrl Pts',(9.4756046317945,23.5009523924046,-23.0187493368808));
#56754=CARTESIAN_POINT('Ctrl Pts',(9.48257224642999,23.5761241008637,-23.013397473722));
#56755=CARTESIAN_POINT('Ctrl Pts',(9.48784091893683,23.6515208762116,-23.0093485597976));
#56756=CARTESIAN_POINT('Ctrl Pts',(9.48920116350281,23.6709865108331,-23.0083032275708));
#56757=CARTESIAN_POINT('Ctrl Pts',(9.49044795297831,23.6904671255976,-23.0073449072976));
#56758=CARTESIAN_POINT('Ctrl Pts',(9.49158074820728,23.7099626891003,-23.0064741240536));
#56759=CARTESIAN_POINT('Ctrl Pts',(9.49161858693997,23.7106138989546,-23.0064450373012));
#56760=CARTESIAN_POINT('Ctrl Pts',(9.49165629872179,23.7112651256649,-23.0064160480089));
#56761=CARTESIAN_POINT('Ctrl Pts',(9.49169388354751,23.7119163692475,-23.0063871561828));
#56762=CARTESIAN_POINT('Ctrl Pts',(9.49444525199611,23.7595901580923,-23.0042721521318));
#56763=CARTESIAN_POINT('Ctrl Pts',(9.49651672032079,23.8073536980638,-23.0026791277276));
#56764=CARTESIAN_POINT('Ctrl Pts',(9.49790308066639,23.855207727697,-23.0016128839398));
#56765=CARTESIAN_POINT('Ctrl Pts',(9.49790768768555,23.8553667515986,-23.0016093407011));
#56766=CARTESIAN_POINT('Ctrl Pts',(9.49791228713674,23.8555257765012,-23.0016058032811));
#56767=CARTESIAN_POINT('Ctrl Pts',(9.49791687901979,23.8556848024049,-23.0016022716799));
#56768=CARTESIAN_POINT('Ctrl Pts',(9.49860889038041,23.8796505112222,-23.001070048161));
#56769=CARTESIAN_POINT('Ctrl Pts',(9.49912904440715,23.9036389170042,-23.0006699492993));
#56770=CARTESIAN_POINT('Ctrl Pts',(9.49947652234889,23.9276501335531,-23.0004026681431));
#56771=CARTESIAN_POINT('Ctrl Pts',(9.49947711854897,23.927691331821,-23.0004022095441));
#56772=CARTESIAN_POINT('Ctrl Pts',(9.49947771424067,23.927732530156,-23.0004017513361));
#56773=CARTESIAN_POINT('Ctrl Pts',(9.49947830942397,23.9277737285583,-23.0004012935191));
#56774=CARTESIAN_POINT('Ctrl Pts',(9.49965176461952,23.939780243019,-23.0002678712071));
#56775=CARTESIAN_POINT('Ctrl Pts',(9.49978204199234,23.9517924031958,-23.0001676588957));
#56776=CARTESIAN_POINT('Ctrl Pts',(9.49986902956221,23.9638103980238,-23.0001007462648));
#56777=CARTESIAN_POINT('Ctrl Pts',(9.49986917252242,23.9638301490662,-23.0001006362969));
#56778=CARTESIAN_POINT('Ctrl Pts',(9.49986931536621,23.9638499000761,-23.0001005264185));
#56779=CARTESIAN_POINT('Ctrl Pts',(9.49986945809355,23.9638696510541,-23.0001004166297));
#56780=CARTESIAN_POINT('Ctrl Pts',(9.49991295239155,23.9698885043324,-23.0000669599194));
#56781=CARTESIAN_POINT('Ctrl Pts',(9.49994564654914,23.975908791834,-23.0000418550542));
#56782=CARTESIAN_POINT('Ctrl Pts',(9.49996740821826,23.9819305160761,-23.0000251152831));
#56783=CARTESIAN_POINT('Ctrl Pts',(9.49997828905281,23.9849413781972,-23.0000167453976));
#56784=CARTESIAN_POINT('Ctrl Pts',(9.49998644052914,23.9879525994516,-23.0000104666332));
#56785=CARTESIAN_POINT('Ctrl Pts',(9.49999186825306,23.9909641800319,-23.0000062802908));
#56786=CARTESIAN_POINT('Ctrl Pts',(9.49999458211502,23.9924699703221,-23.0000041871195));
#56787=CARTESIAN_POINT('Ctrl Pts',(9.49999661789029,23.9939777893432,-23.000002617044));
#56788=CARTESIAN_POINT('Ctrl Pts',(9.49999797235682,23.9954847287786,-23.0000015702666));
#56789=CARTESIAN_POINT('Ctrl Pts',(9.49999932682335,23.996991668214,-23.0000005234893));
#56790=CARTESIAN_POINT('Ctrl Pts',(9.5,23.9984977280603,-23.));
#56791=CARTESIAN_POINT('Ctrl Pts',(9.5,24.,-23.));
#56792=CARTESIAN_POINT('Ctrl Pts',(9.5,24.,-23.));
#56793=CARTESIAN_POINT('Ctrl Pts',(9.5,24.,-23.));
#56794=CARTESIAN_POINT('Ctrl Pts',(9.5,24.,-23.));
#56795=CARTESIAN_POINT('Ctrl Pts',(9.5,24.0107707732946,-23.0036032454852));
#56796=CARTESIAN_POINT('Ctrl Pts',(9.5,24.0113713024762,-23.0018019637283));
#56797=CARTESIAN_POINT('Ctrl Pts',(9.5,24.0119705177798,-22.9999999997818));
#56798=CARTESIAN_POINT('Ctrl Pts',(9.5,24.0215761177811,-23.0072252079635));
#56799=CARTESIAN_POINT('Ctrl Pts',(9.50000000000038,24.0227863409126,-23.0036292697814));
#56800=CARTESIAN_POINT('Ctrl Pts',(9.49995688111502,24.0239955794358,-23.0000331685107));
#56801=CARTESIAN_POINT('Ctrl Pts',(9.5,24.043142522989,-23.0145455206898));
#56802=CARTESIAN_POINT('Ctrl Pts',(9.49999999999963,24.0455947193631,-23.007354661754));
#56803=CARTESIAN_POINT('Ctrl Pts',(9.49978362345037,24.0480449740998,-23.0001664423046));
#56804=CARTESIAN_POINT('Ctrl Pts',(9.5,24.0539140788076,-23.0182343307261));
#56805=CARTESIAN_POINT('Ctrl Pts',(9.49999999999958,24.0569979580795,-23.0092477784199));
#56806=CARTESIAN_POINT('Ctrl Pts',(9.49965355251852,24.0600779429846,-23.0002664951942));
#56807=CARTESIAN_POINT('Ctrl Pts',(9.5,24.0861946039291,-23.0293847585427));
#56808=CARTESIAN_POINT('Ctrl Pts',(9.50000000000091,24.0912049332124,-23.0150154749917));
#56809=CARTESIAN_POINT('Ctrl Pts',(9.49913249141161,24.0961995403903,-23.0006672945158));
#56810=CARTESIAN_POINT('Ctrl Pts',(9.5,24.1076694276147,-23.0369303821088));
#56811=CARTESIAN_POINT('Ctrl Pts',(9.49999999999987,24.11400596502,-23.0189785154945));
#56812=CARTESIAN_POINT('Ctrl Pts',(9.49861063759759,24.1203108890296,-23.0010686949064));
#56813=CARTESIAN_POINT('Ctrl Pts',(9.5,24.1719637401203,-23.0598874716861));
#56814=CARTESIAN_POINT('Ctrl Pts',(9.50000000000028,24.1824051319777,-23.0311985864123));
#56815=CARTESIAN_POINT('Ctrl Pts',(9.49651797711653,24.1927178505562,-23.002678159501));
#56816=CARTESIAN_POINT('Ctrl Pts',(9.5,24.2146530324576,-23.0756192498966));
#56817=CARTESIAN_POINT('Ctrl Pts',(9.5,24.2279999517257,-23.0397882481961));
#56818=CARTESIAN_POINT('Ctrl Pts',(9.49441978273465,24.2410867609359,-23.0042917444127));
#56819=CARTESIAN_POINT('Ctrl Pts',(9.5,24.342252592613,-23.1239667477747));
#56820=CARTESIAN_POINT('Ctrl Pts',(9.50000000000001,24.3648279313251,-23.0666954340358));
#56821=CARTESIAN_POINT('Ctrl Pts',(9.4859961316791,24.3863285463,-23.0107670313098));
#56822=CARTESIAN_POINT('Ctrl Pts',(9.5,24.4266936912028,-23.1577367277137));
#56823=CARTESIAN_POINT('Ctrl Pts',(9.5,24.456115688764,-23.0861754816071));
#56824=CARTESIAN_POINT('Ctrl Pts',(9.47753582904777,24.4833406390942,-23.0172682908757));
#56825=CARTESIAN_POINT('Ctrl Pts',(9.5,24.5946215322546,-23.2276246151516));
#56826=CARTESIAN_POINT('Ctrl Pts',(9.5,24.6380844425336,-23.1268503195308));
#56827=CARTESIAN_POINT('Ctrl Pts',(9.4549436591157,24.6767676391327,-23.0345986860669));
#56828=CARTESIAN_POINT('Ctrl Pts',(9.5,24.6781079464887,-23.2637433301653));
#56829=CARTESIAN_POINT('Ctrl Pts',(9.5,24.7293174158525,-23.1481886748754));
#56830=CARTESIAN_POINT('Ctrl Pts',(9.44081101359461,24.7731794793018,-23.0454283451806));
#56831=CARTESIAN_POINT('Ctrl Pts',(9.5,24.8444527832798,-23.3375257588818));
#56832=CARTESIAN_POINT('Ctrl Pts',(9.5,24.911229778195,-23.1912116065894));
#56833=CARTESIAN_POINT('Ctrl Pts',(9.40708347472986,24.9643400592328,-23.0712092888382));
#56834=CARTESIAN_POINT('Ctrl Pts',(9.5,24.9273157101134,-23.3751926161801));
#56835=CARTESIAN_POINT('Ctrl Pts',(9.49999999999999,25.0024985119011,-23.2130417643524));
#56836=CARTESIAN_POINT('Ctrl Pts',(9.38748745363412,25.0590910627534,-23.0861612580384));
#56837=CARTESIAN_POINT('Ctrl Pts',(9.5,25.0927535278966,-23.4511555606396));
#56838=CARTESIAN_POINT('Ctrl Pts',(9.5,25.1844829408851,-23.2553985341106));
#56839=CARTESIAN_POINT('Ctrl Pts',(9.34325331477361,25.2458349876977,-23.1198043547188));
#56840=CARTESIAN_POINT('Ctrl Pts',(9.5,25.1753282792467,-23.489453136662));
#56841=CARTESIAN_POINT('Ctrl Pts',(9.50000000000008,25.2758237696641,-23.2760366549509));
#56842=CARTESIAN_POINT('Ctrl Pts',(9.318617008943,25.337826228914,-23.1384938689611));
#56843=CARTESIAN_POINT('Ctrl Pts',(9.5,25.3406539206004,-23.5656620578112));
#56844=CARTESIAN_POINT('Ctrl Pts',(9.49999999999992,25.4579441583579,-23.313966433972));
#56845=CARTESIAN_POINT('Ctrl Pts',(9.26488590318243,25.5181275405444,-23.1790959473744));
#56846=CARTESIAN_POINT('Ctrl Pts',(9.5,25.423403494808,-23.6035762881703));
#56847=CARTESIAN_POINT('Ctrl Pts',(9.5,25.5494052497834,-23.3312829901189));
#56848=CARTESIAN_POINT('Ctrl Pts',(9.23579261828811,25.6064362448348,-23.2010070869905));
#56849=CARTESIAN_POINT('Ctrl Pts',(9.5,25.5480717646467,-23.6592549694445));
#56850=CARTESIAN_POINT('Ctrl Pts',(9.5,25.6844789749892,-23.3524683984995));
#56851=CARTESIAN_POINT('Ctrl Pts',(9.18934162578665,25.7355596799467,-23.2358304718725));
#56852=CARTESIAN_POINT('Ctrl Pts',(9.5,25.5897238328085,-23.6776159939313));
#56853=CARTESIAN_POINT('Ctrl Pts',(9.5,25.7300285903091,-23.358820780593));
#56854=CARTESIAN_POINT('Ctrl Pts',(9.17338849315615,25.7780500646053,-23.2477650930033));
#56855=CARTESIAN_POINT('Ctrl Pts',(9.5,25.6732669052373,-23.7137476754764));
#56856=CARTESIAN_POINT('Ctrl Pts',(9.50000000000001,25.8208995483994,-23.3695293737685));
#56857=CARTESIAN_POINT('Ctrl Pts',(9.1406536309599,25.8618152227635,-23.2721956166015));
#56858=CARTESIAN_POINT('Ctrl Pts',(9.5,25.7151562043981,-23.7315179679288));
#56859=CARTESIAN_POINT('Ctrl Pts',(9.50000000000004,25.8663165149287,-23.3738465749513));
#56860=CARTESIAN_POINT('Ctrl Pts',(9.12387264986927,25.9030885502717,-23.2846909536321));
#56861=CARTESIAN_POINT('Ctrl Pts',(9.5,25.799252971265,-23.7662600488738));
#56862=CARTESIAN_POINT('Ctrl Pts',(9.49999999999996,25.9567720637753,-23.3799202018829));
#56863=CARTESIAN_POINT('Ctrl Pts',(9.08958987284599,25.9843409786744,-23.310153196582));
#56864=CARTESIAN_POINT('Ctrl Pts',(9.5,25.8414602653049,-23.7832322732144));
#56865=CARTESIAN_POINT('Ctrl Pts',(9.49999999999993,26.001911994365,-23.3816095528176));
#56866=CARTESIAN_POINT('Ctrl Pts',(9.0720880958929,26.0243201247937,-23.3231200767674));
#56867=CARTESIAN_POINT('Ctrl Pts',(9.5,25.9262896923711,-23.8161356052345));
#56868=CARTESIAN_POINT('Ctrl Pts',(9.50000000000008,26.091562040964,-23.381710222438));
#56869=CARTESIAN_POINT('Ctrl Pts',(9.0364737853881,26.1029187167218,-23.3494349509243));
#56870=CARTESIAN_POINT('Ctrl Pts',(9.5,25.9689115826802,-23.8320674299984));
#56871=CARTESIAN_POINT('Ctrl Pts',(9.49999999999992,26.1361727648094,-23.3800129429126));
#56872=CARTESIAN_POINT('Ctrl Pts',(9.01836122083488,26.1415382980706,-23.3627829574348));
#56873=CARTESIAN_POINT('Ctrl Pts',(9.5,26.0117995124034,-23.8473313628081));
#56874=CARTESIAN_POINT('Ctrl Pts',(9.5,26.1794494717704,-23.3762756430421));
#56875=CARTESIAN_POINT('Ctrl Pts',(9.,26.1794494717703,-23.3762756430421));
#56876=CARTESIAN_POINT('Ctrl Pts',(9.5,24.0000000040242,-23.));
#56877=CARTESIAN_POINT('Ctrl Pts',(9.49999999999996,24.0000472133395,-23.));
#56878=CARTESIAN_POINT('Ctrl Pts',(9.49999999932927,24.0000944225004,-23.0000000005142));
#56879=CARTESIAN_POINT('Ctrl Pts',(9.49999999798799,24.000141631506,-23.0000000015451));
#56880=CARTESIAN_POINT('Ctrl Pts',(9.49999965791715,24.0121110966267,-23.0000002629244));
#56881=CARTESIAN_POINT('Ctrl Pts',(9.49995633974189,24.0240707258725,-23.0000335849474));
#56882=CARTESIAN_POINT('Ctrl Pts',(9.4998702522827,24.0360202767678,-23.0000998054077));
#56883=CARTESIAN_POINT('Ctrl Pts',(9.49978349403696,24.0480629376004,-23.0001665418524));
#56884=CARTESIAN_POINT('Ctrl Pts',(9.49965329563524,24.0600957509431,-23.0002666927884));
#56885=CARTESIAN_POINT('Ctrl Pts',(9.49947986548288,24.0721184754532,-23.0004000949681));
#56886=CARTESIAN_POINT('Ctrl Pts',(9.49913150351934,24.0962680241944,-23.0006680544009));
#56887=CARTESIAN_POINT('Ctrl Pts',(9.4986087194461,24.1203772579043,-23.0010701701562));
#56888=CARTESIAN_POINT('Ctrl Pts',(9.4979130841039,24.1444465428718,-23.0016051831046));
#56889=CARTESIAN_POINT('Ctrl Pts',(9.49652417723532,24.1925033237533,-23.0026733909914));
#56890=CARTESIAN_POINT('Ctrl Pts',(9.49444633029441,24.2404008834145,-23.0042713242624));
#56891=CARTESIAN_POINT('Ctrl Pts',(9.49169052182656,24.2881418631175,-23.0063897356217));
#56892=CARTESIAN_POINT('Ctrl Pts',(9.49166437530495,24.2885948193269,-23.0064098346558));
#56893=CARTESIAN_POINT('Ctrl Pts',(9.49163816771039,24.2890477614159,-23.0064299805766));
#56894=CARTESIAN_POINT('Ctrl Pts',(9.49161189904947,24.2895006893906,-23.0064501733784));
#56895=CARTESIAN_POINT('Ctrl Pts',(9.48730051344177,24.3638382110829,-23.0097643489723));
#56896=CARTESIAN_POINT('Ctrl Pts',(9.48134411970086,24.4377967804438,-23.0143417189762));
#56897=CARTESIAN_POINT('Ctrl Pts',(9.47377934160028,24.5113827873064,-23.020148189609));
#56898=CARTESIAN_POINT('Ctrl Pts',(9.47168117088454,24.531792639735,-23.0217586752678));
#56899=CARTESIAN_POINT('Ctrl Pts',(9.46945903057479,24.5521739042804,-23.0234638993713));
#56900=CARTESIAN_POINT('Ctrl Pts',(9.46711315648692,24.57252684519,-23.0252635570472));
#56901=CARTESIAN_POINT('Ctrl Pts',(9.46682390991272,24.5750363653997,-23.0254854550682));
#56902=CARTESIAN_POINT('Ctrl Pts',(9.46653278205055,24.5775454534323,-23.0257087886514));
#56903=CARTESIAN_POINT('Ctrl Pts',(9.46623977302995,24.5800541104005,-23.0259335574633));
#56904=CARTESIAN_POINT('Ctrl Pts',(9.45768749975581,24.653276156256,-23.0324940527649));
#56905=CARTESIAN_POINT('Ctrl Pts',(9.44753564798023,24.7261294634645,-23.0402748674687));
#56906=CARTESIAN_POINT('Ctrl Pts',(9.43580765439745,24.7986205596957,-23.0492484623702));
#56907=CARTESIAN_POINT('Ctrl Pts',(9.43285767757367,24.8168544589815,-23.0515056171681));
#56908=CARTESIAN_POINT('Ctrl Pts',(9.42980777682099,24.8350654145798,-23.0538383945911));
#56909=CARTESIAN_POINT('Ctrl Pts',(9.42665792176129,24.8532534454377,-23.0562466662163));
#56910=CARTESIAN_POINT('Ctrl Pts',(9.4257624556697,24.8584240849108,-23.0569313090138));
#56911=CARTESIAN_POINT('Ctrl Pts',(9.42485891395591,24.8635928460027,-23.0576220492631));
#56912=CARTESIAN_POINT('Ctrl Pts',(9.42394729195393,24.8687597382769,-23.0583188868783));
#56913=CARTESIAN_POINT('Ctrl Pts',(9.41145567335872,24.9395597491057,-23.0678673945851));
#56914=CARTESIAN_POINT('Ctrl Pts',(9.39744936228768,25.0100120041573,-23.0785588266677));
#56915=CARTESIAN_POINT('Ctrl Pts',(9.38193889032673,25.0801218265281,-23.0903723732737));
#56916=CARTESIAN_POINT('Ctrl Pts',(9.37822780110935,25.0968965453431,-23.0931989233322));
#56917=CARTESIAN_POINT('Ctrl Pts',(9.37443043919756,25.1136515462175,-23.0960898323589));
#56918=CARTESIAN_POINT('Ctrl Pts',(9.37054664849349,25.1303866581631,-23.0990450356101));
#56919=CARTESIAN_POINT('Ctrl Pts',(9.36883796974238,25.1377492923413,-23.1003451811085));
#56920=CARTESIAN_POINT('Ctrl Pts',(9.36711255863857,25.1451080841838,-23.1016577737905));
#56921=CARTESIAN_POINT('Ctrl Pts',(9.36537039239686,25.152463021566,-23.1029828143487));
#56922=CARTESIAN_POINT('Ctrl Pts',(9.34910220872428,25.2211427315552,-23.1153559178207));
#56923=CARTESIAN_POINT('Ctrl Pts',(9.33137622513788,25.2894886756205,-23.1288120750233));
#56924=CARTESIAN_POINT('Ctrl Pts',(9.31218977706049,25.357505871556,-23.1433366982879));
#56925=CARTESIAN_POINT('Ctrl Pts',(9.30781686779381,25.3730081169535,-23.1466471004745));
#56926=CARTESIAN_POINT('Ctrl Pts',(9.30336798794396,25.3884931139944,-23.1500130748811));
#56927=CARTESIAN_POINT('Ctrl Pts',(9.29884292932147,25.403960598041,-23.1534345633324));
#56928=CARTESIAN_POINT('Ctrl Pts',(9.29649960113489,25.4119705255062,-23.1552064012238));
#56929=CARTESIAN_POINT('Ctrl Pts',(9.29413504811856,25.4199784648416,-23.1569937465278));
#56930=CARTESIAN_POINT('Ctrl Pts',(9.29175146133725,25.4279768831427,-23.1587949116094));
#56931=CARTESIAN_POINT('Ctrl Pts',(9.29076497192154,25.4312871695809,-23.1595403555358));
#56932=CARTESIAN_POINT('Ctrl Pts',(9.28977522583227,25.4345958245047,-23.1602881635823));
#56933=CARTESIAN_POINT('Ctrl Pts',(9.28878238789445,25.4379023226279,-23.1610382090628));
#56934=CARTESIAN_POINT('Ctrl Pts',(9.28539062367631,25.4491980856065,-23.1636005380451));
#56935=CARTESIAN_POINT('Ctrl Pts',(9.2819628000743,25.4604686495923,-23.1661889748205));
#56936=CARTESIAN_POINT('Ctrl Pts',(9.27849919458189,25.4717142458895,-23.1688032058496));
#56937=CARTESIAN_POINT('Ctrl Pts',(9.27157198359708,25.4942054384839,-23.1740316679079));
#56938=CARTESIAN_POINT('Ctrl Pts',(9.26450166607491,25.5165967715549,-23.1793632829727));
#56939=CARTESIAN_POINT('Ctrl Pts',(9.25729019799641,25.5388898580472,-23.1847957915743));
#56940=CARTESIAN_POINT('Ctrl Pts',(9.24286726183941,25.5834760310319,-23.1956608087775));
#56941=CARTESIAN_POINT('Ctrl Pts',(9.22787987878526,25.6276693970273,-23.2069289952489));
#56942=CARTESIAN_POINT('Ctrl Pts',(9.21234040799161,25.671480427866,-23.2185867719651));
#56943=CARTESIAN_POINT('Ctrl Pts',(9.20984952418265,25.6785030728981,-23.2204554435342));
#56944=CARTESIAN_POINT('Ctrl Pts',(9.20734448156849,25.6855157445879,-23.222334090199));
#56945=CARTESIAN_POINT('Ctrl Pts',(9.20482529266609,25.6925185344127,-23.2242226780239));
#56946=CARTESIAN_POINT('Ctrl Pts',(9.18941669728229,25.7353510329467,-23.2357742078093));
#56947=CARTESIAN_POINT('Ctrl Pts',(9.17347821168034,25.7778206195918,-23.2476981969414));
#56948=CARTESIAN_POINT('Ctrl Pts',(9.15702114870062,25.8199326323079,-23.259980381107));
#56949=CARTESIAN_POINT('Ctrl Pts',(9.14259793406752,25.856840226256,-23.270744669887));
#56950=CARTESIAN_POINT('Ctrl Pts',(9.1277768646073,25.8934718677887,-23.2817837311289));
#56951=CARTESIAN_POINT('Ctrl Pts',(9.11256256614465,25.9298360791784,-23.2930899518817));
#56952=CARTESIAN_POINT('Ctrl Pts',(9.11062517609986,25.9344667009126,-23.2945296869825));
#56953=CARTESIAN_POINT('Ctrl Pts',(9.10868143263058,25.9390929204726,-23.2959737374947));
#56954=CARTESIAN_POINT('Ctrl Pts',(9.10673134009713,25.943714757904,-23.2974220910081));
#56955=CARTESIAN_POINT('Ctrl Pts',(9.08972898401147,25.9840113717474,-23.3100499134061));
#56956=CARTESIAN_POINT('Ctrl Pts',(9.0722440168628,26.0239760614906,-23.3230048868648));
#56957=CARTESIAN_POINT('Ctrl Pts',(9.05428095101056,26.0636194203482,-23.3362775149017));
#56958=CARTESIAN_POINT('Ctrl Pts',(9.03664587444704,26.1025389274324,-23.3493077967898));
#56959=CARTESIAN_POINT('Ctrl Pts',(9.01854981494457,26.1411488999954,-23.3626443696441));
#56960=CARTESIAN_POINT('Ctrl Pts',(9.,26.1794494717703,-23.3762756430421));
#56961=CARTESIAN_POINT('Origin',(0.5,48.5249973351313,-4.97500266486866));
#56962=CARTESIAN_POINT('Ctrl Pts',(9.5,24.,-36.));
#56963=CARTESIAN_POINT('Ctrl Pts',(9.5,24.,-36.));
#56964=CARTESIAN_POINT('Ctrl Pts',(9.5,24.,-36.));
#56965=CARTESIAN_POINT('Ctrl Pts',(9.5,23.9892292267054,-35.9963967545148));
#56966=CARTESIAN_POINT('Ctrl Pts',(9.5,23.9886286975238,-35.9981980362717));
#56967=CARTESIAN_POINT('Ctrl Pts',(9.5,23.9880294822202,-36.0000000002183));
#56968=CARTESIAN_POINT('Ctrl Pts',(9.5,23.9784238822189,-35.9927747920365));
#56969=CARTESIAN_POINT('Ctrl Pts',(9.50000000000064,23.9772136590874,-35.9963707302186));
#56970=CARTESIAN_POINT('Ctrl Pts',(9.49995688111502,23.9760044205641,-35.9999668314893));
#56971=CARTESIAN_POINT('Ctrl Pts',(9.5,23.956857477011,-35.9854544793102));
#56972=CARTESIAN_POINT('Ctrl Pts',(9.49999999999976,23.9544052806369,-35.992645338246));
#56973=CARTESIAN_POINT('Ctrl Pts',(9.49978362345037,23.9519550259002,-35.9998335576954));
#56974=CARTESIAN_POINT('Ctrl Pts',(9.5,23.9460859211924,-35.9817656692739));
#56975=CARTESIAN_POINT('Ctrl Pts',(9.49999999999952,23.9430020419206,-35.9907522215798));
#56976=CARTESIAN_POINT('Ctrl Pts',(9.49965355251852,23.9399220570155,-35.9997335048058));
#56977=CARTESIAN_POINT('Ctrl Pts',(9.5,23.9138053960708,-35.9706152414573));
#56978=CARTESIAN_POINT('Ctrl Pts',(9.50000000000086,23.9087950667873,-35.9849845250087));
#56979=CARTESIAN_POINT('Ctrl Pts',(9.49913249141161,23.9038004596097,-35.9993327054842));
#56980=CARTESIAN_POINT('Ctrl Pts',(9.5,23.8923305723853,-35.9630696178911));
#56981=CARTESIAN_POINT('Ctrl Pts',(9.49999999999997,23.88599403498,-35.9810214845054));
#56982=CARTESIAN_POINT('Ctrl Pts',(9.49861063759758,23.8796891109704,-35.9989313050937));
#56983=CARTESIAN_POINT('Ctrl Pts',(9.5,23.8280362598797,-35.940112528314));
#56984=CARTESIAN_POINT('Ctrl Pts',(9.50000000000009,23.8175948680224,-35.9688014135879));
#56985=CARTESIAN_POINT('Ctrl Pts',(9.49651797711654,23.8072821494439,-35.9973218404989));
#56986=CARTESIAN_POINT('Ctrl Pts',(9.5,23.7853469675425,-35.9243807501034));
#56987=CARTESIAN_POINT('Ctrl Pts',(9.50000000000004,23.7720000482745,-35.9602117518039));
#56988=CARTESIAN_POINT('Ctrl Pts',(9.49441978273462,23.7589132390644,-35.9957082555875));
#56989=CARTESIAN_POINT('Ctrl Pts',(9.5,23.6577474073867,-35.8760332522253));
#56990=CARTESIAN_POINT('Ctrl Pts',(9.49999999999992,23.6351720686746,-35.9333045659642));
#56991=CARTESIAN_POINT('Ctrl Pts',(9.48599613167915,23.6136714536995,-35.9892329686897));
#56992=CARTESIAN_POINT('Ctrl Pts',(9.5,23.5733063087972,-35.842263272286));
#56993=CARTESIAN_POINT('Ctrl Pts',(9.49999999999999,23.5438843112363,-35.9138245183926));
#56994=CARTESIAN_POINT('Ctrl Pts',(9.47753582904787,23.5166593609058,-35.982731709124));
#56995=CARTESIAN_POINT('Ctrl Pts',(9.5,23.4053784677454,-35.7723753848487));
#56996=CARTESIAN_POINT('Ctrl Pts',(9.5,23.361915557466,-35.8731496804695));
#56997=CARTESIAN_POINT('Ctrl Pts',(9.45494365911559,23.3232323608673,-35.9654013139334));
#56998=CARTESIAN_POINT('Ctrl Pts',(9.5,23.3218920535115,-35.7362566698346));
#56999=CARTESIAN_POINT('Ctrl Pts',(9.49999999999992,23.2706825841475,-35.8518113251246));
#57000=CARTESIAN_POINT('Ctrl Pts',(9.44081101359471,23.2268205206985,-35.9545716548194));
#57001=CARTESIAN_POINT('Ctrl Pts',(9.5,23.15554721672,-35.6624742411183));
#57002=CARTESIAN_POINT('Ctrl Pts',(9.50000000000008,23.088770221805,-35.8087883934105));
#57003=CARTESIAN_POINT('Ctrl Pts',(9.40708347472976,23.035659940767,-35.9287907111618));
#57004=CARTESIAN_POINT('Ctrl Pts',(9.5,23.0726842898868,-35.6248073838195));
#57005=CARTESIAN_POINT('Ctrl Pts',(9.5,22.9975014880992,-35.7869582356476));
#57006=CARTESIAN_POINT('Ctrl Pts',(9.38748745363404,22.9409089372467,-35.9138387419617));
#57007=CARTESIAN_POINT('Ctrl Pts',(9.5,22.9072464721032,-35.5488444393607));
#57008=CARTESIAN_POINT('Ctrl Pts',(9.5,22.8155170591146,-35.7446014658894));
#57009=CARTESIAN_POINT('Ctrl Pts',(9.34325331477368,22.7541650123022,-35.8801956452811));
#57010=CARTESIAN_POINT('Ctrl Pts',(9.5,22.8246717207533,-35.5105468633386));
#57011=CARTESIAN_POINT('Ctrl Pts',(9.5,22.7241762303391,-35.7239633450498));
#57012=CARTESIAN_POINT('Ctrl Pts',(9.31861700894411,22.6621737710915,-35.8615061310396));
#57013=CARTESIAN_POINT('Ctrl Pts',(9.5,22.6593460793993,-35.4343379421891));
#57014=CARTESIAN_POINT('Ctrl Pts',(9.50000000000001,22.5420558416456,-35.6860335660284));
#57015=CARTESIAN_POINT('Ctrl Pts',(9.26488590318484,22.4818724594602,-35.8209040526278));
#57016=CARTESIAN_POINT('Ctrl Pts',(9.5,22.5765965051919,-35.3964237118294));
#57017=CARTESIAN_POINT('Ctrl Pts',(9.5,22.4505947502163,-35.6687170098806));
#57018=CARTESIAN_POINT('Ctrl Pts',(9.23579261828804,22.3935637551648,-35.7989929130094));
#57019=CARTESIAN_POINT('Ctrl Pts',(9.5,22.4519282353534,-35.3407450305557));
#57020=CARTESIAN_POINT('Ctrl Pts',(9.5,22.3155210250109,-35.6475316015007));
#57021=CARTESIAN_POINT('Ctrl Pts',(9.18934162578669,22.2644403200535,-35.7641695281276));
#57022=CARTESIAN_POINT('Ctrl Pts',(9.5,22.4102761671915,-35.3223840060685));
#57023=CARTESIAN_POINT('Ctrl Pts',(9.50000000000004,22.2699714096911,-35.641179219407));
#57024=CARTESIAN_POINT('Ctrl Pts',(9.17338849315615,22.2219499353948,-35.7522349069968));
#57025=CARTESIAN_POINT('Ctrl Pts',(9.5,22.3267330947627,-35.2862523245238));
#57026=CARTESIAN_POINT('Ctrl Pts',(9.49999999999996,22.1791004516003,-35.6304706262315));
#57027=CARTESIAN_POINT('Ctrl Pts',(9.1406536309599,22.1381847772365,-35.7278043833984));
#57028=CARTESIAN_POINT('Ctrl Pts',(9.5,22.2848437956018,-35.2684820320708));
#57029=CARTESIAN_POINT('Ctrl Pts',(9.49999999999997,22.1336834850712,-35.6261534250485));
#57030=CARTESIAN_POINT('Ctrl Pts',(9.12387264986921,22.0969114497283,-35.7153090463679));
#57031=CARTESIAN_POINT('Ctrl Pts',(9.5,22.2007470287351,-35.2337399511265));
#57032=CARTESIAN_POINT('Ctrl Pts',(9.50000000000004,22.0432279362249,-35.6200797981173));
#57033=CARTESIAN_POINT('Ctrl Pts',(9.08958987284604,22.0156590213257,-35.689846803418));
#57034=CARTESIAN_POINT('Ctrl Pts',(9.5,22.1585397346952,-35.2167677267856));
#57035=CARTESIAN_POINT('Ctrl Pts',(9.5,21.998088005635,-35.6183904471824));
#57036=CARTESIAN_POINT('Ctrl Pts',(9.07208809589285,21.9756798752063,-35.6768799232326));
#57037=CARTESIAN_POINT('Ctrl Pts',(9.5,22.0737103076288,-35.1838643947655));
#57038=CARTESIAN_POINT('Ctrl Pts',(9.5,21.908437959036,-35.618289777562));
#57039=CARTESIAN_POINT('Ctrl Pts',(9.03647378538813,21.8970812832782,-35.6505650490757));
#57040=CARTESIAN_POINT('Ctrl Pts',(9.5,22.0310884173198,-35.1679325700017));
#57041=CARTESIAN_POINT('Ctrl Pts',(9.5,21.8638272351906,-35.619987057087));
#57042=CARTESIAN_POINT('Ctrl Pts',(9.0183612208349,21.8584617019294,-35.6372170425652));
#57043=CARTESIAN_POINT('Ctrl Pts',(9.5,21.9882004875966,-35.1526686371919));
#57044=CARTESIAN_POINT('Ctrl Pts',(9.5,21.8205505282297,-35.6237243569579));
#57045=CARTESIAN_POINT('Ctrl Pts',(9.,21.8205505282297,-35.6237243569579));
#57046=CARTESIAN_POINT('Origin',(4.5,24.,6.93889390390723E-15));
#57047=CARTESIAN_POINT('',(-0.474937191429098,24.5000000003648,-16.9721648040778));
#57048=CARTESIAN_POINT('',(-0.474937185533101,24.5,6.93889390390723E-15));
#57049=CARTESIAN_POINT('',(-0.474939105079448,23.4999999870496,-16.9721648040678));
#57050=CARTESIAN_POINT('Ctrl Pts',(-0.474937185533101,24.5,-16.9721648040778));
#57051=CARTESIAN_POINT('Ctrl Pts',(-0.470797194023869,24.5411923954141,
-16.9724257278495));
#57052=CARTESIAN_POINT('Ctrl Pts',(-0.466146469130312,24.5823254588545,
-16.9727170296826));
#57053=CARTESIAN_POINT('Ctrl Pts',(-0.458404454236442,24.6439360926595,
-16.9731972461152));
#57054=CARTESIAN_POINT('Ctrl Pts',(-0.455695504183399,24.6644618374713,
-16.9733645613487));
#57055=CARTESIAN_POINT('Ctrl Pts',(-0.45003097975852,24.7054224004596,-16.9737126265433));
#57056=CARTESIAN_POINT('Ctrl Pts',(-0.435248508164381,24.8076327210798,
-16.9746165749486));
#57057=CARTESIAN_POINT('Ctrl Pts',(-0.417381523850264,24.9088942257275,
-16.975683228821));
#57058=CARTESIAN_POINT('Ctrl Pts',(-0.368686732985424,25.150134146398,-16.9784953288194));
#57059=CARTESIAN_POINT('Ctrl Pts',(-0.288284000987233,25.4670286188676,
-16.9829238382787));
#57060=CARTESIAN_POINT('Ctrl Pts',(-0.177378303243287,25.7745546543069,
-16.9878975211825));
#57061=CARTESIAN_POINT('Ctrl Pts',(-0.0825936022986651,26.0016402971975,
-16.9914298199687));
#57062=CARTESIAN_POINT('Ctrl Pts',(-0.0490609928049965,26.0767413134168,
-16.9925731939087));
#57063=CARTESIAN_POINT('Ctrl Pts',(-0.00467819423663701,26.169861750507,
-16.9939088357422));
#57064=CARTESIAN_POINT('Ctrl Pts',(0.00432179345813184,26.1884480232583,
-16.9941712588045));
#57065=CARTESIAN_POINT('Ctrl Pts',(0.0225700581715561,26.2255445183813,
-16.9946853096135));
#57066=CARTESIAN_POINT('Ctrl Pts',(0.0318248797997421,26.2440674949246,
-16.9949371041111));
#57067=CARTESIAN_POINT('Ctrl Pts',(0.0599035246156764,26.2994030954782,
-16.995672587935));
#57068=CARTESIAN_POINT('Ctrl Pts',(0.0790429353757529,26.3359874557493,
-16.9961364897616));
#57069=CARTESIAN_POINT('Ctrl Pts',(0.176818437108739,26.5173957465966,-16.9982977437359));
#57070=CARTESIAN_POINT('Ctrl Pts',(0.261674360831238,26.6576904507745,-16.9995234138429));
#57071=CARTESIAN_POINT('Ctrl Pts',(0.444321993216878,26.9288562035493,-17.0002526361575));
#57072=CARTESIAN_POINT('Ctrl Pts',(0.542114396216129,27.0597267530717,-16.9997573671339));
#57073=CARTESIAN_POINT('Ctrl Pts',(0.750680443960419,27.3120068120101,-16.9962341377482));
#57074=CARTESIAN_POINT('Ctrl Pts',(0.861452940867902,27.4334171664224,-16.9932079888594));
#57075=CARTESIAN_POINT('Ctrl Pts',(0.99361456223937,27.5645040251486,-16.9878439808329));
#57076=CARTESIAN_POINT('Ctrl Pts',(1.00840115368406,27.5789893043023,-16.9872207317832));
#57077=CARTESIAN_POINT('Ctrl Pts',(1.03810042360633,27.6077248047586,-16.9859214394814));
#57078=CARTESIAN_POINT('Ctrl Pts',(1.08286917614699,27.6505060822827,-16.9838920859762));
#57079=CARTESIAN_POINT('Ctrl Pts',(1.188858130302,27.7480881794548,-16.9785796041949));
#57080=CARTESIAN_POINT('Ctrl Pts',(1.28229298272252,27.8279292267126,-16.9729868122735));
#57081=CARTESIAN_POINT('Ctrl Pts',(1.47254721988554,27.9826187514255,-16.9602800962833));
#57082=CARTESIAN_POINT('Ctrl Pts',(1.60388844894043,28.0790994660127,-16.9497830742527));
#57083=CARTESIAN_POINT('Ctrl Pts',(1.87542831134558,28.2588892942784,-16.923971022276));
#57084=CARTESIAN_POINT('Ctrl Pts',(2.01562691262817,28.3421986363132,-16.9086574377018));
#57085=CARTESIAN_POINT('Ctrl Pts',(2.19646956016925,28.4379525039625,-16.8859701915491));
#57086=CARTESIAN_POINT('Ctrl Pts',(2.23291842136431,28.4566832330055,-16.8812551930949));
#57087=CARTESIAN_POINT('Ctrl Pts',(2.2880151864085,28.4841436490512,-16.873905381881));
#57088=CARTESIAN_POINT('Ctrl Pts',(2.30645431779413,28.4931925899314,-16.8714088149193));
#57089=CARTESIAN_POINT('Ctrl Pts',(2.34346217828623,28.5110715948272,-16.8663230193847));
#57090=CARTESIAN_POINT('Ctrl Pts',(2.43612492640257,28.5551344144511,-16.8534017967175));
#57091=CARTESIAN_POINT('Ctrl Pts',(2.52949327362936,28.5960520347272,-16.8394382727757));
#57092=CARTESIAN_POINT('Ctrl Pts',(2.75487169864856,28.6883783411955,-16.803857516293));
#57093=CARTESIAN_POINT('Ctrl Pts',(2.90684631178956,28.7421072493515,-16.7773800236118));
#57094=CARTESIAN_POINT('Ctrl Pts',(3.21401274740079,28.834455152834,-16.7185414151844));
#57095=CARTESIAN_POINT('Ctrl Pts',(3.3692050437863,28.873072940841,-16.686180930445));
#57096=CARTESIAN_POINT('Ctrl Pts',(3.60431757046051,28.9197700419179,-16.6329277059702));
#57097=CARTESIAN_POINT('Ctrl Pts',(3.72245604807308,28.9403067675921,-16.6051225169927));
#57098=CARTESIAN_POINT('Ctrl Pts',(3.84146173671369,28.9566050075574,-16.5754879243563));
#57099=CARTESIAN_POINT('Ctrl Pts',(3.90110916247106,28.964043838043,-16.5603602636752));
#57100=CARTESIAN_POINT('Ctrl Pts',(3.92102330682397,28.966405932644,-16.5552640265692));
#57101=CARTESIAN_POINT('Ctrl Pts',(3.96086673143964,28.9708889766091,-16.544975726032));
#57102=CARTESIAN_POINT('Ctrl Pts',(4.13998708103765,28.9899485771674,-16.4983101446476));
#57103=CARTESIAN_POINT('Ctrl Pts',(4.31754265331675,28.9991242551688,-16.4483414929103));
#57104=CARTESIAN_POINT('Ctrl Pts',(4.63080514657345,29.0007423464527,-16.3543944500403));
#57105=CARTESIAN_POINT('Ctrl Pts',(4.94167551686651,28.9876617690864,-16.2553333964929));
#57106=CARTESIAN_POINT('Ctrl Pts',(5.24786893282216,28.946165318101,-16.146223149621));
#57107=CARTESIAN_POINT('Ctrl Pts',(5.43779727915631,28.9114180710996,-16.0749371695464));
#57108=CARTESIAN_POINT('Ctrl Pts',(5.47571076690044,28.9040271040352,-16.060525344647));
#57109=CARTESIAN_POINT('Ctrl Pts',(5.55139363775732,28.8883601295569,-16.0313935531728));
#57110=CARTESIAN_POINT('Ctrl Pts',(5.5891799220155,28.8800794888932,-16.016666632018));
#57111=CARTESIAN_POINT('Ctrl Pts',(5.70195424529067,28.8539943215851,-15.9721724441926));
#57112=CARTESIAN_POINT('Ctrl Pts',(5.85099160100143,28.8158563894363,-15.9119240256477));
#57113=CARTESIAN_POINT('Ctrl Pts',(5.99743544461135,28.7711143481946,-15.8499070518029));
#57114=CARTESIAN_POINT('Ctrl Pts',(6.08816789477528,28.7411062055865,-15.8106180317806));
#57115=CARTESIAN_POINT('Ctrl Pts',(6.10627462109521,28.7350022996597,-15.8027338085013));
#57116=CARTESIAN_POINT('Ctrl Pts',(6.14240887067895,28.7225901831169,-15.7869131363904));
#57117=CARTESIAN_POINT('Ctrl Pts',(6.16043745190374,28.7162814808635,-15.7789761765381));
#57118=CARTESIAN_POINT('Ctrl Pts',(6.21431854028686,28.6970805928907,-15.7551263393622));
#57119=CARTESIAN_POINT('Ctrl Pts',(6.24999547230599,28.6839038442371,-15.7391618389056));
#57120=CARTESIAN_POINT('Ctrl Pts',(6.42718457724082,28.6161661156919,-15.659032731462));
#57121=CARTESIAN_POINT('Ctrl Pts',(6.56511818970728,28.5560582468655,-15.5939476458852));
#57122=CARTESIAN_POINT('Ctrl Pts',(6.83381314471484,28.4244430261726,-15.4622423546226));
#57123=CARTESIAN_POINT('Ctrl Pts',(6.96457354178166,28.3529347516141,-15.3956213100042));
#57124=CARTESIAN_POINT('Ctrl Pts',(7.21919473296188,28.1985882983322,-15.2613017155268));
#57125=CARTESIAN_POINT('Ctrl Pts',(7.34305540407025,28.1157508742713,-15.1936020965576));
#57126=CARTESIAN_POINT('Ctrl Pts',(7.52374793236161,27.9827805317339,-15.0916317207699));
#57127=CARTESIAN_POINT('Ctrl Pts',(7.58312770045258,27.9370018403625,-15.0575719928629));
#57128=CARTESIAN_POINT('Ctrl Pts',(7.65628611371722,27.8779133193801,-15.0149561206365));
#57129=CARTESIAN_POINT('Ctrl Pts',(7.67087193525932,27.8659960500774,-15.0064264965047));
#57130=CARTESIAN_POINT('Ctrl Pts',(7.69988883952031,27.8420132357583,-14.989392534012));
#57131=CARTESIAN_POINT('Ctrl Pts',(7.74318619480258,27.8058137690161,-14.963877248045));
#57132=CARTESIAN_POINT('Ctrl Pts',(7.89944767767118,27.6706041349955,-14.8707339720428));
#57133=CARTESIAN_POINT('Ctrl Pts',(8.03404572312412,27.5402060694125,-14.7874203361386));
#57134=CARTESIAN_POINT('Ctrl Pts',(8.24008043953904,27.3217971781574,-14.6565549244909));
#57135=CARTESIAN_POINT('Ctrl Pts',(8.33843721101683,27.2077082196918,-14.5923386141809));
#57136=CARTESIAN_POINT('Ctrl Pts',(8.47893005098055,27.0288386736179,-14.4984704418604));
#57137=CARTESIAN_POINT('Ctrl Pts',(8.52458497644703,26.9679233156009,-14.4675917513094));
#57138=CARTESIAN_POINT('Ctrl Pts',(8.59127443651523,26.874532439389,-14.4219830489157));
#57139=CARTESIAN_POINT('Ctrl Pts',(8.62417068589193,26.827332220894,-14.3993562003764));
#57140=CARTESIAN_POINT('Ctrl Pts',(8.65638641071583,26.77935680123,-14.3770147803195));
#57141=CARTESIAN_POINT('Ctrl Pts',(8.67771128879629,26.7471986843312,-14.3621861888618));
#57142=CARTESIAN_POINT('Ctrl Pts',(8.68830265601785,26.7310244203614,-14.3548011832054));
#57143=CARTESIAN_POINT('Ctrl Pts',(8.78274530658054,26.5849561141366,-14.2887748070903));
#57144=CARTESIAN_POINT('Ctrl Pts',(8.86068739391458,26.451236520966,-14.2330361409186));
#57145=CARTESIAN_POINT('Ctrl Pts',(9.00450920734481,26.1756727304695,-14.1284366214839));
#57146=CARTESIAN_POINT('Ctrl Pts',(9.07039068412542,26.0338301335152,-14.0795735600124));
#57147=CARTESIAN_POINT('Ctrl Pts',(9.15981295337757,25.8144909048872,-14.0123396480294));
#57148=CARTESIAN_POINT('Ctrl Pts',(9.18805026088068,25.7402795991016,-13.9909404624635));
#57149=CARTESIAN_POINT('Ctrl Pts',(9.22797174914896,25.6272308447628,-13.9604942443429));
#57150=CARTESIAN_POINT('Ctrl Pts',(9.24087290416293,25.5892591123023,-13.9506210958618));
#57151=CARTESIAN_POINT('Ctrl Pts',(9.25960317580872,25.5318559702848,-13.9362431667154));
#57152=CARTESIAN_POINT('Ctrl Pts',(9.26574746248233,25.5126328195426,-13.9315190639132));
#57153=CARTESIAN_POINT('Ctrl Pts',(9.27779745460633,25.4741297112776,-13.9222404425594));
#57154=CARTESIAN_POINT('Ctrl Pts',(9.33095684496213,25.3005840318675,-13.8812425302914));
#57155=CARTESIAN_POINT('Ctrl Pts',(9.37458706885838,25.1245081402695,-13.8470876782007));
#57156=CARTESIAN_POINT('Ctrl Pts',(9.43702932022959,24.8073779416153,-13.7979107470922));
#57157=CARTESIAN_POINT('Ctrl Pts',(9.4606902410544,24.6467599064343,-13.7790931247428));
#57158=CARTESIAN_POINT('Ctrl Pts',(9.48443586383693,24.4025985970691,-13.7601683668309));
#57159=CARTESIAN_POINT('Ctrl Pts',(9.49038965464922,24.3206716651867,-13.7554114608306));
#57160=CARTESIAN_POINT('Ctrl Pts',(9.49530693739123,24.2175656283315,-13.7514807390208));
#57161=CARTESIAN_POINT('Ctrl Pts',(9.49616405833992,24.196909533951,-13.7507953914246));
#57162=CARTESIAN_POINT('Ctrl Pts',(9.4976234388156,24.1555269308167,-13.7496283039473));
#57163=CARTESIAN_POINT('Ctrl Pts',(9.49822591174895,24.134783546786,-13.7491463933653));
#57164=CARTESIAN_POINT('Ctrl Pts',(9.4996434096454,24.0726722356942,-13.7480124558415));
#57165=CARTESIAN_POINT('Ctrl Pts',(9.50007135421376,24.0313686878477,-13.7476699921584));
#57166=CARTESIAN_POINT('Ctrl Pts',(9.4996662443851,23.8253629087153,-13.7479941330758));
#57167=CARTESIAN_POINT('Ctrl Pts',(9.49121911949272,23.6621935801189,-13.7547654157194));
#57168=CARTESIAN_POINT('Ctrl Pts',(9.4587721863421,23.338970590622,-13.7806183021659));
#57169=CARTESIAN_POINT('Ctrl Pts',(9.43477056821329,23.1789172141967,-13.7997005349618));
#57170=CARTESIAN_POINT('Ctrl Pts',(9.38725771360426,22.9411107629561,-13.837102628237));
#57171=CARTESIAN_POINT('Ctrl Pts',(9.36949809616687,22.8622214000734,-13.8510338887471));
#57172=CARTESIAN_POINT('Ctrl Pts',(9.33996284664004,22.7444532641515,-13.8740766634445));
#57173=CARTESIAN_POINT('Ctrl Pts',(9.32963490023978,22.7052915694536,-13.8821152835491));
#57174=CARTESIAN_POINT('Ctrl Pts',(9.31341500812318,22.6466904430213,-13.8947039518392));
#57175=CARTESIAN_POINT('Ctrl Pts',(9.30788663841741,22.6271794837453,-13.8989889326369));
#57176=CARTESIAN_POINT('Ctrl Pts',(9.29660876340497,22.5882796068097,-13.9077176220116));
#57177=CARTESIAN_POINT('Ctrl Pts',(9.29085668943634,22.5688812453494,-13.9121633262109));
#57178=CARTESIAN_POINT('Ctrl Pts',(9.27326264463063,22.5108396460112,-13.9257410693577));
#57179=CARTESIAN_POINT('Ctrl Pts',(9.26110733127937,22.4724312394044,-13.9350948377905));
#57180=CARTESIAN_POINT('Ctrl Pts',(9.2359836490324,22.396233117187,-13.9543649402863));
#57181=CARTESIAN_POINT('Ctrl Pts',(9.197068435466,22.2828327167101,-13.9841216702419));
#57182=CARTESIAN_POINT('Ctrl Pts',(9.15454267066618,22.1720448817502,-14.0163206782906));
#57183=CARTESIAN_POINT('Ctrl Pts',(9.06483682491421,21.9537804830714,-14.0837069534237));
#57184=CARTESIAN_POINT('Ctrl Pts',(8.99884082066844,21.8126764667367,-14.1326074671));
#57185=CARTESIAN_POINT('Ctrl Pts',(8.85494723107187,21.5386207964925,-14.2371585789696));
#57186=CARTESIAN_POINT('Ctrl Pts',(8.77704782875675,21.405670813631,-14.2928114145769));
#57187=CARTESIAN_POINT('Ctrl Pts',(8.6722724453834,21.2443471245385,-14.3659925148));
#57188=CARTESIAN_POINT('Ctrl Pts',(8.65094634731038,21.2123262139482,-14.3808099693033));
#57189=CARTESIAN_POINT('Ctrl Pts',(8.61839852912271,21.1646580921797,-14.4032980035455));
#57190=CARTESIAN_POINT('Ctrl Pts',(8.59649962691598,21.132980772232,-14.418386962775));
#57191=CARTESIAN_POINT('Ctrl Pts',(8.52993454319089,21.0390293942814,-14.4639952925715));
#57192=CARTESIAN_POINT('Ctrl Pts',(8.47266948695129,20.9629552569587,-14.5026850770815));
#57193=CARTESIAN_POINT('Ctrl Pts',(8.33186317621717,20.7844442014006,-14.5966605629362));
#57194=CARTESIAN_POINT('Ctrl Pts',(8.23350761084378,20.6708469934847,-14.6607986501892));
#57195=CARTESIAN_POINT('Ctrl Pts',(8.02798664018915,20.4537838351751,-14.7911955493999));
#57196=CARTESIAN_POINT('Ctrl Pts',(7.92082023511189,20.3503201317579,-14.8574563737388));
#57197=CARTESIAN_POINT('Ctrl Pts',(7.69756024180074,20.1532113754902,-14.9914043212885));
#57198=CARTESIAN_POINT('Ctrl Pts',(7.58146698708323,20.0595668291864,-15.0590928014651));
#57199=CARTESIAN_POINT('Ctrl Pts',(7.43053348243285,19.9486574100401,-15.1442265889065));
#57200=CARTESIAN_POINT('Ctrl Pts',(7.40005526334361,19.9267836397779,-15.1612797131196));
#57201=CARTESIAN_POINT('Ctrl Pts',(7.35389412278319,19.8944377549658,-15.1868925868012));
#57202=CARTESIAN_POINT('Ctrl Pts',(7.33842746673253,19.8837295297804,-15.1954388107376));
#57203=CARTESIAN_POINT('Ctrl Pts',(7.30740967665893,19.8625123594981,-15.2125058309299));
#57204=CARTESIAN_POINT('Ctrl Pts',(7.22961967073317,19.8099434141611,-15.2551289862951));
#57205=CARTESIAN_POINT('Ctrl Pts',(7.15060295917947,19.7597291386256,-15.2975172041686));
#57206=CARTESIAN_POINT('Ctrl Pts',(6.95859784236151,19.643663379666,-15.398706660168));
#57207=CARTESIAN_POINT('Ctrl Pts',(6.82744572738336,19.5722063013797,-15.4654418783362));
#57208=CARTESIAN_POINT('Ctrl Pts',(6.55867899441322,19.4410306593027,-15.5970216671956));
#57209=CARTESIAN_POINT('Ctrl Pts',(6.42106479588649,19.3813120766787,-15.661867088802));
#57210=CARTESIAN_POINT('Ctrl Pts',(6.20955760065134,19.3007335858868,-15.7574134301996));
#57211=CARTESIAN_POINT('Ctrl Pts',(6.10253067277946,19.2626984080434,-15.8047564438638));
#57212=CARTESIAN_POINT('Ctrl Pts',(5.97536382738032,19.2223584409551,-15.8591722850903));
#57213=CARTESIAN_POINT('Ctrl Pts',(5.92036101970489,19.2059472624311,-15.8823112157504));
#57214=CARTESIAN_POINT('Ctrl Pts',(5.88357966585399,19.1952029819019,-15.8976959200338));
#57215=CARTESIAN_POINT('Ctrl Pts',(5.86512256314497,19.1899263506937,-15.9053717649071));
#57216=CARTESIAN_POINT('Ctrl Pts',(5.69882430287088,19.1434188736361,-15.9741299312613));
#57217=CARTESIAN_POINT('Ctrl Pts',(5.39999274864541,19.074492569445,-16.0919981634691));
#57218=CARTESIAN_POINT('Ctrl Pts',(5.09467072163286,19.0330721579535,-16.2008146577535));
#57219=CARTESIAN_POINT('Ctrl Pts',(4.78600084505622,19.0057824464796,-16.3049424979477));
#57220=CARTESIAN_POINT('Ctrl Pts',(4.62999231317816,18.9992009497136,-16.3546623504514));
#57221=CARTESIAN_POINT('Ctrl Pts',(4.43279168890305,19.0002961473357,-16.4137722265256));
#57222=CARTESIAN_POINT('Ctrl Pts',(4.39324191842869,19.0009823911873,-16.4254421625891));
#57223=CARTESIAN_POINT('Ctrl Pts',(4.33375048997517,19.0027252741403,-16.442716809202));
#57224=CARTESIAN_POINT('Ctrl Pts',(4.29400704792877,19.004126493904,-16.45416404485));
#57225=CARTESIAN_POINT('Ctrl Pts',(4.17492350751609,19.0097483902536,-16.4879062795999));
#57226=CARTESIAN_POINT('Ctrl Pts',(4.07599373020815,19.0173787327952,-16.5147842062619));
#57227=CARTESIAN_POINT('Ctrl Pts',(3.83915890730805,19.0413234540751,-16.576965626304));
#57228=CARTESIAN_POINT('Ctrl Pts',(3.68206240407646,19.0647839505093,-16.6153200819377));
#57229=CARTESIAN_POINT('Ctrl Pts',(3.36955057108897,19.1268630786063,-16.6861010074616));
#57230=CARTESIAN_POINT('Ctrl Pts',(3.21413490427825,19.1654805263442,-16.7185270353234));
#57231=CARTESIAN_POINT('Ctrl Pts',(2.98239736299467,19.2351926447607,-16.7629034595391));
#57232=CARTESIAN_POINT('Ctrl Pts',(2.90538310626411,19.2603975176526,-16.7769850004889));
#57233=CARTESIAN_POINT('Ctrl Pts',(2.8094228570208,19.2944327021957,-16.7937169440387));
#57234=CARTESIAN_POINT('Ctrl Pts',(2.7710695434467,19.3082998337379,-16.8003227201479));
#57235=CARTESIAN_POINT('Ctrl Pts',(2.73277863773367,19.3226775130946,-16.8067553480941));
#57236=CARTESIAN_POINT('Ctrl Pts',(2.67556054843687,19.344563538547,-16.8162472115744));
#57237=CARTESIAN_POINT('Ctrl Pts',(2.63764917640111,19.3596003724586,-16.8223756344838));
#57238=CARTESIAN_POINT('Ctrl Pts',(2.44925570337053,19.4369969838961,-16.8520532630584));
#57239=CARTESIAN_POINT('Ctrl Pts',(2.30225568162101,19.5059792674876,-16.8727129885635));
#57240=CARTESIAN_POINT('Ctrl Pts',(2.01564514479671,19.6578480696034,-16.908641038543));
#57241=CARTESIAN_POINT('Ctrl Pts',(1.87603458294445,19.740734767493,-16.9239080748372));
#57242=CARTESIAN_POINT('Ctrl Pts',(1.60436758268191,19.9205579138168,-16.9497428239691));
#57243=CARTESIAN_POINT('Ctrl Pts',(1.47231010770517,20.0174927724321,-16.9603095097621));
#57244=CARTESIAN_POINT('Ctrl Pts',(1.32821025370583,20.1347476282247,-16.9699182992239));
#57245=CARTESIAN_POINT('Ctrl Pts',(1.3122526256191,20.1478975984186,-16.9709547966923));
#57246=CARTESIAN_POINT('Ctrl Pts',(1.28055048950018,20.1743535076429,-16.9729602735448));
#57247=CARTESIAN_POINT('Ctrl Pts',(1.23329014449646,20.214292636092,-16.9758690827517));
#57248=CARTESIAN_POINT('Ctrl Pts',(1.12505457098844,20.3092604112095,-16.9819822090053));
#57249=CARTESIAN_POINT('Ctrl Pts',(1.03573996025468,20.3936740696511,-16.9861392336332));
#57250=CARTESIAN_POINT('Ctrl Pts',(0.861658081702048,20.5664587608291,-16.9931895344418));
#57251=CARTESIAN_POINT('Ctrl Pts',(0.751656022760932,20.6869158203573,-16.9962081940318));
#57252=CARTESIAN_POINT('Ctrl Pts',(0.543679601113993,20.9382785472121,-16.9997402754155));
#57253=CARTESIAN_POINT('Ctrl Pts',(0.445704806056031,21.0691838702689,-17.0002523791264));
#57254=CARTESIAN_POINT('Ctrl Pts',(0.307964555949979,21.2735394717123,-16.9997110755045));
#57255=CARTESIAN_POINT('Ctrl Pts',(0.263586336154467,21.3430007932556,-16.9993117133576));
#57256=CARTESIAN_POINT('Ctrl Pts',(0.177996277698543,21.4846214320167,-16.9981645073496));
#57257=CARTESIAN_POINT('Ctrl Pts',(0.137138960301268,21.5561932637163,-16.997421818723));
#57258=CARTESIAN_POINT('Ctrl Pts',(0.0202552462301792,21.7731461194819,
-16.9948346932133));
#57259=CARTESIAN_POINT('Ctrl Pts',(-0.0500966079618834,21.9207591671011,
-16.9926356455613));
#57260=CARTESIAN_POINT('Ctrl Pts',(-0.175972691707234,22.2218265075116,
-16.9879550338172));
#57261=CARTESIAN_POINT('Ctrl Pts',(-0.231496448747289,22.3752809718075,
-16.9854724072299));
#57262=CARTESIAN_POINT('Ctrl Pts',(-0.303568940988182,22.6098855908799,
-16.9819362864954));
#57263=CARTESIAN_POINT('Ctrl Pts',(-0.32572090828689,22.6888255880473,-16.9807879632478));
#57264=CARTESIAN_POINT('Ctrl Pts',(-0.356097812468616,22.808360712486,-16.9791534736861));
#57265=CARTESIAN_POINT('Ctrl Pts',(-0.370573166407556,22.8684096884495,
-16.9783581512183));
#57266=CARTESIAN_POINT('Ctrl Pts',(-0.383967695011297,22.9288852925971,
-16.9776029855594));
#57267=CARTESIAN_POINT('Ctrl Pts',(-0.392655725938007,22.9692977589163,
-16.9771092273512));
#57268=CARTESIAN_POINT('Ctrl Pts',(-0.396879263255509,22.9895540629632,
-16.9768671715761));
#57269=CARTESIAN_POINT('Ctrl Pts',(-0.433731147228075,23.1719555303405,
-16.9747394571526));
#57270=CARTESIAN_POINT('Ctrl Pts',(-0.458389000150122,23.3353476343703,
-16.9732077566867));
#57271=CARTESIAN_POINT('Ctrl Pts',(-0.4749371855331,23.5,-16.9721648040778));
#57272=CARTESIAN_POINT('',(-0.4749371855331,23.5,6.93889390390723E-15));
#57273=CARTESIAN_POINT('Origin',(33.,26.4545372843263,5.29429254368814));
#57274=CARTESIAN_POINT('Ctrl Pts',(16.0339928845406,26.2575775584219,4.83472006151403));
#57275=CARTESIAN_POINT('Ctrl Pts',(16.0482886954921,26.2396927012492,4.84238500383155));
#57276=CARTESIAN_POINT('Ctrl Pts',(16.0628693069814,26.2226807213726,4.85090739382797));
#57277=CARTESIAN_POINT('Ctrl Pts',(16.077753848377,26.2064867817649,4.86016013510863));
#57278=CARTESIAN_POINT('Ctrl Pts',(16.0870581940121,26.1963639296529,4.86594403537529));
#57279=CARTESIAN_POINT('Ctrl Pts',(16.0964813007413,26.1865604802237,4.87201444823721));
#57280=CARTESIAN_POINT('Ctrl Pts',(16.1060278410909,26.1770625127317,4.87835053916283));
#57281=CARTESIAN_POINT('Ctrl Pts',(16.1235862887443,26.159593402571,4.89000417668698));
#57282=CARTESIAN_POINT('Ctrl Pts',(16.1415613272045,26.1431606937632,4.90255192203326));
#57283=CARTESIAN_POINT('Ctrl Pts',(16.1599798307474,26.1277228536324,4.91588492234545));
#57284=CARTESIAN_POINT('Ctrl Pts',(16.1675955531722,26.1213395823205,4.92139787996607));
#57285=CARTESIAN_POINT('Ctrl Pts',(16.175287093708,26.1151264693412,4.92704572621618));
#57286=CARTESIAN_POINT('Ctrl Pts',(16.1830563521511,26.1090811176398,4.93282326850936));
#57287=CARTESIAN_POINT('Ctrl Pts',(16.1896961237522,26.1039146329825,4.93776087761618));
#57288=CARTESIAN_POINT('Ctrl Pts',(16.1964043280784,26.0988626434749,4.94280180897596));
#57289=CARTESIAN_POINT('Ctrl Pts',(16.2031398739707,26.0939549260933,4.94791072700146));
#57290=CARTESIAN_POINT('Ctrl Pts',(16.209875419863,26.0890472087118,4.95301964502696));
#57291=CARTESIAN_POINT('Ctrl Pts',(16.2166324893586,26.0842872989932,4.95819191194151));
#57292=CARTESIAN_POINT('Ctrl Pts',(16.2234120418664,26.0796699800677,4.9634232277976));
#57293=CARTESIAN_POINT('Ctrl Pts',(16.236971146882,26.0704353422166,4.97388585950979));
#57294=CARTESIAN_POINT('Ctrl Pts',(16.2506201839462,26.0617705217472,4.98458418684746));
#57295=CARTESIAN_POINT('Ctrl Pts',(16.2643659505407,26.0536422887736,4.99548959433719));
#57296=CARTESIAN_POINT('Ctrl Pts',(16.2852187040666,26.041311507683,5.01203343515676));
#57297=CARTESIAN_POINT('Ctrl Pts',(16.3062940068527,26.0302132424319,5.02905416908863));
#57298=CARTESIAN_POINT('Ctrl Pts',(16.3276138236464,26.0202722072282,5.04647437887169));
#57299=CARTESIAN_POINT('Ctrl Pts',(16.3344012997453,26.0171073329943,5.05202035793349));
#57300=CARTESIAN_POINT('Ctrl Pts',(16.3412135588188,26.0140599452802,5.05760717962358));
#57301=CARTESIAN_POINT('Ctrl Pts',(16.3480513096296,26.0111282125913,5.06323325453684));
#57302=CARTESIAN_POINT('Ctrl Pts',(16.3716350535321,26.0010165201885,5.08263786777905));
#57303=CARTESIAN_POINT('Ctrl Pts',(16.3955215054915,25.992278737261,5.10250485728671));
#57304=CARTESIAN_POINT('Ctrl Pts',(16.419743160732,25.9848775660295,5.1227706820804));
#57305=CARTESIAN_POINT('Ctrl Pts',(16.4246028876691,25.9833926274139,5.12683672850353));
#57306=CARTESIAN_POINT('Ctrl Pts',(16.4294761080983,25.9819616241679,5.13091893625157));
#57307=CARTESIAN_POINT('Ctrl Pts',(16.4343630844679,25.980584459025,5.13501693542079));
#57308=CARTESIAN_POINT('Ctrl Pts',(16.4416741962513,25.9785241649818,5.141147705809));
#57309=CARTESIAN_POINT('Ctrl Pts',(16.4490048161393,25.9765878758654,5.14730420709631));
#57310=CARTESIAN_POINT('Ctrl Pts',(16.4563305291426,25.9747798143556,5.15346367588301));
#57311=CARTESIAN_POINT('Ctrl Pts',(16.4636562421459,25.9729717528457,5.15962314466971));
#57312=CARTESIAN_POINT('Ctrl Pts',(16.4709846055243,25.9712897602985,5.1657919159592));
#57313=CARTESIAN_POINT('Ctrl Pts',(16.478316560937,25.9697312787863,5.17196864172131));
#57314=CARTESIAN_POINT('Ctrl Pts',(16.4929804717623,25.9666143157621,5.18432209324552));
#57315=CARTESIAN_POINT('Ctrl Pts',(16.5076587507244,25.9639910105231,5.19670725815659));
#57316=CARTESIAN_POINT('Ctrl Pts',(16.5223584328467,25.9618460415304,5.20911426434256));
#57317=CARTESIAN_POINT('Ctrl Pts',(16.5479617237647,25.9581100243382,5.23072426829765));
#57318=CARTESIAN_POINT('Ctrl Pts',(16.5736298479289,25.9558224013621,5.25240059770458));
#57319=CARTESIAN_POINT('Ctrl Pts',(16.5993986719124,25.954945341985,5.27409622848867));
#57320=CARTESIAN_POINT('Ctrl Pts',(16.6032192880079,25.9548153047285,5.277312932372));
#57321=CARTESIAN_POINT('Ctrl Pts',(16.6070421177399,25.9547163648842,5.28053008665054));
#57322=CARTESIAN_POINT('Ctrl Pts',(16.6108672780061,25.9546484933932,5.2837475591227));
#57323=CARTESIAN_POINT('Ctrl Pts',(16.6256795946141,25.9543856719837,5.29620670269277));
#57324=CARTESIAN_POINT('Ctrl Pts',(16.6405268572356,25.9545883150099,5.30867030528035));
#57325=CARTESIAN_POINT('Ctrl Pts',(16.6554162650306,25.9552580516208,5.3211299762963));
#57326=CARTESIAN_POINT('Ctrl Pts',(16.6628609689281,25.9555929199262,5.32735981180427));
#57327=CARTESIAN_POINT('Ctrl Pts',(16.670316209119,25.9560446440895,5.33358865896399));
#57328=CARTESIAN_POINT('Ctrl Pts',(16.6777829536176,25.9566139320155,5.33981545246558));
#57329=CARTESIAN_POINT('Ctrl Pts',(16.681516325867,25.9568985759785,5.34292884921637));
#57330=CARTESIAN_POINT('Ctrl Pts',(16.6852525741933,25.9572126162338,5.34604173240083));
#57331=CARTESIAN_POINT('Ctrl Pts',(16.6889918234758,25.9575561736078,5.34915396537015));
#57332=CARTESIAN_POINT('Ctrl Pts',(16.690861448117,25.9577279522947,5.35071008185481));
#57333=CARTESIAN_POINT('Ctrl Pts',(16.6927318229973,25.9579071106011,5.35226603574635));
#57334=CARTESIAN_POINT('Ctrl Pts',(16.6946029640567,25.958093665698,5.35382180979552));
#57335=CARTESIAN_POINT('Ctrl Pts',(16.6955385345864,25.9581869432465,5.3545996968201));
#57336=CARTESIAN_POINT('Ctrl Pts',(16.6964618802871,25.9582808193014,5.35536728062135));
#57337=CARTESIAN_POINT('Ctrl Pts',(16.6973887994847,25.9583768342247,5.35613757384417));
#57338=CARTESIAN_POINT('Ctrl Pts',(16.6983157186823,25.9584728491481,5.35690786706699));
#57339=CARTESIAN_POINT('Ctrl Pts',(16.6992426416197,25.9585706572376,5.35767793144793));
#57340=CARTESIAN_POINT('Ctrl Pts',(16.7001695682977,25.9586702584785,5.3584477669892));
#57341=CARTESIAN_POINT('Ctrl Pts',(0.321034048597817,44.2777095070773,-16.496876587392));
#57342=CARTESIAN_POINT('Ctrl Pts',(0.334078182671872,44.0705712895835,-16.4966227447236));
#57343=CARTESIAN_POINT('Ctrl Pts',(0.346147593727982,43.9243235322772,-16.6433959637249));
#57344=CARTESIAN_POINT('Ctrl Pts',(0.307535768851996,44.2768333852379,-16.497139267868));
#57345=CARTESIAN_POINT('Ctrl Pts',(0.32115157242211,44.0697030498192,-16.4968849768605));
#57346=CARTESIAN_POINT('Ctrl Pts',(0.333504576783726,43.9234749343164,-16.6436941271133));
#57347=CARTESIAN_POINT('Ctrl Pts',(0.294017346932686,44.2758981934479,-16.4973857263738));
#57348=CARTESIAN_POINT('Ctrl Pts',(0.308206040614918,44.0687776043361,-16.4971323872042));
#57349=CARTESIAN_POINT('Ctrl Pts',(0.320842694094729,43.9225707071434,-16.6439790196373));
#57350=CARTESIAN_POINT('Ctrl Pts',(0.267039396841221,44.27391662747,-16.4978444642199));
#57351=CARTESIAN_POINT('Ctrl Pts',(0.282371646107752,44.0668191614445,-16.4975958245399));
#57352=CARTESIAN_POINT('Ctrl Pts',(0.295574090707277,43.9206577286911,-16.6445202461941));
#57353=CARTESIAN_POINT('Ctrl Pts',(0.253563318677811,44.2728691821441,-16.4980570656251));
#57354=CARTESIAN_POINT('Ctrl Pts',(0.269466916331725,44.0657850965016,-16.4978121729084));
#57355=CARTESIAN_POINT('Ctrl Pts',(0.282951868731823,43.9196479380401,-16.644776944703));
#57356=CARTESIAN_POINT('Ctrl Pts',(0.213173600931101,44.2695576149692,-16.4986448596443));
#57357=CARTESIAN_POINT('Ctrl Pts',(0.230789208343801,44.0625190499157,-16.4984153937458));
#57358=CARTESIAN_POINT('Ctrl Pts',(0.245121279113449,43.9164593690092,-16.6455055488628));
#57359=CARTESIAN_POINT('Ctrl Pts',(0.186298475258698,44.2671242747577,-16.4989700430965));
#57360=CARTESIAN_POINT('Ctrl Pts',(0.205054254630706,44.0601233301731,-16.4987564104361));
#57361=CARTESIAN_POINT('Ctrl Pts',(0.219948985085661,43.9141214063132,-16.6459359637993));
#57362=CARTESIAN_POINT('Ctrl Pts',(0.105825878010724,44.2591529071548,-16.4997478557418));
#57363=CARTESIAN_POINT('Ctrl Pts',(0.127994124910921,44.0522861114256,-16.4995982912245));
#57364=CARTESIAN_POINT('Ctrl Pts',(0.144575202554741,43.906475946942,-16.6470632548686));
#57365=CARTESIAN_POINT('Ctrl Pts',(0.0523811410166356,44.2529437369118,
-16.5000027615431));
#57366=CARTESIAN_POINT('Ctrl Pts',(0.0768198248561238,44.0461951243862,
-16.4999178604957));
#57367=CARTESIAN_POINT('Ctrl Pts',(0.0945167711882191,43.9005370741829,
-16.6475961824246));
#57368=CARTESIAN_POINT('Ctrl Pts',(-0.107350614477069,44.2316680864431,
-16.4999944092424));
#57369=CARTESIAN_POINT('Ctrl Pts',(-0.0761321294294826,44.0253574854767,
-16.5001684527276));
#57370=CARTESIAN_POINT('Ctrl Pts',(-0.0550942394312359,43.8802288896034,
-16.6485550431313));
#57371=CARTESIAN_POINT('Ctrl Pts',(-0.213035833808924,44.2139564350666,
-16.4989582457926));
#57372=CARTESIAN_POINT('Ctrl Pts',(-0.177314759062477,44.0080500010336,
-16.4993908078766));
#57373=CARTESIAN_POINT('Ctrl Pts',(-0.154083150146027,43.8633708391614,
-16.6483410814393));
#57374=CARTESIAN_POINT('Ctrl Pts',(-0.422829790157967,44.1715971665048,
-16.4949150477184));
#57375=CARTESIAN_POINT('Ctrl Pts',(-0.378133313017958,43.9667246375007,
-16.4960324415121));
#57376=CARTESIAN_POINT('Ctrl Pts',(-0.350584376434533,43.8231263425323,
-16.6462901344215));
#57377=CARTESIAN_POINT('Ctrl Pts',(-0.526938468414131,44.1469492910955,
-16.491907937397));
#57378=CARTESIAN_POINT('Ctrl Pts',(-0.477778440005314,43.9427009960084,
-16.4934505609926));
#57379=CARTESIAN_POINT('Ctrl Pts',(-0.448096637091592,43.7997396541264,
-16.6444530862772));
#57380=CARTESIAN_POINT('Ctrl Pts',(-0.733587594662706,44.0907445802113,
-16.4840086388606));
#57381=CARTESIAN_POINT('Ctrl Pts',(-0.675522285528619,43.8879685573675,
-16.4865649802999));
#57382=CARTESIAN_POINT('Ctrl Pts',(-0.641652292512058,43.7464596423238,
-16.6392391144044));
#57383=CARTESIAN_POINT('Ctrl Pts',(-0.836128020523552,44.0591876523663,
-16.4791163820797));
#57384=CARTESIAN_POINT('Ctrl Pts',(-0.773630842788747,43.85725253155,-16.4822597770412));
#57385=CARTESIAN_POINT('Ctrl Pts',(-0.737695666593328,43.7165662342863,
-16.6358621269656));
#57386=CARTESIAN_POINT('Ctrl Pts',(-0.988754343263762,44.0066257334661,
-16.4704268781621));
#57387=CARTESIAN_POINT('Ctrl Pts',(-0.919592667679679,43.8061296100387,
-16.4745719708769));
#57388=CARTESIAN_POINT('Ctrl Pts',(-0.880651450997229,43.6668004399974,
-16.62970542955));
#57389=CARTESIAN_POINT('Ctrl Pts',(-1.03943225076959,43.988233336078,-16.4673051794513));
#57390=CARTESIAN_POINT('Ctrl Pts',(-0.968061533919264,43.7882402439072,
-16.471803341561));
#57391=CARTESIAN_POINT('Ctrl Pts',(-0.92811836158864,43.6493902559039,-16.6274713470767));
#57392=CARTESIAN_POINT('Ctrl Pts',(-1.11515046567206,43.9593254565497,-16.462292648905));
#57393=CARTESIAN_POINT('Ctrl Pts',(-1.04046157511159,43.760131242437,-16.4673503544702));
#57394=CARTESIAN_POINT('Ctrl Pts',(-0.999039003666644,43.6220311175392,
-16.6238556629229));
#57395=CARTESIAN_POINT('Ctrl Pts',(-1.14034008702055,43.9494695740836,-16.4605668083992));
#57396=CARTESIAN_POINT('Ctrl Pts',(-1.06454821112494,43.7505474186053,-16.4658157518771));
#57397=CARTESIAN_POINT('Ctrl Pts',(-1.02263258838498,43.6127040541935,-16.6226063432779));
#57398=CARTESIAN_POINT('Ctrl Pts',(-1.19061925892548,43.9293155100069,-16.4570064394505));
#57399=CARTESIAN_POINT('Ctrl Pts',(-1.11262228707775,43.7309512076575,-16.4626476168865));
#57400=CARTESIAN_POINT('Ctrl Pts',(-1.06972602765263,43.5936328230074,-16.6200209173139));
#57401=CARTESIAN_POINT('Ctrl Pts',(-1.21573107838862,43.9190077883623,-16.4551701883059));
#57402=CARTESIAN_POINT('Ctrl Pts',(-1.13663118653057,43.7209293797071,-16.4610125155677));
#57403=CARTESIAN_POINT('Ctrl Pts',(-1.09324674012034,43.5838796294641,-16.618683550189));
#57404=CARTESIAN_POINT('Ctrl Pts',(-1.3406740926079,43.8665114056024,-16.4457484072491));
#57405=CARTESIAN_POINT('Ctrl Pts',(-1.25611592982861,43.6698761529651,-16.4526150324278));
#57406=CARTESIAN_POINT('Ctrl Pts',(-1.21027325465697,43.5342106859547,-16.6118037002477));
#57407=CARTESIAN_POINT('Ctrl Pts',(-1.43874378672612,43.8214268381111,-16.4374378027854));
#57408=CARTESIAN_POINT('Ctrl Pts',(-1.34984750421121,43.6260493224596,-16.445193094768));
#57409=CARTESIAN_POINT('Ctrl Pts',(-1.3021291667423,43.4915646194171,-16.6056797596469));
#57410=CARTESIAN_POINT('Ctrl Pts',(-1.72749788443196,43.6771991720061,-16.4104580032492));
#57411=CARTESIAN_POINT('Ctrl Pts',(-1.62585456299005,43.4858144841423,-16.4210581992283));
#57412=CARTESIAN_POINT('Ctrl Pts',(-1.5725875499331,43.3551562723534,-16.5857017103286));
#57413=CARTESIAN_POINT('Ctrl Pts',(-1.9127446936616,43.5691113883,-16.3897439917078));
#57414=CARTESIAN_POINT('Ctrl Pts',(-1.80274205830027,43.3807393221566,-16.4024878858354));
#57415=CARTESIAN_POINT('Ctrl Pts',(-1.74609695837727,43.2529516481594,-16.5702431598975));
#57416=CARTESIAN_POINT('Ctrl Pts',(-2.1801557392676,43.3896071926388,-16.3555799666888));
#57417=CARTESIAN_POINT('Ctrl Pts',(-2.05760446502451,43.2064579036073,-16.3718931324892));
#57418=CARTESIAN_POINT('Ctrl Pts',(-1.99656460420932,43.0832067018407,-16.5448031114995));
#57419=CARTESIAN_POINT('Ctrl Pts',(-2.26754491058278,43.3268692367125,-16.3436754924434));
#57420=CARTESIAN_POINT('Ctrl Pts',(-2.14090553035905,43.1454987345458,-16.3612235417513));
#57421=CARTESIAN_POINT('Ctrl Pts',(-2.07841672068826,43.0238779812105,-16.5359471304104));
#57422=CARTESIAN_POINT('Ctrl Pts',(-2.39602241125449,43.2284104250473,-16.3251630538784));
#57423=CARTESIAN_POINT('Ctrl Pts',(-2.26324112913542,43.0498815519994,-16.3446457798798));
#57424=CARTESIAN_POINT('Ctrl Pts',(-2.19875377361068,42.9307615436581,-16.5222160833336));
#57425=CARTESIAN_POINT('Ctrl Pts',(-2.4384136297981,43.1948651021794,-16.3188829280199));
#57426=CARTESIAN_POINT('Ctrl Pts',(-2.30360778271325,43.0172911666837,-16.3390206470251));
#57427=CARTESIAN_POINT('Ctrl Pts',(-2.23845904720143,42.8990351188427,-16.5175645484453));
#57428=CARTESIAN_POINT('Ctrl Pts',(-2.5013483955168,43.1434553651894,-16.3093134885055));
#57429=CARTESIAN_POINT('Ctrl Pts',(-2.36350239470388,42.9673565647272,-16.3304535133341));
#57430=CARTESIAN_POINT('Ctrl Pts',(-2.29740621067309,42.8504103436033,-16.5104900878419));
#57431=CARTESIAN_POINT('Ctrl Pts',(-2.52221795974619,43.1261368034609,-16.3060987995381));
#57432=CARTESIAN_POINT('Ctrl Pts',(-2.38336413494237,42.9505314385688,-16.3275753119188));
#57433=CARTESIAN_POINT('Ctrl Pts',(-2.31695346092089,42.8340295394261,-16.508115741492));
#57434=CARTESIAN_POINT('Ctrl Pts',(-2.56373951624231,43.0911348998851,-16.2996221180008));
#57435=CARTESIAN_POINT('Ctrl Pts',(-2.42287279694903,42.9165270650644,-16.321777494731));
#57436=CARTESIAN_POINT('Ctrl Pts',(-2.3558441749912,42.8009219471062,-16.5033371082496));
#57437=CARTESIAN_POINT('Ctrl Pts',(-2.58440772848289,43.0734372910358,-16.2963575090795));
#57438=CARTESIAN_POINT('Ctrl Pts',(-2.44253529767474,42.8993336069646,-16.3188554855158));
#57439=CARTESIAN_POINT('Ctrl Pts',(-2.37520283114705,42.7841816631336,-16.5009308965196));
#57440=CARTESIAN_POINT('Ctrl Pts',(-2.76898876271576,42.9129091805958,-16.2668469274607));
#57441=CARTESIAN_POINT('Ctrl Pts',(-2.61835540789446,42.7431513199272,-16.2924080344925));
#57442=CARTESIAN_POINT('Ctrl Pts',(-2.54808864778449,42.6323323225514,-16.4792048254679));
#57443=CARTESIAN_POINT('Ctrl Pts',(-2.92301708649477,42.7613001461326,-16.2396947338131));
#57444=CARTESIAN_POINT('Ctrl Pts',(-2.76462847126197,42.5957682985728,-16.2681310777436));
#57445=CARTESIAN_POINT('Ctrl Pts',(-2.69235760204375,42.488886199182,-16.4593927479317));
#57446=CARTESIAN_POINT('Ctrl Pts',(-3.21259129366432,42.4414613853005,-16.1848994780706));
#57447=CARTESIAN_POINT('Ctrl Pts',(-3.03897378350019,42.2850128986459,-16.2192940222789));
#57448=CARTESIAN_POINT('Ctrl Pts',(-2.96358413143859,42.1861517320565,-16.4200413247235));
#57449=CARTESIAN_POINT('Ctrl Pts',(-3.34812899112022,42.2732247223232,-16.1572537757578));
#57450=CARTESIAN_POINT('Ctrl Pts',(-3.16707816112672,42.1214334676319,-16.1947098049125));
#57451=CARTESIAN_POINT('Ctrl Pts',(-3.09053404151204,42.0268568930642,-16.4004996968118));
#57452=CARTESIAN_POINT('Ctrl Pts',(-3.53828868842179,42.0088979382797,-16.1162873356813));
#57453=CARTESIAN_POINT('Ctrl Pts',(-3.34597462567252,41.8649168770618,-16.1584948890192));
#57454=CARTESIAN_POINT('Ctrl Pts',(-3.26864505239508,41.7764635010048,-16.3722252421456));
#57455=CARTESIAN_POINT('Ctrl Pts',(-3.5994799346103,41.9187901440346,-16.1027143504919));
#57456=CARTESIAN_POINT('Ctrl Pts',(-3.40351260983138,41.7773425460961,-16.1465055224545));
#57457=CARTESIAN_POINT('Ctrl Pts',(-3.32595916749315,41.6910871652366,-16.362972412406));
#57458=CARTESIAN_POINT('Ctrl Pts',(-3.67327289887432,41.8036856256223,-16.0859347036074));
#57459=CARTESIAN_POINT('Ctrl Pts',(-3.47268299468521,41.6656131275086,-16.1317391824527));
#57460=CARTESIAN_POINT('Ctrl Pts',(-3.3950765443778,41.5820004939642,-16.3517021387782));
#57461=CARTESIAN_POINT('Ctrl Pts',(-3.68790324489889,41.7805305132082,-16.0825865601582));
#57462=CARTESIAN_POINT('Ctrl Pts',(-3.48640397870713,41.6431129782816,-16.1287915877042));
#57463=CARTESIAN_POINT('Ctrl Pts',(-3.40877989888389,41.5600546868429,-16.3494618416137));
#57464=CARTESIAN_POINT('Ctrl Pts',(-3.71686467531462,41.7340227710879,-16.0759179456141));
#57465=CARTESIAN_POINT('Ctrl Pts',(-3.51355022417322,41.5979213056804,-16.122924842068));
#57466=CARTESIAN_POINT('Ctrl Pts',(-3.43590630737669,41.5159732371528,-16.3450174403968));
#57467=CARTESIAN_POINT('Ctrl Pts',(-3.73118318182571,41.7106906886745,-16.0726003938663));
#57468=CARTESIAN_POINT('Ctrl Pts',(-3.52696370022908,41.5752492629553,-16.1200082324879));
#57469=CARTESIAN_POINT('Ctrl Pts',(-3.44931758085173,41.493857071485,-16.3428152733996));
#57470=CARTESIAN_POINT('Ctrl Pts',(-3.77365910783509,41.6404628298273,-16.0627003448006));
#57471=CARTESIAN_POINT('Ctrl Pts',(-3.56674649451528,41.5069837011863,-16.1113077604514));
#57472=CARTESIAN_POINT('Ctrl Pts',(-3.48910219450987,41.427285026544,-16.3362710369363));
#57473=CARTESIAN_POINT('Ctrl Pts',(-3.80133703055952,41.5933354841588,-16.0561704793561));
#57474=CARTESIAN_POINT('Ctrl Pts',(-3.59262873818026,41.4611883744804,-16.105579589636));
#57475=CARTESIAN_POINT('Ctrl Pts',(-3.51502641995466,41.3826056395206,-16.3319912551902));
#57476=CARTESIAN_POINT('Ctrl Pts',(-3.93661737229858,41.3561924516797,-16.0239016028219));
#57477=CARTESIAN_POINT('Ctrl Pts',(-3.71926534359318,41.2302267666986,-16.0772522172006));
#57478=CARTESIAN_POINT('Ctrl Pts',(-3.64173527925152,41.1577530499255,-16.3110349773682));
#57479=CARTESIAN_POINT('Ctrl Pts',(-4.03491747293985,41.1616690216634,-15.9993106710039));
#57480=CARTESIAN_POINT('Ctrl Pts',(-3.8105351856191,41.0410889990247,-16.0558581848326));
#57481=CARTESIAN_POINT('Ctrl Pts',(-3.73380699989436,40.9732232360452,-16.2956924811267));
#57482=CARTESIAN_POINT('Ctrl Pts',(-4.21346560575097,40.7637707951905,-15.9532193788555));
#57483=CARTESIAN_POINT('Ctrl Pts',(-3.97517918815052,40.6545075845859,-16.0161173849287));
#57484=CARTESIAN_POINT('Ctrl Pts',(-3.90104216471963,40.5955698374873,-16.2684493117706));
#57485=CARTESIAN_POINT('Ctrl Pts',(-4.29370773194948,40.5603934046897,-15.9317175178876));
#57486=CARTESIAN_POINT('Ctrl Pts',(-4.04850396862992,40.4567958249106,-15.9977704901831));
#57487=CARTESIAN_POINT('Ctrl Pts',(-3.97620007983221,40.4024438484038,-16.2565472800635));
#57488=CARTESIAN_POINT('Ctrl Pts',(-4.40146481480481,40.2490824569658,-15.9021537778166));
#57489=CARTESIAN_POINT('Ctrl Pts',(-4.14571728004939,40.1550827275247,-15.9729333571334));
#57490=CARTESIAN_POINT('Ctrl Pts',(-4.0771295784449,40.1066679258703,-16.2416226946648));
#57491=CARTESIAN_POINT('Ctrl Pts',(-4.43527916848801,40.1442697315678,-15.8927463879809));
#57492=CARTESIAN_POINT('Ctrl Pts',(-4.17607991924084,40.0532812588022,-15.965075967575));
#57493=CARTESIAN_POINT('Ctrl Pts',(-4.10880142516048,40.007059981848,-16.2371350135424));
#57494=CARTESIAN_POINT('Ctrl Pts',(-4.47498970331547,40.0119814226891,-15.8815784864466));
#57495=CARTESIAN_POINT('Ctrl Pts',(-4.21141132770978,39.9250565429304,-15.955847181276));
#57496=CARTESIAN_POINT('Ctrl Pts',(-4.14599586533176,39.8813077925278,-16.2321648104482));
#57497=CARTESIAN_POINT('Ctrl Pts',(-4.48280713505993,39.9854484820733,-15.8793735332333));
#57498=CARTESIAN_POINT('Ctrl Pts',(-4.21836394867178,39.8992957517518,-15.9540264515764));
#57499=CARTESIAN_POINT('Ctrl Pts',(-4.15331797782398,39.8560841569777,-16.2312023454786));
#57500=CARTESIAN_POINT('Ctrl Pts',(-4.49815720553132,39.9323631382508,-15.8750321376815));
#57501=CARTESIAN_POINT('Ctrl Pts',(-4.23198682506552,39.8477579670653,-15.9504505711255));
#57502=CARTESIAN_POINT('Ctrl Pts',(-4.16769545413477,39.805615099322,-16.2293456787121));
#57503=CARTESIAN_POINT('Ctrl Pts',(-4.50569299128003,39.9058006819841,-15.8728948158664));
#57504=CARTESIAN_POINT('Ctrl Pts',(-4.23865969846769,39.8219707212385,-15.9486947308374));
#57505=CARTESIAN_POINT('Ctrl Pts',(-4.1747537660165,39.7803601224423,-16.2284510688984));
#57506=CARTESIAN_POINT('Ctrl Pts',(-4.52788908225558,39.8260548181995,-15.8665830325155));
#57507=CARTESIAN_POINT('Ctrl Pts',(-4.25828083324603,39.7445109973632,-15.9435203785516));
#57508=CARTESIAN_POINT('Ctrl Pts',(-4.19554349286319,39.7045346637349,-16.2258684245472));
#57509=CARTESIAN_POINT('Ctrl Pts',(-4.54213820519509,39.7728129265089,-15.8625087615832));
#57510=CARTESIAN_POINT('Ctrl Pts',(-4.27080745248769,39.6928283677743,-15.9402013833087));
#57511=CARTESIAN_POINT('Ctrl Pts',(-4.20888977911923,39.6539036641976,-16.2242815829051));
#57512=CARTESIAN_POINT('Ctrl Pts',(-4.61072350551952,39.5062243012366,-15.8428055513534));
#57513=CARTESIAN_POINT('Ctrl Pts',(-4.33101064476337,39.4331423066517,-15.9241892497505));
#57514=CARTESIAN_POINT('Ctrl Pts',(-4.27312945361112,39.4003554433727,-16.2170217104017));
#57515=CARTESIAN_POINT('Ctrl Pts',(-4.65710151667135,39.2917430094221,-15.8291830985343));
#57516=CARTESIAN_POINT('Ctrl Pts',(-4.37047377111817,39.2249262086857,-15.9134966630587));
#57517=CARTESIAN_POINT('Ctrl Pts',(-4.3165689141374,39.1962612675561,-16.2133735716419));
#57518=CARTESIAN_POINT('Ctrl Pts',(-4.73455890330831,38.860584008785,-15.8061881582692));
#57519=CARTESIAN_POINT('Ctrl Pts',(-4.43416228480996,38.806836206605,-15.8961542515918));
#57520=CARTESIAN_POINT('Ctrl Pts',(-4.38911853157358,38.7857773011577,-16.2103568495108));
#57521=CARTESIAN_POINT('Ctrl Pts',(-4.7656335172996,38.6439056908728,-15.7968150887316));
#57522=CARTESIAN_POINT('Ctrl Pts',(-4.45824992940577,38.596715083291,-15.8895386759589));
#57523=CARTESIAN_POINT('Ctrl Pts',(-4.41822423140701,38.5793869570085,-16.2109877211159));
#57524=CARTESIAN_POINT('Ctrl Pts',(-4.81366277021719,38.2085119119448,-15.7822457370113));
#57525=CARTESIAN_POINT('Ctrl Pts',(-4.49228715046657,38.1750784013236,-15.8802583836643));
#57526=CARTESIAN_POINT('Ctrl Pts',(-4.46321030786492,38.1644661155498,-16.2164498115114));
#57527=CARTESIAN_POINT('Ctrl Pts',(-4.83061473177268,37.989796110882,-15.7770490650161));
#57528=CARTESIAN_POINT('Ctrl Pts',(-4.50207912059962,37.963297937123,-15.8776364690345));
#57529=CARTESIAN_POINT('Ctrl Pts',(-4.47908817873774,37.9559353121758,-16.2212806621887));
#57530=CARTESIAN_POINT('Ctrl Pts',(-4.85119740418559,37.5504372754616,-15.7707323746352));
#57531=CARTESIAN_POINT('Ctrl Pts',(-4.50825772146479,37.5385831425256,-15.8762196986871));
#57532=CARTESIAN_POINT('Ctrl Pts',(-4.49836671444632,37.5368431558517,-16.2350392361057));
#57533=CARTESIAN_POINT('Ctrl Pts',(-4.85482680237322,37.3297940775806,-15.7696120833341));
#57534=CARTESIAN_POINT('Ctrl Pts',(-4.50446088793284,37.3253626831583,-15.8774765117451));
#57535=CARTESIAN_POINT('Ctrl Pts',(-4.50176615109278,37.3262816596819,-16.2439666982713));
#57536=CARTESIAN_POINT('Ctrl Pts',(-4.85133542686646,37.0528279294366,-15.7706862599499));
#57537=CARTESIAN_POINT('Ctrl Pts',(-4.49167305004904,37.059789020437,-15.8813246755956));
#57538=CARTESIAN_POINT('Ctrl Pts',(-4.49849599207902,37.0618545761177,-16.2576124902641));
#57539=CARTESIAN_POINT('Ctrl Pts',(-4.85023355700303,36.9973424024009,-15.7710252327459));
#57540=CARTESIAN_POINT('Ctrl Pts',(-4.4886839703737,37.0062991010676,-15.8822165992224));
#57541=CARTESIAN_POINT('Ctrl Pts',(-4.49746393778067,37.0088752437307,-16.2604679296177));
#57542=CARTESIAN_POINT('Ctrl Pts',(-4.84724165567112,36.8866091092228,-15.7719450538262));
#57543=CARTESIAN_POINT('Ctrl Pts',(-4.48191083668474,36.8995910435531,-15.884223449632));
#57544=CARTESIAN_POINT('Ctrl Pts',(-4.49466160577087,36.9031322050459,-16.2664058785488));
#57545=CARTESIAN_POINT('Ctrl Pts',(-4.84535166014932,36.8313248270939,-15.7725258903161));
#57546=CARTESIAN_POINT('Ctrl Pts',(-4.47812221634299,36.846334338376,-15.8853396943));
#57547=CARTESIAN_POINT('Ctrl Pts',(-4.49289136220764,36.8503336431165,-16.2694900363544));
#57548=CARTESIAN_POINT('Ctrl Pts',(-4.83852205833163,36.6657142912634,-15.7746228790373));
#57549=CARTESIAN_POINT('Ctrl Pts',(-4.46555605276301,36.6865436945369,-15.8890228148251));
#57550=CARTESIAN_POINT('Ctrl Pts',(-4.48649448972876,36.6921526528426,-16.2790801157266));
#57551=CARTESIAN_POINT('Ctrl Pts',(-4.83242355820479,36.5556302061425,-15.7764934506682));
#57552=CARTESIAN_POINT('Ctrl Pts',(-4.45560823761615,36.5806099310771,-15.8919151266673));
#57553=CARTESIAN_POINT('Ctrl Pts',(-4.48078239625453,36.5869847872263,-16.2859235908837));
#57554=CARTESIAN_POINT('Ctrl Pts',(-4.80964445731595,36.2263139098162,-15.7834588216173));
#57555=CARTESIAN_POINT('Ctrl Pts',(-4.42108305755237,36.2626839420804,-15.9018687747033));
#57556=CARTESIAN_POINT('Ctrl Pts',(-4.45944659885922,36.2723112115469,-16.3077427542653));
#57557=CARTESIAN_POINT('Ctrl Pts',(-4.78849025521988,36.0080156926272,-15.7899064986773));
#57558=CARTESIAN_POINT('Ctrl Pts',(-4.39194405386607,36.0530811161892,-15.9101712621084));
#57559=CARTESIAN_POINT('Ctrl Pts',(-4.43963274611102,36.0636336832212,-16.3240065044515));
#57560=CARTESIAN_POINT('Ctrl Pts',(-4.73479895287024,35.5737873220669,-15.806089492256));
#57561=CARTESIAN_POINT('Ctrl Pts',(-4.32221309888832,35.6372576288513,-15.9296899223679));
#57562=CARTESIAN_POINT('Ctrl Pts',(-4.38934337165934,35.6483850846731,-16.3596596636497));
#57563=CARTESIAN_POINT('Ctrl Pts',(-4.70226083470289,35.3578573765994,-15.8158250321208));
#57564=CARTESIAN_POINT('Ctrl Pts',(-4.28136065754713,35.4308416469974,-15.9409730418437));
#57565=CARTESIAN_POINT('Ctrl Pts',(-4.35886689759704,35.4418142023149,-16.3790492831481));
#57566=CARTESIAN_POINT('Ctrl Pts',(-4.62604323000226,34.9283028530584,-15.838285969081));
#57567=CARTESIAN_POINT('Ctrl Pts',(-4.18843254356921,35.0215742894843,-15.9661140402609));
#57568=CARTESIAN_POINT('Ctrl Pts',(-4.28747850736095,35.030732994809,-16.4206641704048));
#57569=CARTESIAN_POINT('Ctrl Pts',(-4.58236381820235,34.7146782724582,-15.851011583154));
#57570=CARTESIAN_POINT('Ctrl Pts',(-4.13606020425487,34.8185183918786,-15.9800423530578));
#57571=CARTESIAN_POINT('Ctrl Pts',(-4.24656666166447,34.8262226570115,-16.4428896521688));
#57572=CARTESIAN_POINT('Ctrl Pts',(-4.48381152977406,34.2897290978801,-15.8791706501668));
#57573=CARTESIAN_POINT('Ctrl Pts',(-4.02005922178393,34.4162818436401,-16.0101335970749));
#57574=CARTESIAN_POINT('Ctrl Pts',(-4.15425873313437,34.4192706098088,-16.489899151371));
#57575=CARTESIAN_POINT('Ctrl Pts',(-4.42893989399129,34.0784042783794,-15.8946043422336));
#57576=CARTESIAN_POINT('Ctrl Pts',(-3.95608545255841,34.2168878693719,-16.0263702668423));
#57577=CARTESIAN_POINT('Ctrl Pts',(-4.10286381244933,34.2168286739799,-16.5146834150258));
#57578=CARTESIAN_POINT('Ctrl Pts',(-4.30763827259879,33.6581098781651,-15.9279065885377));
#57579=CARTESIAN_POINT('Ctrl Pts',(-3.81658438476888,33.822448010845,-16.0607242667002));
#57580=CARTESIAN_POINT('Ctrl Pts',(-3.9892479689298,33.814078955275,-16.5665395015097));
#57581=CARTESIAN_POINT('Ctrl Pts',(-4.24121110891681,33.4491397713452,-15.9457754442683));
#57582=CARTESIAN_POINT('Ctrl Pts',(-3.7406469800499,33.6271818424222,-16.0789181512321));
#57583=CARTESIAN_POINT('Ctrl Pts',(-3.92702968859027,33.6137706563386,-16.593611645947));
#57584=CARTESIAN_POINT('Ctrl Pts',(-4.15956467569048,33.2154445308089,-15.9670945891216));
#57585=CARTESIAN_POINT('Ctrl Pts',(-3.64949552390511,33.4129433397945,-16.0999721147917));
#57586=CARTESIAN_POINT('Ctrl Pts',(-3.8505564455756,33.3896995093833,-16.6252009188576));
#57587=CARTESIAN_POINT('Ctrl Pts',(-4.15039805956273,33.189502508749,-15.9694798681321));
#57588=CARTESIAN_POINT('Ctrl Pts',(-3.63914933651993,33.3888967259962,-16.102351301209));
#57589=CARTESIAN_POINT('Ctrl Pts',(-3.84197063429969,33.3648249628758,-16.6287259546484));
#57590=CARTESIAN_POINT('Ctrl Pts',(-4.13189835567043,33.1377349934672,-15.9742764246118));
#57591=CARTESIAN_POINT('Ctrl Pts',(-3.61829077577786,33.3409526006064,-16.1071260478771));
#57592=CARTESIAN_POINT('Ctrl Pts',(-3.82464308795729,33.3151858843453,-16.635796298032));
#57593=CARTESIAN_POINT('Ctrl Pts',(-4.12256202229053,33.111900164225,-15.9766885508706));
#57594=CARTESIAN_POINT('Ctrl Pts',(-3.60777388976757,33.3170463264599,-16.1095225753306));
#57595=CARTESIAN_POINT('Ctrl Pts',(-3.81589831288601,33.2904124009369,-16.6393428649039));
#57596=CARTESIAN_POINT('Ctrl Pts',(-4.09429258351795,33.0345428662843,-15.9839653076811));
#57597=CARTESIAN_POINT('Ctrl Pts',(-3.57590653652943,33.2454014404084,-16.1167504752498));
#57598=CARTESIAN_POINT('Ctrl Pts',(-3.78942005068434,33.2162305590499,-16.6500155854832));
#57599=CARTESIAN_POINT('Ctrl Pts',(-4.07509908358835,32.9831675632239,-15.9888703159868));
#57600=CARTESIAN_POINT('Ctrl Pts',(-3.55434588845088,33.1979873053765,-16.1215955300393));
#57601=CARTESIAN_POINT('Ctrl Pts',(-3.77144266781143,33.1669607859179,-16.6571747604242));
#57602=CARTESIAN_POINT('Ctrl Pts',(-4.01646745258513,32.829634429189,-16.0037375413478));
#57603=CARTESIAN_POINT('Ctrl Pts',(-3.48838399516754,33.0560510137945,-16.1362734133368));
#57604=CARTESIAN_POINT('Ctrl Pts',(-3.71652598867197,33.0197101694359,-16.6787750251782));
#57605=CARTESIAN_POINT('Ctrl Pts',(-3.9759789438393,32.728068962807,-16.0138519706474));
#57606=CARTESIAN_POINT('Ctrl Pts',(-3.44313323859855,32.9628501297851,-16.1461489724732));
#57607=CARTESIAN_POINT('Ctrl Pts',(-3.67860286745824,32.9222876367011,-16.6933388861798));
#57608=CARTESIAN_POINT('Ctrl Pts',(-3.85020901317665,32.4257893774983,-16.0447294945566));
#57609=CARTESIAN_POINT('Ctrl Pts',(-3.30213588601185,32.6845768004043,-16.1762600178974));
#57610=CARTESIAN_POINT('Ctrl Pts',(-3.56080183062287,32.6323019776143,-16.7374460185429));
#57611=CARTESIAN_POINT('Ctrl Pts',(-3.76063777621999,32.2274841877532,-16.0660275892435));
#57612=CARTESIAN_POINT('Ctrl Pts',(-3.20289234856102,32.5050107524786,-16.1965656821621));
#57613=CARTESIAN_POINT('Ctrl Pts',(-3.47690590589959,32.4420132288924,-16.767405951522));
#57614=CARTESIAN_POINT('Ctrl Pts',(-3.56918607340305,31.8377243308601,-16.1096415154308));
#57615=CARTESIAN_POINT('Ctrl Pts',(-2.99311023840048,32.1562009537945,-16.2372785343144));
#57616=CARTESIAN_POINT('Ctrl Pts',(-3.29758475214954,32.0679272033942,-16.8280153427249));
#57617=CARTESIAN_POINT('Ctrl Pts',(-3.46731167512559,31.6462664711462,-16.1319583909726));
#57618=CARTESIAN_POINT('Ctrl Pts',(-2.88201843494523,31.9870356344035,-16.2577213825395));
#57619=CARTESIAN_POINT('Ctrl Pts',(-3.20216520503585,31.8841268311116,-16.8586659752245));
#57620=CARTESIAN_POINT('Ctrl Pts',(-3.24986431304015,31.2709079333655,-16.1771664307246));
#57621=CARTESIAN_POINT('Ctrl Pts',(-2.6480156494036,31.6607525771679,-16.2980633785119));
#57622=CARTESIAN_POINT('Ctrl Pts',(-2.99849550013316,31.5237128636391,-16.9201885252478));
#57623=CARTESIAN_POINT('Ctrl Pts',(-3.13430309790084,31.087001037092,-16.2000593106867));
#57624=CARTESIAN_POINT('Ctrl Pts',(-2.52446501017816,31.5038249498316,-16.3179747703128));
#57625=CARTESIAN_POINT('Ctrl Pts',(-2.89025634469189,31.3470932540427,-16.9510624162517));
#57626=CARTESIAN_POINT('Ctrl Pts',(-2.97992813214864,30.8625464320075,-16.2287095736517));
#57627=CARTESIAN_POINT('Ctrl Pts',(-2.36471133653988,31.3195585189969,-16.3416730253026));
#57628=CARTESIAN_POINT('Ctrl Pts',(-2.74566271341961,31.1314993826496,-16.9894416021804));
#57629=CARTESIAN_POINT('Ctrl Pts',(-2.94855445916935,30.817928300523,-16.2344410657162));
#57630=CARTESIAN_POINT('Ctrl Pts',(-2.33186814409271,31.2826216760433,-16.3464413005094));
#57631=CARTESIAN_POINT('Ctrl Pts',(-2.71627690378355,31.0886409312827,-16.9971064561535));
#57632=CARTESIAN_POINT('Ctrl Pts',(-2.88476410492296,30.7292614499473,-16.2458975182613));
#57633=CARTESIAN_POINT('Ctrl Pts',(-2.26536475661494,31.2097212908695,-16.3558796919869));
#57634=CARTESIAN_POINT('Ctrl Pts',(-2.65652836285939,31.0034678637871,-17.0124038567864));
#57635=CARTESIAN_POINT('Ctrl Pts',(-2.85231509096079,30.6851711096193,-16.2516279588096));
#57636=CARTESIAN_POINT('Ctrl Pts',(-2.23166075706606,31.1737321819387,-16.3605534424715));
#57637=CARTESIAN_POINT('Ctrl Pts',(-2.62613534683824,30.9611132622823,-17.0200436860762));
#57638=CARTESIAN_POINT('Ctrl Pts',(-2.75371586507387,30.5543032513299,-16.2687276605509));
#57639=CARTESIAN_POINT('Ctrl Pts',(-2.12916708502008,31.0671513308951,-16.3744245592637));
#57640=CARTESIAN_POINT('Ctrl Pts',(-2.53378345502449,30.8353931303199,-17.0428092866419));
#57641=CARTESIAN_POINT('Ctrl Pts',(-2.68624145339725,30.4688168020419,-16.280019596665));
#57642=CARTESIAN_POINT('Ctrl Pts',(-2.05994523352376,30.9990432166992,-16.3833298319653));
#57643=CARTESIAN_POINT('Ctrl Pts',(-2.47058428125334,30.7532636055963,-17.057800327605));
#57644=CARTESIAN_POINT('Ctrl Pts',(-2.54757388740944,30.3015880840125,-16.3022942711121));
#57645=CARTESIAN_POINT('Ctrl Pts',(-1.9192454319902,30.8681341748231,-16.4004596153518));
#57646=CARTESIAN_POINT('Ctrl Pts',(-2.34070281481905,30.5925930259895,-17.0873081301815));
#57647=CARTESIAN_POINT('Ctrl Pts',(-2.476381206771,30.2198453486412,-16.3132771209141));
#57648=CARTESIAN_POINT('Ctrl Pts',(-1.84771884517628,30.8054525230851,-16.4086687974615));
#57649=CARTESIAN_POINT('Ctrl Pts',(-2.27402096482143,30.5140515215888,-17.1018250250437));
#57650=CARTESIAN_POINT('Ctrl Pts',(-2.32998205788182,30.0603897553416,-16.334829595528));
#57651=CARTESIAN_POINT('Ctrl Pts',(-1.70258673578777,30.6857855527938,-16.4242870257666));
#57652=CARTESIAN_POINT('Ctrl Pts',(-2.13689779545945,30.3608345647763,-17.1302692409457));
#57653=CARTESIAN_POINT('Ctrl Pts',(-2.25477627281575,29.982676223402,-16.345399374049));
#57654=CARTESIAN_POINT('Ctrl Pts',(-1.62894510471729,30.6289401059803,-16.4316764817347));
#57655=CARTESIAN_POINT('Ctrl Pts',(-2.06645711480206,30.2861584632619,-17.1441967467396));
#57656=CARTESIAN_POINT('Ctrl Pts',(-2.09997874346892,29.831641210054,-16.3660070272072));
#57657=CARTESIAN_POINT('Ctrl Pts',(-1.47982485477628,30.5213540438189,-16.4455349971866));
#57658=CARTESIAN_POINT('Ctrl Pts',(-1.92146769383922,30.1410235804603,-17.1713290042148));
#57659=CARTESIAN_POINT('Ctrl Pts',(-2.02038800914664,29.7583187312675,-16.3760451220302));
#57660=CARTESIAN_POINT('Ctrl Pts',(-1.40432964804446,30.4707756283822,-16.4519799689631));
#57661=CARTESIAN_POINT('Ctrl Pts',(-1.84691989810708,30.0705638387238,-17.1845340213945));
#57662=CARTESIAN_POINT('Ctrl Pts',(-1.89735688368434,29.6519763755937,-16.3905992032782));
#57663=CARTESIAN_POINT('Ctrl Pts',(-1.29061421420031,30.4002010119293,-16.4608187862555));
#57664=CARTESIAN_POINT('Ctrl Pts',(-1.73168413361204,29.9683736297906,-17.2036812816511));
#57665=CARTESIAN_POINT('Ctrl Pts',(-1.855738117802,29.6171366953533,-16.3953665421613));
#57666=CARTESIAN_POINT('Ctrl Pts',(-1.25230151783671,30.3773864795662,-16.4636476099762));
#57667=CARTESIAN_POINT('Ctrl Pts',(-1.69270236914862,29.9348943080071,-17.2099534441512));
#57668=CARTESIAN_POINT('Ctrl Pts',(-1.79234339952953,29.5658416895116,-16.4023765699238));
#57669=CARTESIAN_POINT('Ctrl Pts',(-1.19475183342288,30.3445305772294,-16.4676726412067));
#57670=CARTESIAN_POINT('Ctrl Pts',(-1.63332439632481,29.8856025996842,-17.2191791942467));
#57671=CARTESIAN_POINT('Ctrl Pts',(-1.77105066057652,29.5489041771658,-16.4046897342604));
#57672=CARTESIAN_POINT('Ctrl Pts',(-1.17547199819176,30.333762872091,-16.4689831252204));
#57673=CARTESIAN_POINT('Ctrl Pts',(-1.6133807839376,29.8693266444902,-17.2222240118077));
#57674=CARTESIAN_POINT('Ctrl Pts',(-1.72813291087157,29.5153605402291,-16.409266356606));
#57675=CARTESIAN_POINT('Ctrl Pts',(-1.13683610528857,30.3126589001511,-16.4715332981359));
#57676=CARTESIAN_POINT('Ctrl Pts',(-1.57318234083472,29.8370933859026,-17.2282496978405));
#57677=CARTESIAN_POINT('Ctrl Pts',(-1.70649633572161,29.4987461608599,-16.4115309334004));
#57678=CARTESIAN_POINT('Ctrl Pts',(-1.11747086839056,30.3023210014394,-16.4727730500227));
#57679=CARTESIAN_POINT('Ctrl Pts',(-1.5529166780537,29.8211281512158,-17.231232043014));
#57680=CARTESIAN_POINT('Ctrl Pts',(-1.59782880094616,29.416805054283,-16.4226849288261));
#57681=CARTESIAN_POINT('Ctrl Pts',(-1.01994827144306,30.2514460679374,-16.4788242146341));
#57682=CARTESIAN_POINT('Ctrl Pts',(-1.45113441423997,29.7423892766781,-17.2459262700218));
#57683=CARTESIAN_POINT('Ctrl Pts',(-1.50908967345445,29.3546606084382,-16.4310964828382));
#57684=CARTESIAN_POINT('Ctrl Pts',(-0.94294827805055,30.2151476418465,-16.4829741135679));
#57685=CARTESIAN_POINT('Ctrl Pts',(-1.36801787580905,29.6826756493925,-17.2570235387147));
#57686=CARTESIAN_POINT('Ctrl Pts',(-1.32773854032885,29.2376739642212,-16.446744165317));
#57687=CARTESIAN_POINT('Ctrl Pts',(-0.789958819385205,30.1499851126795,
-16.4900488930594));
#57688=CARTESIAN_POINT('Ctrl Pts',(-1.19815731065464,29.570273767709,-17.2777301553418));
#57689=CARTESIAN_POINT('Ctrl Pts',(-1.23512712642901,29.1828306555037,-16.4539805128856));
#57690=CARTESIAN_POINT('Ctrl Pts',(-0.714148771847181,30.1213547087018,
-16.4929390217047));
#57691=CARTESIAN_POINT('Ctrl Pts',(-1.11141383725493,29.5175844450748,-17.2873397728772));
#57692=CARTESIAN_POINT('Ctrl Pts',(-1.04569979909049,29.0810615938186,-16.4671043497951));
#57693=CARTESIAN_POINT('Ctrl Pts',(-0.564018986317464,30.0710934810012,
-16.4975516672181));
#57694=CARTESIAN_POINT('Ctrl Pts',(-0.933988792708237,29.4198266340564,
-17.3048725518148));
#57695=CARTESIAN_POINT('Ctrl Pts',(-0.948884762668731,29.0341341932451,
-16.4729921490482));
#57696=CARTESIAN_POINT('Ctrl Pts',(-0.489933276919771,30.0496744036365,
-16.4992439979384));
#57697=CARTESIAN_POINT('Ctrl Pts',(-0.843308041987629,29.3747565609294,
-17.3127960973893));
#57698=CARTESIAN_POINT('Ctrl Pts',(-0.800191680576077,28.9702716007703,
-16.4806600727396));
#57699=CARTESIAN_POINT('Ctrl Pts',(-0.380586307990408,30.0223765474346,
-16.5009885630312));
#57700=CARTESIAN_POINT('Ctrl Pts',(-0.704036284927813,29.3134377089103,
-17.3232401222866));
#57701=CARTESIAN_POINT('Ctrl Pts',(-0.750048107089607,28.9500736446709,
-16.483021826383));
#57702=CARTESIAN_POINT('Ctrl Pts',(-0.344229360090164,30.014052241189,-16.5014375482369));
#57703=CARTESIAN_POINT('Ctrl Pts',(-0.657069852279363,29.2940472367443,
-17.3264809285521));
#57704=CARTESIAN_POINT('Ctrl Pts',(-0.673915805988587,28.9215008203245,
-16.486251322221));
#57705=CARTESIAN_POINT('Ctrl Pts',(-0.290130099099646,30.0026923249378,
-16.501926978582));
#57706=CARTESIAN_POINT('Ctrl Pts',(-0.585761361026588,29.2666219330869,
-17.3309558082814));
#57707=CARTESIAN_POINT('Ctrl Pts',(-0.648385485598382,28.91226401611,-16.4872756105357));
#57708=CARTESIAN_POINT('Ctrl Pts',(-0.272119298069543,29.9990851554066,
-16.5020595144662));
#57709=CARTESIAN_POINT('Ctrl Pts',(-0.561848664151634,29.2577570144913,
-17.3323830214636));
#57710=CARTESIAN_POINT('Ctrl Pts',(-0.597010216853532,28.8943818767733,
-16.4892158575437));
#57711=CARTESIAN_POINT('Ctrl Pts',(-0.2362023844278,29.9922245088925,-16.5022661141874));
#57712=CARTESIAN_POINT('Ctrl Pts',(-0.513728577814346,29.2405968337917,
-17.3351040222603));
#57713=CARTESIAN_POINT('Ctrl Pts',(-0.571233147511417,28.8857606891544,
-16.4901291611817));
#57714=CARTESIAN_POINT('Ctrl Pts',(-0.218349366931985,29.9889826962993,
-16.5023396092702));
#57715=CARTESIAN_POINT('Ctrl Pts',(-0.4895847662591,29.2323247467198,-17.3363941024547));
#57716=CARTESIAN_POINT('Ctrl Pts',(-0.442166073327688,28.8443554178395,
-16.4943979018314));
#57717=CARTESIAN_POINT('Ctrl Pts',(-0.129239837306087,29.9735906916381,
-16.5025703106399));
#57718=CARTESIAN_POINT('Ctrl Pts',(-0.368695495698975,29.1926016196164,
-17.342474342916));
#57719=CARTESIAN_POINT('Ctrl Pts',(-0.338061778022354,28.8165747708187,
-16.4968705077674));
#57720=CARTESIAN_POINT('Ctrl Pts',(-0.0605317814243137,29.9642648979254,
-16.5023091130787));
#57721=CARTESIAN_POINT('Ctrl Pts',(-0.271187340267436,29.1659679325416,
-17.3461688365462));
#57722=CARTESIAN_POINT('Ctrl Pts',(-0.128108295013126,28.7719728676628,
-16.499836683451));
#57723=CARTESIAN_POINT('Ctrl Pts',(0.074456716006171,29.94974338385,-16.5011651314723));
#57724=CARTESIAN_POINT('Ctrl Pts',(-0.0745366950826016,29.1232544765027,
-17.3511133431508));
#57725=CARTESIAN_POINT('Ctrl Pts',(-0.0222591829595038,28.755151135902,
-16.5003303276454));
#57726=CARTESIAN_POINT('Ctrl Pts',(0.140356992327616,29.9446203245694,-16.5002807332538));
#57727=CARTESIAN_POINT('Ctrl Pts',(0.0246057239760995,29.1071742509764,
-17.3523634528138));
#57728=CARTESIAN_POINT('Ctrl Pts',(0.191245793985154,28.7328543901453,-16.499236995659));
#57729=CARTESIAN_POINT('Ctrl Pts',(0.27161304708856,29.937520037568,-16.4980385051));
#57730=CARTESIAN_POINT('Ctrl Pts',(0.224582837315142,29.0859421960738,-17.3523016800784));
#57731=CARTESIAN_POINT('Ctrl Pts',(0.298901540034271,28.7273786281084,-16.4976501104633));
#57732=CARTESIAN_POINT('Ctrl Pts',(0.336593949719366,29.9355704487499,-16.496686377349));
#57733=CARTESIAN_POINT('Ctrl Pts',(0.325417420428351,29.080789649795,-17.3509899235518));
#57734=CARTESIAN_POINT('Ctrl Pts',(0.434652344247154,28.7279511908531,-16.4942964360642));
#57735=CARTESIAN_POINT('Ctrl Pts',(0.41904432966663,29.9349828888683,-16.4946901599378));
#57736=CARTESIAN_POINT('Ctrl Pts',(0.452566934002955,29.0814932456998,-17.3476656555962));
#57737=CARTESIAN_POINT('Ctrl Pts',(0.461791435185215,28.7284371115372,-16.4935588164354));
#57738=CARTESIAN_POINT('Ctrl Pts',(0.435530517342106,29.9349612139799,-16.4942766579394));
#57739=CARTESIAN_POINT('Ctrl Pts',(0.477986468216754,29.0819916232635,-17.3469181407489));
#57740=CARTESIAN_POINT('Ctrl Pts',(0.515943690984539,28.7301437164452,-16.4919536704588));
#57741=CARTESIAN_POINT('Ctrl Pts',(0.468495969700064,29.9351121018813,-16.4934206136822));
#57742=CARTESIAN_POINT('Ctrl Pts',(0.528707589352712,29.0836958274767,-17.3452619533545));
#57743=CARTESIAN_POINT('Ctrl Pts',(0.542973446398712,28.7313644483332,-16.4910857384778));
#57744=CARTESIAN_POINT('Ctrl Pts',(0.484979151558676,29.9352844403668,-16.4929780058774));
#57745=CARTESIAN_POINT('Ctrl Pts',(0.554024715635541,29.084901718379,-17.344352879355));
#57746=CARTESIAN_POINT('Ctrl Pts',(0.623924958202809,28.7361181266015,-16.4882877715005));
#57747=CARTESIAN_POINT('Ctrl Pts',(0.534479466208411,29.9361010848821,-16.4916034160629));
#57748=CARTESIAN_POINT('Ctrl Pts',(0.629847068288364,29.0895703548083,-17.3413850837553));
#57749=CARTESIAN_POINT('Ctrl Pts',(0.677708990090665,28.7407423067484,-16.4861635783227));
#57750=CARTESIAN_POINT('Ctrl Pts',(0.567561890649228,29.9370419497641,-16.490624834322));
#57751=CARTESIAN_POINT('Ctrl Pts',(0.680223296507896,29.0940838248501,-17.339085810858));
#57752=CARTESIAN_POINT('Ctrl Pts',(0.838519927256103,28.7589030127749,-16.4790291084593));
#57753=CARTESIAN_POINT('Ctrl Pts',(0.667392543733618,29.9411882626693,-16.4874678461666));
#57754=CARTESIAN_POINT('Ctrl Pts',(0.830845110920096,29.1117531657169,-17.3312437799614));
#57755=CARTESIAN_POINT('Ctrl Pts',(0.945006106505387,28.7767241011346,-16.4732571040723));
#57756=CARTESIAN_POINT('Ctrl Pts',(0.734797573094118,29.9456748746285,-16.4850736283494));
#57757=CARTESIAN_POINT('Ctrl Pts',(0.930584232001352,29.1290345185376,-17.3247571305769));
#57758=CARTESIAN_POINT('Ctrl Pts',(1.07723807457993,28.8059438373021,-16.4648188690481));
#57759=CARTESIAN_POINT('Ctrl Pts',(0.821934628374837,29.9543140629695,-16.481507158621));
#57760=CARTESIAN_POINT('Ctrl Pts',(1.05443786599453,29.1573212640841,-17.315130200981));
#57761=CARTESIAN_POINT('Ctrl Pts',(1.10366391397319,28.8121410610613,-16.4630684410996));
#57762=CARTESIAN_POINT('Ctrl Pts',(0.839404777360703,29.9561838764168,-16.4807692180936));
#57763=CARTESIAN_POINT('Ctrl Pts',(1.07918934093606,29.1633187716124,-17.3131270133982));
#57764=CARTESIAN_POINT('Ctrl Pts',(1.15632374754114,28.8252003709767,-16.4594535730141));
#57765=CARTESIAN_POINT('Ctrl Pts',(0.874521011859752,29.9602382847319,-16.4792360955938));
#57766=CARTESIAN_POINT('Ctrl Pts',(1.12851260097818,29.1759537682257,-17.3089782907615));
#57767=CARTESIAN_POINT('Ctrl Pts',(1.18250126727682,28.8320477321608,-16.4575931395356));
#57768=CARTESIAN_POINT('Ctrl Pts',(0.892123466946685,29.9624166282505,-16.4784430213444));
#57769=CARTESIAN_POINT('Ctrl Pts',(1.15303149003764,29.1825770131165,-17.3068373640129));
#57770=CARTESIAN_POINT('Ctrl Pts',(1.26059001577615,28.8535152040682,-16.4518581803553));
#57771=CARTESIAN_POINT('Ctrl Pts',(0.945006269189896,29.9694228223987,-16.4759818429639));
#57772=CARTESIAN_POINT('Ctrl Pts',(1.22617246651459,29.2033372707004,-17.3002214041692));
#57773=CARTESIAN_POINT('Ctrl Pts',(1.31205768956044,28.8690601669617,-16.4478300726312));
#57774=CARTESIAN_POINT('Ctrl Pts',(0.980523921137524,29.974736003371,-16.4742254675058));
#57775=CARTESIAN_POINT('Ctrl Pts',(1.27437910322739,29.2183642879055,-17.2955532864967));
#57776=CARTESIAN_POINT('Ctrl Pts',(1.4647831287284,28.9191944472757,-16.43517107612));
#57777=CARTESIAN_POINT('Ctrl Pts',(1.08747216242771,29.9927517710206,-16.4685881506749));
#57778=CARTESIAN_POINT('Ctrl Pts',(1.41742772376219,29.2668125837537,-17.2808247001297));
#57779=CARTESIAN_POINT('Ctrl Pts',(1.56436648530266,28.957276499474,-16.4259664459877));
#57780=CARTESIAN_POINT('Ctrl Pts',(1.15996351383399,30.0075731994565,-16.4643154615969));
#57781=CARTESIAN_POINT('Ctrl Pts',(1.51070139131698,29.3035947033487,-17.2700412085024));
#57782=CARTESIAN_POINT('Ctrl Pts',(1.75949339397493,29.0418768304825,-16.4062122131103));
#57783=CARTESIAN_POINT('Ctrl Pts',(1.30740732628336,30.0440019520787,-16.4545229469892));
#57784=CARTESIAN_POINT('Ctrl Pts',(1.69346488679426,29.385274695068,-17.246768023877));
#57785=CARTESIAN_POINT('Ctrl Pts',(1.85503603822308,29.0883970101933,-16.3956623294501));
#57786=CARTESIAN_POINT('Ctrl Pts',(1.38208746912005,30.0654311191767,-16.449040555324));
#57787=CARTESIAN_POINT('Ctrl Pts',(1.78295386512358,29.4301743920079,-17.2342779633839));
#57788=CARTESIAN_POINT('Ctrl Pts',(2.04241537792939,29.1891877116256,-16.3733759911771));
#57789=CARTESIAN_POINT('Ctrl Pts',(1.53349668675425,30.1157894070632,-16.4367176133733));
#57790=CARTESIAN_POINT('Ctrl Pts',(1.95846068444071,29.5274274114621,-17.2077786001255));
#57791=CARTESIAN_POINT('Ctrl Pts',(2.13425146341608,29.2434595083696,-16.3616393385331));
#57792=CARTESIAN_POINT('Ctrl Pts',(1.61000429268926,30.1445060379138,-16.4299192937042));
#57793=CARTESIAN_POINT('Ctrl Pts',(2.04447795482465,29.5797819581103,-17.1937690407036));
#57794=CARTESIAN_POINT('Ctrl Pts',(2.3144828178405,29.3592119103105,-16.3371184864176));
#57795=CARTESIAN_POINT('Ctrl Pts',(1.76445361782877,30.2098541291851,-16.4149279831066));
#57796=CARTESIAN_POINT('Ctrl Pts',(2.21328969153138,29.6914212472574,-17.1643920201756));
#57797=CARTESIAN_POINT('Ctrl Pts',(2.40287766710257,29.4206933906018,-16.3243341414413));
#57798=CARTESIAN_POINT('Ctrl Pts',(1.84222493333582,30.2462536617642,-16.4067789597616));
#57799=CARTESIAN_POINT('Ctrl Pts',(2.29608376542315,29.7507068302044,-17.1490243729861));
#57800=CARTESIAN_POINT('Ctrl Pts',(2.51135285252538,29.5017829309144,-16.3077769328132));
#57801=CARTESIAN_POINT('Ctrl Pts',(1.94077379223057,30.2972459914495,-16.3956391132683));
#57802=CARTESIAN_POINT('Ctrl Pts',(2.39768586735591,29.8288858890433,-17.1290549495678));
#57803=CARTESIAN_POINT('Ctrl Pts',(2.53290170127805,29.5181794566019,-16.3044434790811));
#57804=CARTESIAN_POINT('Ctrl Pts',(1.96028897303141,30.3075771594425,-16.3933941774779));
#57805=CARTESIAN_POINT('Ctrl Pts',(2.41786936214229,29.8446932300906,-17.1250312972996));
#57806=CARTESIAN_POINT('Ctrl Pts',(2.57565545767622,29.5512731693992,-16.2977442351459));
#57807=CARTESIAN_POINT('Ctrl Pts',(1.99921568638862,30.3286552806381,-16.3888383057235));
#57808=CARTESIAN_POINT('Ctrl Pts',(2.45791420271846,29.8765964221614,-17.1169385254278));
#57809=CARTESIAN_POINT('Ctrl Pts',(2.59687024481893,29.5679777347785,-16.2943769383145));
#57810=CARTESIAN_POINT('Ctrl Pts',(2.01863572271277,30.3394038774272,-16.3865268648834));
#57811=CARTESIAN_POINT('Ctrl Pts',(2.47778480237176,29.8926993859692,-17.1128675875488));
#57812=CARTESIAN_POINT('Ctrl Pts',(2.66004324798223,29.6185503436459,-16.2842251711301));
#57813=CARTESIAN_POINT('Ctrl Pts',(2.07658934638655,30.3721820016165,-16.3795138210175));
#57814=CARTESIAN_POINT('Ctrl Pts',(2.53695510817887,29.9414486673533,-17.100584863834));
#57815=CARTESIAN_POINT('Ctrl Pts',(2.70153038913429,29.6528770266069,-16.2773908679428));
#57816=CARTESIAN_POINT('Ctrl Pts',(2.11515348080612,30.3949183678539,-16.3746953336256));
#57817=CARTESIAN_POINT('Ctrl Pts',(2.57581358773611,29.9745351098867,-17.0923032197876));
#57818=CARTESIAN_POINT('Ctrl Pts',(2.82421530443451,29.7575890425693,-16.2567120771395));
#57819=CARTESIAN_POINT('Ctrl Pts',(2.22956819594977,30.4651684504852,-16.3599495397914));
#57820=CARTESIAN_POINT('Ctrl Pts',(2.69072507829928,30.0754559176024,-17.0672065911949));
#57821=CARTESIAN_POINT('Ctrl Pts',(2.90364008546083,29.8297029496513,-16.2426922301433));
#57822=CARTESIAN_POINT('Ctrl Pts',(2.30547175408465,30.5154143020214,-16.3495803497904));
#57823=CARTESIAN_POINT('Ctrl Pts',(2.7651174356246,30.1449484959329,-17.0501405710026));
#57824=CARTESIAN_POINT('Ctrl Pts',(3.05823671500216,29.9780894969754,-16.2142950763844));
#57825=CARTESIAN_POINT('Ctrl Pts',(2.45531918886263,30.6220505261989,-16.3279618812435));
#57826=CARTESIAN_POINT('Ctrl Pts',(2.90991868602117,30.2879200951006,-17.0154679498268));
#57827=CARTESIAN_POINT('Ctrl Pts',(3.13340755103014,30.0543631118974,-16.1999176059517));
#57828=CARTESIAN_POINT('Ctrl Pts',(2.52928950864992,30.6782919897607,-16.316734700869));
#57829=CARTESIAN_POINT('Ctrl Pts',(2.98032663199793,30.3614000520084,-16.9978611399441));
#57830=CARTESIAN_POINT('Ctrl Pts',(3.27987015132021,30.210715992756,-16.1709005658607));
#57831=CARTESIAN_POINT('Ctrl Pts',(2.67504196758113,30.7964541736505,-16.2935360824409));
#57832=CARTESIAN_POINT('Ctrl Pts',(3.11750923246245,30.5120049089877,-16.9622167722053));
#57833=CARTESIAN_POINT('Ctrl Pts',(3.35116123035258,30.2907959175364,-16.156260881267));
#57834=CARTESIAN_POINT('Ctrl Pts',(2.74686657696321,30.8582478680463,-16.2815815826731));
#57835=CARTESIAN_POINT('Ctrl Pts',(3.18428324621236,30.5891304417996,-16.9441790683909));
#57836=CARTESIAN_POINT('Ctrl Pts',(3.55966298596679,30.5363244595009,-16.1120758578107));
#57837=CARTESIAN_POINT('Ctrl Pts',(2.95660210195659,31.049475646984,-16.2451814165979));
#57838=CARTESIAN_POINT('Ctrl Pts',(3.37957414633138,30.8255678671554,-16.8895639888451));
#57839=CARTESIAN_POINT('Ctrl Pts',(3.69152422416695,30.7070404100115,-16.0822670185369));
#57840=CARTESIAN_POINT('Ctrl Pts',(3.0935680110286,31.188233012752,-16.2194870411642));
#57841=CARTESIAN_POINT('Ctrl Pts',(3.50308054074258,30.9899200073615,-16.8524880403649));
#57842=CARTESIAN_POINT('Ctrl Pts',(3.84850625888578,30.9282217390845,-16.0449381752436));
#57843=CARTESIAN_POINT('Ctrl Pts',(3.2607646882954,31.3759330382798,-16.1859089389379));
#57844=CARTESIAN_POINT('Ctrl Pts',(3.6501160551046,31.2027958226833,-16.8057225066586));
#57845=CARTESIAN_POINT('Ctrl Pts',(3.87953256866694,30.9728856431268,-16.0374628392411));
#57846=CARTESIAN_POINT('Ctrl Pts',(3.29342662187892,31.4134934654484,-16.1792418772485));
#57847=CARTESIAN_POINT('Ctrl Pts',(3.67917651069663,31.2457796337213,-16.7963405521398));
#57848=CARTESIAN_POINT('Ctrl Pts',(3.94058434545197,31.0626285007038,-16.022571026142));
#57849=CARTESIAN_POINT('Ctrl Pts',(3.35787539127852,31.4893981914476,-16.1658790869078));
#57850=CARTESIAN_POINT('Ctrl Pts',(3.73635999288582,31.3321406834297,-16.7776156643026));
#57851=CARTESIAN_POINT('Ctrl Pts',(3.97063463723664,31.1077409109996,-16.0151487999533));
#57852=CARTESIAN_POINT('Ctrl Pts',(3.38969847622929,31.5277649299416,-16.1591781972395));
#57853=CARTESIAN_POINT('Ctrl Pts',(3.76450627188365,31.3755501268062,-16.7682655550614));
#57854=CARTESIAN_POINT('Ctrl Pts',(4.05941717087094,31.2437732562028,-15.9929626480247));
#57855=CARTESIAN_POINT('Ctrl Pts',(3.48351050644036,31.6435098716445,-16.1391308660064));
#57856=CARTESIAN_POINT('Ctrl Pts',(3.84766346564603,31.5064382047407,-16.7402628285028));
#57857=CARTESIAN_POINT('Ctrl Pts',(4.1167828254897,31.3353874419429,-15.978279338896));
#57858=CARTESIAN_POINT('Ctrl Pts',(3.54479499845881,31.7226089412723,-16.1256471238317));
#57859=CARTESIAN_POINT('Ctrl Pts',(3.90139438215665,31.5945757570875,-16.7216579368768));
#57860=CARTESIAN_POINT('Ctrl Pts',(4.28380788594745,31.6128203257638,-15.9346238064299));
#57861=CARTESIAN_POINT('Ctrl Pts',(3.72231473431664,31.9620905398297,-16.0855354656462));
#57862=CARTESIAN_POINT('Ctrl Pts',(4.05783658707824,31.8614425296594,-16.6661133987202));
#57863=CARTESIAN_POINT('Ctrl Pts',(4.3884148581878,31.8012197189447,-15.9060466319014));
#57864=CARTESIAN_POINT('Ctrl Pts',(3.83587999076983,32.1288604724229,-16.0584933410282));
#57865=CARTESIAN_POINT('Ctrl Pts',(4.15581556986088,32.0426166386068,-16.6294449643945));
#57866=CARTESIAN_POINT('Ctrl Pts',(4.58567200756637,32.1841943988468,-15.8503033618542));
#57867=CARTESIAN_POINT('Ctrl Pts',(4.05086579113235,32.4720636118671,-16.0050120263636));
#57868=CARTESIAN_POINT('Ctrl Pts',(4.34057433194744,32.4107939451974,-16.5572151315481));
#57869=CARTESIAN_POINT('Ctrl Pts',(4.67831544203237,32.3787729501169,-15.8231365471297));
#57870=CARTESIAN_POINT('Ctrl Pts',(4.152839616667,32.6484592325927,-15.9785118187779));
#57871=CARTESIAN_POINT('Ctrl Pts',(4.4273477970609,32.5978002916929,-16.5216528747722));
#57872=CARTESIAN_POINT('Ctrl Pts',(4.8526074647995,32.7736749069825,-15.7705575791359));
#57873=CARTESIAN_POINT('Ctrl Pts',(4.34531777018242,33.0096063680591,-15.9266467671527));
#57874=CARTESIAN_POINT('Ctrl Pts',(4.59059652338769,32.9772145356856,-16.4519928922655));
#57875=CARTESIAN_POINT('Ctrl Pts',(4.93425250225085,32.9740000075212,-15.7451448786754));
#57876=CARTESIAN_POINT('Ctrl Pts',(4.43629332140126,33.1943793675723,-15.9012113154715));
#57877=CARTESIAN_POINT('Ctrl Pts',(4.66706845943702,33.1696240761953,-16.4178945495574));
#57878=CARTESIAN_POINT('Ctrl Pts',(5.08711281849313,33.3801631316144,-15.6964237384943));
#57879=CARTESIAN_POINT('Ctrl Pts',(4.60722078767624,33.5714101157215,-15.8519572579756));
#57880=CARTESIAN_POINT('Ctrl Pts',(4.81024341123228,33.5596069464454,-16.3515167576984));
#57881=CARTESIAN_POINT('Ctrl Pts',(5.15832642133817,33.5860019204558,-15.6731147994769));
#57882=CARTESIAN_POINT('Ctrl Pts',(4.68757869339825,33.7637237962017,-15.8280627301349));
#57883=CARTESIAN_POINT('Ctrl Pts',(4.87694485739314,33.7571810298932,-16.3192367814774));
#57884=CARTESIAN_POINT('Ctrl Pts',(5.24097629968965,33.8467036990582,-15.6455255940079));
#57885=CARTESIAN_POINT('Ctrl Pts',(4.78213072770676,34.0107071083605,-15.7992314731343));
#57886=CARTESIAN_POINT('Ctrl Pts',(4.95435796666611,34.0073247840893,-16.2802535152582));
#57887=CARTESIAN_POINT('Ctrl Pts',(5.25719362818707,33.8990359684241,-15.6400829974654));
#57888=CARTESIAN_POINT('Ctrl Pts',(4.80054957120818,34.0598870173825,-15.793578275618));
#57889=CARTESIAN_POINT('Ctrl Pts',(4.96954775094229,34.0575332013725,-16.2725221393888));
#57890=CARTESIAN_POINT('Ctrl Pts',(5.28896226944923,34.0039467757404,-15.6293684812982));
#57891=CARTESIAN_POINT('Ctrl Pts',(4.83669604861666,34.1585897884646,-15.7824156043202));
#57892=CARTESIAN_POINT('Ctrl Pts',(4.99930350304212,34.1581771173989,-16.2572160497018));
#57893=CARTESIAN_POINT('Ctrl Pts',(5.30449626492683,34.0564670383293,-15.624102431784));
#57894=CARTESIAN_POINT('Ctrl Pts',(4.85440974566674,34.2080603224636,-15.7769108872987));
#57895=CARTESIAN_POINT('Ctrl Pts',(5.0138532509136,34.208556714705,-16.2496497575703));
#57896=CARTESIAN_POINT('Ctrl Pts',(5.3500593030389,34.2142207349753,-15.6085840212356));
#57897=CARTESIAN_POINT('Ctrl Pts',(4.90631386646526,34.3563731632076,-15.7606865923713));
#57898=CARTESIAN_POINT('Ctrl Pts',(5.05652937471128,34.3598665463188,-16.2272172272366));
#57899=CARTESIAN_POINT('Ctrl Pts',(5.37905002720047,34.3196469683343,-15.598611350614));
#57900=CARTESIAN_POINT('Ctrl Pts',(4.9396069834735,34.4560073796611,-15.7501529654412));
#57901=CARTESIAN_POINT('Ctrl Pts',(5.08368322108408,34.460967717809,-16.2126172924642));
#57902=CARTESIAN_POINT('Ctrl Pts',(5.46194078461707,34.6366877503115,-15.569862681342));
#57903=CARTESIAN_POINT('Ctrl Pts',(5.03466043352864,34.7544911380799,-15.7197631997284));
#57904=CARTESIAN_POINT('Ctrl Pts',(5.16132194699471,34.7649439115857,-16.1699328633975));
#57905=CARTESIAN_POINT('Ctrl Pts',(5.51176846617966,34.8490627904254,-15.5522551143952));
#57906=CARTESIAN_POINT('Ctrl Pts',(5.09291260313501,34.9564096240105,-15.7007118502892));
#57907=CARTESIAN_POINT('Ctrl Pts',(5.2079925027011,34.968490137579,-16.1429629194519));
#57908=CARTESIAN_POINT('Ctrl Pts',(5.60071361456991,35.275833071767,-15.5204457982229));
#57909=CARTESIAN_POINT('Ctrl Pts',(5.19800485837501,35.3631027727456,-15.6657772117967));
#57910=CARTESIAN_POINT('Ctrl Pts',(5.29130200819381,35.3773514622423,-16.0922807281473));
#57911=CARTESIAN_POINT('Ctrl Pts',(5.63983069135891,35.4902283652519,-15.5062438204224));
#57912=CARTESIAN_POINT('Ctrl Pts',(5.24514293116004,35.5680932299173,-15.649807466499));
#57913=CARTESIAN_POINT('Ctrl Pts',(5.32794059231136,35.5826666215459,-16.0685682530086));
#57914=CARTESIAN_POINT('Ctrl Pts',(5.70722219029865,35.9210809846202,-15.4815665394735));
#57915=CARTESIAN_POINT('Ctrl Pts',(5.32796042195972,35.9807456339375,-15.6213886714218));
#57916=CARTESIAN_POINT('Ctrl Pts',(5.39106210676183,35.9950907162295,-16.0247146511509));
#57917=CARTESIAN_POINT('Ctrl Pts',(5.73549725525296,36.1375381840345,-15.4710909455289));
#57918=CARTESIAN_POINT('Ctrl Pts',(5.36389926796403,36.1886130621991,-15.6088583771076));
#57919=CARTESIAN_POINT('Ctrl Pts',(5.41754563828522,36.2021995446388,-16.004573243818));
#57920=CARTESIAN_POINT('Ctrl Pts',(5.78078346060784,36.5726077638088,-15.4542268131215));
#57921=CARTESIAN_POINT('Ctrl Pts',(5.42398393004534,36.606935192749,-15.5876972584938));
#57922=CARTESIAN_POINT('Ctrl Pts',(5.45996247023453,36.6182830146743,-15.9682119674733));
#57923=CARTESIAN_POINT('Ctrl Pts',(5.7977963957715,36.7912198164816,-15.4478378834369));
#57924=CARTESIAN_POINT('Ctrl Pts',(5.44836047329696,36.8175859984048,-15.5789899469686));
#57925=CARTESIAN_POINT('Ctrl Pts',(5.47589745022953,36.8272573619824,-15.9519917284049));
#57926=CARTESIAN_POINT('Ctrl Pts',(5.81430843554853,37.1208676336436,-15.4416272457358));
#57927=CARTESIAN_POINT('Ctrl Pts',(5.47569053932407,37.1367087944884,-15.5691295274642));
#57928=CARTESIAN_POINT('Ctrl Pts',(5.49136327314324,37.1422120437367,-15.9308997542));
#57929=CARTESIAN_POINT('Ctrl Pts',(5.81830852011158,37.2310390122662,-15.4401195822918));
#57930=CARTESIAN_POINT('Ctrl Pts',(5.48324669152352,37.243039155561,-15.5663815273683));
#57931=CARTESIAN_POINT('Ctrl Pts',(5.49510990843326,37.2474462392647,-15.924409220868));
#57932=CARTESIAN_POINT('Ctrl Pts',(5.8219552680468,37.3967483415922,-15.4387447204924));
#57933=CARTESIAN_POINT('Ctrl Pts',(5.49218973652234,37.4033363287178,-15.5630995045285));
#57934=CARTESIAN_POINT('Ctrl Pts',(5.49852559552139,37.4056877138083,-15.9155248418178));
#57935=CARTESIAN_POINT('Ctrl Pts',(5.82277787197035,37.4520779924035,-15.4384344431652));
#57936=CARTESIAN_POINT('Ctrl Pts',(5.49476863526362,37.4567795900761,-15.5621468243714));
#57937=CARTESIAN_POINT('Ctrl Pts',(5.49929607838327,37.4585169113888,-15.9127047089119));
#57938=CARTESIAN_POINT('Ctrl Pts',(5.82361937406439,37.5625395576871,-15.438117035061));
#57939=CARTESIAN_POINT('Ctrl Pts',(5.49909810504416,37.5635003468084,-15.5605340956755));
#57940=CARTESIAN_POINT('Ctrl Pts',(5.50008426225533,37.5639723612738,-15.9073715669842));
#57941=CARTESIAN_POINT('Ctrl Pts',(5.82363950904436,37.6177133458351,-15.438109438589));
#57942=CARTESIAN_POINT('Ctrl Pts',(5.5008542982352,37.6168225419558,-15.5598720284282));
#57943=CARTESIAN_POINT('Ctrl Pts',(5.50010312136638,37.6166386057181,-15.9048561966123));
#57944=CARTESIAN_POINT('Ctrl Pts',(5.8217154307924,37.893294229626,-15.4388351940587));
#57945=CARTESIAN_POINT('Ctrl Pts',(5.50752491944064,37.881853217054,-15.5573104201885));
#57946=CARTESIAN_POINT('Ctrl Pts',(5.49830095467151,37.8796590971548,-15.8930435523112));
#57947=CARTESIAN_POINT('Ctrl Pts',(5.8137104043734,38.1128388502149,-15.4418594419708));
#57948=CARTESIAN_POINT('Ctrl Pts',(5.50636898532151,38.0944392377558,-15.5575651542258));
#57949=CARTESIAN_POINT('Ctrl Pts',(5.49080313325399,38.0890827853353,-15.886038511744));
#57950=CARTESIAN_POINT('Ctrl Pts',(5.7840049154644,38.5499825598019,-15.4530106720142));
#57951=CARTESIAN_POINT('Ctrl Pts',(5.48999166329811,38.5177567680441,-15.5630532663817));
#57952=CARTESIAN_POINT('Ctrl Pts',(5.46297981094671,38.5058340924418,-15.8771352552735));
#57953=CARTESIAN_POINT('Ctrl Pts',(5.76230703860224,38.7675819658764,-15.4611377904124));
#57954=CARTESIAN_POINT('Ctrl Pts',(5.47493356768806,38.7287614510696,-15.568229955048));
#57955=CARTESIAN_POINT('Ctrl Pts',(5.44265672992744,38.7131620074787,-15.8752371590965));
#57956=CARTESIAN_POINT('Ctrl Pts',(5.70407395336722,39.2006823460781,-15.4827163158072));
#57957=CARTESIAN_POINT('Ctrl Pts',(5.42972855746396,39.1486876692357,-15.5837780636752));
#57958=CARTESIAN_POINT('Ctrl Pts',(5.38811334519547,39.1255654423464,-15.8767726336669));
#57959=CARTESIAN_POINT('Ctrl Pts',(5.66754335828454,39.4161838894492,-15.4961678890182));
#57960=CARTESIAN_POINT('Ctrl Pts',(5.39972357971351,39.3578660216,-15.5941025574047));
#57961=CARTESIAN_POINT('Ctrl Pts',(5.35389735978674,39.3306414973316,-15.88020634219));
#57962=CARTESIAN_POINT('Ctrl Pts',(5.60039918974671,39.7377021629651,-15.5205056507883));
#57963=CARTESIAN_POINT('Ctrl Pts',(5.34213771584874,39.6706104721975,-15.6136918367253));
#57964=CARTESIAN_POINT('Ctrl Pts',(5.29100750584286,39.6364055190875,-15.8895273598811));
#57965=CARTESIAN_POINT('Ctrl Pts',(5.57595554966988,39.8445853883982,-15.5293116329089));
#57966=CARTESIAN_POINT('Ctrl Pts',(5.32093394283459,39.7743589127886,-15.6208743387635));
#57967=CARTESIAN_POINT('Ctrl Pts',(5.26811263571756,39.7380180145649,-15.8933294601772));
#57968=CARTESIAN_POINT('Ctrl Pts',(5.53599851525571,40.004450203368,-15.5435813267104));
#57969=CARTESIAN_POINT('Ctrl Pts',(5.28579906825781,39.929705256497,-15.632690927334));
#57970=CARTESIAN_POINT('Ctrl Pts',(5.23068731473301,39.8899479695032,-15.9000967087543));
#57971=CARTESIAN_POINT('Ctrl Pts',(5.5221305599358,40.0576617611033,-15.5485146750299));
#57972=CARTESIAN_POINT('Ctrl Pts',(5.27355459719845,39.9813594979742,-15.6367961486595));
#57973=CARTESIAN_POINT('Ctrl Pts',(5.2176980449392,39.9405097816184,-15.9025298069678));
#57974=CARTESIAN_POINT('Ctrl Pts',(5.50047699149048,40.1373603819414,-15.556182420383));
#57975=CARTESIAN_POINT('Ctrl Pts',(5.25432923497206,40.0587687077115,-15.6432168973992));
#57976=CARTESIAN_POINT('Ctrl Pts',(5.19741646594872,40.0162266424403,-15.9064481481372));
#57977=CARTESIAN_POINT('Ctrl Pts',(5.49311741536451,40.1639050501549,-15.5587828592327));
#57978=CARTESIAN_POINT('Ctrl Pts',(5.24778336468827,40.0845377385951,-15.6453990618431));
#57979=CARTESIAN_POINT('Ctrl Pts',(5.19052319892915,40.041442951149,-15.907799028716));
#57980=CARTESIAN_POINT('Ctrl Pts',(5.47814593729634,40.2168282263209,-15.5640605270417));
#57981=CARTESIAN_POINT('Ctrl Pts',(5.23443708951077,40.1359150171577,-15.649839332167));
#57982=CARTESIAN_POINT('Ctrl Pts',(5.17650032697911,40.0917133649177,-15.9105838634));
#57983=CARTESIAN_POINT('Ctrl Pts',(5.470529823742,40.2432224288697,-15.5667392494243));
#57984=CARTESIAN_POINT('Ctrl Pts',(5.22763310795184,40.1615391166161,-15.6520986436733));
#57985=CARTESIAN_POINT('Ctrl Pts',(5.16936677702167,40.1167823811518,-15.9120185729299));
#57986=CARTESIAN_POINT('Ctrl Pts',(5.40080286686056,40.4801601691466,-15.5912040190124));
#57987=CARTESIAN_POINT('Ctrl Pts',(5.1654386504834,40.3907259377088,-15.672707312104));
#57988=CARTESIAN_POINT('Ctrl Pts',(5.10405778192814,40.3418044912576,-15.9253090687417));
#57989=CARTESIAN_POINT('Ctrl Pts',(5.33043670111554,40.6864411445816,-15.6154875831029));
#57990=CARTESIAN_POINT('Ctrl Pts',(5.10156582395526,40.5911762940015,-15.6935809949587));
#57991=CARTESIAN_POINT('Ctrl Pts',(5.03815007775546,40.5375718116029,-15.9398148438705));
#57992=CARTESIAN_POINT('Ctrl Pts',(5.17171535959732,41.0898251595944,-15.6687704725657));
#57993=CARTESIAN_POINT('Ctrl Pts',(4.9558472522213,40.9828549133869,-15.739985220476));
#57994=CARTESIAN_POINT('Ctrl Pts',(4.88948546120424,40.9201248480408,-15.9738813871344));
#57995=CARTESIAN_POINT('Ctrl Pts',(5.08336558250042,41.2869305832741,-15.6977708167442));
#57996=CARTESIAN_POINT('Ctrl Pts',(4.87405064261176,41.1743746865059,-15.7655101753502));
#57997=CARTESIAN_POINT('Ctrl Pts',(4.80673360287453,41.1069127909073,-15.9934430495542));
#57998=CARTESIAN_POINT('Ctrl Pts',(4.88694399553687,41.671218731313,-15.7600251473423));
#57999=CARTESIAN_POINT('Ctrl Pts',(4.69092137437619,41.5474552367694,-15.8207627043341));
#58000=CARTESIAN_POINT('Ctrl Pts',(4.62275746195378,41.4708178044506,-16.0372007396695));
#58001=CARTESIAN_POINT('Ctrl Pts',(4.77888228918939,41.858405974228,-15.7932806671364));
#58002=CARTESIAN_POINT('Ctrl Pts',(4.58961749308463,41.7292760041513,-15.8504958068979));
#58003=CARTESIAN_POINT('Ctrl Pts',(4.5215426392795,41.6479391144314,-16.0613980705431));
#58004=CARTESIAN_POINT('Ctrl Pts',(4.64482519461143,42.0628061930575,-15.8327458139082));
#58005=CARTESIAN_POINT('Ctrl Pts',(4.46310917160174,41.9280541129356,-15.8860546410961));
#58006=CARTESIAN_POINT('Ctrl Pts',(4.39597952121523,41.8412001847982,-16.0909199817576));
#58007=CARTESIAN_POINT('Ctrl Pts',(4.62976965412125,42.0854096858801,-15.8371551458627));
#58008=CARTESIAN_POINT('Ctrl Pts',(4.44892446825342,41.9499886943975,-15.8900217942609));
#58009=CARTESIAN_POINT('Ctrl Pts',(4.38187791293436,41.8625697484028,-16.0942290007409));
#58010=CARTESIAN_POINT('Ctrl Pts',(4.59939878543121,42.1303067904093,-15.8460020502624));
#58011=CARTESIAN_POINT('Ctrl Pts',(4.42029652797858,41.9935550766478,-15.8979866657635));
#58012=CARTESIAN_POINT('Ctrl Pts',(4.35343136929109,41.9050117576583,-16.1008888977657));
#58013=CARTESIAN_POINT('Ctrl Pts',(4.58407427222009,42.1526144588579,-15.8504423301015));
#58014=CARTESIAN_POINT('Ctrl Pts',(4.40584455629757,42.0152010592343,-15.9019868666117));
#58015=CARTESIAN_POINT('Ctrl Pts',(4.3390778307107,41.9260974941438,-16.1042417996911));
#58016=CARTESIAN_POINT('Ctrl Pts',(4.53768208250935,42.2191142602777,-15.8638103017682));
#58017=CARTESIAN_POINT('Ctrl Pts',(4.36208642108868,42.0797067591165,-15.914033937939));
#58018=CARTESIAN_POINT('Ctrl Pts',(4.2956250910933,41.9889485291262,-16.1143660947964));
#58019=CARTESIAN_POINT('Ctrl Pts',(4.50619581303838,42.2628832431857,-15.8727851349316));
#58020=CARTESIAN_POINT('Ctrl Pts',(4.33235251838812,42.1221742523451,-15.9221344733298));
#58021=CARTESIAN_POINT('Ctrl Pts',(4.26613381932855,42.0303077037197,-16.121203084525));
#58022=CARTESIAN_POINT('Ctrl Pts',(4.41004926624052,42.3924912295783,-15.8998710702299));
#58023=CARTESIAN_POINT('Ctrl Pts',(4.24153152750805,42.2478448168248,-15.9465961576241));
#58024=CARTESIAN_POINT('Ctrl Pts',(4.1760792026318,42.1527559308387,-16.1419500461017));
#58025=CARTESIAN_POINT('Ctrl Pts',(4.34370225939985,42.4766322174293,-15.9181437877767));
#58026=CARTESIAN_POINT('Ctrl Pts',(4.17872361398144,42.3294747743511,-15.9631463234755));
#58027=CARTESIAN_POINT('Ctrl Pts',(4.11393600041315,42.2322165809747,-16.1560961451583));
#58028=CARTESIAN_POINT('Ctrl Pts',(4.13777251537753,42.7221794291726,-15.9733854419649));
#58029=CARTESIAN_POINT('Ctrl Pts',(3.98370692807761,42.5673833142134,-16.0132260504743));
#58030=CARTESIAN_POINT('Ctrl Pts',(3.92105414688791,42.4640154815466,-16.1992634768941));
#58031=CARTESIAN_POINT('Ctrl Pts',(3.99132195149594,42.8767293832158,-16.0107821043782));
#58032=CARTESIAN_POINT('Ctrl Pts',(3.84451111612512,42.7173047864165,-16.0473039779341));
#58033=CARTESIAN_POINT('Ctrl Pts',(3.78388281919657,42.6097890780496,-16.2290170151344));
#58034=CARTESIAN_POINT('Ctrl Pts',(3.75700972962784,43.0941951466418,-16.0667771043254));
#58035=CARTESIAN_POINT('Ctrl Pts',(3.62129524685035,42.9281698633173,-16.0984923203175));
#58036=CARTESIAN_POINT('Ctrl Pts',(3.56441682684187,42.8147476794126,-16.2742016702415));
#58037=CARTESIAN_POINT('Ctrl Pts',(3.67646144559015,43.1642860455141,-16.0854244903344));
#58038=CARTESIAN_POINT('Ctrl Pts',(3.54454660494019,42.9960786893441,-16.115553648241));
#58039=CARTESIAN_POINT('Ctrl Pts',(3.48897215266966,42.8807793342241,-16.2893548851606));
#58040=CARTESIAN_POINT('Ctrl Pts',(3.55180835016696,43.2656968454944,-16.1132389634261));
#58041=CARTESIAN_POINT('Ctrl Pts',(3.42566053370466,43.0943214418982,-16.1410401047175));
#58042=CARTESIAN_POINT('Ctrl Pts',(3.37221718759655,42.9762779466704,-16.3121000330166));
#58043=CARTESIAN_POINT('Ctrl Pts',(3.50961052575669,43.2988851470272,-16.122485966165));
#58044=CARTESIAN_POINT('Ctrl Pts',(3.38541262458361,43.1264600581356,-16.1495163495703));
#58045=CARTESIAN_POINT('Ctrl Pts',(3.33269305445803,43.0075246336688,-16.3196856337079));
#58046=CARTESIAN_POINT('Ctrl Pts',(3.4239361870611,43.3639679820918,-16.1408977680494));
#58047=CARTESIAN_POINT('Ctrl Pts',(3.30367271591507,43.189473362121,-16.1664034224739));
#58048=CARTESIAN_POINT('Ctrl Pts',(3.25244711732724,43.0687868973452,-16.3348347973778));
#58049=CARTESIAN_POINT('Ctrl Pts',(3.38069422093024,43.3956846955611,-16.1500121560905));
#58050=CARTESIAN_POINT('Ctrl Pts',(3.26240299114715,43.2201782549395,-16.1747684968875));
#58051=CARTESIAN_POINT('Ctrl Pts',(3.21194500033968,43.0986350973994,-16.3423568657999));
#58052=CARTESIAN_POINT('Ctrl Pts',(3.16247293665689,43.5501883769039,-16.1950777040967));
#58053=CARTESIAN_POINT('Ctrl Pts',(3.05423596689228,43.3696142664887,-16.2161210510762));
#58054=CARTESIAN_POINT('Ctrl Pts',(3.00755040891255,43.2440053764108,-16.3796546335878));
#58055=CARTESIAN_POINT('Ctrl Pts',(2.98147832252801,43.660776482398,-16.2295084233055));
#58056=CARTESIAN_POINT('Ctrl Pts',(2.88121816202138,43.4766418873115,-16.2478293654573));
#58057=CARTESIAN_POINT('Ctrl Pts',(2.83802377309921,43.3479542916528,-16.4084895185999));
#58058=CARTESIAN_POINT('Ctrl Pts',(2.70037397572554,43.8074863821001,-16.277807578224));
#58059=CARTESIAN_POINT('Ctrl Pts',(2.61232205384454,43.6184982166501,-16.2923899551782));
#58060=CARTESIAN_POINT('Ctrl Pts',(2.57473044561691,43.4857336160062,-16.4493217081974));
#58061=CARTESIAN_POINT('Ctrl Pts',(2.60506670587299,43.8531862697985,-16.2933497575293));
#58062=CARTESIAN_POINT('Ctrl Pts',(2.52114721824606,43.6626594710407,-16.3067415552332));
#58063=CARTESIAN_POINT('Ctrl Pts',(2.48546192830491,43.528628365131,-16.4625297245561));
#58064=CARTESIAN_POINT('Ctrl Pts',(2.41119452256951,43.9381353686842,-16.3231663545269));
#58065=CARTESIAN_POINT('Ctrl Pts',(2.3356478240054,43.7447042632128,-16.3342999073));
#58066=CARTESIAN_POINT('Ctrl Pts',(2.3038736575641,43.6083197721399,-16.4879921624111));
#58067=CARTESIAN_POINT('Ctrl Pts',(2.31262977609044,43.9773848957545,-16.3374408791774));
#58068=CARTESIAN_POINT('Ctrl Pts',(2.24131140491693,43.7825970865653,-16.3475093049691));
#58069=CARTESIAN_POINT('Ctrl Pts',(2.21155406016932,43.6451167254636,-16.5002466751902));
#58070=CARTESIAN_POINT('Ctrl Pts',(2.16227751834144,44.0313312810579,-16.3577844977291));
#58071=CARTESIAN_POINT('Ctrl Pts',(2.09738048924219,43.8346499499766,-16.3663562334774));
#58072=CARTESIAN_POINT('Ctrl Pts',(2.07072825413426,43.6956582712672,-16.5178019271295));
#58073=CARTESIAN_POINT('Ctrl Pts',(2.11174227376284,44.0484914663749,-16.3643876348749));
#58074=CARTESIAN_POINT('Ctrl Pts',(2.04900260649854,43.8512017716587,-16.3724769498617));
#58075=CARTESIAN_POINT('Ctrl Pts',(2.02339496711712,43.7117292100671,-16.523515913095));
#58076=CARTESIAN_POINT('Ctrl Pts',(2.03530194931424,44.072981459843,-16.3740100616474));
#58077=CARTESIAN_POINT('Ctrl Pts',(1.97581878875163,43.8748161029352,-16.3814021297576));
#58078=CARTESIAN_POINT('Ctrl Pts',(1.95179796907649,43.7346553851609,-16.5318661099767));
#58079=CARTESIAN_POINT('Ctrl Pts',(2.00971557668972,44.0809363660402,-16.3771704866985));
#58080=CARTESIAN_POINT('Ctrl Pts',(1.95132227885587,43.8824850165059,-16.3843344340238));
#58081=CARTESIAN_POINT('Ctrl Pts',(1.92783277153264,43.742100695679,-16.5346127099434));
#58082=CARTESIAN_POINT('Ctrl Pts',(1.95832824291746,44.0964258747234,-16.3833946525917));
#58083=CARTESIAN_POINT('Ctrl Pts',(1.90212235254287,43.8974148464812,-16.3901112587382));
#58084=CARTESIAN_POINT('Ctrl Pts',(1.87970138457326,43.7565946460749,-16.5400299284974));
#58085=CARTESIAN_POINT('Ctrl Pts',(1.93251110054407,44.1039650287676,-16.3864602701835));
#58086=CARTESIAN_POINT('Ctrl Pts',(1.87740326220016,43.9046802305651,-16.392957550475));
#58087=CARTESIAN_POINT('Ctrl Pts',(1.85552003909345,43.7636475423924,-16.5427021859492));
#58088=CARTESIAN_POINT('Ctrl Pts',(1.8030633147258,44.1405497707181,-16.4015192016935));
#58089=CARTESIAN_POINT('Ctrl Pts',(1.75346736507588,43.9399264952154,-16.4069429652539));
#58090=CARTESIAN_POINT('Ctrl Pts',(1.73427417901659,43.7978641021233,-16.5558492664266));
#58091=CARTESIAN_POINT('Ctrl Pts',(1.69906639420128,44.1660683153088,-16.4126226120353));
#58092=CARTESIAN_POINT('Ctrl Pts',(1.65387335486775,43.9644920355918,-16.417272571238));
#58093=CARTESIAN_POINT('Ctrl Pts',(1.63686659515066,43.8217027186776,-16.5656092158287));
#58094=CARTESIAN_POINT('Ctrl Pts',(1.49021426166529,44.2098252495483,-16.4329020282884));
#58095=CARTESIAN_POINT('Ctrl Pts',(1.45386135654879,44.0065631227143,-16.4361701532582));
#58096=CARTESIAN_POINT('Ctrl Pts',(1.44124751778221,43.862520976467,-16.5835644832772));
#58097=CARTESIAN_POINT('Ctrl Pts',(1.38535902634819,44.2280633796216,-16.4420780728859));
#58098=CARTESIAN_POINT('Ctrl Pts',(1.35343204203413,44.0240714574058,-16.4447394017829));
#58099=CARTESIAN_POINT('Ctrl Pts',(1.34303600264843,43.8795003686096,-16.5917598520244));
#58100=CARTESIAN_POINT('Ctrl Pts',(1.17479908853176,44.2573750378148,-16.4584628106134));
#58101=CARTESIAN_POINT('Ctrl Pts',(1.15176493152459,44.0521448192979,-16.4600782830589));
#58102=CARTESIAN_POINT('Ctrl Pts',(1.14581732809311,43.906712349358,-16.6065414193849));
#58103=CARTESIAN_POINT('Ctrl Pts',(1.06909438111656,44.2684484921629,-16.4656715398477));
#58104=CARTESIAN_POINT('Ctrl Pts',(1.05051664045048,44.0627110998794,-16.4668487116589));
#58105=CARTESIAN_POINT('Ctrl Pts',(1.04681016412825,43.9169448659429,-16.6131276573267));
#58106=CARTESIAN_POINT('Ctrl Pts',(0.856834555596582,44.2834493850702,-16.4780804888865));
#58107=CARTESIAN_POINT('Ctrl Pts',(0.847217272305147,44.0769219395685,-16.4785516187993));
#58108=CARTESIAN_POINT('Ctrl Pts',(0.847999308275245,43.9306827648361,-16.6246496409757));
#58109=CARTESIAN_POINT('Ctrl Pts',(0.750279450442107,44.2873769285557,-16.4832807449414));
#58110=CARTESIAN_POINT('Ctrl Pts',(0.745156101872444,44.0805664549735,-16.483484482518));
#58111=CARTESIAN_POINT('Ctrl Pts',(0.748195628510673,43.9341882452755,-16.62958541764));
#58112=CARTESIAN_POINT('Ctrl Pts',(0.58980086051462,44.2878495874714,-16.4895421642784));
#58113=CARTESIAN_POINT('Ctrl Pts',(0.591467911154747,44.0807865596362,-16.4894752008505));
#58114=CARTESIAN_POINT('Ctrl Pts',(0.597885103513613,43.9343461853688,-16.6357218580272));
#58115=CARTESIAN_POINT('Ctrl Pts',(0.536200263354332,44.2871032596941,-16.4913727887242));
#58116=CARTESIAN_POINT('Ctrl Pts',(0.540132926138202,44.0799845128224,-16.4912375073698));
#58117=CARTESIAN_POINT('Ctrl Pts',(0.547680687440361,43.9335480497144,-16.6375561481366));
#58118=CARTESIAN_POINT('Ctrl Pts',(0.455636014550893,44.284613337201,-16.4937296454446));
#58119=CARTESIAN_POINT('Ctrl Pts',(0.462979747202555,44.0774546459417,-16.4935249270376));
#58120=CARTESIAN_POINT('Ctrl Pts',(0.47222106046037,43.9310609294277,-16.6399872269088));
#58121=CARTESIAN_POINT('Ctrl Pts',(0.428754034222533,44.2835549068502,-16.4944504159164));
#58122=CARTESIAN_POINT('Ctrl Pts',(0.437235366462993,44.0763900837954,-16.4942280935165));
#58123=CARTESIAN_POINT('Ctrl Pts',(0.447042346105144,43.9300168543709,-16.6407441942414));
#58124=CARTESIAN_POINT('Ctrl Pts',(0.388389950057066,44.2816222765731,-16.4954337434013));
#58125=CARTESIAN_POINT('Ctrl Pts',(0.398580882778724,44.0744592385522,-16.4951933304063));
#58126=CARTESIAN_POINT('Ctrl Pts',(0.409235765892974,43.9281260198428,-16.6417991152495));
#58127=CARTESIAN_POINT('Ctrl Pts',(0.374928402732455,44.2809205658472,-16.4957452143992));
#58128=CARTESIAN_POINT('Ctrl Pts',(0.385689351820399,44.0737599283669,-16.4955001651808));
#58129=CARTESIAN_POINT('Ctrl Pts',(0.396627154075427,43.9274416182168,-16.6421373338812));
#58130=CARTESIAN_POINT('Ctrl Pts',(0.347991554057913,44.2794017185444,-16.4963354525741));
#58131=CARTESIAN_POINT('Ctrl Pts',(0.359893363301771,44.072249540534,-16.4960839175124));
#58132=CARTESIAN_POINT('Ctrl Pts',(0.371397047876984,43.9259641674669,-16.6427868545954));
#58133=CARTESIAN_POINT('Ctrl Pts',(0.334532328343637,44.2785856289167,-16.4966139069159));
#58134=CARTESIAN_POINT('Ctrl Pts',(0.347004279162573,44.0714394948401,-16.496360523009));
#58135=CARTESIAN_POINT('Ctrl Pts',(0.358790610672238,43.925172130238,-16.6430978003365));
#58136=CARTESIAN_POINT('Ctrl Pts',(0.321034048597817,44.2777095070773,-16.496876587392));
#58137=CARTESIAN_POINT('Ctrl Pts',(0.334078182671872,44.0705712895835,-16.4966227447236));
#58138=CARTESIAN_POINT('Ctrl Pts',(0.346147593727982,43.9243235322772,-16.6433959637249));
#58139=CARTESIAN_POINT('Ctrl Pts',(-0.962949743629567,23.7058553936807,
-16.4718768751861));
#58140=CARTESIAN_POINT('Ctrl Pts',(-0.492765517354465,23.7311233306727,
-16.4993627999076));
#58141=CARTESIAN_POINT('Ctrl Pts',(-0.492844382849881,23.7325958701808,
-16.9710247304714));
#58142=CARTESIAN_POINT('Ctrl Pts',(-0.953542544970481,23.5248859568717,
-16.4724268222023));
#58143=CARTESIAN_POINT('Ctrl Pts',(-0.483855216134323,23.5656632201722,
-16.4996141685673));
#58144=CARTESIAN_POINT('Ctrl Pts',(-0.484033232848877,23.5680782136333,
-16.9715913419337));
#58145=CARTESIAN_POINT('Ctrl Pts',(-0.935468634918637,23.344260801378,-16.4734824711073));
#58146=CARTESIAN_POINT('Ctrl Pts',(-0.466721831624295,23.4005201515163,
-16.5000965390465));
#58147=CARTESIAN_POINT('Ctrl Pts',(-0.467104505517941,23.4038735842938,
-16.9726789786417));
#58148=CARTESIAN_POINT('Ctrl Pts',(-0.89510523809019,23.0738487819855,-16.4757084274388));
#58149=CARTESIAN_POINT('Ctrl Pts',(-0.428567886035457,23.1537264435047,
-16.5010528910333));
#58150=CARTESIAN_POINT('Ctrl Pts',(-0.429298576219848,23.1580445293623,
-16.9749723845983));
#58151=CARTESIAN_POINT('Ctrl Pts',(-0.87943798870027,22.9837992435457,-16.4765564083283));
#58152=CARTESIAN_POINT('Ctrl Pts',(-0.413753117119786,23.0715250912475,
-16.5014098047918));
#58153=CARTESIAN_POINT('Ctrl Pts',(-0.414624019763036,23.0761813304592,
-16.9758460607511));
#58154=CARTESIAN_POINT('Ctrl Pts',(-0.857029346731565,22.871349346421,-16.4777280242054));
#58155=CARTESIAN_POINT('Ctrl Pts',(-0.392594063617177,22.9689868879305,
-16.501882689752));
#58156=CARTESIAN_POINT('Ctrl Pts',(-0.393635213114529,22.9739541736211,
-16.9770531781636));
#58157=CARTESIAN_POINT('Ctrl Pts',(-0.852405448376484,22.8488621194965,
-16.477967944935));
#58158=CARTESIAN_POINT('Ctrl Pts',(-0.388226665517808,22.9484751168198,
-16.5019786523467));
#58159=CARTESIAN_POINT('Ctrl Pts',(-0.389304289803603,22.953511244517,-16.9773003688871));
#58160=CARTESIAN_POINT('Ctrl Pts',(-0.842901150174904,22.8040262491542,
-16.4784568541402));
#58161=CARTESIAN_POINT('Ctrl Pts',(-0.379251273164189,22.9075837307647,
-16.5021720691143));
#58162=CARTESIAN_POINT('Ctrl Pts',(-0.380402193782386,22.9127513713192,
-16.9778040926919));
#58163=CARTESIAN_POINT('Ctrl Pts',(-0.838017665072762,22.7816617177292,
-16.4787060049652));
#58164=CARTESIAN_POINT('Ctrl Pts',(-0.374640213962693,22.8871893178798,
-16.5022695915681));
#58165=CARTESIAN_POINT('Ctrl Pts',(-0.37582813152086,22.892419983537,-16.9780607931916));
#58166=CARTESIAN_POINT('Ctrl Pts',(-0.822975496592716,22.7147273874846,
-16.4794663794692));
#58167=CARTESIAN_POINT('Ctrl Pts',(-0.360437617319141,22.8261502697624,
-16.5025636559244));
#58168=CARTESIAN_POINT('Ctrl Pts',(-0.361739050443223,22.8315706057323,
-16.9788442080374));
#58169=CARTESIAN_POINT('Ctrl Pts',(-0.812425165219932,22.6703168263289,
-16.4799905377545));
#58170=CARTESIAN_POINT('Ctrl Pts',(-0.350480426682779,22.7856681155344,
-16.5027616215283));
#58171=CARTESIAN_POINT('Ctrl Pts',(-0.351857199315679,22.7911973771194,
-16.9793842491552));
#58172=CARTESIAN_POINT('Ctrl Pts',(-0.757088938658021,22.4493146639893,
-16.4826812356247));
#58173=CARTESIAN_POINT('Ctrl Pts',(-0.298223330345641,22.5840652733162,
-16.5037483172792));
#58174=CARTESIAN_POINT('Ctrl Pts',(-0.300027133564499,22.5902863641164,
-16.9821564785501));
#58175=CARTESIAN_POINT('Ctrl Pts',(-0.704568880777145,22.2758671068484,
-16.485061716078));
#58176=CARTESIAN_POINT('Ctrl Pts',(-0.248694534639063,22.4261536301923,
-16.5045273833023));
#58177=CARTESIAN_POINT('Ctrl Pts',(-0.250834802041656,22.4326068013007,
-16.9846090911103));
#58178=CARTESIAN_POINT('Ctrl Pts',(-0.583383247271744,21.9355291968338,
-16.4897950586838));
#58179=CARTESIAN_POINT('Ctrl Pts',(-0.134788012211473,22.1169078656145,
-16.5056480962526));
#58180=CARTESIAN_POINT('Ctrl Pts',(-0.137327617879236,22.1232087702482,
-16.9894858582894));
#58181=CARTESIAN_POINT('Ctrl Pts',(-0.514717124843465,21.7686390767122,
-16.4921487116152));
#58182=CARTESIAN_POINT('Ctrl Pts',(-0.0703104071456902,21.965477603616,
-16.5059887383307));
#58183=CARTESIAN_POINT('Ctrl Pts',(-0.0730122532846286,21.9714905132742,
-16.9919108295178));
#58184=CARTESIAN_POINT('Ctrl Pts',(-0.399512762791793,21.5232549343589,
-16.4952073422415));
#58185=CARTESIAN_POINT('Ctrl Pts',(0.0373481064066343,21.7435521241675,
-16.5057799897692));
#58186=CARTESIAN_POINT('Ctrl Pts',(0.0348926376623413,21.7484140712811,
-16.9950621368967));
#58187=CARTESIAN_POINT('Ctrl Pts',(-0.359073410724847,21.4422868841008,
-16.4961472443844));
#58188=CARTESIAN_POINT('Ctrl Pts',(0.0751411787183878,21.6703115153897,
-16.5055887897801));
#58189=CARTESIAN_POINT('Ctrl Pts',(0.072769709688035,21.6748067697522,-16.996030518433));
#58190=CARTESIAN_POINT('Ctrl Pts',(-0.295310930681003,21.3220928627162,
-16.4973708014316));
#58191=CARTESIAN_POINT('Ctrl Pts',(0.134596754045265,21.5617672788568,-16.5050629722566));
#58192=CARTESIAN_POINT('Ctrl Pts',(0.132492130847063,21.5655395026313,-16.9972911481565));
#58193=CARTESIAN_POINT('Ctrl Pts',(-0.273539280243306,21.2822379645823,
-16.4977475258198));
#58194=CARTESIAN_POINT('Ctrl Pts',(0.154896674034376,21.5257721875215,-16.5048475037642));
#58195=CARTESIAN_POINT('Ctrl Pts',(0.152884306494302,21.5293077854622,-16.9976792871469));
#58196=CARTESIAN_POINT('Ctrl Pts',(-0.240097413338021,21.2227734744632,
-16.4982568025543));
#58197=CARTESIAN_POINT('Ctrl Pts',(0.18604366839339,21.472111121502,-16.504456559693));
#58198=CARTESIAN_POINT('Ctrl Pts',(0.184207260913047,21.4752491704785,-16.9982039940394));
#58199=CARTESIAN_POINT('Ctrl Pts',(-0.228819376074745,21.2030049605629,
-16.4984172542104));
#58200=CARTESIAN_POINT('Ctrl Pts',(0.196547253522777,21.4542711189745,-16.5043148697831));
#58201=CARTESIAN_POINT('Ctrl Pts',(0.19477070980231,21.4572777983998,-16.9983693072139));
#58202=CARTESIAN_POINT('Ctrl Pts',(-0.206000240323432,21.1635745131237,
-16.4987179532799));
#58203=CARTESIAN_POINT('Ctrl Pts',(0.217791152556636,21.4186966483038,-16.5040074771837));
#58204=CARTESIAN_POINT('Ctrl Pts',(0.216144000673567,21.4214319452995,-16.9986791167097));
#58205=CARTESIAN_POINT('Ctrl Pts',(-0.194452744209423,21.1439021274209,
-16.4988582584087));
#58206=CARTESIAN_POINT('Ctrl Pts',(0.228537608365471,21.4009527421141,-16.5038416501483));
#58207=CARTESIAN_POINT('Ctrl Pts',(0.226959835108923,21.4035479624256,-16.9988236728386));
#58208=CARTESIAN_POINT('Ctrl Pts',(-0.089617584523493,20.9678046097149,
-16.5000198041065));
#58209=CARTESIAN_POINT('Ctrl Pts',(0.326274277831968,21.2418141732983,-16.5022358569792));
#58210=CARTESIAN_POINT('Ctrl Pts',(0.325152528104813,21.2434593463896,-17.0000204094314));
#58211=CARTESIAN_POINT('Ctrl Pts',(0.0103895000608808,20.8173601426308,
-16.5003410554286));
#58212=CARTESIAN_POINT('Ctrl Pts',(0.419074339645924,21.1064783083436,-16.5000224206461));
#58213=CARTESIAN_POINT('Ctrl Pts',(0.418823056213946,21.1066916807028,-17.0003513900864));
#58214=CARTESIAN_POINT('Ctrl Pts',(0.223577828128103,20.5282445580889,-16.4988295294443));
#58215=CARTESIAN_POINT('Ctrl Pts',(0.616138593215655,20.8468543167526,-16.4934517294574));
#58216=CARTESIAN_POINT('Ctrl Pts',(0.618503542756773,20.8438593932758,-16.9987940467289));
#58217=CARTESIAN_POINT('Ctrl Pts',(0.336760364078229,20.3895745669501,-16.4969979144061));
#58218=CARTESIAN_POINT('Ctrl Pts',(0.720448287574235,20.7226376096344,-16.4890852353886));
#58219=CARTESIAN_POINT('Ctrl Pts',(0.724514711017868,20.7177957950236,-16.9969069228523));
#58220=CARTESIAN_POINT('Ctrl Pts',(0.576232686432668,20.1239652559013,-16.4903700268213));
#58221=CARTESIAN_POINT('Ctrl Pts',(0.940326943553951,20.4850026896863,-16.4775707284051));
#58222=CARTESIAN_POINT('Ctrl Pts',(0.948813807316047,20.4763328427083,-16.9900781771338));
#58223=CARTESIAN_POINT('Ctrl Pts',(0.702521851144169,19.9970253470419,-16.4855754457147));
#58224=CARTESIAN_POINT('Ctrl Pts',(1.0558985496554,20.3716874051054,-16.4704138841867));
#58225=CARTESIAN_POINT('Ctrl Pts',(1.06710115351391,20.3609329538988,-16.9851383009696));
#58226=CARTESIAN_POINT('Ctrl Pts',(0.868773037863646,19.8458702850025,-16.4771460462422));
#58227=CARTESIAN_POINT('Ctrl Pts',(1.20728915622331,20.2370055044214,-16.4592899829426));
#58228=CARTESIAN_POINT('Ctrl Pts',(1.22281848263862,20.2235192945973,-16.9764534578773));
#58229=CARTESIAN_POINT('Ctrl Pts',(0.902443746971063,19.816016149053,-16.4753379800747));
#58230=CARTESIAN_POINT('Ctrl Pts',(1.23797338983554,20.2103694135477,-16.4569512657965));
#58231=CARTESIAN_POINT('Ctrl Pts',(1.25435577897425,20.1963791777396,-16.974590600823));
#58232=CARTESIAN_POINT('Ctrl Pts',(0.953587295856246,19.7718065477056,-16.4724303864898));
#58233=CARTESIAN_POINT('Ctrl Pts',(1.28453203163021,20.1709385549961,-16.4532690756911));
#58234=CARTESIAN_POINT('Ctrl Pts',(1.30225881653627,20.1561886407066,-16.971594896244));
#58235=CARTESIAN_POINT('Ctrl Pts',(0.970754191649368,19.7571546013071,-16.4714278213924));
#58236=CARTESIAN_POINT('Ctrl Pts',(1.30015758473307,20.157868088241,-16.452011212648));
#58237=CARTESIAN_POINT('Ctrl Pts',(1.31833799903477,20.1428686926593,-16.9705619498875));
#58238=CARTESIAN_POINT('Ctrl Pts',(1.00522776483883,19.7281045215425,-16.4693598939589));
#58239=CARTESIAN_POINT('Ctrl Pts',(1.33152367544567,20.1319543908634,-16.4494410173175));
#58240=CARTESIAN_POINT('Ctrl Pts',(1.35062728897796,20.1164595357428,-16.9684313566742));
#58241=CARTESIAN_POINT('Ctrl Pts',(1.02253286102999,19.7137073645744,-16.4682946770178));
#58242=CARTESIAN_POINT('Ctrl Pts',(1.34726260060578,20.1191123389068,-16.4481288375936));
#58243=CARTESIAN_POINT('Ctrl Pts',(1.36683591525823,20.1033712143075,-16.9673338599297));
#58244=CARTESIAN_POINT('Ctrl Pts',(1.10939730941571,19.6423569831041,-16.4628091753718));
#58245=CARTESIAN_POINT('Ctrl Pts',(1.42629119516503,20.0554244701247,-16.441425558252));
#58246=CARTESIAN_POINT('Ctrl Pts',(1.4481965373725,20.0385072470155,-16.9616821277774));
#58247=CARTESIAN_POINT('Ctrl Pts',(1.17997289092976,19.5873087525872,-16.4579107068088));
#58248=CARTESIAN_POINT('Ctrl Pts',(1.4903494741532,20.0063372584577,-16.4356263390571));
#58249=CARTESIAN_POINT('Ctrl Pts',(1.51430037239319,19.9884634129435,-16.9566352189892));
#58250=CARTESIAN_POINT('Ctrl Pts',(1.39486926268553,19.4281362425253,-16.4415626740924));
#58251=CARTESIAN_POINT('Ctrl Pts',(1.68530301764386,19.8642142740128,-16.4168034493466));
#58252=CARTESIAN_POINT('Ctrl Pts',(1.71558067464331,19.8437611662803,-16.9397917847999));
#58253=CARTESIAN_POINT('Ctrl Pts',(1.54235226719088,19.3299705812408,-16.4284621948059));
#58254=CARTESIAN_POINT('Ctrl Pts',(1.81854043497645,19.7766504246625,-16.4023921233297));
#58255=CARTESIAN_POINT('Ctrl Pts',(1.85371899319303,19.7545196774371,-16.9262943189646));
#58256=CARTESIAN_POINT('Ctrl Pts',(1.8455081137815,19.1492250077106,-16.3971741591057));
#58257=CARTESIAN_POINT('Ctrl Pts',(2.09201064403488,19.6148487582272,-16.3692914888457));
#58258=CARTESIAN_POINT('Ctrl Pts',(2.13766655088791,19.5902055590468,-16.8940581558081));
#58259=CARTESIAN_POINT('Ctrl Pts',(2.00118134550501,19.0666455566031,-16.3789878356581));
#58260=CARTESIAN_POINT('Ctrl Pts',(2.23204313940034,19.5407583231452,-16.3506228147975));
#58261=CARTESIAN_POINT('Ctrl Pts',(2.28347615445228,19.5151333486988,-16.8753207313665));
#58262=CARTESIAN_POINT('Ctrl Pts',(2.24082421386082,18.9545554863542,-16.3473300317566));
#58263=CARTESIAN_POINT('Ctrl Pts',(2.44755457756016,19.4395071081516,-16.3189516367199));
#58264=CARTESIAN_POINT('Ctrl Pts',(2.50793498547555,19.4132333079427,-16.8427035993773));
#58265=CARTESIAN_POINT('Ctrl Pts',(2.32172912386916,18.9191586223815,-16.3360470573507));
#58266=CARTESIAN_POINT('Ctrl Pts',(2.52026069725735,19.4074307794645,-16.3077882731722));
#58267=CARTESIAN_POINT('Ctrl Pts',(2.58371367100673,19.3810543481895,-16.8310787173966));
#58268=CARTESIAN_POINT('Ctrl Pts',(2.42415296888238,18.8774057450501,-16.3209653852811));
#58269=CARTESIAN_POINT('Ctrl Pts',(2.61232353439924,19.3694170191855,-16.2930124644539));
#58270=CARTESIAN_POINT('Ctrl Pts',(2.67964782784832,19.3430971951672,-16.8155400254028));
#58271=CARTESIAN_POINT('Ctrl Pts',(2.44470241052432,18.8691798998893,-16.3179001338654));
#58272=CARTESIAN_POINT('Ctrl Pts',(2.63079004346867,19.3619205223288,-16.2900170229615));
#58273=CARTESIAN_POINT('Ctrl Pts',(2.69889523418508,19.3356191558291,-16.8123818878633));
#58274=CARTESIAN_POINT('Ctrl Pts',(2.48593111009814,18.8529788338351,-16.3116700914));
#58275=CARTESIAN_POINT('Ctrl Pts',(2.6678392301345,19.3471377665628,-16.2839429469447));
#58276=CARTESIAN_POINT('Ctrl Pts',(2.7375116377121,19.3208909170966,-16.8059630564883));
#58277=CARTESIAN_POINT('Ctrl Pts',(2.50661987329755,18.8450002475771,-16.3085037647573));
#58278=CARTESIAN_POINT('Ctrl Pts',(2.68642985951431,19.3398486136801,-16.2808629383133));
#58279=CARTESIAN_POINT('Ctrl Pts',(2.75688953799591,19.3136376584055,-16.8027007808385));
#58280=CARTESIAN_POINT('Ctrl Pts',(2.5686809342295,18.821516920274,-16.2988843543115));
#58281=CARTESIAN_POINT('Ctrl Pts',(2.74219268886266,19.3183677676536,-16.2715271448004));
#58282=CARTESIAN_POINT('Ctrl Pts',(2.81501834153598,19.2922891838504,-16.7927898737225));
#58283=CARTESIAN_POINT('Ctrl Pts',(2.61012992508159,18.8064320620533,-16.2922985348497));
#58284=CARTESIAN_POINT('Ctrl Pts',(2.77943541677509,19.3045303867492,-16.2651626675075));
#58285=CARTESIAN_POINT('Ctrl Pts',(2.85384107841252,19.2785756790292,-16.7860044845856));
#58286=CARTESIAN_POINT('Ctrl Pts',(2.81773937785444,18.7338190214716,-16.2584950468795));
#58287=CARTESIAN_POINT('Ctrl Pts',(2.96587020075137,19.2377636805501,-16.2326478240223));
#58288=CARTESIAN_POINT('Ctrl Pts',(3.04829616661998,19.2125638384852,-16.751176651373));
#58289=CARTESIAN_POINT('Ctrl Pts',(2.9849895752519,18.6847044470942,-16.2286549196291));
#58290=CARTESIAN_POINT('Ctrl Pts',(3.11604918687771,19.1919225453077,-16.2043747173323));
#58291=CARTESIAN_POINT('Ctrl Pts',(3.20494920623192,19.1679142333196,-16.7204322819396));
#58292=CARTESIAN_POINT('Ctrl Pts',(3.32161623394242,18.6036838578296,-16.1631144542047));
#58293=CARTESIAN_POINT('Ctrl Pts',(3.41910319125249,19.1146585110534,-16.1428992719901));
#58294=CARTESIAN_POINT('Ctrl Pts',(3.52024682897757,19.0942591651346,-16.6529057512598));
#58295=CARTESIAN_POINT('Ctrl Pts',(3.49099316674984,18.5717797729774,-16.1274145820174));
#58296=CARTESIAN_POINT('Ctrl Pts',(3.5716609663928,19.083259988654,-16.1097791546225));
#58297=CARTESIAN_POINT('Ctrl Pts',(3.67889185273297,19.0652554551678,-16.6161240713731));
#58298=CARTESIAN_POINT('Ctrl Pts',(3.74656986701161,18.5366323538023,-16.069251626303));
#58299=CARTESIAN_POINT('Ctrl Pts',(3.80309044573612,19.0468400841815,-16.0560272802084));
#58300=CARTESIAN_POINT('Ctrl Pts',(3.91827493418733,19.033303258113,-16.5561986123435));
#58301=CARTESIAN_POINT('Ctrl Pts',(3.83201461596044,18.5270381829345,-16.049094870664));
#58302=CARTESIAN_POINT('Ctrl Pts',(3.88043400857609,19.0365067070544,-16.0374888868254));
#58303=CARTESIAN_POINT('Ctrl Pts',(3.99830581044114,19.0245812847932,-16.5354310500837));
#58304=CARTESIAN_POINT('Ctrl Pts',(3.9605555485118,18.5158358162941,-16.017676026607));
#58305=CARTESIAN_POINT('Ctrl Pts',(3.99711396115319,19.0237071198211,-16.0086240190836));
#58306=CARTESIAN_POINT('Ctrl Pts',(4.11870224954153,19.0143973144301,-16.503060126001));
#58307=CARTESIAN_POINT('Ctrl Pts',(4.00346486557186,18.5126333940285,-16.0070057718171));
#58308=CARTESIAN_POINT('Ctrl Pts',(4.03605994925758,19.019895083143,-15.9988412256294));
#58309=CARTESIAN_POINT('Ctrl Pts',(4.15889278554975,19.011486021175,-16.4920665324453));
#58310=CARTESIAN_POINT('Ctrl Pts',(4.08940780911621,18.5072956852501,-15.9852653553081));
#58311=CARTESIAN_POINT('Ctrl Pts',(4.11414010512615,19.0131810195212,-15.9789257486132));
#58312=CARTESIAN_POINT('Ctrl Pts',(4.23939029066013,19.0066335576006,-16.4696673198694));
#58313=CARTESIAN_POINT('Ctrl Pts',(4.13245806836038,18.5051597914318,-15.9741908394575));
#58314=CARTESIAN_POINT('Ctrl Pts',(4.15328411493104,19.0102768074715,-15.9687909906719));
#58315=CARTESIAN_POINT('Ctrl Pts',(4.27971283869093,19.0046918351941,-16.4582572149842));
#58316=CARTESIAN_POINT('Ctrl Pts',(4.34784672550312,18.4971683714463,-15.9178500886953));
#58317=CARTESIAN_POINT('Ctrl Pts',(4.3487542282718,18.9980972539458,-15.9174161894257));
#58318=CARTESIAN_POINT('Ctrl Pts',(4.4814542353807,18.9974269049179,-16.4002091813211));
#58319=CARTESIAN_POINT('Ctrl Pts',(4.51834575570717,18.4994317728118,-15.8702720675625));
#58320=CARTESIAN_POINT('Ctrl Pts',(4.50442609142234,18.9957318186494,-15.8740794573458));
#58321=CARTESIAN_POINT('Ctrl Pts',(4.64115026261982,18.9994845360441,-16.3511894124623));
#58322=CARTESIAN_POINT('Ctrl Pts',(4.85588770099964,18.5202816685198,-15.7702675469788));
#58323=CARTESIAN_POINT('Ctrl Pts',(4.81424862806617,19.0054597207642,-15.7829152581971));
#58324=CARTESIAN_POINT('Ctrl Pts',(4.95730518812699,19.0184389728909,-16.2481544747099));
#58325=CARTESIAN_POINT('Ctrl Pts',(5.02293020096387,18.5388709869828,-15.717840780607));
#58326=CARTESIAN_POINT('Ctrl Pts',(4.96817008474715,19.0174140221494,-15.7352002323915));
#58327=CARTESIAN_POINT('Ctrl Pts',(5.11376369695387,19.0353383433437,-16.1941390305004));
#58328=CARTESIAN_POINT('Ctrl Pts',(5.35366345256434,18.5918857067752,-15.6082873578935));
#58329=CARTESIAN_POINT('Ctrl Pts',(5.27463071593156,19.05568949738,-15.6352352679861));
#58330=CARTESIAN_POINT('Ctrl Pts',(5.42354133961961,19.0835335214419,-16.0812658326074));
#58331=CARTESIAN_POINT('Ctrl Pts',(5.51735404460432,18.626311704008,-15.5511604175382));
#58332=CARTESIAN_POINT('Ctrl Pts',(5.42697409841425,19.0818325558241,-15.5831012458257));
#58333=CARTESIAN_POINT('Ctrl Pts',(5.57686032344895,19.1148298694965,-16.0224077860923));
#58334=CARTESIAN_POINT('Ctrl Pts',(5.71990424855873,18.67921397641,-15.4769039866353));
#58335=CARTESIAN_POINT('Ctrl Pts',(5.61739054976128,19.1238638166436,-15.514780928748));
#58336=CARTESIAN_POINT('Ctrl Pts',(5.76657673742069,19.1629228269299,-15.9459011766186));
#58337=CARTESIAN_POINT('Ctrl Pts',(5.7603110112591,18.6902890021976,-15.4619103121913));
#58338=CARTESIAN_POINT('Ctrl Pts',(5.65525437053189,19.1326840835,-15.5010398404495));
#58339=CARTESIAN_POINT('Ctrl Pts',(5.80442328554253,19.1729910285574,-15.9304531518085));
#58340=CARTESIAN_POINT('Ctrl Pts',(5.82076645659554,18.7076461532893,-15.4392079207446));
#58341=CARTESIAN_POINT('Ctrl Pts',(5.7120216468109,19.1466132281685,-15.4802028149947));
#58342=CARTESIAN_POINT('Ctrl Pts',(5.86104821118419,19.1887702511317,-15.9070628142843));
#58343=CARTESIAN_POINT('Ctrl Pts',(5.84090083204721,18.7135586164393,-15.431601930293));
#58344=CARTESIAN_POINT('Ctrl Pts',(5.73092530850596,19.1513689910166,-15.4732248266298));
#58345=CARTESIAN_POINT('Ctrl Pts',(5.87990685170539,19.1941452156697,-15.8992263409633));
#58346=CARTESIAN_POINT('Ctrl Pts',(5.88102767187931,18.7256047794529,-15.4163541146221));
#58347=CARTESIAN_POINT('Ctrl Pts',(5.76862341141302,19.1610883165219,-15.4592309087857));
#58348=CARTESIAN_POINT('Ctrl Pts',(5.91749121334782,19.2050962692109,-15.8835164738311));
#58349=CARTESIAN_POINT('Ctrl Pts',(5.90102969963314,18.7317411147533,-15.408708735978));
#58350=CARTESIAN_POINT('Ctrl Pts',(5.78742667675602,19.1660535865446,-15.4522118926581));
#58351=CARTESIAN_POINT('Ctrl Pts',(5.93622589191204,19.2106747537697,-15.8756394187103));
#58352=CARTESIAN_POINT('Ctrl Pts',(6.00073572818559,18.7629847662334,-15.3703764930614));
#58353=CARTESIAN_POINT('Ctrl Pts',(5.88100137903186,19.1913491554074,-15.4170877663835));
#58354=CARTESIAN_POINT('Ctrl Pts',(6.0296144427393,19.2390780635469,-15.8361456018249));
#58355=CARTESIAN_POINT('Ctrl Pts',(6.07952793866853,18.7897768131789,-15.3393735694147));
#58356=CARTESIAN_POINT('Ctrl Pts',(5.95530612330359,19.2133034465851,-15.3885782624779));
#58357=CARTESIAN_POINT('Ctrl Pts',(6.10341429757601,19.2634344611989,-15.8042032023619));
#58358=CARTESIAN_POINT('Ctrl Pts',(6.3130827298411,18.875408878203,-15.2454305378321));
#58359=CARTESIAN_POINT('Ctrl Pts',(6.17541857033644,19.2839556861349,-15.3023083477907));
#58360=CARTESIAN_POINT('Ctrl Pts',(6.32217081560629,19.3412817673883,-15.7074134345399));
#58361=CARTESIAN_POINT('Ctrl Pts',(6.46502925485296,18.939491446264,-15.1815553755486));
#58362=CARTESIAN_POINT('Ctrl Pts',(6.31979410155795,19.3377274535367,-15.2433154114145));
#58363=CARTESIAN_POINT('Ctrl Pts',(6.46448985405949,19.3995386285318,-15.6416026748871));
#58364=CARTESIAN_POINT('Ctrl Pts',(6.76176840236203,19.0812662510744,-15.0517346163669));
#58365=CARTESIAN_POINT('Ctrl Pts',(6.60303555768087,19.4585649747456,-15.1229332761854));
#58366=CARTESIAN_POINT('Ctrl Pts',(6.74242730949661,19.5284247765807,-15.5078479818444));
#58367=CARTESIAN_POINT('Ctrl Pts',(6.90656044807258,19.1589588891342,-14.985788123841));
#58368=CARTESIAN_POINT('Ctrl Pts',(6.74191080864818,19.5254379131911,-15.0615983721264));
#58369=CARTESIAN_POINT('Ctrl Pts',(6.87804518597047,19.5990544270626,-15.439903124207));
#58370=CARTESIAN_POINT('Ctrl Pts',(7.11851697824708,19.2857408919594,-14.8856582575188));
#58371=CARTESIAN_POINT('Ctrl Pts',(6.94669094873197,19.6362246024488,-14.967804995196));
#58372=CARTESIAN_POINT('Ctrl Pts',(7.07657194161257,19.7143107625128,-15.3367390395514));
#58373=CARTESIAN_POINT('Ctrl Pts',(7.18829589041354,19.3297120059879,-14.8520803094002));
#58374=CARTESIAN_POINT('Ctrl Pts',(7.01403806331814,19.6746887916144,-14.936401435585));
#58375=CARTESIAN_POINT('Ctrl Pts',(7.14192959263245,19.7542844918657,-15.3021435844138));
#58376=CARTESIAN_POINT('Ctrl Pts',(7.29165902215419,19.3982694262532,-14.8014587300021));
#58377=CARTESIAN_POINT('Ctrl Pts',(7.11415554816123,19.7350433954885,-14.8888967056587));
#58378=CARTESIAN_POINT('Ctrl Pts',(7.23874353497939,19.8166094030417,-15.249988027825));
#58379=CARTESIAN_POINT('Ctrl Pts',(7.3258957750402,19.4215555778275,-14.784542462985));
#58380=CARTESIAN_POINT('Ctrl Pts',(7.14729834641863,19.7555520830343,-14.8730341341912));
#58381=CARTESIAN_POINT('Ctrl Pts',(7.27081101338128,19.8377786262931,-15.2325591498893));
#58382=CARTESIAN_POINT('Ctrl Pts',(7.39393376089708,19.4690038300525,-14.7506334876184));
#58383=CARTESIAN_POINT('Ctrl Pts',(7.21322647966689,19.797430733529,-14.8412096765173));
#58384=CARTESIAN_POINT('Ctrl Pts',(7.33453804573537,19.8809133897312,-15.1976226366084));
#58385=CARTESIAN_POINT('Ctrl Pts',(7.42775939794765,19.4931849686784,-14.7336281269098));
#58386=CARTESIAN_POINT('Ctrl Pts',(7.24603686392702,19.818815013828,-14.8252361070978));
#58387=CARTESIAN_POINT('Ctrl Pts',(7.36622045719149,19.9028962373553,-15.180101965099));
#58388=CARTESIAN_POINT('Ctrl Pts',(7.59506589867206,19.6157601057687,-14.6488051829882));
#58389=CARTESIAN_POINT('Ctrl Pts',(7.40770361714788,19.9269175872,-14.745870258467));
#58390=CARTESIAN_POINT('Ctrl Pts',(7.52292625224057,20.0143281505988,-15.0927086470378));
#58391=CARTESIAN_POINT('Ctrl Pts',(7.72362179982455,19.7195008596405,-14.5813365909781));
#58392=CARTESIAN_POINT('Ctrl Pts',(7.53309970113241,20.0194651615337,-14.6822094135442));
#58393=CARTESIAN_POINT('Ctrl Pts',(7.64333672678021,20.1086379031159,-15.0231955640876));
#58394=CARTESIAN_POINT('Ctrl Pts',(7.97062286550307,19.9382205720063,-14.4477985043873));
#58395=CARTESIAN_POINT('Ctrl Pts',(7.77465365444886,20.2159950446239,-14.5558500950358));
#58396=CARTESIAN_POINT('Ctrl Pts',(7.87468756705251,20.3074739578748,-14.8856108938969));
#58397=CARTESIAN_POINT('Ctrl Pts',(8.08906736132104,20.0531994360158,-14.3817276587201));
#58398=CARTESIAN_POINT('Ctrl Pts',(7.89097239699678,20.3198807121421,-14.493112481288));
#58399=CARTESIAN_POINT('Ctrl Pts',(7.98562730607927,20.4120001735958,-14.8175379122407));
#58400=CARTESIAN_POINT('Ctrl Pts',(8.31600323145087,20.294652390103,-14.2517083706198));
#58401=CARTESIAN_POINT('Ctrl Pts',(8.11429680827963,20.5393096561358,-14.3693578331021));
#58402=CARTESIAN_POINT('Ctrl Pts',(8.19818430429942,20.6315028094719,-14.6835786686257));
#58403=CARTESIAN_POINT('Ctrl Pts',(8.42449547871763,20.4211244360891,-14.1877579569348));
#58404=CARTESIAN_POINT('Ctrl Pts',(8.22147030516298,20.6547792674814,-14.3082854478819));
#58405=CARTESIAN_POINT('Ctrl Pts',(8.29980237977681,20.7464773718416,-14.6176903733931));
#58406=CARTESIAN_POINT('Ctrl Pts',(8.57965570414123,20.6199525825303,-14.0940823744386));
#58407=CARTESIAN_POINT('Ctrl Pts',(8.37539273565275,20.8376518525986,-14.2184166621781));
#58408=CARTESIAN_POINT('Ctrl Pts',(8.44513150955405,20.9272301946537,-14.5211761516265));
#58409=CARTESIAN_POINT('Ctrl Pts',(8.63011026247902,20.6877520189069,-14.0632335704244));
#58410=CARTESIAN_POINT('Ctrl Pts',(8.42538599398931,20.8999711961408,-14.1888588770955));
#58411=CARTESIAN_POINT('Ctrl Pts',(8.49238921931927,20.9888660332051,-14.4893925398783));
#58412=CARTESIAN_POINT('Ctrl Pts',(8.70385476035904,20.7918332707026,-14.0176227553152));
#58413=CARTESIAN_POINT('Ctrl Pts',(8.49861509669621,20.9959548800499,-14.1450582060422));
#58414=CARTESIAN_POINT('Ctrl Pts',(8.56146119773943,21.0834853334181,-14.442399585989));
#58415=CARTESIAN_POINT('Ctrl Pts',(8.72811318594382,20.8269242967422,-14.0025296682918));
#58416=CARTESIAN_POINT('Ctrl Pts',(8.52268865375042,21.0283052437927,-14.130573551022));
#58417=CARTESIAN_POINT('Ctrl Pts',(8.58418258654386,21.1153862597525,-14.4268491348457));
#58418=CARTESIAN_POINT('Ctrl Pts',(8.77597501193154,20.897920431518,-13.9725824201542));
#58419=CARTESIAN_POINT('Ctrl Pts',(8.5702088349925,21.0938179609117,-14.1018188553834));
#58420=CARTESIAN_POINT('Ctrl Pts',(8.62901184306147,21.179928186994,-14.3959943990639));
#58421=CARTESIAN_POINT('Ctrl Pts',(8.7994896585319,20.9336941025988,-13.9577838001673));
#58422=CARTESIAN_POINT('Ctrl Pts',(8.59357050615549,21.1268592854661,-14.0876006312119));
#58423=CARTESIAN_POINT('Ctrl Pts',(8.65103657958592,21.2124496995907,-14.3807473380954));
#58424=CARTESIAN_POINT('Ctrl Pts',(8.91495935746604,21.1138958131933,-13.8847199993329));
#58425=CARTESIAN_POINT('Ctrl Pts',(8.70792670494221,21.2928426773794,-14.0176222210528));
#58426=CARTESIAN_POINT('Ctrl Pts',(8.75919001035479,21.3762694014718,-14.305469494962));
#58427=CARTESIAN_POINT('Ctrl Pts',(9.00065683266863,21.2623657685385,-13.8292130781874));
#58428=CARTESIAN_POINT('Ctrl Pts',(8.79340445777157,21.4305988476776,-13.9640890064058));
#58429=CARTESIAN_POINT('Ctrl Pts',(8.83945761419094,21.5112420614924,-14.2482805529682));
#58430=CARTESIAN_POINT('Ctrl Pts',(9.15871068236081,21.5682334421585,-13.7250492319199));
#58431=CARTESIAN_POINT('Ctrl Pts',(8.95109569231193,21.7151215946974,-13.8635721361939));
#58432=CARTESIAN_POINT('Ctrl Pts',(8.98749702761635,21.789303528528,-14.140960241944));
#58433=CARTESIAN_POINT('Ctrl Pts',(9.23106853128776,21.7256297738407,-13.6763903437594));
#58434=CARTESIAN_POINT('Ctrl Pts',(9.02351685850879,21.8619866213685,-13.8164716865597));
#58435=CARTESIAN_POINT('Ctrl Pts',(9.05527021632604,21.9323910758609,-14.0908268477781));
#58436=CARTESIAN_POINT('Ctrl Pts',(9.36200027235301,22.0499603000645,-13.5870979228432));
#58437=CARTESIAN_POINT('Ctrl Pts',(9.15454270838474,22.1651688960518,-13.7300319644641));
#58438=CARTESIAN_POINT('Ctrl Pts',(9.17790600436843,22.2272369528839,-13.9988286084952));
#58439=CARTESIAN_POINT('Ctrl Pts',(9.42057845052407,22.2168912940591,-13.546461187714));
#58440=CARTESIAN_POINT('Ctrl Pts',(9.21333491179549,22.3216229093717,-13.6905787947584));
#58441=CARTESIAN_POINT('Ctrl Pts',(9.23277261467539,22.378992374506,-13.9569604616345));
#58442=CARTESIAN_POINT('Ctrl Pts',(9.4781725544487,22.4106027511509,-13.5060840404267));
#58443=CARTESIAN_POINT('Ctrl Pts',(9.27124287178487,22.5038190489669,-13.6513005654783));
#58444=CARTESIAN_POINT('Ctrl Pts',(9.28671750556737,22.5550936679072,-13.9153597695754));
#58445=CARTESIAN_POINT('Ctrl Pts',(9.48444711786266,22.4321789243944,-13.5016783842282));
#58446=CARTESIAN_POINT('Ctrl Pts',(9.27753750017006,22.5240683387227,-13.6470243760949));
#58447=CARTESIAN_POINT('Ctrl Pts',(9.29259450685464,22.5747083672934,-13.9108206091289));
#58448=CARTESIAN_POINT('Ctrl Pts',(9.49672536685248,22.4753618131691,-13.4930450095317));
#58449=CARTESIAN_POINT('Ctrl Pts',(9.28985611838946,22.564602870967,-13.6386438680677));
#58450=CARTESIAN_POINT('Ctrl Pts',(9.30409479488525,22.6139655317586,-13.901925618187));
#58451=CARTESIAN_POINT('Ctrl Pts',(9.50273249627371,22.4969800713172,-13.4888148772171));
#58452=CARTESIAN_POINT('Ctrl Pts',(9.29588389997394,22.5848994479116,-13.6345369851084));
#58453=CARTESIAN_POINT('Ctrl Pts',(9.30972130716465,22.6336184901156,-13.8975673005029));
#58454=CARTESIAN_POINT('Ctrl Pts',(9.52035918168828,22.5619152496179,-13.476385561487));
#58455=CARTESIAN_POINT('Ctrl Pts',(9.31356710910104,22.6458558854866,-13.6224724720524));
#58456=CARTESIAN_POINT('Ctrl Pts',(9.32623114985529,22.6926504596105,-13.8847613405295));
#58457=CARTESIAN_POINT('Ctrl Pts',(9.53158409879775,22.6053125634296,-13.468447447099));
#58458=CARTESIAN_POINT('Ctrl Pts',(9.32483548260588,22.6866238631496,-13.6147621214551));
#58459=CARTESIAN_POINT('Ctrl Pts',(9.3367448460817,22.732102555901,-13.8765826780708));
#58460=CARTESIAN_POINT('Ctrl Pts',(9.56368814998023,22.7358261581148,-13.4456891694235));
#58461=CARTESIAN_POINT('Ctrl Pts',(9.35704811788232,22.8091939866226,-13.5926671654132));
#58462=CARTESIAN_POINT('Ctrl Pts',(9.36681475560692,22.8507512566856,-13.8531347586999));
#58463=CARTESIAN_POINT('Ctrl Pts',(9.5829975742177,22.823263935959,-13.4319248824045));
#58464=CARTESIAN_POINT('Ctrl Pts',(9.37645126647122,22.8914279771673,-13.5792841202355));
#58465=CARTESIAN_POINT('Ctrl Pts',(9.38490071726704,22.9302401313564,-13.8389533735087));
#58466=CARTESIAN_POINT('Ctrl Pts',(9.63467303059377,23.086869673514,-13.3949568797211));
#58467=CARTESIAN_POINT('Ctrl Pts',(9.4283215850424,23.1391952104619,-13.5433774600759));
#58468=CARTESIAN_POINT('Ctrl Pts',(9.43330197030269,23.1698816673068,-13.8008651332953));
#58469=CARTESIAN_POINT('Ctrl Pts',(9.66080205100456,23.264327543883,-13.3760749408244));
#58470=CARTESIAN_POINT('Ctrl Pts',(9.45464141905301,23.3064610473423,-13.5249723329533));
#58471=CARTESIAN_POINT('Ctrl Pts',(9.45777543217764,23.3312069757732,-13.7814110162615));
#58472=CARTESIAN_POINT('Ctrl Pts',(9.69618216865947,23.6227778055913,-13.3504504958979));
#58473=CARTESIAN_POINT('Ctrl Pts',(9.49022252619599,23.6442122621145,-13.5000339915227));
#58474=CARTESIAN_POINT('Ctrl Pts',(9.49091383452651,23.6570707923046,-13.7550100763112));
#58475=CARTESIAN_POINT('Ctrl Pts',(9.70543536945587,23.8037698369644,-13.3437073024875));
#58476=CARTESIAN_POINT('Ctrl Pts',(9.49954967786973,23.8149979384621,-13.4934560518724));
#58477=CARTESIAN_POINT('Ctrl Pts',(9.4995807433815,23.8216089741294,-13.7480625443467));
#58478=CARTESIAN_POINT('Ctrl Pts',(9.70597513873851,24.0323294734863,-13.3433146790455));
#58479=CARTESIAN_POINT('Ctrl Pts',(9.50009270586957,24.0304786994239,-13.4930737933728));
#58480=CARTESIAN_POINT('Ctrl Pts',(9.50008631309344,24.0293904252603,-13.7476580232753));
#58481=CARTESIAN_POINT('Ctrl Pts',(9.70553034474903,24.0781576052184,-13.3436382698279));
#58482=CARTESIAN_POINT('Ctrl Pts',(9.49964517461909,24.0736863887931,-13.4933888785566));
#58483=CARTESIAN_POINT('Ctrl Pts',(9.49966970135809,24.0710523558596,-13.7479914198069));
#58484=CARTESIAN_POINT('Ctrl Pts',(9.70402058186149,24.1470768987552,-13.3447362257199));
#58485=CARTESIAN_POINT('Ctrl Pts',(9.49812638956954,24.1386573118864,-13.4944577823999));
#58486=CARTESIAN_POINT('Ctrl Pts',(9.49825559862898,24.1337062480285,-13.7491226469482));
#58487=CARTESIAN_POINT('Ctrl Pts',(9.70337612425004,24.1700954524399,-13.3452048589811));
#58488=CARTESIAN_POINT('Ctrl Pts',(9.49747804813204,24.160357728836,-13.4949140382431));
#58489=CARTESIAN_POINT('Ctrl Pts',(9.49765197443261,24.1546322022357,-13.7496054811704));
#58490=CARTESIAN_POINT('Ctrl Pts',(9.70181039353469,24.2160242659793,-13.3463431704996));
#58491=CARTESIAN_POINT('Ctrl Pts',(9.49590295559263,24.2036548244372,-13.4960222310312));
#58492=CARTESIAN_POINT('Ctrl Pts',(9.49618544965948,24.1963856617205,-13.7507782868312));
#58493=CARTESIAN_POINT('Ctrl Pts',(9.70088893502563,24.2389518587485,-13.3470129835802));
#58494=CARTESIAN_POINT('Ctrl Pts',(9.49497597105382,24.225268486177,-13.4966743322698));
#58495=CARTESIAN_POINT('Ctrl Pts',(9.49532237574291,24.2172289242047,-13.7514683972106));
#58496=CARTESIAN_POINT('Ctrl Pts',(9.69559422432726,24.3534073082494,-13.3508606484318));
#58497=CARTESIAN_POINT('Ctrl Pts',(9.48964887351038,24.3331782299118,-13.5004206915048));
#58498=CARTESIAN_POINT('Ctrl Pts',(9.49036314227762,24.3212793145206,-13.7554326574748));
#58499=CARTESIAN_POINT('Ctrl Pts',(9.68916022224817,24.4443879326826,-13.3555339196467));
#58500=CARTESIAN_POINT('Ctrl Pts',(9.48317387006694,24.4189497885899,-13.504972050757));
#58501=CARTESIAN_POINT('Ctrl Pts',(9.48433680488061,24.4039889585799,-13.7602475425037));
#58502=CARTESIAN_POINT('Ctrl Pts',(9.6634393151647,24.715630632223,-13.3741687205965));
#58503=CARTESIAN_POINT('Ctrl Pts',(9.45729426491734,24.674657571566,-13.52311676352));
#58504=CARTESIAN_POINT('Ctrl Pts',(9.4602455967653,24.650573187534,-13.7794470320152));
#58505=CARTESIAN_POINT('Ctrl Pts',(9.63775002362843,24.8941969109951,-13.3927413312077));
#58506=CARTESIAN_POINT('Ctrl Pts',(9.43141637017533,24.8429770623408,-13.541221148463));
#58507=CARTESIAN_POINT('Ctrl Pts',(9.43618400243639,24.8129061398801,-13.798582447208));
#58508=CARTESIAN_POINT('Ctrl Pts',(9.56979665799707,25.2469945208445,-13.441381543842));
#58509=CARTESIAN_POINT('Ctrl Pts',(9.36314059164007,25.174907732864,-13.5885109273976));
#58510=CARTESIAN_POINT('Ctrl Pts',(9.37253622263319,25.1336311822155,-13.8486965992851));
#58511=CARTESIAN_POINT('Ctrl Pts',(9.52753173217289,25.4212256474459,-13.4714495820274));
#58512=CARTESIAN_POINT('Ctrl Pts',(9.320621388888,25.3387948465226,-13.6177780168233));
#58513=CARTESIAN_POINT('Ctrl Pts',(9.33294924072412,25.2920230872501,-13.8796757870884));
#58514=CARTESIAN_POINT('Ctrl Pts',(9.47065193933464,25.6148436317644,-13.5113586085727));
#58515=CARTESIAN_POINT('Ctrl Pts',(9.26369917506079,25.5200585720568,-13.6564194462368));
#58516=CARTESIAN_POINT('Ctrl Pts',(9.27967340329896,25.4680394032114,-13.9207941723777));
#58517=CARTESIAN_POINT('Ctrl Pts',(9.46420202333222,25.6363234509834,-13.5158774981925));
#58518=CARTESIAN_POINT('Ctrl Pts',(9.25722980273212,25.5402115827205,-13.6608046879957));
#58519=CARTESIAN_POINT('Ctrl Pts',(9.27363215982219,25.4875665080051,-13.9254499975484));
#58520=CARTESIAN_POINT('Ctrl Pts',(9.45104171472625,25.6792165551332,-13.5250831787126));
#58521=CARTESIAN_POINT('Ctrl Pts',(9.24403189021062,25.580446362938,-13.6697366125152));
#58522=CARTESIAN_POINT('Ctrl Pts',(9.26130570026585,25.5265602319081,-13.9349346368283));
#58523=CARTESIAN_POINT('Ctrl Pts',(9.44433889025821,25.7006047210845,-13.5297646668679));
#58524=CARTESIAN_POINT('Ctrl Pts',(9.23731060205227,25.6005049962199,-13.6742783692687));
#58525=CARTESIAN_POINT('Ctrl Pts',(9.25502757293848,25.546004015586,-13.9397579877384));
#58526=CARTESIAN_POINT('Ctrl Pts',(9.42389557569635,25.7645001936973,-13.5440196484565));
#58527=CARTESIAN_POINT('Ctrl Pts',(9.21680681254345,25.6604369459517,-13.6881105608007));
#58528=CARTESIAN_POINT('Ctrl Pts',(9.23587956495122,25.6040907981566,-13.9544449365423));
#58529=CARTESIAN_POINT('Ctrl Pts',(9.40980812022507,25.806778431026,-13.5538121533282));
#58530=CARTESIAN_POINT('Ctrl Pts',(9.20268515890637,25.7000622918785,-13.6976073638699));
#58531=CARTESIAN_POINT('Ctrl Pts',(9.22268470384003,25.6425255523807,-13.9645341828734));
#58532=CARTESIAN_POINT('Ctrl Pts',(9.36619491727129,25.932680699603,-13.5840216342671));
#58533=CARTESIAN_POINT('Ctrl Pts',(9.1589493065576,25.8180973351854,-13.7269154264562));
#58534=CARTESIAN_POINT('Ctrl Pts',(9.18183487229295,25.756982139071,-13.9956590985482));
#58535=CARTESIAN_POINT('Ctrl Pts',(9.33531944381127,26.0153730275513,-13.6052699759399));
#58536=CARTESIAN_POINT('Ctrl Pts',(9.12801654872368,25.8954988194392,-13.7475086852288));
#58537=CARTESIAN_POINT('Ctrl Pts',(9.15291569757583,25.8321569688563,-14.0175513269118));
#58538=CARTESIAN_POINT('Ctrl Pts',(9.23744936372985,26.2598841203837,-13.6720799513866));
#58539=CARTESIAN_POINT('Ctrl Pts',(9.02989846070897,26.124492810673,-13.8123018789954));
#58540=CARTESIAN_POINT('Ctrl Pts',(9.06124675341241,26.054439739586,-14.0863858380353));
#58541=CARTESIAN_POINT('Ctrl Pts',(9.16522614835605,26.418146799207,-13.720699066088));
#58542=CARTESIAN_POINT('Ctrl Pts',(8.95760403593686,26.272189807985,-13.8593692962326));
#58543=CARTESIAN_POINT('Ctrl Pts',(8.99359966771377,26.1983148751026,-14.1364782535083));
#58544=CARTESIAN_POINT('Ctrl Pts',(9.04675320711485,26.6488731358305,-13.7988584568673));
#58545=CARTESIAN_POINT('Ctrl Pts',(8.8396384118494,26.4864000763885,-13.9346421962668));
#58546=CARTESIAN_POINT('Ctrl Pts',(8.88263328090294,26.4080660479035,-14.2170060986102));
#58547=CARTESIAN_POINT('Ctrl Pts',(9.00556864379736,26.724668077879,-13.8257853617022));
#58548=CARTESIAN_POINT('Ctrl Pts',(8.79856477912204,26.5568225974011,-13.9606137985784));
#58549=CARTESIAN_POINT('Ctrl Pts',(8.84405820972172,26.4769705271959,-14.2447489668247));
#58550=CARTESIAN_POINT('Ctrl Pts',(8.94125888839501,26.8367243925892,-13.8673912960299));
#58551=CARTESIAN_POINT('Ctrl Pts',(8.73458393580632,26.6606514330639,-14.0006470656152));
#58552=CARTESIAN_POINT('Ctrl Pts',(8.78382317974531,26.5788398835889,-14.287615680565));
#58553=CARTESIAN_POINT('Ctrl Pts',(8.91939992829263,26.8738036722238,-13.8814626371617));
#58554=CARTESIAN_POINT('Ctrl Pts',(8.71282066028938,26.6950205492259,-14.0141961613619));
#58555=CARTESIAN_POINT('Ctrl Pts',(8.76334922367439,26.6125483128922,-14.3021134241213));
#58556=CARTESIAN_POINT('Ctrl Pts',(8.87483584131177,26.947420683523,-13.9099960035042));
#58557=CARTESIAN_POINT('Ctrl Pts',(8.66847764979718,26.7631998723909,-14.0416544795966));
#58558=CARTESIAN_POINT('Ctrl Pts',(8.72160875835307,26.6794728551709,-14.3315114335205));
#58559=CARTESIAN_POINT('Ctrl Pts',(8.85211849071852,26.9839775314368,-13.9244657683607));
#58560=CARTESIAN_POINT('Ctrl Pts',(8.64588225815288,26.7970289078062,-14.0555729736903));
#58561=CARTESIAN_POINT('Ctrl Pts',(8.70033080036421,26.7127063466435,-14.34641967414));
#58562=CARTESIAN_POINT('Ctrl Pts',(8.73653994314236,27.1652095745738,-13.9976729904853));
#58563=CARTESIAN_POINT('Ctrl Pts',(8.5305769785088,26.9651990737812,-14.126204210908));
#58564=CARTESIAN_POINT('Ctrl Pts',(8.59207541474747,26.8774627173519,-14.4218452863613));
#58565=CARTESIAN_POINT('Ctrl Pts',(8.63857581146634,27.3039232901101,-14.0584339961704));
#58566=CARTESIAN_POINT('Ctrl Pts',(8.43329573465729,27.0929766694405,-14.184537001276));
#58567=CARTESIAN_POINT('Ctrl Pts',(8.50031838267292,27.0035660693995,-14.4844475260831));
#58568=CARTESIAN_POINT('Ctrl Pts',(8.43205452679184,27.5697679631042,-14.1832653127355));
#58569=CARTESIAN_POINT('Ctrl Pts',(8.22893898206923,27.336891173593,-14.303993073037));
#58570=CARTESIAN_POINT('Ctrl Pts',(8.30688247951664,27.245242992928,-14.6130615891751));
#58571=CARTESIAN_POINT('Ctrl Pts',(8.32349524991498,27.696895500351,-14.2473383251373));
#58572=CARTESIAN_POINT('Ctrl Pts',(8.12167890826586,27.4529918698611,-14.3651939112398));
#58573=CARTESIAN_POINT('Ctrl Pts',(8.20520162130922,27.3608134562285,-14.6790761982849));
#58574=CARTESIAN_POINT('Ctrl Pts',(8.0958209230527,27.940066659269,-14.3779312179124));
#58575=CARTESIAN_POINT('Ctrl Pts',(7.89760049643352,27.6740297912245,-14.4895090431896));
#58576=CARTESIAN_POINT('Ctrl Pts',(7.99195295573568,27.5818780963411,-14.8136264284226));
#58577=CARTESIAN_POINT('Ctrl Pts',(7.97670562766047,28.0561091060765,-14.4444528576548));
#58578=CARTESIAN_POINT('Ctrl Pts',(7.78060080854458,27.7789047025113,-14.5526858646747));
#58579=CARTESIAN_POINT('Ctrl Pts',(7.88038491947146,27.6873712051867,-14.8821638645775));
#58580=CARTESIAN_POINT('Ctrl Pts',(7.82103135401305,28.1943068383712,-14.5286861673289));
#58581=CARTESIAN_POINT('Ctrl Pts',(7.62904494836334,27.9025325222122,-14.63203155862));
#58582=CARTESIAN_POINT('Ctrl Pts',(7.73457431964004,27.8130054758372,-14.9689496818345));
#58583=CARTESIAN_POINT('Ctrl Pts',(7.78955667512429,28.2216027048998,-14.5455871841282));
#58584=CARTESIAN_POINT('Ctrl Pts',(7.598286999393,27.9270226975393,-14.6480127292069));
#58585=CARTESIAN_POINT('Ctrl Pts',(7.70509390682786,27.8378198938992,-14.9863628477604));
#58586=CARTESIAN_POINT('Ctrl Pts',(7.72591977577152,28.2755052515132,-14.579487760013));
#58587=CARTESIAN_POINT('Ctrl Pts',(7.53615718432266,27.9753071204984,-14.6800419075361));
#58588=CARTESIAN_POINT('Ctrl Pts',(7.6454891029661,27.8868221972088,-15.0212907073461));
#58589=CARTESIAN_POINT('Ctrl Pts',(7.69383664689685,28.3020444414061,-14.5964450623165));
#58590=CARTESIAN_POINT('Ctrl Pts',(7.50486038355863,27.9990389548318,-14.6960503341127));
#58591=CARTESIAN_POINT('Ctrl Pts',(7.61543879232438,27.9109487275864,-15.0387618643017));
#58592=CARTESIAN_POINT('Ctrl Pts',(7.5969094767131,28.3803480091191,-14.647262188812));
#58593=CARTESIAN_POINT('Ctrl Pts',(7.41024929743659,28.0690530186176,-14.7440600614543));
#58594=CARTESIAN_POINT('Ctrl Pts',(7.52465302114093,27.982133771713,-15.091118894199));
#58595=CARTESIAN_POINT('Ctrl Pts',(7.53133940020973,28.4308406046357,-14.681092957269));
#58596=CARTESIAN_POINT('Ctrl Pts',(7.34645413992588,28.1139578323579,-14.7759196021834));
#58597=CARTESIAN_POINT('Ctrl Pts',(7.46323752886183,28.0280361199399,-15.125974831266));
#58598=CARTESIAN_POINT('Ctrl Pts',(7.33178100387479,28.5773010543634,-14.782328694575));
#58599=CARTESIAN_POINT('Ctrl Pts',(7.1520743196714,28.2441717263217,-14.871402064795));
#58600=CARTESIAN_POINT('Ctrl Pts',(7.27632334582098,28.1611819502916,-15.2302782990676));
#58601=CARTESIAN_POINT('Ctrl Pts',(7.19495063365634,28.6682647836609,-14.849474803097));
#58602=CARTESIAN_POINT('Ctrl Pts',(7.01967189155258,28.3240420533312,-14.9343096208533));
#58603=CARTESIAN_POINT('Ctrl Pts',(7.1481626829883,28.2438762276959,-15.2994591252776));
#58604=CARTESIAN_POINT('Ctrl Pts',(6.9135955853759,28.8370962326483,-14.9825369223229));
#58605=CARTESIAN_POINT('Ctrl Pts',(6.74867575496167,28.4711445942248,-15.058566331689));
#58606=CARTESIAN_POINT('Ctrl Pts',(6.88463457001264,28.3973593211239,-15.4365534020641));
#58607=CARTESIAN_POINT('Ctrl Pts',(6.76907115430593,28.914963455736,-15.0484540472046));
#58608=CARTESIAN_POINT('Ctrl Pts',(6.61002452272855,28.5381997925323,-15.1198862928276));
#58609=CARTESIAN_POINT('Ctrl Pts',(6.74926735169343,28.4681476850395,-15.5044680022405));
#58610=CARTESIAN_POINT('Ctrl Pts',(6.47201687898309,29.0574380438273,-15.1785800066827));
#58611=CARTESIAN_POINT('Ctrl Pts',(6.32644002885306,28.6596820173027,-15.2405646922931));
#58612=CARTESIAN_POINT('Ctrl Pts',(6.4710347352573,28.5976699998072,-15.6385371439425));
#58613=CARTESIAN_POINT('Ctrl Pts',(6.3194882860113,29.1220469515791,-15.2427897294257));
#58614=CARTESIAN_POINT('Ctrl Pts',(6.18147732116283,28.7139248359103,-15.2998772546999));
#58615=CARTESIAN_POINT('Ctrl Pts',(6.32817050912569,28.656405351216,-15.70469260229));
#58616=CARTESIAN_POINT('Ctrl Pts',(6.12349203741434,29.1941487275923,-15.3217045706728));
#58617=CARTESIAN_POINT('Ctrl Pts',(5.99703656673586,28.7733421722218,-15.3722356540574));
#58618=CARTESIAN_POINT('Ctrl Pts',(6.14459278632615,28.721952398637,-15.7859987832458));
#58619=CARTESIAN_POINT('Ctrl Pts',(6.08402359052547,29.2081344154966,-15.3374205374095));
#58620=CARTESIAN_POINT('Ctrl Pts',(5.95976665824897,28.7848674248604,-15.3867016540606));
#58621=CARTESIAN_POINT('Ctrl Pts',(6.10762510082632,28.7346666559994,-15.8021909879922));
#58622=CARTESIAN_POINT('Ctrl Pts',(6.00481108118076,29.235136099283,-15.3686061720222));
#58623=CARTESIAN_POINT('Ctrl Pts',(5.88506002432616,28.8070167605749,-15.4153866452692));
#58624=CARTESIAN_POINT('Ctrl Pts',(6.03343157769096,28.7592136330259,-15.8343216346973));
#58625=CARTESIAN_POINT('Ctrl Pts',(5.96503423890355,29.2481644638745,-15.3840891406583));
#58626=CARTESIAN_POINT('Ctrl Pts',(5.84759340501311,28.8176478244873,-15.4296164975149));
#58627=CARTESIAN_POINT('Ctrl Pts',(5.99617503723461,28.7710575967267,-15.8502737807819));
#58628=CARTESIAN_POINT('Ctrl Pts',(5.84518801096566,29.285827922622,-15.4302010924098));
#58629=CARTESIAN_POINT('Ctrl Pts',(5.73467502532393,28.8482698420827,-15.4720336723545));
#58630=CARTESIAN_POINT('Ctrl Pts',(5.88392238984605,28.8052970930209,-15.8977830539599));
#58631=CARTESIAN_POINT('Ctrl Pts',(5.76460316441166,29.309042283798,-15.4604931073141));
#58632=CARTESIAN_POINT('Ctrl Pts',(5.65906122614119,28.8668766739417,-15.4998090557935));
#58633=CARTESIAN_POINT('Ctrl Pts',(5.80844348291024,28.8264010499212,-15.9289930019522));
#58634=CARTESIAN_POINT('Ctrl Pts',(5.6426748606603,29.3409890436428,-15.5052279766528));
#58635=CARTESIAN_POINT('Ctrl Pts',(5.54510753066133,28.8921201145448,-15.540725306626));
#58636=CARTESIAN_POINT('Ctrl Pts',(5.69424068407321,28.8554435481393,-15.9750834627829));
#58637=CARTESIAN_POINT('Ctrl Pts',(5.60185686122977,29.3511586098101,-15.5200224119935));
#58638=CARTESIAN_POINT('Ctrl Pts',(5.50695179331065,28.9001039225748,-15.5542677227203));
#58639=CARTESIAN_POINT('Ctrl Pts',(5.65600895573945,28.8646886046383,-15.9903262110367));
#58640=CARTESIAN_POINT('Ctrl Pts',(5.51986632851016,29.3705308152709,-15.5493720669948));
#58641=CARTESIAN_POINT('Ctrl Pts',(5.43040476978069,28.9151886717053,-15.5811202430405));
#58642=CARTESIAN_POINT('Ctrl Pts',(5.57921342901242,28.8822996938417,-16.0205652426492));
#58643=CARTESIAN_POINT('Ctrl Pts',(5.47867048511738,29.3797375986075,-15.5639351530272));
#58644=CARTESIAN_POINT('Ctrl Pts',(5.39199408493733,28.9222895153009,-15.5944358228649));
#58645=CARTESIAN_POINT('Ctrl Pts',(5.54062779747857,28.8906694935097,-16.0355696310093));
#58646=CARTESIAN_POINT('Ctrl Pts',(5.35495705072016,29.4058100316881,-15.607115874279));
#58647=CARTESIAN_POINT('Ctrl Pts',(5.27662176045004,28.9422275091807,-15.6339576546548));
#58648=CARTESIAN_POINT('Ctrl Pts',(5.42475297585001,28.9143716957695,-16.0800588491233));
#58649=CARTESIAN_POINT('Ctrl Pts',(5.27219555306174,29.4211589388003,-15.6352680825888));
#58650=CARTESIAN_POINT('Ctrl Pts',(5.19975787711073,28.9536492950679,-15.6596539110981));
#58651=CARTESIAN_POINT('Ctrl Pts',(5.3472353340361,28.9283252417574,-16.1090641481402));
#58652=CARTESIAN_POINT('Ctrl Pts',(5.02305213210112,29.4611376714299,-15.7178103797378));
#58653=CARTESIAN_POINT('Ctrl Pts',(4.96827292910735,28.9825980821897,-15.7351752246276));
#58654=CARTESIAN_POINT('Ctrl Pts',(5.11387790237459,28.9646695277837,-16.1941077084662));
#58655=CARTESIAN_POINT('Ctrl Pts',(4.8558120579994,29.4797132570353,-15.7702865042745));
#58656=CARTESIAN_POINT('Ctrl Pts',(4.81418315067994,28.9945338902948,-15.7829316553988));
#58657=CARTESIAN_POINT('Ctrl Pts',(4.95723433795089,28.9815564141466,-16.2481740063996));
#58658=CARTESIAN_POINT('Ctrl Pts',(4.51901742036134,29.5005364682645,-15.8700765191147));
#58659=CARTESIAN_POINT('Ctrl Pts',(4.50504494020981,29.0042572601608,-15.8739002545569));
#58660=CARTESIAN_POINT('Ctrl Pts',(4.64177936989425,29.0004865920627,-16.3509879384084));
#58661=CARTESIAN_POINT('Ctrl Pts',(4.3494629500257,29.502785301074,-15.9173905277554));
#58662=CARTESIAN_POINT('Ctrl Pts',(4.3502429631541,29.0019042207245,-15.9169948174607));
#58663=CARTESIAN_POINT('Ctrl Pts',(4.48296805417846,29.0025309794379,-16.399735694321));
#58664=CARTESIAN_POINT('Ctrl Pts',(4.09335666867169,29.4934411267723,-15.9844367581263));
#58665=CARTESIAN_POINT('Ctrl Pts',(4.11757727073345,28.9875429702007,-15.9781904236519));
#58666=CARTESIAN_POINT('Ctrl Pts',(4.24308894583155,28.9940362716043,-16.4688136139354));
#58667=CARTESIAN_POINT('Ctrl Pts',(4.00769193386057,29.488203178257,-16.0061312589015));
#58668=CARTESIAN_POINT('Ctrl Pts',(4.03976686665927,28.9809127305293,-15.9980533071268));
#58669=CARTESIAN_POINT('Ctrl Pts',(4.16285202190648,28.9892744987069,-16.4911655193356));
#58670=CARTESIAN_POINT('Ctrl Pts',(3.87874392389429,29.4770663983519,-16.0376838633684));
#58671=CARTESIAN_POINT('Ctrl Pts',(3.92291316792116,28.9681807792558,-16.0269890641618));
#58672=CARTESIAN_POINT('Ctrl Pts',(4.04207429867147,28.9791501531594,-16.5236742568235));
#58673=CARTESIAN_POINT('Ctrl Pts',(3.83568608727203,29.4728072307827,-16.0480365319683));
#58674=CARTESIAN_POINT('Ctrl Pts',(3.88389492951693,28.9634647647606,-16.0365012625793));
#58675=CARTESIAN_POINT('Ctrl Pts',(4.001744653625,28.9752781822712,-16.5343406406146));
#58676=CARTESIAN_POINT('Ctrl Pts',(3.77098556634597,29.4655837062055,-16.0633171833005));
#58677=CARTESIAN_POINT('Ctrl Pts',(3.82533008776607,28.955682491492,-16.0505552670575));
#58678=CARTESIAN_POINT('Ctrl Pts',(3.94114362844063,28.9687113421149,-16.5500843389504));
#58679=CARTESIAN_POINT('Ctrl Pts',(3.74939141393193,29.4630354881802,-16.0683712143744));
#58680=CARTESIAN_POINT('Ctrl Pts',(3.80578374002981,28.9529673365255,-16.0552084803821));
#58681=CARTESIAN_POINT('Ctrl Pts',(3.92091770513547,28.9663947803014,-16.5552915214721));
#58682=CARTESIAN_POINT('Ctrl Pts',(3.70628810723345,29.4576742045361,-16.0783680118345));
#58683=CARTESIAN_POINT('Ctrl Pts',(3.76678170918465,28.9473145341322,-16.0644192570448));
#58684=CARTESIAN_POINT('Ctrl Pts',(3.88054547112458,28.9615208862491,-16.5655912503298));
#58685=CARTESIAN_POINT('Ctrl Pts',(3.68476473814926,29.4548596671818,-16.083314174015));
#58686=CARTESIAN_POINT('Ctrl Pts',(3.74731382458174,28.9443751898187,-16.0689797247386));
#58687=CARTESIAN_POINT('Ctrl Pts',(3.86038584624321,28.9589622161346,-16.5706872952021));
#58688=CARTESIAN_POINT('Ctrl Pts',(3.49130865587881,29.4283277337408,-16.127363937821));
#58689=CARTESIAN_POINT('Ctrl Pts',(3.57193400752812,28.9168380011473,-16.1097329329338));
#58690=CARTESIAN_POINT('Ctrl Pts',(3.67918735214675,28.9348422779537,-16.6160718926013));
#58691=CARTESIAN_POINT('Ctrl Pts',(3.32115082183791,29.3962214040903,-16.1632103665466));
#58692=CARTESIAN_POINT('Ctrl Pts',(3.41868379435837,28.885249246741,-16.1429885986858));
#58693=CARTESIAN_POINT('Ctrl Pts',(3.51981090582723,28.905654709583,-16.6530045699382));
#58694=CARTESIAN_POINT('Ctrl Pts',(2.98447140597061,29.3151535083114,-16.2287504929071));
#58695=CARTESIAN_POINT('Ctrl Pts',(3.11558321115816,28.8079438698407,-16.2044649622416));
#58696=CARTESIAN_POINT('Ctrl Pts',(3.20446386879709,28.8319566350224,-16.7205307514468));
#58697=CARTESIAN_POINT('Ctrl Pts',(2.81794971294387,29.2661918358164,-16.2584434074366));
#58698=CARTESIAN_POINT('Ctrl Pts',(2.96606141020008,28.7622515268809,-16.2326005398578));
#58699=CARTESIAN_POINT('Ctrl Pts',(3.04849317455918,28.7874460320186,-16.7511234470313));
#58700=CARTESIAN_POINT('Ctrl Pts',(2.48868900652383,29.1511550976376,-16.3120890644351));
#58701=CARTESIAN_POINT('Ctrl Pts',(2.67017594325405,28.6563940412766,-16.284231703085));
#58702=CARTESIAN_POINT('Ctrl Pts',(2.74009479036264,28.6828672014999,-16.8063947256689));
#58703=CARTESIAN_POINT('Ctrl Pts',(2.32594930549035,29.0850820592773,-16.3360411540186));
#58704=CARTESIAN_POINT('Ctrl Pts',(2.52411048001744,28.5963080017393,-16.3076661076437));
#58705=CARTESIAN_POINT('Ctrl Pts',(2.58766645743185,28.6228008156417,-16.831072634431));
#58706=CARTESIAN_POINT('Ctrl Pts',(2.1250599072148,28.9913388786302,-16.3626331297301));
#58707=CARTESIAN_POINT('Ctrl Pts',(2.34344451308294,28.5116156314395,-16.3342596418995));
#58708=CARTESIAN_POINT('Ctrl Pts',(2.39950563332105,28.537579762439,-16.8584704278843));
#58709=CARTESIAN_POINT('Ctrl Pts',(2.08500913587358,28.9720313848574,-16.3677840722747));
#58710=CARTESIAN_POINT('Ctrl Pts',(2.30741972529226,28.4942013857767,-16.3394412041397));
#58711=CARTESIAN_POINT('Ctrl Pts',(2.36199252324546,28.5200274991674,-16.8637774595515));
#58712=CARTESIAN_POINT('Ctrl Pts',(2.0051675717704,28.9322819172796,-16.3777569142544));
#58713=CARTESIAN_POINT('Ctrl Pts',(2.23557690953715,28.458397994944,-16.3495362389501));
#58714=CARTESIAN_POINT('Ctrl Pts',(2.28720980878386,28.4838916282115,-16.8740525092714));
#58715=CARTESIAN_POINT('Ctrl Pts',(1.96554728119832,28.9119246509324,-16.3825574991731));
#58716=CARTESIAN_POINT('Ctrl Pts',(2.19991626407161,28.4400872660864,-16.3544276110724));
#58717=CARTESIAN_POINT('Ctrl Pts',(2.25009990362284,28.4653850267029,-16.8789985664897));
#58718=CARTESIAN_POINT('Ctrl Pts',(1.84762852982704,28.8494438636152,-16.3964183323368));
#58719=CARTESIAN_POINT('Ctrl Pts',(2.09374858695216,28.3839559804985,-16.3686452334824));
#58720=CARTESIAN_POINT('Ctrl Pts',(2.13965261480346,28.408584324102,-16.8932794261332));
#58721=CARTESIAN_POINT('Ctrl Pts',(1.77025016417281,28.8059015325617,-16.4049406057559));
#58722=CARTESIAN_POINT('Ctrl Pts',(2.0240311102136,28.3449272621931,-16.3775190668833));
#58723=CARTESIAN_POINT('Ctrl Pts',(2.06717702770033,28.369000396413,-16.9020599505988));
#58724=CARTESIAN_POINT('Ctrl Pts',(1.54177444682283,28.6696922285513,-16.4285233433696));
#58725=CARTESIAN_POINT('Ctrl Pts',(1.81802054001897,28.2230482321264,-16.4024562776685));
#58726=CARTESIAN_POINT('Ctrl Pts',(1.85317778430319,28.245173785856,-16.9263573205953));
#58727=CARTESIAN_POINT('Ctrl Pts',(1.39432796702046,28.5714557232892,-16.4416026489042));
#58728=CARTESIAN_POINT('Ctrl Pts',(1.68481012920359,28.1354202701133,-16.416850048029));
#58729=CARTESIAN_POINT('Ctrl Pts',(1.71507367590203,28.1558678938527,-16.9398329709249));
#58730=CARTESIAN_POINT('Ctrl Pts',(1.1091581197396,28.3602462452578,-16.4632990742983));
#58731=CARTESIAN_POINT('Ctrl Pts',(1.42630999988166,27.9469834669516,-16.4418103773245));
#58732=CARTESIAN_POINT('Ctrl Pts',(1.44797250333451,27.9638593241193,-16.9621868725179));
#58733=CARTESIAN_POINT('Ctrl Pts',(0.97143433369676,28.2472737238628,-16.4719148498968));
#58734=CARTESIAN_POINT('Ctrl Pts',(1.30115362468154,27.8463289268546,-16.4523713139938));
#58735=CARTESIAN_POINT('Ctrl Pts',(1.31897504755037,27.8611570567861,-16.9710637360526));
#58736=CARTESIAN_POINT('Ctrl Pts',(0.772335964035815,28.0665436198457,-16.4820482049561));
#58737=CARTESIAN_POINT('Ctrl Pts',(1.11938409554033,27.6848732656992,-16.4657595070228));
#58738=CARTESIAN_POINT('Ctrl Pts',(1.13249176716596,27.6968570019834,-16.9815041710235));
#58739=CARTESIAN_POINT('Ctrl Pts',(0.707219927244881,28.0044184229425,-16.4849604530816));
#58740=CARTESIAN_POINT('Ctrl Pts',(1.05990308308362,27.6294199257431,-16.4698065678274));
#58741=CARTESIAN_POINT('Ctrl Pts',(1.07150155369664,27.640379563638,-16.9845046714466));
#58742=CARTESIAN_POINT('Ctrl Pts',(0.627425661641159,27.9243604283892,-16.4880742390367));
#58743=CARTESIAN_POINT('Ctrl Pts',(0.986825074194957,27.5578383302768,-16.4743952087767));
#58744=CARTESIAN_POINT('Ctrl Pts',(0.996763139213813,27.5675995862004,-16.9877128184167));
#58745=CARTESIAN_POINT('Ctrl Pts',(0.611540473924973,27.9082218095615,-16.4886708677361));
#58746=CARTESIAN_POINT('Ctrl Pts',(0.972283286896175,27.5434186810164,-16.4752888037803));
#58747=CARTESIAN_POINT('Ctrl Pts',(0.981884454263182,27.5529281180705,-16.9883275273789));
#58748=CARTESIAN_POINT('Ctrl Pts',(0.580018327330572,27.8757931855677,-16.4898098071427));
#58749=CARTESIAN_POINT('Ctrl Pts',(0.943414684059886,27.5144388040394,-16.4770249256736));
#58750=CARTESIAN_POINT('Ctrl Pts',(0.952359585218988,27.5234475578251,-16.9895009817092));
#58751=CARTESIAN_POINT('Ctrl Pts',(0.564371283292323,27.8594932366258,-16.4903525315996));
#58752=CARTESIAN_POINT('Ctrl Pts',(0.9290786686879,27.4998699251214,-16.4778680690466));
#58753=CARTESIAN_POINT('Ctrl Pts',(0.937703954811051,27.5086294260622,-16.9900601529576));
#58754=CARTESIAN_POINT('Ctrl Pts',(0.517770310560036,27.8103379398031,-16.4919034726953));
#58755=CARTESIAN_POINT('Ctrl Pts',(0.886376806082585,27.4559394538946,-16.4803243487277));
#58756=CARTESIAN_POINT('Ctrl Pts',(0.894055670458409,27.4639428032576,-16.9916580947053));
#58757=CARTESIAN_POINT('Ctrl Pts',(0.487156485366989,27.777227184081,-16.4928344795921));
#58758=CARTESIAN_POINT('Ctrl Pts',(0.858291786859998,27.4263293129875,-16.4818659359195));
#58759=CARTESIAN_POINT('Ctrl Pts',(0.865381570302197,27.4338421235899,-16.992617315159));
#58760=CARTESIAN_POINT('Ctrl Pts',(0.336332590426369,27.6099874673847,-16.4970133717404));
#58761=CARTESIAN_POINT('Ctrl Pts',(0.720060538634519,27.2769753235213,-16.4891085915155));
#58762=CARTESIAN_POINT('Ctrl Pts',(0.724114041754052,27.2818060543167,-16.9969228486531));
#58763=CARTESIAN_POINT('Ctrl Pts',(0.222841397833277,27.470813335503,-16.4988386846704));
#58764=CARTESIAN_POINT('Ctrl Pts',(0.615458588915073,27.152300128901,-16.4934777845921));
#58765=CARTESIAN_POINT('Ctrl Pts',(0.617813773293677,27.1552841466947,-16.9988034793985));
#58766=CARTESIAN_POINT('Ctrl Pts',(0.00990321376705526,27.1819234494132,
-16.5003405467281));
#58767=CARTESIAN_POINT('Ctrl Pts',(0.418623080759106,26.8928768176219,-16.500034082667));
#58768=CARTESIAN_POINT('Ctrl Pts',(0.418367581724231,26.8926570393483,-17.0003508660311));
#58769=CARTESIAN_POINT('Ctrl Pts',(-0.0895433703373462,27.0322073820898,
-16.5000155646105));
#58770=CARTESIAN_POINT('Ctrl Pts',(0.326337742518627,26.7581881683623,-16.5022304055355));
#58771=CARTESIAN_POINT('Ctrl Pts',(0.325222039785076,26.7565515553554,-17.0000160414432));
#58772=CARTESIAN_POINT('Ctrl Pts',(-0.22808532752021,26.7996588451688,-16.4984881124101));
#58773=CARTESIAN_POINT('Ctrl Pts',(0.197300595381823,26.5482355425314,-16.5043570320983));
#58774=CARTESIAN_POINT('Ctrl Pts',(0.195458248265802,26.545143842926,-16.9984423127055));
#58775=CARTESIAN_POINT('Ctrl Pts',(-0.272491460913673,26.7208111901634,
-16.4978048280384));
#58776=CARTESIAN_POINT('Ctrl Pts',(0.155921684887115,26.4770642935037,-16.5048709970138));
#58777=CARTESIAN_POINT('Ctrl Pts',(0.153865735050095,26.4734641729081,-16.9977383254034));
#58778=CARTESIAN_POINT('Ctrl Pts',(-0.336397061068505,26.600511460516,-16.4965842207539));
#58779=CARTESIAN_POINT('Ctrl Pts',(0.096263783369711,26.3682980360483,-16.5054035854578));
#58780=CARTESIAN_POINT('Ctrl Pts',(0.0940092613899049,26.364100807324,-16.9964807347913));
#58781=CARTESIAN_POINT('Ctrl Pts',(-0.357248112372307,26.5600733475937,
-16.4961447004054));
#58782=CARTESIAN_POINT('Ctrl Pts',(0.0767954341642,26.3317400093734,-16.5055413589327));
#58783=CARTESIAN_POINT('Ctrl Pts',(0.0744793550369163,26.3273388947892,
-16.9960278969377));
#58784=CARTESIAN_POINT('Ctrl Pts',(-0.387841216089795,26.498903476538,-16.4954443177129));
#58785=CARTESIAN_POINT('Ctrl Pts',(0.0482046831755837,26.2763955006129,
-16.5056949266238));
#58786=CARTESIAN_POINT('Ctrl Pts',(0.0458246627006021,26.2717299338042,
-16.9953062928579));
#58787=CARTESIAN_POINT('Ctrl Pts',(-0.397929989940197,26.4784177145172,
-16.4952038798439));
#58788=CARTESIAN_POINT('Ctrl Pts',(0.0387756143308138,26.2578613891262,
-16.5057372758339));
#58789=CARTESIAN_POINT('Ctrl Pts',(0.0363751242704468,26.2531065180243,
-16.995058569621));
#58790=CARTESIAN_POINT('Ctrl Pts',(-0.41785522716858,26.4373219520784,-16.4947111621768));
#58791=CARTESIAN_POINT('Ctrl Pts',(0.020147303064918,26.2206715650669,-16.5058052567056));
#58792=CARTESIAN_POINT('Ctrl Pts',(0.0177123713203404,26.215746742428,-16.9945509226647));
#58793=CARTESIAN_POINT('Ctrl Pts',(-0.427682464432081,26.4167313372239,
-16.4944591218899));
#58794=CARTESIAN_POINT('Ctrl Pts',(0.0109564801403263,26.2020333124516,
-16.5058308763942));
#58795=CARTESIAN_POINT('Ctrl Pts',(0.00850779813750384,26.1970280059491,
-16.9942912454038));
#58796=CARTESIAN_POINT('Ctrl Pts',(-0.514916549790388,26.2310334534057,
-16.4921459441983));
#58797=CARTESIAN_POINT('Ctrl Pts',(-0.0704930411183981,26.0342333549254,
-16.5059913084747));
#58798=CARTESIAN_POINT('Ctrl Pts',(-0.0731990422494235,26.0282117868214,
-16.991907978272));
#58799=CARTESIAN_POINT('Ctrl Pts',(-0.583868202739844,26.0632566591539,
-16.4897780154229));
#58800=CARTESIAN_POINT('Ctrl Pts',(-0.135243030695479,25.8819909514499,
-16.5056453064897));
#58801=CARTESIAN_POINT('Ctrl Pts',(-0.137781846254395,25.8756874627897,
-16.9894682985939));
#58802=CARTESIAN_POINT('Ctrl Pts',(-0.705119344738234,25.7224378966208,
-16.4850383010123));
#58803=CARTESIAN_POINT('Ctrl Pts',(-0.249212478633839,25.5723054059926,
-16.5045205921069));
#58804=CARTESIAN_POINT('Ctrl Pts',(-0.251350387828509,25.5658522930326,
-16.98458496655));
#58805=CARTESIAN_POINT('Ctrl Pts',(-0.757417463412148,25.5493955100128,
-16.4826653704805));
#58806=CARTESIAN_POINT('Ctrl Pts',(-0.298533978119679,25.4147565405257,
-16.5037425494566));
#58807=CARTESIAN_POINT('Ctrl Pts',(-0.300334842855957,25.4085410670984,
-16.9821401326672));
#58808=CARTESIAN_POINT('Ctrl Pts',(-0.845380072148487,25.1980454046336,
-16.4783880116582));
#58809=CARTESIAN_POINT('Ctrl Pts',(-0.381512922806825,25.0945912805061,
-16.5021755819352));
#58810=CARTESIAN_POINT('Ctrl Pts',(-0.382724048673311,25.0891319505675,
-16.9777331645216));
#58811=CARTESIAN_POINT('Ctrl Pts',(-0.88104566901821,25.0197380423049,-16.4764831102671));
#58812=CARTESIAN_POINT('Ctrl Pts',(-0.415254760524545,24.9318357068706,
-16.5013859883012));
#58813=CARTESIAN_POINT('Ctrl Pts',(-0.416129835547799,24.9270343835225,
-16.9757705414227));
#58814=CARTESIAN_POINT('Ctrl Pts',(-0.911543766590598,24.8160928395057,
-16.4748019557039));
#58815=CARTESIAN_POINT('Ctrl Pts',(-0.44411885392913,24.7457485251799,-16.5006631669498));
#58816=CARTESIAN_POINT('Ctrl Pts',(-0.444695542276101,24.7419024208988,
-16.9740384454876));
#58817=CARTESIAN_POINT('Ctrl Pts',(-0.914798413228078,24.7934231348861,
-16.4746215017785));
#58818=CARTESIAN_POINT('Ctrl Pts',(-0.447197123951018,24.7250475825129,
-16.5005851404517));
#58819=CARTESIAN_POINT('Ctrl Pts',(-0.447743970993952,24.7212936029764,
-16.9738525234988));
#58820=CARTESIAN_POINT('Ctrl Pts',(-0.921038106174053,24.7479983123345,
-16.4742738404667));
#58821=CARTESIAN_POINT('Ctrl Pts',(-0.453099183041882,24.6835643674665,
-16.5004340097327));
#58822=CARTESIAN_POINT('Ctrl Pts',(-0.453588310581765,24.6799983187254,
-16.9734943275512));
#58823=CARTESIAN_POINT('Ctrl Pts',(-0.924024713623736,24.7252305558544,
-16.4741065451602));
#58824=CARTESIAN_POINT('Ctrl Pts',(-0.455924553911642,24.6627702033824,
-16.5003608644188));
#58825=CARTESIAN_POINT('Ctrl Pts',(-0.456385683463281,24.6593003627783,
-16.9733219629078));
#58826=CARTESIAN_POINT('Ctrl Pts',(-0.932566535330723,24.6568879141791,
-16.4736259575042));
#58827=CARTESIAN_POINT('Ctrl Pts',(-0.464005080455623,24.6003531735753,
-16.5001497685869));
#58828=CARTESIAN_POINT('Ctrl Pts',(-0.464386286247165,24.5971707019928,
-16.9728268127538));
#58829=CARTESIAN_POINT('Ctrl Pts',(-0.93769515390498,24.6113486125014,-16.4733344755913));
#58830=CARTESIAN_POINT('Ctrl Pts',(-0.468858612305496,24.558750101885,-16.5000203424063));
#58831=CARTESIAN_POINT('Ctrl Pts',(-0.46918995040038,24.5557713458215,-16.9725264984295));
#58832=CARTESIAN_POINT('Ctrl Pts',(-0.951402889619917,24.4747973150587,
-16.4725503892664));
#58833=CARTESIAN_POINT('Ctrl Pts',(-0.481829948120828,24.4340092880389,
-16.4996699330201));
#58834=CARTESIAN_POINT('Ctrl Pts',(-0.482029149367011,24.4316338295858,
-16.9717186531439));
#58835=CARTESIAN_POINT('Ctrl Pts',(-0.958304970217346,24.3838519341024,
-16.4721484267205));
#58836=CARTESIAN_POINT('Ctrl Pts',(-0.488366769549358,24.3508831821315,
-16.4994869083559));
#58837=CARTESIAN_POINT('Ctrl Pts',(-0.488493906800559,24.3489562298645,
-16.9713045105041));
#58838=CARTESIAN_POINT('Ctrl Pts',(-0.963009452978601,24.2929936995252,
-16.4718733844551));
#58839=CARTESIAN_POINT('Ctrl Pts',(-0.492822054870804,24.2678247304756,
-16.4993612048297));
#58840=CARTESIAN_POINT('Ctrl Pts',(-0.492900308952224,24.2663578511416,
-16.9710211339658));
#58841=CARTESIAN_POINT('Origin',(-0.976753528407678,24.4999999958215,-16.9714356779612));
#58842=CARTESIAN_POINT('Ctrl Pts',(6.78574855947051,19.4906334205529,-15.2493774847029));
#58843=CARTESIAN_POINT('Ctrl Pts',(7.09365200449485,19.6230994530404,-15.0579941028986));
#58844=CARTESIAN_POINT('Ctrl Pts',(7.39169961590562,19.7784989217241,-14.8605142516318));
#58845=CARTESIAN_POINT('Ctrl Pts',(7.96341514878726,20.1269516722891,-14.4823196206633));
#58846=CARTESIAN_POINT('Ctrl Pts',(8.24170752937464,20.3223222055852,-14.2982311601103));
#58847=CARTESIAN_POINT('Ctrl Pts',(8.51515294794751,20.5398470862767,-14.1330198635429));
#58848=CARTESIAN_POINT('Ctrl Pts',(8.51772116533781,20.5418925937812,-14.1314696945114));
#58849=CARTESIAN_POINT('Ctrl Pts',(8.52036854006083,20.5440034843838,-14.1298733170473));
#58850=CARTESIAN_POINT('Origin',(-0.976758640922575,23.4999998309184,-16.9714360885196));
#58851=CARTESIAN_POINT('Origin',(-27.5,23.5,-23.));
#58852=CARTESIAN_POINT('',(-27.5,23.5,-23.));
#58853=CARTESIAN_POINT('',(-27.5,24.5,-23.));
#58854=CARTESIAN_POINT('Origin',(1.59198825996909E-15,23.5,4.71469806142367E-15));
#58855=CARTESIAN_POINT('Origin',(-36.5,3.36766747301154E-16,-24.));
#58856=CARTESIAN_POINT('',(-36.5,49.3978607591793,-24.5));
#58857=CARTESIAN_POINT('',(-36.5,54.4282032302755,-24.5));
#58858=CARTESIAN_POINT('Origin',(-36.5000000000003,50.0331217848142,-24.0000000000004));
#58859=CARTESIAN_POINT('Origin',(-37.5,41.9220413888134,-36.7681064455182));
#58860=CARTESIAN_POINT('',(-37.5,49.6110803960012,-23.7318935544818));
#58861=CARTESIAN_POINT('Origin',(-37.5,50.0331217848147,-24.));
#58862=CARTESIAN_POINT('',(-37.5,41.5,-36.5));
#58863=CARTESIAN_POINT('Ctrl Pts',(-37.4999999984477,49.6111157620785,-23.7318378827565));
#58864=CARTESIAN_POINT('Ctrl Pts',(-36.999945703858,49.6111031628287,-23.7318577159421));
#58865=CARTESIAN_POINT('Ctrl Pts',(-37.0000000019487,50.0331903787841,-23.9999932725221));
#58866=CARTESIAN_POINT('Ctrl Pts',(-37.5000026475399,49.5809381372911,-23.7793421740157));
#58867=CARTESIAN_POINT('Ctrl Pts',(-37.0125257432584,49.5919210538653,-23.7620533492161));
#58868=CARTESIAN_POINT('Ctrl Pts',(-37.0000003236668,50.0030123006108,-24.0237451732358));
#58869=CARTESIAN_POINT('Ctrl Pts',(-37.4966146037487,49.5507607813308,-23.8268460420991));
#58870=CARTESIAN_POINT('Ctrl Pts',(-37.0226617091426,49.5716751064898,-23.7939236301844));
#58871=CARTESIAN_POINT('Ctrl Pts',(-36.9983053346281,49.9728345473706,-24.0474967093262));
#58872=CARTESIAN_POINT('Ctrl Pts',(-37.4831283980406,49.491028778915,-23.9208735363186));
#58873=CARTESIAN_POINT('Ctrl Pts',(-37.0369947679708,49.5303132082949,-23.8590337133256));
#58874=CARTESIAN_POINT('Ctrl Pts',(-36.9915604437569,49.9131017946599,-24.0945094462342));
#58875=CARTESIAN_POINT('Ctrl Pts',(-37.4730329455306,49.4614743777896,-23.967396776267));
#58876=CARTESIAN_POINT('Ctrl Pts',(-37.0413371805881,49.5091937801452,-23.8922789893572));
#58877=CARTESIAN_POINT('Ctrl Pts',(-36.9865118906715,49.8835470446703,-24.1177704508956));
#58878=CARTESIAN_POINT('Ctrl Pts',(-37.446338975696,49.4035751035746,-24.0585392702631));
#58879=CARTESIAN_POINT('Ctrl Pts',(-37.0439552690129,49.4668675528739,-23.9589070769676));
#58880=CARTESIAN_POINT('Ctrl Pts',(-36.9731634448554,49.8256471127136,-24.1633403049858));
#58881=CARTESIAN_POINT('Ctrl Pts',(-37.429740631672,49.3752306064593,-24.1031579324689));
#58882=CARTESIAN_POINT('Ctrl Pts',(-37.0423583210133,49.4456316816316,-23.9923356526007));
#58883=CARTESIAN_POINT('Ctrl Pts',(-36.9648636339063,49.7973023126176,-24.1856488539623));
#58884=CARTESIAN_POINT('Ctrl Pts',(-37.390377073182,49.3203254093101,-24.1895872818758));
#58885=CARTESIAN_POINT('Ctrl Pts',(-37.0332157434799,49.4038164073336,-24.0581594204861));
#58886=CARTESIAN_POINT('Ctrl Pts',(-36.9451808008242,49.7423965456869,-24.2288618610315));
#58887=CARTESIAN_POINT('Ctrl Pts',(-37.3676121138729,49.2937650652586,-24.231397408705));
#58888=CARTESIAN_POINT('Ctrl Pts',(-37.0257725875086,49.3831899562253,-24.0906286737161));
#58889=CARTESIAN_POINT('Ctrl Pts',(-36.9337979027379,49.7158359419089,-24.2497660334815));
#58890=CARTESIAN_POINT('Ctrl Pts',(-37.3163764581199,49.2429663043523,-24.311362586571));
#58891=CARTESIAN_POINT('Ctrl Pts',(-37.0052677332731,49.3432758528686,-24.1534597018221));
#58892=CARTESIAN_POINT('Ctrl Pts',(-36.9081794773421,49.6650366944085,-24.289746799377));
#58893=CARTESIAN_POINT('Ctrl Pts',(-37.287906093082,49.2187282161604,-24.3495171202411));
#58894=CARTESIAN_POINT('Ctrl Pts',(-36.9922786439071,49.3239297683643,-24.1839134581893));
#58895=CARTESIAN_POINT('Ctrl Pts',(-36.8939441137087,49.6407983870913,-24.308823128154));
#58896=CARTESIAN_POINT('Ctrl Pts',(-37.2258363558164,49.173065055751,-24.4213980614082));
#58897=CARTESIAN_POINT('Ctrl Pts',(-36.9611889277236,49.2871849199918,-24.2417555843231));
#58898=CARTESIAN_POINT('Ctrl Pts',(-36.8629091218297,49.5951348186603,-24.3447617436394));
#58899=CARTESIAN_POINT('Ctrl Pts',(-37.1922373840171,49.1516402781994,-24.455124005055));
#58900=CARTESIAN_POINT('Ctrl Pts',(-36.9431292563272,49.2697227239588,-24.2692438062169));
#58901=CARTESIAN_POINT('Ctrl Pts',(-36.8461096933389,49.5737098600968,-24.3616237923194));
#58902=CARTESIAN_POINT('Ctrl Pts',(-37.1205910755058,49.1120378371204,-24.517464428095));
#58903=CARTESIAN_POINT('Ctrl Pts',(-36.9025509928616,49.2372711703841,-24.3203276162804));
#58904=CARTESIAN_POINT('Ctrl Pts',(-36.8102868777744,49.534107085388,-24.3927922372483));
#58905=CARTESIAN_POINT('Ctrl Pts',(-37.0825441996165,49.0938604283893,-24.5460785063992));
#58906=CARTESIAN_POINT('Ctrl Pts',(-36.8800425170188,49.2222192372126,-24.3440217082585));
#58907=CARTESIAN_POINT('Ctrl Pts',(-36.791263722181,49.5159295315503,-24.4070984271328));
#58908=CARTESIAN_POINT('Ctrl Pts',(-37.0027728479139,49.061121037485,-24.5976154173431));
#58909=CARTESIAN_POINT('Ctrl Pts',(-36.8313364551817,49.1950237103828,-24.3868317119147));
#58910=CARTESIAN_POINT('Ctrl Pts',(-36.7513788065511,49.4831898778153,-24.4328653160013));
#58911=CARTESIAN_POINT('Ctrl Pts',(-36.9610488835586,49.0465592652919,-24.6205379194415));
#58912=CARTESIAN_POINT('Ctrl Pts',(-36.8051210511832,49.182823514119,-24.4060367249271));
#58913=CARTESIAN_POINT('Ctrl Pts',(-36.7305173047078,49.4686279945608,-24.4443258445491));
#58914=CARTESIAN_POINT('Ctrl Pts',(-36.8747686270439,49.0213462124955,-24.6602271995625));
#58915=CARTESIAN_POINT('Ctrl Pts',(-36.7498616197956,49.1616716404749,-24.4393330752317));
#58916=CARTESIAN_POINT('Ctrl Pts',(-36.6873782930618,49.443414746811,-24.4641692147401));
#58917=CARTESIAN_POINT('Ctrl Pts',(-36.8302128863916,49.0106950931136,-24.6769937237974));
#58918=CARTESIAN_POINT('Ctrl Pts',(-36.7207763816884,49.1526735677021,-24.4534974461114));
#58919=CARTESIAN_POINT('Ctrl Pts',(-36.6651010626569,49.4327635489392,-24.4725519253));
#58920=CARTESIAN_POINT('Ctrl Pts',(-36.7391717313683,48.9935191854961,-24.7040312830438));
#58921=CARTESIAN_POINT('Ctrl Pts',(-36.6607031513577,49.1381669860886,-24.4763330696242));
#58922=CARTESIAN_POINT('Ctrl Pts',(-36.6195818726028,49.4155875120346,-24.4860698090038));
#58923=CARTESIAN_POINT('Ctrl Pts',(-36.6926868974402,48.9869945068099,-24.7143021456072));
#58924=CARTESIAN_POINT('Ctrl Pts',(-36.6296563273817,49.1326255446801,-24.4850561632574));
#58925=CARTESIAN_POINT('Ctrl Pts',(-36.5963402077165,49.409062786363,-24.4912048929667));
#58926=CARTESIAN_POINT('Ctrl Pts',(-36.5987293041569,48.9782037218442,-24.7281402131275));
#58927=CARTESIAN_POINT('Ctrl Pts',(-36.5666266668979,49.1251717354285,-24.4967896223414));
#58928=CARTESIAN_POINT('Ctrl Pts',(-36.5493629685859,49.4002719362922,-24.4981234586691));
#58929=CARTESIAN_POINT('Ctrl Pts',(-36.5512571427956,48.9759376715364,-24.7317073299761));
#58930=CARTESIAN_POINT('Ctrl Pts',(-36.5345740079014,49.1232421108123,-24.499827152645));
#58931=CARTESIAN_POINT('Ctrl Pts',(-36.5256276984433,49.3980058698557,-24.4999068948091));
#58932=CARTESIAN_POINT('Ctrl Pts',(-36.4562866573806,48.9757101072324,-24.7320655517066));
#58933=CARTESIAN_POINT('Ctrl Pts',(-36.4705163089246,49.123048899448,-24.5001312974868));
#58934=CARTESIAN_POINT('Ctrl Pts',(-36.4781440730316,49.3977783038758,-24.500085993473));
#58935=CARTESIAN_POINT('Ctrl Pts',(-36.4087889373822,48.9777485946843,-24.7288566543092));
#58936=CARTESIAN_POINT('Ctrl Pts',(-36.43843759609,49.1247848624327,-24.4973986208165));
#58937=CARTESIAN_POINT('Ctrl Pts',(-36.4543960250934,49.3998168058322,-24.4984816548169));
#58938=CARTESIAN_POINT('Ctrl Pts',(-36.3147296267512,48.9860888614095,-24.7157277728121));
#58939=CARTESIAN_POINT('Ctrl Pts',(-36.3753047257849,49.1318576224222,-24.4862649927414));
#58940=CARTESIAN_POINT('Ctrl Pts',(-36.4073679332755,49.4081571342912,-24.4919176584518));
#58941=CARTESIAN_POINT('Ctrl Pts',(-36.2681686347218,48.992390587583,-24.7058078723002));
#58942=CARTESIAN_POINT('Ctrl Pts',(-36.3441803599222,49.1372108049169,-24.4778382480196));
#58943=CARTESIAN_POINT('Ctrl Pts',(-36.3840881938228,49.4144589058036,-24.4869580440036));
#58944=CARTESIAN_POINT('Ctrl Pts',(-36.1769261057559,49.0091297146586,-24.6794578737954));
#58945=CARTESIAN_POINT('Ctrl Pts',(-36.2839031722063,49.1513523853739,-24.4555771932943));
#58946=CARTESIAN_POINT('Ctrl Pts',(-36.338468328439,49.4311981587367,-24.473783919146));
#58947=CARTESIAN_POINT('Ctrl Pts',(-36.1322451504778,49.0195670088094,-24.6630279438459));
#58948=CARTESIAN_POINT('Ctrl Pts',(-36.2546907643748,49.1601729318861,-24.4416922764546));
#58949=CARTESIAN_POINT('Ctrl Pts',(-36.3161284979174,49.4416355296862,-24.4655694956441));
#58950=CARTESIAN_POINT('Ctrl Pts',(-36.0456679431823,49.0443658677742,-24.6239906694594));
#58951=CARTESIAN_POINT('Ctrl Pts',(-36.1991315589116,49.1809863110149,-24.4089287693469));
#58952=CARTESIAN_POINT('Ctrl Pts',(-36.2728410275264,49.4664345800778,-24.4460521102632));
#58953=CARTESIAN_POINT('Ctrl Pts',(-36.003772244485,49.0587272740393,-24.601383574603));
#58954=CARTESIAN_POINT('Ctrl Pts',(-36.1727424636104,49.1930248987828,-24.3899781533289));
#58955=CARTESIAN_POINT('Ctrl Pts',(-36.2518936680164,49.480796095646,-24.4347492773044));
#58956=CARTESIAN_POINT('Ctrl Pts',(-35.9236143812708,49.0910834492376,-24.5504499049892));
#58957=CARTESIAN_POINT('Ctrl Pts',(-36.1236482291063,49.2199185380588,-24.3476433677986));
#58958=CARTESIAN_POINT('Ctrl Pts',(-36.2118155173364,49.5131525300135,-24.4092839956601));
#58959=CARTESIAN_POINT('Ctrl Pts',(-35.8853531222871,49.1090777974647,-24.5221239924888));
#58960=CARTESIAN_POINT('Ctrl Pts',(-36.1009245697621,49.2348292308243,-24.3241716102623));
#58961=CARTESIAN_POINT('Ctrl Pts',(-36.1926854283368,49.5311467527012,-24.395122094762));
#58962=CARTESIAN_POINT('Ctrl Pts',(-35.8492954555149,49.1287069943377,-24.4912245730675));
#58963=CARTESIAN_POINT('Ctrl Pts',(-36.0805222911065,49.2508329082794,-24.2989793242432));
#58964=CARTESIAN_POINT('Ctrl Pts',(-36.1746565192972,49.5507763940651,-24.3796730443644));
#58965=CARTESIAN_POINT('',(-35.8596780097302,49.1231323091022,-24.4999999976734));
#58966=CARTESIAN_POINT('Ctrl Pts',(-35.8596780097302,49.1231323076242,-24.5));
#58967=CARTESIAN_POINT('Ctrl Pts',(-35.8897007194235,49.1231323141072,-24.5));
#58968=CARTESIAN_POINT('Ctrl Pts',(-35.9492795917087,49.12628580103,-24.5));
#58969=CARTESIAN_POINT('Ctrl Pts',(-36.0079619111141,49.1354984450364,-24.5));
#58970=CARTESIAN_POINT('Ctrl Pts',(-36.0516397569449,49.1446647887917,-24.5));
#58971=CARTESIAN_POINT('Ctrl Pts',(-36.0733950255041,49.1498133203893,-24.5));
#58972=CARTESIAN_POINT('Ctrl Pts',(-36.1022332978191,49.1578185056805,-24.5));
#58973=CARTESIAN_POINT('Ctrl Pts',(-36.116596336941,49.1622047284401,-24.5));
#58974=CARTESIAN_POINT('Ctrl Pts',(-36.1522448462494,49.1735909724898,-24.5));
#58975=CARTESIAN_POINT('Ctrl Pts',(-36.1800852563754,49.1840820076817,-24.5));
#58976=CARTESIAN_POINT('Ctrl Pts',(-36.2344635854011,49.2077175303379,-24.5));
#58977=CARTESIAN_POINT('Ctrl Pts',(-36.2610010813319,49.2208628794797,-24.5));
#58978=CARTESIAN_POINT('Ctrl Pts',(-36.3127941023519,49.2497652256379,-24.5));
#58979=CARTESIAN_POINT('Ctrl Pts',(-36.3380490893341,49.2655233188928,-24.5));
#58980=CARTESIAN_POINT('Ctrl Pts',(-36.3688173582917,49.2868516528285,-24.5));
#58981=CARTESIAN_POINT('Ctrl Pts',(-36.3749341691932,49.2912014358321,-24.5));
#58982=CARTESIAN_POINT('Ctrl Pts',(-36.3870418406883,49.3000299236013,-24.5));
#58983=CARTESIAN_POINT('Ctrl Pts',(-36.4050308157833,49.3134769801761,-24.5));
#58984=CARTESIAN_POINT('Ctrl Pts',(-36.4341648250175,49.3368925485922,-24.5));
#58985=CARTESIAN_POINT('Ctrl Pts',(-36.4622110995748,49.3615962902832,-24.5));
#58986=CARTESIAN_POINT('Ctrl Pts',(-36.4812975745014,49.3795354237726,-24.5));
#58987=CARTESIAN_POINT('Ctrl Pts',(-36.4907080161569,49.3886622568197,-24.5));
#58988=CARTESIAN_POINT('Ctrl Pts',(-36.4947130222966,49.3926069640088,-24.5));
#58989=CARTESIAN_POINT('Ctrl Pts',(-36.4973768431774,49.3952440914044,-24.5));
#58990=CARTESIAN_POINT('Ctrl Pts',(-36.4986848184451,49.3965508641444,-24.5));
#58991=CARTESIAN_POINT('Ctrl Pts',(-36.5,49.3978607591793,-24.5));
#58992=CARTESIAN_POINT('Origin',(-36.4999950467498,49.6110877386296,-23.7318819960386));
#58993=CARTESIAN_POINT('Origin',(-50.,38.1236688894923,-34.3551484358543));
#58994=CARTESIAN_POINT('',(-45.2221315177632,44.0220106908928,-25.0702378819582));
#58995=CARTESIAN_POINT('',(-10.,39.7323075626015,-31.8229001029736));
#58996=CARTESIAN_POINT('',(-10.,39.7323075626015,-31.8229001029736));
#58997=CARTESIAN_POINT('',(-10.,38.1236688894923,-34.3551484358543));
#58998=CARTESIAN_POINT('Origin',(6.61363325216158E-15,52.,24.));
#58999=CARTESIAN_POINT('',(-3.43565291283912,52.,26.90625));
#59000=CARTESIAN_POINT('',(-3.43565291283912,52.,26.90625));
#59001=CARTESIAN_POINT('',(-27.1034840901754,52.,1.07291666666665));
#59002=CARTESIAN_POINT('',(-11.,52.,24.));
#59003=CARTESIAN_POINT('',(-6.,52.,-16.7705098312484));
#59004=CARTESIAN_POINT('Origin',(-5.,52.,-16.7705098312484));
#59005=CARTESIAN_POINT('',(-6.,52.,-23.8747810831708));
#59006=CARTESIAN_POINT('',(-6.,52.,-12.1904119063322));
#59007=CARTESIAN_POINT('',(-27.1034840901754,52.,1.07291666666665));
#59008=CARTESIAN_POINT('',(15.2695685015073,52.,-12.9166666666667));
#59009=CARTESIAN_POINT('',(27.1034840901754,52.,1.07291666666666));
#59010=CARTESIAN_POINT('',(15.2695685015073,52.,12.9166666666666));
#59011=CARTESIAN_POINT('Origin',(6.61287431064084E-15,52.,0.));
#59012=CARTESIAN_POINT('',(3.43565291283914,52.,26.90625));
#59013=CARTESIAN_POINT('',(3.43565291283914,52.,26.90625));
#59014=CARTESIAN_POINT('Origin',(6.61363325216158E-15,52.,24.));
#59015=CARTESIAN_POINT('Origin',(-50.,41.5,-36.5));
#59016=CARTESIAN_POINT('Origin',(-50.,-2.17497943900684,-3.42375708761853));
#59017=CARTESIAN_POINT('Origin',(-6.,3.67381906146713E-16,1.84889274661174E-32));
#59018=CARTESIAN_POINT('',(-6.,40.2323075626015,-16.7705098312484));
#59019=CARTESIAN_POINT('',(-6.,3.67381906146713E-16,-16.7705098312484));
#59020=CARTESIAN_POINT('',(-6.,40.2323075626015,1.46930375624346E-14));
#59021=CARTESIAN_POINT('',(-6.,52.0032753870454,-24.));
#59022=CARTESIAN_POINT('',(-6.,3.67381906146713E-16,-24.));
#59023=CARTESIAN_POINT('Origin',(-6.00000000000972,54.3934990501575,-23.8748259395246));
#59024=CARTESIAN_POINT('Origin',(-50.,3.67381906146713E-16,1.84889274661174E-32));
#59025=CARTESIAN_POINT('Origin',(-50.,3.67381906146713E-16,1.84889274661174E-32));
#59026=CARTESIAN_POINT('',(-50.,40.4835859155314,-25.7842093518926));
#59027=CARTESIAN_POINT('Origin',(1.59198825996909E-15,24.5,4.71469806142367E-15));
#59028=CARTESIAN_POINT('Origin',(-50.,51.6880449296918,-20.4624272250886));
#59029=CARTESIAN_POINT('Origin',(-10.,39.7323075626015,-31.8229001029736));
#59030=CARTESIAN_POINT('',(-6.5,39.7323075626015,-16.2480768092719));
#59031=CARTESIAN_POINT('',(-6.5,39.7323075626015,-31.8229001029736));
#59032=CARTESIAN_POINT('',(-10.,39.7323075626015,-14.3614066163451));
#59033=CARTESIAN_POINT('Origin',(6.61363325216158E-15,39.7323075626015,
1.23256668029931E-15));
#59034=CARTESIAN_POINT('',(-10.,39.7323075626015,-31.8229001029736));
#59035=CARTESIAN_POINT('Origin',(-45.2221315177632,40.4835859155314,-25.7842093518926));
#59036=CARTESIAN_POINT('Origin',(-4.19913133791448,57.,-27.5520833333334));
#59037=CARTESIAN_POINT('',(-4.19913133791448,53.,-27.5520833333334));
#59038=CARTESIAN_POINT('',(-6.78091634720693,53.,-24.5));
#59039=CARTESIAN_POINT('',(-4.19913133791448,53.,-27.5520833333334));
#59040=CARTESIAN_POINT('',(-6.78091634720693,57.,-24.5));
#59041=CARTESIAN_POINT('Origin',(-10.,3.67381906146713E-16,0.));
#59042=CARTESIAN_POINT('',(-10.,39.5242048993244,-13.6106575888162));
#59043=CARTESIAN_POINT('Ctrl Pts',(-10.,39.7323075626015,-14.3614066163451));
#59044=CARTESIAN_POINT('Ctrl Pts',(-10.,39.7323075626015,-14.200398990526));
#59045=CARTESIAN_POINT('Ctrl Pts',(-10.,39.699502446739,-14.009995208009));
#59046=CARTESIAN_POINT('Ctrl Pts',(-10.,39.6147673433497,-13.7776180829596));
#59047=CARTESIAN_POINT('Ctrl Pts',(-10.,39.5738101323051,-13.6904818142623));
#59048=CARTESIAN_POINT('Ctrl Pts',(-10.,39.5242048993244,-13.6106575888162));
#59049=CARTESIAN_POINT('',(-10.,51.,-13.6106575888162));
#59050=CARTESIAN_POINT('',(-10.,3.67381906146713E-16,-13.6106575888162));
#59051=CARTESIAN_POINT('',(-10.,51.,0.));
#59052=CARTESIAN_POINT('Origin',(-10.,45.4641016151378,-17.5));
#59053=CARTESIAN_POINT('Ctrl Pts',(16.2770594071445,26.117084953911,2.70320865940617));
#59054=CARTESIAN_POINT('Ctrl Pts',(16.1847747722226,25.1844547539906,3.25888995310305));
#59055=CARTESIAN_POINT('Ctrl Pts',(17.2635478560624,25.2642374615925,3.38919957270747));
#59056=CARTESIAN_POINT('Ctrl Pts',(16.2967231208785,26.0401987677082,2.58480587333236));
#59057=CARTESIAN_POINT('Ctrl Pts',(16.2046985714116,25.1219174064774,3.16392715346833));
#59058=CARTESIAN_POINT('Ctrl Pts',(17.2844032861437,25.2001657110687,3.28455076234357));
#59059=CARTESIAN_POINT('Ctrl Pts',(16.3146546406934,25.9585491601778,2.46884251835106));
#59060=CARTESIAN_POINT('Ctrl Pts',(16.2234217236847,25.0559444309027,3.07071608610299));
#59061=CARTESIAN_POINT('Ctrl Pts',(17.303421588318,25.1321242999822,3.18205778145459));
#59062=CARTESIAN_POINT('Ctrl Pts',(16.3473809405565,25.7855724308805,2.24193572830452));
#59063=CARTESIAN_POINT('Ctrl Pts',(16.2586774276057,24.9166403886353,2.88760736217028));
#59064=CARTESIAN_POINT('Ctrl Pts',(17.3381313008865,24.9879770258997,2.98150885069049));
#59065=CARTESIAN_POINT('Ctrl Pts',(16.3621754499714,25.694246003057,2.13099201606505));
#59066=CARTESIAN_POINT('Ctrl Pts',(16.2751973635875,24.8433767087607,2.79778198770337));
#59067=CARTESIAN_POINT('Ctrl Pts',(17.353822446655,24.9118716689619,2.88345253963371));
#59068=CARTESIAN_POINT('Ctrl Pts',(16.3788998863479,25.5738507355765,1.99559089989728));
#59069=CARTESIAN_POINT('Ctrl Pts',(16.2945840207838,24.7468003055873,2.68754694707923));
#59070=CARTESIAN_POINT('Ctrl Pts',(17.3715604855917,24.8115422797102,2.76377983572222));
#59071=CARTESIAN_POINT('Ctrl Pts',(16.382158257244,25.5494440782525,1.9686582620157));
#59072=CARTESIAN_POINT('Ctrl Pts',(16.2983964036959,24.727243668477,2.66561253202148));
#59073=CARTESIAN_POINT('Ctrl Pts',(17.375016333334,24.7912033985914,2.73997573657795));
#59074=CARTESIAN_POINT('Ctrl Pts',(16.3884940923374,25.5000673076495,1.91519865899398));
#59075=CARTESIAN_POINT('Ctrl Pts',(16.3058846588611,24.6876852903887,2.62202284398017));
#59076=CARTESIAN_POINT('Ctrl Pts',(17.3817361586463,24.7500560896602,2.69272608754677));
#59077=CARTESIAN_POINT('Ctrl Pts',(16.3915654053909,25.4751465153454,1.88872442372019));
#59078=CARTESIAN_POINT('Ctrl Pts',(16.3095531288558,24.6677240764023,2.60041130993974));
#59079=CARTESIAN_POINT('Ctrl Pts',(17.3849936116739,24.7292887628288,2.66932714213006));
#59080=CARTESIAN_POINT('Ctrl Pts',(16.4005017546482,25.3996926651759,1.81006291261778));
#59081=CARTESIAN_POINT('Ctrl Pts',(16.3203356992417,24.6073073367928,2.53613976226817));
#59082=CARTESIAN_POINT('Ctrl Pts',(17.3944715581686,24.6664105542314,2.59980307942765));
#59083=CARTESIAN_POINT('Ctrl Pts',(16.4060893408832,25.3484683787228,1.75863656568711));
#59084=CARTESIAN_POINT('Ctrl Pts',(16.3272331794214,24.5662888812604,2.49400781955273));
#59085=CARTESIAN_POINT('Ctrl Pts',(17.4003977855862,24.6237236489918,2.55435049990395));
#59086=CARTESIAN_POINT('Ctrl Pts',(16.4218345582109,25.1920672215291,1.60736737169908));
#59087=CARTESIAN_POINT('Ctrl Pts',(16.3470874651384,24.4410877110629,2.36984780965278));
#59088=CARTESIAN_POINT('Ctrl Pts',(17.4170972591065,24.493389351162,2.42065298018113));
#59089=CARTESIAN_POINT('Ctrl Pts',(16.4309764402636,25.0841657011645,1.51053038267463));
#59090=CARTESIAN_POINT('Ctrl Pts',(16.3592331968953,24.3546376676092,2.28990440593928));
#59091=CARTESIAN_POINT('Ctrl Pts',(17.4267931938554,24.4034714176583,2.33506473211196));
#59092=CARTESIAN_POINT('Ctrl Pts',(16.446994092363,24.8611997872063,1.3247921132227));
#59093=CARTESIAN_POINT('Ctrl Pts',(16.3815748016209,24.1756367993131,2.13577662546436));
#59094=CARTESIAN_POINT('Ctrl Pts',(17.4437816134758,24.2176664893174,2.17090212032256));
#59095=CARTESIAN_POINT('Ctrl Pts',(16.4538694171321,24.7461353014014,1.23589090041249));
#59096=CARTESIAN_POINT('Ctrl Pts',(16.3917723398782,24.0831327303185,2.06160077217661));
#59097=CARTESIAN_POINT('Ctrl Pts',(17.4510736238994,24.1217794177785,2.09232781607564));
#59098=CARTESIAN_POINT('Ctrl Pts',(16.4657444941948,24.5088324285203,1.06606911860916));
#59099=CARTESIAN_POINT('Ctrl Pts',(16.41043203463,23.8918442069889,1.91919542169583));
#59100=CARTESIAN_POINT('Ctrl Pts',(17.4636684032655,23.924027023823,1.94223280679702));
#59101=CARTESIAN_POINT('Ctrl Pts',(16.4707439330845,24.3865942689554,0.985148265534012));
#59102=CARTESIAN_POINT('Ctrl Pts',(16.4188978329588,23.7930962833668,1.85095941313437));
#59103=CARTESIAN_POINT('Ctrl Pts',(17.4689708378186,23.8221618906762,1.87071185102215));
#59104=CARTESIAN_POINT('Ctrl Pts',(16.4770987515012,24.1977602110029,0.869883576612304));
#59105=CARTESIAN_POINT('Ctrl Pts',(16.430448838457,23.6399653599251,1.75322510898323));
#59106=CARTESIAN_POINT('Ctrl Pts',(17.4757107971974,23.6648001758957,1.76883649439488));
#59107=CARTESIAN_POINT('Ctrl Pts',(16.4790260107452,24.1339017821622,0.832482487139682));
#59108=CARTESIAN_POINT('Ctrl Pts',(16.4341038189509,23.588155056693,1.72145552621991));
#59109=CARTESIAN_POINT('Ctrl Pts',(17.4777548597382,23.611584818395,1.73577997612498));
#59110=CARTESIAN_POINT('Ctrl Pts',(16.481660834336,24.0367224738724,0.777937966978324));
#59111=CARTESIAN_POINT('Ctrl Pts',(16.439316110871,23.5091625905436,1.67499684370208));
#59112=CARTESIAN_POINT('Ctrl Pts',(17.4805493698219,23.5306020615971,1.68757143540179));
#59113=CARTESIAN_POINT('Ctrl Pts',(16.4824963319283,24.0040971394492,0.76001668658966));
#59114=CARTESIAN_POINT('Ctrl Pts',(16.4410074506687,23.4826353866685,1.65971950289981));
#59115=CARTESIAN_POINT('Ctrl Pts',(17.4814355034805,23.5034142828847,1.67173191994441));
#59116=CARTESIAN_POINT('Ctrl Pts',(16.4840825264792,23.9385710072358,0.724799252308877));
#59117=CARTESIAN_POINT('Ctrl Pts',(16.4442928704461,23.4293188181548,1.62966302113361));
#59118=CARTESIAN_POINT('Ctrl Pts',(17.483117831194,23.4488091726861,1.64060539978915));
#59119=CARTESIAN_POINT('Ctrl Pts',(16.4848338838812,23.9056467056935,0.707489718603382));
#59120=CARTESIAN_POINT('Ctrl Pts',(16.4458883265545,23.402510427123,1.61487200588415));
#59121=CARTESIAN_POINT('Ctrl Pts',(17.4839147252516,23.4213722547508,1.6253065694588));
#59122=CARTESIAN_POINT('Ctrl Pts',(16.4883963136533,23.7402209980604,0.622434816921749));
#59123=CARTESIAN_POINT('Ctrl Pts',(16.4536288557431,23.2678810456568,1.54219914855875));
#59124=CARTESIAN_POINT('Ctrl Pts',(17.4876930602432,23.2835174983592,1.5501317826884));
#59125=CARTESIAN_POINT('Ctrl Pts',(16.4906265194978,23.6053104048751,0.559161466617183));
#59126=CARTESIAN_POINT('Ctrl Pts',(16.4591061096903,23.1576407614143,1.48778409749428));
#59127=CARTESIAN_POINT('Ctrl Pts',(17.4900584295061,23.1710920040299,1.49420836702546));
#59128=CARTESIAN_POINT('Ctrl Pts',(16.4928461382771,23.43345704006,0.486045567387642));
#59129=CARTESIAN_POINT('Ctrl Pts',(16.4651843052487,23.0166721910829,1.4246163879437));
#59130=CARTESIAN_POINT('Ctrl Pts',(17.492412570966,23.0278808667248,1.42958572873525));
#59131=CARTESIAN_POINT('Ctrl Pts',(16.4932615496334,23.3989227879446,0.47172051602756));
#59132=CARTESIAN_POINT('Ctrl Pts',(16.4663600202752,22.988357063806,1.4122411370019));
#59133=CARTESIAN_POINT('Ctrl Pts',(17.4928531586321,22.9991023233164,1.41692469843949));
#59134=CARTESIAN_POINT('Ctrl Pts',(16.4940398122447,23.32954199818,0.443674950772383));
#59135=CARTESIAN_POINT('Ctrl Pts',(16.4686366864973,22.9314333971575,1.38799006257673));
#59136=CARTESIAN_POINT('Ctrl Pts',(17.4936785888143,22.9412849984541,1.39213695150995));
#59137=CARTESIAN_POINT('Ctrl Pts',(16.4944018726065,23.2947668025916,0.42998321641532));
#59138=CARTESIAN_POINT('Ctrl Pts',(16.4697353860784,22.9028829800878,1.37613850024778));
#59139=CARTESIAN_POINT('Ctrl Pts',(17.494062592092,22.912305668851,1.3800356710121));
#59140=CARTESIAN_POINT('Ctrl Pts',(16.4954144797531,23.19018912733,0.389892224755595));
#59141=CARTESIAN_POINT('Ctrl Pts',(16.4729170185102,22.8170009119346,1.34141701125129));
#59142=CARTESIAN_POINT('Ctrl Pts',(17.4951365695679,22.825157606059,1.34460171392323));
#59143=CARTESIAN_POINT('Ctrl Pts',(16.4959915982081,23.1201346539405,0.364476810515272));
#59144=CARTESIAN_POINT('Ctrl Pts',(16.4748883009626,22.7593742589264,1.31935155897431));
#59145=CARTESIAN_POINT('Ctrl Pts',(17.4957486646468,22.766778878317,1.32213859505898));
#59146=CARTESIAN_POINT('Ctrl Pts',(16.4974846918856,22.908978123431,0.292108636005814));
#59147=CARTESIAN_POINT('Ctrl Pts',(16.480387411174,22.585590732172,1.25646842577618));
#59148=CARTESIAN_POINT('Ctrl Pts',(17.4973322492083,22.5908151027927,1.25817682493942));
#59149=CARTESIAN_POINT('Ctrl Pts',(16.4981644144038,22.7668843481313,0.249028531548178));
#59150=CARTESIAN_POINT('Ctrl Pts',(16.4835124139739,22.4682695938112,1.21884858897264));
#59151=CARTESIAN_POINT('Ctrl Pts',(17.498053166605,22.4724036234601,1.2201009747895));
#59152=CARTESIAN_POINT('Ctrl Pts',(16.4991365090799,22.4800959201519,0.173028058336329));
#59153=CARTESIAN_POINT('Ctrl Pts',(16.4888528045335,22.2310570860755,1.15235685094956));
#59154=CARTESIAN_POINT('Ctrl Pts',(17.4990841764838,22.2334132667759,1.15292883950236));
#59155=CARTESIAN_POINT('Ctrl Pts',(16.4994286224241,22.3354012063648,0.140107924718887));
#59156=CARTESIAN_POINT('Ctrl Pts',(16.4910714022229,22.1111134362735,1.12345029266905));
#59157=CARTESIAN_POINT('Ctrl Pts',(17.4993939933432,22.1128343386246,1.12383276180865));
#59158=CARTESIAN_POINT('Ctrl Pts',(16.4998074835914,22.0434113899889,0.0844280845233825));
#59159=CARTESIAN_POINT('Ctrl Pts',(16.4947342938488,21.8687662112482,1.07450481854977));
#59160=CARTESIAN_POINT('Ctrl Pts',(17.4997958160672,21.8695094916702,1.07462078171355));
#59161=CARTESIAN_POINT('Ctrl Pts',(16.4998941390599,21.8961163485439,0.0616681376515486));
#59162=CARTESIAN_POINT('Ctrl Pts',(16.4961809127729,21.7463003703735,1.0544381008806));
#59163=CARTESIAN_POINT('Ctrl Pts',(17.4998877231583,21.7467636237625,1.05450466730936));
#59164=CARTESIAN_POINT('Ctrl Pts',(16.4999646344616,21.6731910279211,0.0352767822043904));
#59165=CARTESIAN_POINT('Ctrl Pts',(16.4978347597081,21.5607763684425,1.03115602986482));
#59166=CARTESIAN_POINT('Ctrl Pts',(17.4999624911392,21.5609925232796,1.031178974074));
#59167=CARTESIAN_POINT('Ctrl Pts',(16.4999777889481,21.5985517799239,0.0277724453695535));
#59168=CARTESIAN_POINT('Ctrl Pts',(16.4982997216056,21.4986420637007,1.0245316792856));
#59169=CARTESIAN_POINT('Ctrl Pts',(17.499976442793,21.4987931499252,1.02454635336124));
#59170=CARTESIAN_POINT('Ctrl Pts',(16.4999899371909,21.4860893308933,0.0184840127014977));
#59171=CARTESIAN_POINT('Ctrl Pts',(16.4988720208443,21.4049879523016,1.01633002306669));
#59172=CARTESIAN_POINT('Ctrl Pts',(17.499989327339,21.4050744424167,1.01633687984765));
#59173=CARTESIAN_POINT('Ctrl Pts',(16.4999926953601,21.448517894679,0.0157159728075137));
#59174=CARTESIAN_POINT('Ctrl Pts',(16.4990419025216,21.3736970698179,1.01388537562505));
#59175=CARTESIAN_POINT('Ctrl Pts',(17.4999922526425,21.3737649122275,1.01389038008064));
#59176=CARTESIAN_POINT('Ctrl Pts',(16.4999966178257,21.3732055924448,0.0108420698560791));
#59177=CARTESIAN_POINT('Ctrl Pts',(16.4993402987244,21.3109670684979,1.00958040502331));
#59178=CARTESIAN_POINT('Ctrl Pts',(17.4999964128575,21.3110046603757,1.00958263742506));
#59179=CARTESIAN_POINT('Ctrl Pts',(16.4999977775395,21.3355743663222,0.00874340271113735));
#59180=CARTESIAN_POINT('Ctrl Pts',(16.4994683856541,21.2796180343658,1.00772626682737));
#59181=CARTESIAN_POINT('Ctrl Pts',(17.499997642836,21.2796453052717,1.0077277548556));
#59182=CARTESIAN_POINT('Ctrl Pts',(16.5000015057495,21.1476258471459,-6.83792717788806E-5));
#59183=CARTESIAN_POINT('Ctrl Pts',(16.5000052077858,21.1230590208582,0.999941955565308));
#59184=CARTESIAN_POINT('Ctrl Pts',(17.5000015970427,21.1230215392753,0.999939564038385));
#59185=CARTESIAN_POINT('Ctrl Pts',(16.5000002892947,20.9978414168731,-0.00175010211135428));
#59186=CARTESIAN_POINT('Ctrl Pts',(16.5001062656831,20.9981824204012,0.998453734603185));
#59187=CARTESIAN_POINT('Ctrl Pts',(17.5000003068456,20.9982011807243,0.998453192447992));
#59188=CARTESIAN_POINT('Ctrl Pts',(16.4999995141463,20.6993924312047,0.00535189244501871));
#59189=CARTESIAN_POINT('Ctrl Pts',(16.499675246758,20.7494912128809,1.00473020199914));
#59190=CARTESIAN_POINT('Ctrl Pts',(17.4999994846828,20.7494936926738,1.00473020809944));
#59191=CARTESIAN_POINT('Ctrl Pts',(16.4999998611331,20.5507279300157,0.0141361157985634));
#59192=CARTESIAN_POINT('Ctrl Pts',(16.4991427830948,20.6255982356581,1.01249911380526));
#59193=CARTESIAN_POINT('Ctrl Pts',(17.4999998527873,20.6256066083462,1.01249404173988));
#59194=CARTESIAN_POINT('Ctrl Pts',(16.4999522523993,20.2545094474017,0.0420822492766633));
#59195=CARTESIAN_POINT('Ctrl Pts',(16.4974126080831,20.379000809699,1.03716536090374));
#59196=CARTESIAN_POINT('Ctrl Pts',(17.4999493585349,20.378757872835,1.03719390719024));
#59197=CARTESIAN_POINT('Ctrl Pts',(16.4999043691725,20.106955309657,0.0612441917327677));
#59198=CARTESIAN_POINT('Ctrl Pts',(16.49621379071,20.2562217364147,1.05407787581568));
#59199=CARTESIAN_POINT('Ctrl Pts',(17.4998985730686,20.255796045571,1.05412997524387));
#59200=CARTESIAN_POINT('Ctrl Pts',(16.4997777634116,19.9599613252167,0.0856373635093353));
#59201=CARTESIAN_POINT('Ctrl Pts',(16.494639994887,20.1341916960038,1.07553284116397));
#59202=CARTESIAN_POINT('Ctrl Pts',(17.4997642945274,20.1333011043472,1.07568958896027));
#59203=CARTESIAN_POINT('',(16.5375681109059,20.0478523395152,0.351922735556661));
#59204=CARTESIAN_POINT('Ctrl Pts',(17.4999100362562,20.3177786532602,1.04676003808511));
#59205=CARTESIAN_POINT('Ctrl Pts',(17.497412412154,20.317337698044,1.04682077239613));
#59206=CARTESIAN_POINT('Ctrl Pts',(17.4949148321613,20.3168954823132,1.0468722967329));
#59207=CARTESIAN_POINT('Ctrl Pts',(17.4924172962765,20.316452006012,1.04691461131551));
#59208=CARTESIAN_POINT('Ctrl Pts',(17.4915847843149,20.3163041805782,1.04692871617638));
#59209=CARTESIAN_POINT('Ctrl Pts',(17.490762085069,20.3161579632937,1.04694165678216));
#59210=CARTESIAN_POINT('Ctrl Pts',(17.489917898285,20.3160077756803,1.04695388308451));
#59211=CARTESIAN_POINT('Ctrl Pts',(17.4865411511487,20.3154070252269,1.04700278829394));
#59212=CARTESIAN_POINT('Ctrl Pts',(17.4831669066207,20.3148043885298,1.04703482418623));
#59213=CARTESIAN_POINT('Ctrl Pts',(17.4797951548174,20.3141998724626,1.04705005790662));
#59214=CARTESIAN_POINT('Ctrl Pts',(17.4730516512108,20.3129908403283,1.0470805253474));
#59215=CARTESIAN_POINT('Ctrl Pts',(17.4663181182136,20.3117742914819,1.04704378959848));
#59216=CARTESIAN_POINT('Ctrl Pts',(17.4595944841994,20.3105502727928,1.04694032080793));
#59217=CARTESIAN_POINT('Ctrl Pts',(17.446147216171,20.3081022354146,1.04673338322681));
#59218=CARTESIAN_POINT('Ctrl Pts',(17.4327395412199,20.3056243303144,1.04625959729685));
#59219=CARTESIAN_POINT('Ctrl Pts',(17.4193710601051,20.3031168246039,1.04552169141653));
#59220=CARTESIAN_POINT('Ctrl Pts',(17.3926340978756,20.2981018131829,1.0440458796559));
#59221=CARTESIAN_POINT('Ctrl Pts',(17.3660537227381,20.2929685399409,1.04151486242535));
#59222=CARTESIAN_POINT('Ctrl Pts',(17.3396290846692,20.287717410052,1.03793473510459));
#59223=CARTESIAN_POINT('Ctrl Pts',(17.3132044466002,20.2824662801631,1.03435460778383));
#59224=CARTESIAN_POINT('Ctrl Pts',(17.2869355447269,20.2770972972993,1.02972539672272));
#59225=CARTESIAN_POINT('Ctrl Pts',(17.2608245587767,20.2716085915521,1.02403256038389));
#59226=CARTESIAN_POINT('Ctrl Pts',(17.2477690658017,20.2688642386785,1.02118614221447));
#59227=CARTESIAN_POINT('Ctrl Pts',(17.234753135717,20.2660899091362,1.01807350559858));
#59228=CARTESIAN_POINT('Ctrl Pts',(17.2217772917725,20.2632851599956,1.01469078953784));
#59229=CARTESIAN_POINT('Ctrl Pts',(17.2152893698003,20.2618827854253,1.01299943150747));
#59230=CARTESIAN_POINT('Ctrl Pts',(17.2088052768564,20.2604714323889,1.01123870857771));
#59231=CARTESIAN_POINT('Ctrl Pts',(17.20235370637,20.2590573280976,1.009416302857));
#59232=CARTESIAN_POINT('Ctrl Pts',(17.1959021358836,20.2576432238063,1.0075938971363));
#59233=CARTESIAN_POINT('Ctrl Pts',(17.1894803216323,20.2562257911111,1.00570923654773));
#59234=CARTESIAN_POINT('Ctrl Pts',(17.1830880283661,20.2548050536997,1.00376281463061));
#59235=CARTESIAN_POINT('Ctrl Pts',(17.1575188553016,20.249122104054,0.99597712696212));
#59236=CARTESIAN_POINT('Ctrl Pts',(17.1324212808169,20.2433863569365,0.987204804132461));
#59237=CARTESIAN_POINT('Ctrl Pts',(17.1077863027231,20.2375986909455,0.977464745590708));
#59238=CARTESIAN_POINT('Ctrl Pts',(17.0831513246293,20.2318110249545,0.967724687048955));
#59239=CARTESIAN_POINT('Ctrl Pts',(17.0589789712759,20.225971430241,0.957016828161272));
#59240=CARTESIAN_POINT('Ctrl Pts',(17.0352693339654,20.2200798256262,0.945341032704729));
#59241=CARTESIAN_POINT('Ctrl Pts',(17.0115596966549,20.2141882210115,0.933665237248187));
#59242=CARTESIAN_POINT('Ctrl Pts',(16.988312746797,20.2082446154472,0.921021563266389));
#59243=CARTESIAN_POINT('Ctrl Pts',(16.9655376048733,20.2022479693789,0.907390857660355));
#59244=CARTESIAN_POINT('Ctrl Pts',(16.9541500339115,20.1992496463448,0.900575504857338));
#59245=CARTESIAN_POINT('Ctrl Pts',(16.9428805950743,20.1962380202549,0.893513121755632));
#59246=CARTESIAN_POINT('Ctrl Pts',(16.9317313026216,20.1932128989287,0.886199374602489));
#59247=CARTESIAN_POINT('Ctrl Pts',(16.9261566563953,20.1917003382657,0.882542501025918));
#59248=CARTESIAN_POINT('Ctrl Pts',(16.9206120585836,20.1901844007644,0.878822767087584));
#59249=CARTESIAN_POINT('Ctrl Pts',(16.9150978270253,20.1886650515396,0.875039504162688));
#59250=CARTESIAN_POINT('Ctrl Pts',(16.9095835954671,20.1871457023148,0.871256241237792));
#59251=CARTESIAN_POINT('Ctrl Pts',(16.9041070265371,20.1856249264553,0.867414287379847));
#59252=CARTESIAN_POINT('Ctrl Pts',(16.8986841658931,20.184107238926,0.863525316408129));
#59253=CARTESIAN_POINT('Ctrl Pts',(16.8769927233169,20.1780364888088,0.847969432521257));
#59254=CARTESIAN_POINT('Ctrl Pts',(16.8560810285277,20.1719935559081,0.831609081359371));
#59255=CARTESIAN_POINT('Ctrl Pts',(16.835932407024,20.1659779433814,0.814461434518674));
#59256=CARTESIAN_POINT('Ctrl Pts',(16.8157837855203,20.1599623308546,0.797313787677976));
#59257=CARTESIAN_POINT('Ctrl Pts',(16.796398295399,20.153974028425,0.779378781668851));
#59258=CARTESIAN_POINT('Ctrl Pts',(16.7777743700881,20.1480131320867,0.76065799712203));
#59259=CARTESIAN_POINT('Ctrl Pts',(16.7591504447772,20.1420522357484,0.741937212575208));
#59260=CARTESIAN_POINT('Ctrl Pts',(16.7412880466671,20.1361187517238,0.722430687544411));
#59261=CARTESIAN_POINT('Ctrl Pts',(16.7242005076968,20.1302133641119,0.702124551441759));
#59262=CARTESIAN_POINT('Ctrl Pts',(16.7156567382117,20.127260670306,0.691971483390434));
#59263=CARTESIAN_POINT('Ctrl Pts',(16.7073069447631,20.1243149669166,0.681618309087091));
#59264=CARTESIAN_POINT('Ctrl Pts',(16.6991542585567,20.1213764519223,0.67106171344245));
#59265=CARTESIAN_POINT('Ctrl Pts',(16.6950779154534,20.1199071944251,0.665783415620129));
#59266=CARTESIAN_POINT('Ctrl Pts',(16.6910508666661,20.1184397316079,0.660454247788119));
#59267=CARTESIAN_POINT('Ctrl Pts',(16.6870736074572,20.1169740855827,0.65507369560794));
#59268=CARTESIAN_POINT('Ctrl Pts',(16.6830963482483,20.1155084395574,0.649693143427761));
#59269=CARTESIAN_POINT('Ctrl Pts',(16.6791647000557,20.1140430113909,0.644255147297184));
#59270=CARTESIAN_POINT('Ctrl Pts',(16.6752988732391,20.1125852953334,0.638787354378224));
#59271=CARTESIAN_POINT('Ctrl Pts',(16.6598355659724,20.1067544311035,0.616916182702385));
#59272=CARTESIAN_POINT('Ctrl Pts',(16.6453887468324,20.1010345149467,0.594526308078098));
#59273=CARTESIAN_POINT('Ctrl Pts',(16.6319321474346,20.095422943538,0.571631075588535));
#59274=CARTESIAN_POINT('Ctrl Pts',(16.6184755480369,20.0898113721293,0.548735843098972));
#59275=CARTESIAN_POINT('Ctrl Pts',(16.6060092707311,20.084308135995,0.525335196488614));
#59276=CARTESIAN_POINT('Ctrl Pts',(16.594527070435,20.0789128413188,0.501432270733023));
#59277=CARTESIAN_POINT('Ctrl Pts',(16.583044870139,20.0735175466426,0.477529344977431));
#59278=CARTESIAN_POINT('Ctrl Pts',(16.572546719852,20.0682301946996,0.453124147417704));
#59279=CARTESIAN_POINT('Ctrl Pts',(16.5630457927051,20.0630525023684,0.428209898952689));
#59280=CARTESIAN_POINT('Ctrl Pts',(16.5535448655582,20.0578748100371,0.403295650487674));
#59281=CARTESIAN_POINT('Ctrl Pts',(16.54504099411,20.0528067872061,0.377872409037217));
#59282=CARTESIAN_POINT('Ctrl Pts',(16.5375681503014,20.0478524311852,0.35192279925056));
#59283=CARTESIAN_POINT('Ctrl Pts',(16.4999922300468,20.5440053495025,0.0163638449572259));
#59284=CARTESIAN_POINT('Ctrl Pts',(16.4999770343612,20.5198614768197,0.0316719654762678));
#59285=CARTESIAN_POINT('Ctrl Pts',(16.5002263989813,20.4961497241895,0.0468431030935451));
#59286=CARTESIAN_POINT('Ctrl Pts',(16.5020179270435,20.412886263937,0.100672073666557));
#59287=CARTESIAN_POINT('Ctrl Pts',(16.5049029406463,20.3540801618161,0.139580047345334));
#59288=CARTESIAN_POINT('Ctrl Pts',(16.5156498028587,20.2121142842092,0.235607659679802));
#59289=CARTESIAN_POINT('Ctrl Pts',(16.5251347070846,20.1294122583419,0.29333516665824));
#59290=CARTESIAN_POINT('Ctrl Pts',(16.5375680971716,20.0478522665949,0.351922636958438));
#59291=CARTESIAN_POINT('Ctrl Pts',(16.4260332126742,25.1379309164222,1.56059122805689));
#59292=CARTESIAN_POINT('Ctrl Pts',(16.4226910805317,25.1576364103843,1.59576908821006));
#59293=CARTESIAN_POINT('Ctrl Pts',(16.4195841592766,25.176720276254,1.62999587635092));
#59294=CARTESIAN_POINT('Ctrl Pts',(16.4010380336176,25.2940925947309,1.84168171849569));
#59295=CARTESIAN_POINT('Ctrl Pts',(16.3882950542161,25.3896976994372,2.01860511761247));
#59296=CARTESIAN_POINT('Ctrl Pts',(16.3564248514291,25.5987026766223,2.41684917061561));
#59297=CARTESIAN_POINT('Ctrl Pts',(16.3372998166613,25.7068837309083,2.63036802356939));
#59298=CARTESIAN_POINT('Ctrl Pts',(16.3099522015712,25.8138525750283,2.84895274231535));
#59299=CARTESIAN_POINT('Ctrl Pts',(12.0866114872764,19.9820083891277,11.2322670354491));
#59300=CARTESIAN_POINT('Ctrl Pts',(12.3807269288992,20.0835512235879,10.9157806962192));
#59301=CARTESIAN_POINT('Ctrl Pts',(12.8191333955962,20.1516736576064,10.9275087434525));
#59302=CARTESIAN_POINT('Ctrl Pts',(12.0675878268092,20.1081184594252,11.2527376663919));
#59303=CARTESIAN_POINT('Ctrl Pts',(12.3622278967634,20.1967330860491,10.9367605323266));
#59304=CARTESIAN_POINT('Ctrl Pts',(12.7989568015267,20.2567653007514,10.9456014580243));
#59305=CARTESIAN_POINT('Ctrl Pts',(12.0519050645098,20.2355538181535,11.2695119158229));
#59306=CARTESIAN_POINT('Ctrl Pts',(12.3469366141942,20.3114015985704,10.9539972243665));
#59307=CARTESIAN_POINT('Ctrl Pts',(12.7823235531825,20.3629615151636,10.9604271979261));
#59308=CARTESIAN_POINT('Ctrl Pts',(12.0337154085966,20.4287937461634,11.288922538981));
#59309=CARTESIAN_POINT('Ctrl Pts',(12.3292036429553,20.4853989396882,10.9739392026073));
#59310=CARTESIAN_POINT('Ctrl Pts',(12.7630314940089,20.5239947884517,10.9775830523308));
#59311=CARTESIAN_POINT('Ctrl Pts',(12.0285416186745,20.4935550919164,11.2944333696097));
#59312=CARTESIAN_POINT('Ctrl Pts',(12.3241592547639,20.5437171707118,10.9796013224493));
#59313=CARTESIAN_POINT('Ctrl Pts',(12.757544140988,20.5779625766115,10.9824537355451));
#59314=CARTESIAN_POINT('Ctrl Pts',(12.0221588199083,20.5912338278851,11.3012259052763));
#59315=CARTESIAN_POINT('Ctrl Pts',(12.3179359141494,20.6317011591869,10.9865804526371));
#59316=CARTESIAN_POINT('Ctrl Pts',(12.7507745059785,20.6593615232303,10.9884572396224));
#59317=CARTESIAN_POINT('Ctrl Pts',(12.0202608919841,20.6238828763539,11.3032444010669));
#59318=CARTESIAN_POINT('Ctrl Pts',(12.3160853794008,20.6611104736368,10.9886544060349));
#59319=CARTESIAN_POINT('Ctrl Pts',(12.7487615520924,20.6865690636343,10.9902412634538));
#59320=CARTESIAN_POINT('Ctrl Pts',(12.0177642067175,20.6729926478103,11.3058986793241));
#59321=CARTESIAN_POINT('Ctrl Pts',(12.3136509329996,20.7053522841239,10.9913817152174));
#59322=CARTESIAN_POINT('Ctrl Pts',(12.7461135525852,20.7274938731722,10.9925872166321));
#59323=CARTESIAN_POINT('Ctrl Pts',(12.0169904627187,20.6893850602612,11.3067210676687));
#59324=CARTESIAN_POINT('Ctrl Pts',(12.3128964800711,20.7201199078126,10.9922267255499));
#59325=CARTESIAN_POINT('Ctrl Pts',(12.7452929149993,20.7411542168826,10.9933140749918));
#59326=CARTESIAN_POINT('Ctrl Pts',(12.0155640244321,20.7221292061764,11.3082369208426));
#59327=CARTESIAN_POINT('Ctrl Pts',(12.311505593863,20.7496195010182,10.9937842864445));
#59328=CARTESIAN_POINT('Ctrl Pts',(12.7437800259182,20.7684410051488,10.994653844147));
#59329=CARTESIAN_POINT('Ctrl Pts',(12.0149107569711,20.7384917126866,11.3089309950962));
#59330=CARTESIAN_POINT('Ctrl Pts',(12.3108685826693,20.764361377477,10.9944974844729));
#59331=CARTESIAN_POINT('Ctrl Pts',(12.7430871664801,20.7820764272374,10.9952672936768));
#59332=CARTESIAN_POINT('Ctrl Pts',(12.0095689908778,20.8856685275638,11.3146056335284));
#59333=CARTESIAN_POINT('Ctrl Pts',(12.3056609603354,20.8969330014969,11.0003271040206));
#59334=CARTESIAN_POINT('Ctrl Pts',(12.7374216570268,20.9047237729811,11.0002827566569));
#59335=CARTESIAN_POINT('Ctrl Pts',(12.0086433373455,21.0158830521051,11.3155866742477));
#59336=CARTESIAN_POINT('Ctrl Pts',(12.3047572432467,21.0143356842118,11.0013363733449));
#59337=CARTESIAN_POINT('Ctrl Pts',(12.7364399032656,21.0132358767584,11.0011498385414));
#59338=CARTESIAN_POINT('Ctrl Pts',(12.0142277814707,21.2751278248493,11.3096572627521));
#59339=CARTESIAN_POINT('Ctrl Pts',(12.3102031016944,21.2479351155163,10.9952432127086));
#59340=CARTESIAN_POINT('Ctrl Pts',(12.7423627985092,21.2292731873702,10.9959091966857));
#59341=CARTESIAN_POINT('Ctrl Pts',(12.0207379593602,21.4041580408216,11.302746481911));
#59342=CARTESIAN_POINT('Ctrl Pts',(12.3165572121242,21.3642312602987,10.9881354276293));
#59343=CARTESIAN_POINT('Ctrl Pts',(12.7492675327281,21.3367983673583,10.9898011836399));
#59344=CARTESIAN_POINT('Ctrl Pts',(12.0409988281294,21.6610588333447,11.2811597960023));
#59345=CARTESIAN_POINT('Ctrl Pts',(12.3363065386174,21.595548212528,10.9659614584083));
#59346=CARTESIAN_POINT('Ctrl Pts',(12.7707563327911,21.5508823611137,10.9707220417886));
#59347=CARTESIAN_POINT('Ctrl Pts',(12.0547495047205,21.7889294026305,11.2664837866553));
#59348=CARTESIAN_POINT('Ctrl Pts',(12.349718084816,21.7106645499933,10.9508766506942));
#59349=CARTESIAN_POINT('Ctrl Pts',(12.7853403839175,21.6574411688554,10.9577508216129));
#59350=CARTESIAN_POINT('Ctrl Pts',(12.0806691551057,21.9798772439527,11.238665107521));
#59351=CARTESIAN_POINT('Ctrl Pts',(12.3749467442548,21.8822386065852,10.922339947102));
#59352=CARTESIAN_POINT('Ctrl Pts',(12.8128309220202,21.8165643699622,10.9331636050952));
#59353=CARTESIAN_POINT('Ctrl Pts',(12.0901914143202,22.043383452334,11.2284239908148));
#59354=CARTESIAN_POINT('Ctrl Pts',(12.3842191682733,21.9393067824406,10.9118296385023));
#59355=CARTESIAN_POINT('Ctrl Pts',(12.8229302879886,21.869486210272,10.9241121131162));
#59356=CARTESIAN_POINT('Ctrl Pts',(12.1057822814319,22.1384289822797,11.2116053173785));
#59357=CARTESIAN_POINT('Ctrl Pts',(12.399387260399,22.024630165775,10.8945839141828));
#59358=CARTESIAN_POINT('Ctrl Pts',(12.8394660560276,21.9486908185696,10.9092471239345));
#59359=CARTESIAN_POINT('Ctrl Pts',(12.1111971576597,22.1700751906362,11.2057562102194));
#59360=CARTESIAN_POINT('Ctrl Pts',(12.4046562361949,22.0530398313492,10.8885851232551));
#59361=CARTESIAN_POINT('Ctrl Pts',(12.8452091066483,21.9750626588589,10.9040774585348));
#59362=CARTESIAN_POINT('Ctrl Pts',(12.1196444127229,22.2174911125637,11.1966171908215));
#59363=CARTESIAN_POINT('Ctrl Pts',(12.4128724109568,22.0955840554947,10.8792160256234));
#59364=CARTESIAN_POINT('Ctrl Pts',(12.8541683165045,22.0145759271388,10.896000042389));
#59365=CARTESIAN_POINT('Ctrl Pts',(12.1225150265228,22.233290970441,11.1935091880825));
#59366=CARTESIAN_POINT('Ctrl Pts',(12.415664714645,22.1097605880446,10.8760295004639));
#59367=CARTESIAN_POINT('Ctrl Pts',(12.8572129069367,22.0277424753804,10.8932530703498));
#59368=CARTESIAN_POINT('Ctrl Pts',(12.1283510335089,22.2648029487245,11.1871855137895));
#59369=CARTESIAN_POINT('Ctrl Pts',(12.4213408466648,22.1380298284887,10.869546765911));
#59370=CARTESIAN_POINT('Ctrl Pts',(12.8634026112788,22.0540024572575,10.887663964133));
#59371=CARTESIAN_POINT('Ctrl Pts',(12.1313179098281,22.2805235674223,11.1839682389273));
#59372=CARTESIAN_POINT('Ctrl Pts',(12.4242261847655,22.1521303131032,10.8662488345689));
#59373=CARTESIAN_POINT('Ctrl Pts',(12.8665492983217,22.0671029728649,10.8848204132664));
#59374=CARTESIAN_POINT('Ctrl Pts',(12.158453868661,22.4216940521507,11.1545177680223));
#59375=CARTESIAN_POINT('Ctrl Pts',(12.4506457697523,22.2788848408611,10.836026130008));
#59376=CARTESIAN_POINT('Ctrl Pts',(12.8953298605484,22.1847450433553,10.8587909560006));
#59377=CARTESIAN_POINT('Ctrl Pts',(12.185657553851,22.5449416423991,11.1248253769103));
#59378=CARTESIAN_POINT('Ctrl Pts',(12.4770970806105,22.3892794656903,10.8055914845914));
#59379=CARTESIAN_POINT('Ctrl Pts',(12.9241822542658,22.2874513687631,10.8325476820865));
#59380=CARTESIAN_POINT('Ctrl Pts',(12.2456284410546,22.7872847696196,11.0587781318782));
#59381=CARTESIAN_POINT('Ctrl Pts',(12.5352981208323,22.6058827713513,10.7380176167549));
#59382=CARTESIAN_POINT('Ctrl Pts',(12.987787740331,22.4894039745858,10.7741725908326));
#59383=CARTESIAN_POINT('Ctrl Pts',(12.2783962022139,22.9063798510103,11.0224225011533));
#59384=CARTESIAN_POINT('Ctrl Pts',(12.5670873483069,22.7121519963084,10.7008302239268));
#59385=CARTESIAN_POINT('Ctrl Pts',(13.0225414267954,22.5886498759212,10.7420400897768));
#59386=CARTESIAN_POINT('Ctrl Pts',(12.348978997876,23.1406674713625,10.9432869286375));
#59387=CARTESIAN_POINT('Ctrl Pts',(12.6354186655169,22.9206728285625,10.6200488154105));
#59388=CARTESIAN_POINT('Ctrl Pts',(13.0974019672394,22.7838895593894,10.672097032513));
#59389=CARTESIAN_POINT('Ctrl Pts',(12.3867944287769,23.2558597170703,10.9005065193677));
#59390=CARTESIAN_POINT('Ctrl Pts',(12.6720038124617,23.0229760377839,10.5764003243843));
#59391=CARTESIAN_POINT('Ctrl Pts',(13.137509242867,22.8798830976101,10.634286065381));
#59392=CARTESIAN_POINT('Ctrl Pts',(12.4469685868315,23.4258627923054,10.831615883529));
#59393=CARTESIAN_POINT('Ctrl Pts',(12.7300143003336,23.173317069492,10.5063568717909));
#59394=CARTESIAN_POINT('Ctrl Pts',(13.2013303192544,23.0215523268955,10.5733978767148));
#59395=CARTESIAN_POINT('Ctrl Pts',(12.4676023227972,23.4820658196941,10.8078648704614));
#59396=CARTESIAN_POINT('Ctrl Pts',(12.7499178282157,23.2230124750191,10.4821924416464));
#59397=CARTESIAN_POINT('Ctrl Pts',(13.2232145849018,23.0683881830955,10.552405819973));
#59398=CARTESIAN_POINT('Ctrl Pts',(12.4993789165946,23.5656872650545,10.7710625930677));
#59399=CARTESIAN_POINT('Ctrl Pts',(12.7805178446485,23.2967857258851,10.4448117710785));
#59400=CARTESIAN_POINT('Ctrl Pts',(13.2569170326935,23.1380727208702,10.5198785544187));
#59401=CARTESIAN_POINT('Ctrl Pts',(12.5101166355672,23.5934665898445,10.7585899951691));
#59402=CARTESIAN_POINT('Ctrl Pts',(12.7908606252549,23.3212906461701,10.4321395053253));
#59403=CARTESIAN_POINT('Ctrl Pts',(13.2683055226197,23.1612221582558,10.508854793852));
#59404=CARTESIAN_POINT('Ctrl Pts',(12.53179209151,23.6486249072268,10.7333342394064));
#59405=CARTESIAN_POINT('Ctrl Pts',(12.8117286055676,23.3699078275031,10.4064914643755));
#59406=CARTESIAN_POINT('Ctrl Pts',(13.2912946424622,23.2071874226369,10.4865327872123));
#59407=CARTESIAN_POINT('Ctrl Pts',(12.5427358651168,23.6760204684585,10.7205441432531));
#59408=CARTESIAN_POINT('Ctrl Pts',(12.8222602521224,23.3940350953736,10.3935077573717));
#59409=CARTESIAN_POINT('Ctrl Pts',(13.3029016751728,23.2300170570987,10.4752284095746));
#59410=CARTESIAN_POINT('Ctrl Pts',(12.5979638689366,23.8121011103179,10.6557938094435));
#59411=CARTESIAN_POINT('Ctrl Pts',(12.8754924750573,23.5140302972315,10.3276719371624));
#59412=CARTESIAN_POINT('Ctrl Pts',(13.3614768304949,23.3434175917318,10.4179995785188));
#59413=CARTESIAN_POINT('Ctrl Pts',(12.643771837576,23.9180998292818,10.601437989252));
#59414=CARTESIAN_POINT('Ctrl Pts',(12.919492062782,23.6069903768932,10.2725850710442));
#59415=CARTESIAN_POINT('Ctrl Pts',(13.4100610400541,23.4317498578972,10.369957819201));
#59416=CARTESIAN_POINT('Ctrl Pts',(12.7381614324257,24.124811694524,10.487835670056));
#59417=CARTESIAN_POINT('Ctrl Pts',(13.0099210300387,23.7875812880369,10.157752716871));
#59418=CARTESIAN_POINT('Ctrl Pts',(13.5101712160083,23.6040097452743,10.2695517281672));
#59419=CARTESIAN_POINT('Ctrl Pts',(12.786743768146,24.2255239557177,10.4285885456025));
#59420=CARTESIAN_POINT('Ctrl Pts',(13.0563860864973,23.8752192933041,10.0979525157025));
#59421=CARTESIAN_POINT('Ctrl Pts',(13.5616979361181,23.6879366298853,10.2171868461805));
#59422=CARTESIAN_POINT('Ctrl Pts',(12.8862872577475,24.4219918048204,10.3053324039794));
#59423=CARTESIAN_POINT('Ctrl Pts',(13.151326026437,24.0454360470123,9.97389759363243));
#59424=CARTESIAN_POINT('Ctrl Pts',(13.667274364072,23.8516598372297,10.1082483365308));
#59425=CARTESIAN_POINT('Ctrl Pts',(12.937248915859,24.517746816217,10.2413230126633));
#59426=CARTESIAN_POINT('Ctrl Pts',(13.1998342286936,24.1280161508586,9.90958748677937));
#59427=CARTESIAN_POINT('Ctrl Pts',(13.7213246079408,23.9314556802555,10.0516743801166));
#59428=CARTESIAN_POINT('Ctrl Pts',(13.041219018545,24.7045359647819,10.1085959989972));
#59429=CARTESIAN_POINT('Ctrl Pts',(13.2985011177469,24.2883032081281,9.77665045676705));
#59430=CARTESIAN_POINT('Ctrl Pts',(13.8315959285483,24.0871133039103,9.93436515039151));
#59431=CARTESIAN_POINT('Ctrl Pts',(13.0942278294105,24.795569743092,10.0398781851834));
#59432=CARTESIAN_POINT('Ctrl Pts',(13.3486907582046,24.3660062569181,9.7079672620327));
#59433=CARTESIAN_POINT('Ctrl Pts',(13.8878173950481,24.1629747859347,9.87362970929413));
#59434=CARTESIAN_POINT('Ctrl Pts',(13.2020102216455,24.9730727963289,9.89772107757119));
#59435=CARTESIAN_POINT('Ctrl Pts',(13.4504091689276,24.5166541489231,9.56636618824304));
#59436=CARTESIAN_POINT('Ctrl Pts',(14.0021320530417,24.310893996916,9.74798580071625));
#59437=CARTESIAN_POINT('Ctrl Pts',(13.2567840727296,25.0595418800033,9.82428174061243));
#59438=CARTESIAN_POINT('Ctrl Pts',(13.5019665153703,24.5895901088978,9.49339094237622));
#59439=CARTESIAN_POINT('Ctrl Pts',(14.0602255319109,24.3829515666393,9.68307729610358));
#59440=CARTESIAN_POINT('Ctrl Pts',(13.3262035084363,25.1648285421005,9.72948365953242));
#59441=CARTESIAN_POINT('Ctrl Pts',(13.5668872401933,24.6775576076175,9.39982331745309));
#59442=CARTESIAN_POINT('Ctrl Pts',(14.1338522058603,24.4706904517579,9.59929111319616));
#59443=CARTESIAN_POINT('Ctrl Pts',(13.3401350908287,25.1857457215109,9.71037394265934));
#59444=CARTESIAN_POINT('Ctrl Pts',(13.5799441680015,24.6950553454771,9.3809208785823));
#59445=CARTESIAN_POINT('Ctrl Pts',(14.1486281266942,24.4881214345812,9.58240121196993));
#59446=CARTESIAN_POINT('Ctrl Pts',(13.3680902095933,25.2273004400984,9.67185248522811));
#59447=CARTESIAN_POINT('Ctrl Pts',(13.6061221656083,24.7297560468975,9.34285051244273));
#59448=CARTESIAN_POINT('Ctrl Pts',(14.1782774949656,24.5227503667599,9.54835446924372));
#59449=CARTESIAN_POINT('Ctrl Pts',(13.3821134917764,25.2479373475695,9.6524409830328));
#59450=CARTESIAN_POINT('Ctrl Pts',(13.6192433303242,24.7469581458693,9.32368199427145));
#59451=CARTESIAN_POINT('Ctrl Pts',(14.1931506731412,24.5399477896631,9.53119783858767));
#59452=CARTESIAN_POINT('Ctrl Pts',(13.4242368819105,25.3093150518009,9.59386146914878));
#59453=CARTESIAN_POINT('Ctrl Pts',(13.6586630795446,24.7980792953747,9.26582885724692));
#59454=CARTESIAN_POINT('Ctrl Pts',(14.2378269958757,24.591095876457,9.47942301556463));
#59455=CARTESIAN_POINT('Ctrl Pts',(13.4524167277085,25.3495622852733,9.55431246433107));
#59456=CARTESIAN_POINT('Ctrl Pts',(13.6849643583523,24.8314404027354,9.22687348103602));
#59457=CARTESIAN_POINT('Ctrl Pts',(14.2677147112974,24.6246352377576,9.44446808724288));
#59458=CARTESIAN_POINT('Ctrl Pts',(13.5372063494346,25.4683224074992,9.43417480126614));
#59459=CARTESIAN_POINT('Ctrl Pts',(13.7641233205245,24.9297095823926,9.10852127370187));
#59460=CARTESIAN_POINT('Ctrl Pts',(14.3576430977025,24.7236020061896,9.33828580903671));
#59461=CARTESIAN_POINT('Ctrl Pts',(13.5940653376125,25.5448561996849,9.35209697288459));
#59462=CARTESIAN_POINT('Ctrl Pts',(13.8169186749523,24.9923773886975,9.02809366159298));
#59463=CARTESIAN_POINT('Ctrl Pts',(14.417948085536,24.7873801664062,9.26574227412286));
#59464=CARTESIAN_POINT('Ctrl Pts',(13.6654272847918,25.6372918612587,9.24698560403133));
#59465=CARTESIAN_POINT('Ctrl Pts',(13.8827103346352,25.067184492195,8.92587537114921));
#59466=CARTESIAN_POINT('Ctrl Pts',(14.4936349989743,24.8644098843817,9.17284081161668));
#59467=CARTESIAN_POINT('Ctrl Pts',(13.6797141539562,25.6556172191055,9.22583750988905));
#59468=CARTESIAN_POINT('Ctrl Pts',(13.8959117260276,25.0820279842197,8.90526390781971));
#59469=CARTESIAN_POINT('Ctrl Pts',(14.5087877390924,24.8796810159181,9.1541493143201));
#59470=CARTESIAN_POINT('Ctrl Pts',(13.7083139270417,25.6919453148001,9.18328842901607));
#59471=CARTESIAN_POINT('Ctrl Pts',(13.9223129183792,25.1113853618828,8.86383826463687));
#59472=CARTESIAN_POINT('Ctrl Pts',(14.539120831663,24.9099544290033,9.11654280339907));
#59473=CARTESIAN_POINT('Ctrl Pts',(13.7226326555818,25.7099552850125,9.16187867514917));
#59474=CARTESIAN_POINT('Ctrl Pts',(13.9355182094804,25.1259044915328,8.8430149308617));
#59475=CARTESIAN_POINT('Ctrl Pts',(14.5543073620133,24.9249627375437,9.09762004121136));
#59476=CARTESIAN_POINT('Ctrl Pts',(13.7655806510432,25.7634487878384,9.09733261854258));
#59477=CARTESIAN_POINT('Ctrl Pts',(13.9751305079505,25.1689723680322,8.78023637313619));
#59478=CARTESIAN_POINT('Ctrl Pts',(14.5998582661927,24.9695406564653,9.04057175872457));
#59479=CARTESIAN_POINT('Ctrl Pts',(13.7941780979144,25.7983673942214,9.05391542849186));
#59480=CARTESIAN_POINT('Ctrl Pts',(14.0014262760392,25.1969111868538,8.73814081795549));
#59481=CARTESIAN_POINT('Ctrl Pts',(14.6301888917935,24.9986394952372,9.00219797980234));
#59482=CARTESIAN_POINT('Ctrl Pts',(13.8798356042923,25.9009302358346,8.92250522728221));
#59483=CARTESIAN_POINT('Ctrl Pts',(14.080204374513,25.2787388705709,8.6107394872982));
#59484=CARTESIAN_POINT('Ctrl Pts',(14.7210377619961,25.084108529757,8.88605259972134));
#59485=CARTESIAN_POINT('Ctrl Pts',(13.9367602535074,25.9663840884067,8.83335453123031));
#59486=CARTESIAN_POINT('Ctrl Pts',(14.1322279259698,25.330245918761,8.52486074193159));
#59487=CARTESIAN_POINT('Ctrl Pts',(14.7814123902207,25.1386534070522,8.80725779285579));
#59488=CARTESIAN_POINT('Ctrl Pts',(14.0500984561988,26.0915862509637,8.65194613998907));
#59489=CARTESIAN_POINT('Ctrl Pts',(14.2353745951717,25.4276650654009,8.35098471144773));
#59490=CARTESIAN_POINT('Ctrl Pts',(14.9016195746192,25.242988542423,8.64692209332295));
#59491=CARTESIAN_POINT('Ctrl Pts',(14.1065121739022,26.1513343014395,8.55968841168897));
#59492=CARTESIAN_POINT('Ctrl Pts',(14.2864905523139,25.473527188847,8.26296704102961));
#59493=CARTESIAN_POINT('Ctrl Pts',(14.9614523057975,25.2927785845191,8.56538117201096));
#59494=CARTESIAN_POINT('Ctrl Pts',(14.2186950223458,26.2651812652254,8.37201667934135));
#59495=CARTESIAN_POINT('Ctrl Pts',(14.3876971990642,25.5597553401026,8.0848856095321));
#59496=CARTESIAN_POINT('Ctrl Pts',(15.0804341144655,25.3876510543683,8.39950969127342));
#59497=CARTESIAN_POINT('Ctrl Pts',(14.2744642813816,26.3192800792414,8.27660270041679));
#59498=CARTESIAN_POINT('Ctrl Pts',(14.4377774098147,25.6000699835723,7.99480545474144));
#59499=CARTESIAN_POINT('Ctrl Pts',(15.1395833288898,25.4327333992899,8.31517915444208));
#59500=CARTESIAN_POINT('Ctrl Pts',(14.3852368576413,26.4218103331842,8.08253941101095));
#59501=CARTESIAN_POINT('Ctrl Pts',(14.536806721599,25.6752490298323,7.81265136249611));
#59502=CARTESIAN_POINT('Ctrl Pts',(15.2570693943164,25.5181752777314,8.14365857030466));
#59503=CARTESIAN_POINT('Ctrl Pts',(14.4402402789567,26.4702418187271,7.9838901831176));
#59504=CARTESIAN_POINT('Ctrl Pts',(14.5857421530009,25.71006068656,7.72056538801955));
#59505=CARTESIAN_POINT('Ctrl Pts',(15.3154063566312,25.5585348487929,8.05646859620055));
#59506=CARTESIAN_POINT('Ctrl Pts',(14.5493685169342,26.5613453046831,7.7832459506642));
#59507=CARTESIAN_POINT('Ctrl Pts',(14.682393434828,25.7742304787433,7.53443013914731));
#59508=CARTESIAN_POINT('Ctrl Pts',(15.4311484268895,25.6344544207156,7.87913152204095));
#59509=CARTESIAN_POINT('Ctrl Pts',(14.6034934217443,26.604017500099,7.68125109313529));
#59510=CARTESIAN_POINT('Ctrl Pts',(14.7300925300169,25.803534633669,7.4403736510247));
#59511=CARTESIAN_POINT('Ctrl Pts',(15.4885536292969,25.6700145831945,7.78898455200868));
#59512=CARTESIAN_POINT('Ctrl Pts',(14.6839417041762,26.6635790246801,7.52564054729126));
#59513=CARTESIAN_POINT('Ctrl Pts',(14.8005111418582,25.8432706371624,7.29814620728082));
#59514=CARTESIAN_POINT('Ctrl Pts',(15.5738775649483,25.7196491873441,7.65144997866894));
#59515=CARTESIAN_POINT('Ctrl Pts',(14.7106346565754,26.6826911151509,7.47333370333937));
#59516=CARTESIAN_POINT('Ctrl Pts',(14.8238726296942,25.8558472906946,7.25038337988665));
#59517=CARTESIAN_POINT('Ctrl Pts',(15.6021882722161,25.7355759291614,7.6052191822394));
#59518=CARTESIAN_POINT('Ctrl Pts',(14.7504796027575,26.7102247625861,7.39420202921272));
#59519=CARTESIAN_POINT('Ctrl Pts',(14.8586259533269,25.8736455053003,7.17845152574216));
#59520=CARTESIAN_POINT('Ctrl Pts',(15.6444480634853,25.758520635554,7.53527957127637));
#59521=CARTESIAN_POINT('Ctrl Pts',(14.7637288390933,26.7192135210666,7.36771288292358));
#59522=CARTESIAN_POINT('Ctrl Pts',(14.8701815395122,25.8794092498503,7.15438535620414));
#59523=CARTESIAN_POINT('Ctrl Pts',(15.6585002839332,25.7660112674848,7.51186744702555));
#59524=CARTESIAN_POINT('Ctrl Pts',(14.7901608727406,26.7368086126918,7.31450775636524));
#59525=CARTESIAN_POINT('Ctrl Pts',(14.8932084661783,25.8905852574532,7.10612929617896));
#59526=CARTESIAN_POINT('Ctrl Pts',(15.686534258921,25.7806738439805,7.46484271396204));
#59527=CARTESIAN_POINT('Ctrl Pts',(14.8033451749285,26.7454155612302,7.28778833164477));
#59528=CARTESIAN_POINT('Ctrl Pts',(14.9046806639825,25.8959968778302,7.0819365849418));
#59529=CARTESIAN_POINT('Ctrl Pts',(15.7005176097801,25.7878463010393,7.44122706080441));
#59530=CARTESIAN_POINT('Ctrl Pts',(14.9213099621474,26.8208949071534,7.04707639020546));
#59531=CARTESIAN_POINT('Ctrl Pts',(15.0080298043219,25.9433374988707,6.86262545158575));
#59532=CARTESIAN_POINT('Ctrl Pts',(15.8256317779751,25.8507457558477,7.22847660744676));
#59533=CARTESIAN_POINT('Ctrl Pts',(15.0219275551717,26.8744045260676,6.83003873153216));
#59534=CARTESIAN_POINT('Ctrl Pts',(15.0944925963321,25.9727974869176,6.66927856790164));
#59535=CARTESIAN_POINT('Ctrl Pts',(15.9323474070797,25.8953371048986,7.03665039403292));
#59536=CARTESIAN_POINT('Ctrl Pts',(15.166313899323,26.9342469486805,6.4997966771251));
#59537=CARTESIAN_POINT('Ctrl Pts',(15.217408331198,26.0000381535133,6.38029442707274));
#59538=CARTESIAN_POINT('Ctrl Pts',(16.0854844386362,25.9452057906459,6.74476979038736));
#59539=CARTESIAN_POINT('Ctrl Pts',(15.2133526217003,26.9507812969501,6.38893411293837));
#59540=CARTESIAN_POINT('Ctrl Pts',(15.2574505187818,26.0062612054673,6.28360198582695));
#59541=CARTESIAN_POINT('Ctrl Pts',(16.1353739927578,25.9589844139741,6.64678520082825));
#59542=CARTESIAN_POINT('Ctrl Pts',(15.3052181971078,26.9769019217655,6.16562024702973));
#59543=CARTESIAN_POINT('Ctrl Pts',(15.3354770678807,26.0130878248151,6.09018543098795));
#59544=CARTESIAN_POINT('Ctrl Pts',(16.2328071787053,25.9807516016223,6.44941183449709));
#59545=CARTESIAN_POINT('Ctrl Pts',(15.3500450744532,26.9864883979585,6.05316897490136));
#59546=CARTESIAN_POINT('Ctrl Pts',(15.3734229734647,26.0136448619288,5.99351603678512));
#59547=CARTESIAN_POINT('Ctrl Pts',(16.2803508365928,25.9887403314043,6.35002308388268));
#59548=CARTESIAN_POINT('Ctrl Pts',(15.4374530818873,26.9985121419444,5.8266440401815));
#59549=CARTESIAN_POINT('Ctrl Pts',(15.4473305488898,26.0091461456237,5.80010605796439));
#59550=CARTESIAN_POINT('Ctrl Pts',(16.3730562989198,25.9987601185148,6.14981165167035));
#59551=CARTESIAN_POINT('Ctrl Pts',(15.4800342357322,27.0009497744696,5.71257042320435));
#59552=CARTESIAN_POINT('Ctrl Pts',(15.4832543677699,26.0040503216918,5.70342562420715));
#59553=CARTESIAN_POINT('Ctrl Pts',(16.4182181288652,26.0007914784145,6.04898901042871));
#59554=CARTESIAN_POINT('Ctrl Pts',(15.5629140223877,26.9983869468892,5.48275732741083));
#59555=CARTESIAN_POINT('Ctrl Pts',(15.553198440089,25.9881837534892,5.50991450819736));
#59556=CARTESIAN_POINT('Ctrl Pts',(16.5061209327771,25.9986557893846,5.84587137521601));
#59557=CARTESIAN_POINT('Ctrl Pts',(15.6032126798844,26.993387062768,5.36701791538311));
#59558=CARTESIAN_POINT('Ctrl Pts',(15.5871816734266,25.9773800666379,5.41314943781346));
#59559=CARTESIAN_POINT('Ctrl Pts',(16.5488619332758,25.994489218574,5.7435764404109));
#59560=CARTESIAN_POINT('Ctrl Pts',(15.6521341808709,26.9822443529922,5.22126814446177));
#59561=CARTESIAN_POINT('Ctrl Pts',(15.6284283573509,25.9602766635703,5.29230273030841));
#59562=CARTESIAN_POINT('Ctrl Pts',(16.6007483736347,25.9852036275934,5.61475719837616));
#59563=CARTESIAN_POINT('Ctrl Pts',(15.6618458801285,26.9797708939527,5.19206438394472));
#59564=CARTESIAN_POINT('Ctrl Pts',(15.6366386050155,25.9566647485312,5.26807127988625));
#59565=CARTESIAN_POINT('Ctrl Pts',(16.6110486607591,25.9831424115216,5.58894579390439));
#59566=CARTESIAN_POINT('Ctrl Pts',(15.6811234037693,26.974326874309,5.13354825979902));
#59567=CARTESIAN_POINT('Ctrl Pts',(15.6529451403897,25.949071911402,5.2195917195971));
#59568=CARTESIAN_POINT('Ctrl Pts',(16.6314945191325,25.9786057286966,5.53722699728326));
#59569=CARTESIAN_POINT('Ctrl Pts',(15.6906700852009,26.9713614250745,5.10429370826743));
#59570=CARTESIAN_POINT('Ctrl Pts',(15.6610246184452,25.9450979582591,5.19539286772508));
#59571=CARTESIAN_POINT('Ctrl Pts',(16.6416197872961,25.976134520913,5.51137070173943));
#59572=CARTESIAN_POINT('Ctrl Pts',(15.7189906916946,26.9617499071457,5.01668212725527));
#59573=CARTESIAN_POINT('Ctrl Pts',(15.6850272934586,25.9326582303476,5.12297462527296));
#59574=CARTESIAN_POINT('Ctrl Pts',(16.6716567942978,25.9681249225861,5.43393622360837));
#59575=CARTESIAN_POINT('Ctrl Pts',(15.7374648005442,26.9543833549931,4.95841772357253));
#59576=CARTESIAN_POINT('Ctrl Pts',(15.700692464456,25.9236837080238,5.07499871525326));
#59577=CARTESIAN_POINT('Ctrl Pts',(16.6912505459564,25.9619861291773,5.38243990717622));
#59578=CARTESIAN_POINT('Ctrl Pts',(15.7916941691089,26.9294183822048,4.78405831366508));
#59579=CARTESIAN_POINT('Ctrl Pts',(15.7468332080221,25.8946946466028,4.93160995684196));
#59580=CARTESIAN_POINT('Ctrl Pts',(16.748766543145,25.941181985138,5.22833436818176));
#59581=CARTESIAN_POINT('Ctrl Pts',(15.826256817311,26.9089571134584,4.66839662254084));
#59582=CARTESIAN_POINT('Ctrl Pts',(15.7763008752334,25.8726888517142,4.83719393920763));
#59583=CARTESIAN_POINT('Ctrl Pts',(16.785423884099,25.9241309356715,5.12610816476558));
#59584=CARTESIAN_POINT('Ctrl Pts',(15.8592935131526,26.8846780167695,4.55332947014332));
#59585=CARTESIAN_POINT('Ctrl Pts',(15.8045942913409,25.8480831184251,4.74384742394865));
#59586=CARTESIAN_POINT('Ctrl Pts',(16.82046281698,25.9038983473079,5.02440735997516));
#59587=CARTESIAN_POINT('Ctrl Pts',(12.2613198608839,20.1060920634664,11.0892508104087));
#59588=CARTESIAN_POINT('Ctrl Pts',(12.2877096573058,20.1180918018476,11.0727355939116));
#59589=CARTESIAN_POINT('Ctrl Pts',(12.3147120693345,20.1300903154246,11.0577588203659));
#59590=CARTESIAN_POINT('Ctrl Pts',(12.3422975139329,20.1420817712088,11.0442572149087));
#59591=CARTESIAN_POINT('Ctrl Pts',(12.3559433417106,20.1480136437168,11.0375783092223));
#59592=CARTESIAN_POINT('Ctrl Pts',(12.3697324633206,20.1539441026838,11.0312608526765));
#59593=CARTESIAN_POINT('Ctrl Pts',(12.3836643352525,20.1598738261723,11.0253004693755));
#59594=CARTESIAN_POINT('Ctrl Pts',(12.4130618840363,20.1723860956205,11.0127235048641));
#59595=CARTESIAN_POINT('Ctrl Pts',(12.44309018573,20.1848921965551,11.0017350664173));
#59596=CARTESIAN_POINT('Ctrl Pts',(12.4737513223635,20.1973907787835,10.9923335427643));
#59597=CARTESIAN_POINT('Ctrl Pts',(12.4869951325672,20.2027894322264,10.9882726367263));
#59598=CARTESIAN_POINT('Ctrl Pts',(12.5003572194867,20.2081867124763,10.9845084380645));
#59599=CARTESIAN_POINT('Ctrl Pts',(12.5138382575052,20.2135823421314,10.9810437928846));
#59600=CARTESIAN_POINT('Ctrl Pts',(12.5250111044503,20.2180541449871,10.9781723559625));
#59601=CARTESIAN_POINT('Ctrl Pts',(12.5362658706435,20.2225248735315,10.9755066482006));
#59602=CARTESIAN_POINT('Ctrl Pts',(12.5476035673882,20.2269944600046,10.9730491517934));
#59603=CARTESIAN_POINT('Ctrl Pts',(12.5589412641329,20.2314640464776,10.9705916553862));
#59604=CARTESIAN_POINT('Ctrl Pts',(12.5703725446618,20.2359365220228,10.9683411866695));
#59605=CARTESIAN_POINT('Ctrl Pts',(12.5818127411584,20.2403787346282,10.9663142420145));
#59606=CARTESIAN_POINT('Ctrl Pts',(12.6046931341517,20.2492631598391,10.9622603527046));
#59607=CARTESIAN_POINT('Ctrl Pts',(12.6276769122765,20.2580536197943,10.9590831995557));
#59608=CARTESIAN_POINT('Ctrl Pts',(12.6507625114774,20.2667513813436,10.9567688098102));
#59609=CARTESIAN_POINT('Ctrl Pts',(12.6738481106782,20.275449142893,10.9544544200647));
#59610=CARTESIAN_POINT('Ctrl Pts',(12.6970355355578,20.2840542046749,10.9530028263328));
#59611=CARTESIAN_POINT('Ctrl Pts',(12.7203247848531,20.2925665415703,10.952413903835));
#59612=CARTESIAN_POINT('Ctrl Pts',(12.7319694095007,20.296822710018,10.9521194425861));
#59613=CARTESIAN_POINT('Ctrl Pts',(12.7436395141875,20.3010556774401,10.9520408617454));
#59614=CARTESIAN_POINT('Ctrl Pts',(12.7553352452135,20.3052653212751,10.9521794392714));
#59615=CARTESIAN_POINT('Ctrl Pts',(12.7611831107265,20.3073701431925,10.9522487280344));
#59616=CARTESIAN_POINT('Ctrl Pts',(12.7670373831595,20.3094691325677,10.9523723200043));
#59617=CARTESIAN_POINT('Ctrl Pts',(12.7728980912063,20.311562268036,10.9525504583199));
#59618=CARTESIAN_POINT('Ctrl Pts',(12.774363268218,20.3120855519031,10.9525949928988));
#59619=CARTESIAN_POINT('Ctrl Pts',(12.7758288474657,20.3126084698698,10.952642936901));
#59620=CARTESIAN_POINT('Ctrl Pts',(12.7772948299171,20.3131310202127,10.9526942944998));
#59621=CARTESIAN_POINT('Ctrl Pts',(12.7780278211428,20.3133922953841,10.9527199732992));
#59622=CARTESIAN_POINT('Ctrl Pts',(12.7787609131694,20.3136534786491,10.952746505501));
#59623=CARTESIAN_POINT('Ctrl Pts',(12.7794941056814,20.3139145709935,10.9527738918099));
#59624=CARTESIAN_POINT('Ctrl Pts',(12.7802272981934,20.3141756633379,10.9528012781189));
#59625=CARTESIAN_POINT('Ctrl Pts',(12.7809702417849,20.3144401343266,10.9528299067247));
#59626=CARTESIAN_POINT('Ctrl Pts',(12.7816933178538,20.3146973332162,10.9528585865539));
#59627=CARTESIAN_POINT('Ctrl Pts',(12.784585622129,20.3157261287749,10.9529733058707));
#59628=CARTESIAN_POINT('Ctrl Pts',(12.7874779796508,20.3167531168603,10.9531012855059));
#59629=CARTESIAN_POINT('Ctrl Pts',(12.790367822021,20.3177766834169,10.9532422736611));
#59630=CARTESIAN_POINT('Ctrl Pts',(15.8637983830994,26.6272203519198,4.6763017624696));
#59631=CARTESIAN_POINT('Ctrl Pts',(15.8349038320035,26.6601158718637,4.75787351480363));
#59632=CARTESIAN_POINT('Ctrl Pts',(15.8052672194834,26.6925210251888,4.83935638988722));
#59633=CARTESIAN_POINT('Ctrl Pts',(15.7751639364047,26.7244625096831,4.9208424051611));
#59634=CARTESIAN_POINT('Ctrl Pts',(15.7735322678848,26.7261938130293,4.92525913823247));
#59635=CARTESIAN_POINT('Ctrl Pts',(15.7718992639185,26.7279237294146,4.92967580195018));
#59636=CARTESIAN_POINT('Ctrl Pts',(15.7702649656506,26.7296522715952,4.93409242389849));
#59637=CARTESIAN_POINT('Ctrl Pts',(15.7502539098552,26.7508172906735,4.98817145584254));
#59638=CARTESIAN_POINT('Ctrl Pts',(15.7300480550329,26.7717766681125,5.04224424269192));
#59639=CARTESIAN_POINT('Ctrl Pts',(15.709725991688,26.7925423987736,5.09636326895675));
#59640=CARTESIAN_POINT('Ctrl Pts',(15.7010873400666,26.8013696477494,5.11936858126495));
#59641=CARTESIAN_POINT('Ctrl Pts',(15.6924243940276,26.8101626876449,5.14239245762853));
#59642=CARTESIAN_POINT('Ctrl Pts',(15.6837524821722,26.8189188830466,5.1654118929897));
#59643=CARTESIAN_POINT('Ctrl Pts',(15.68209242477,26.8205950747831,5.16981848575752));
#59644=CARTESIAN_POINT('Ctrl Pts',(15.6804314503341,26.8222700879288,5.17422670287004));
#59645=CARTESIAN_POINT('Ctrl Pts',(15.6787696557313,26.8239439009101,5.17863639594407));
#59646=CARTESIAN_POINT('Ctrl Pts',(15.6683658191531,26.8344229797867,5.20624373443547));
#59647=CARTESIAN_POINT('Ctrl Pts',(15.6579486373731,26.844849877472,5.23385227711352));
#59648=CARTESIAN_POINT('Ctrl Pts',(15.6475281571989,26.8552273352648,5.26147252908649));
#59649=CARTESIAN_POINT('Ctrl Pts',(15.6287933916902,26.8738847517249,5.3111304081236));
#59650=CARTESIAN_POINT('Ctrl Pts',(15.6100478265525,26.8923841385894,5.36082626140884));
#59651=CARTESIAN_POINT('Ctrl Pts',(15.5913526570138,26.9107267231326,5.4106217245225));
#59652=CARTESIAN_POINT('Ctrl Pts',(15.5759753763904,26.925813993098,5.45157983450311));
#59653=CARTESIAN_POINT('Ctrl Pts',(15.5606365219061,26.940795775563,5.49259231312282));
#59654=CARTESIAN_POINT('Ctrl Pts',(15.5453788495309,26.9556741079129,5.53367425118021));
#59655=CARTESIAN_POINT('Ctrl Pts',(15.5374315984396,26.9634237724814,5.55507256601038));
#59656=CARTESIAN_POINT('Ctrl Pts',(15.5295055620971,26.9711442394673,5.57649219744023));
#59657=CARTESIAN_POINT('Ctrl Pts',(15.5216083672387,26.9788375422302,5.59793131348772));
#59658=CARTESIAN_POINT('Ctrl Pts',(15.5143439910773,26.9859143645949,5.61765246844561));
#59659=CARTESIAN_POINT('Ctrl Pts',(15.5071040241837,26.9929681813793,5.63739011108275));
#59660=CARTESIAN_POINT('Ctrl Pts',(15.4998946833985,27.,5.65714286308472));
#59661=CARTESIAN_POINT('Origin',(-11.,51.,-13.6106575888162));
#59662=CARTESIAN_POINT('Origin',(-11.,51.,-13.6106575888162));
#59663=CARTESIAN_POINT('Origin',(-11.,51.,-13.6106575888162));
#59664=CARTESIAN_POINT('Origin',(-11.,52.,-13.6106575888162));
#59665=CARTESIAN_POINT('Ctrl Pts',(-10.3714285714286,38.7323075626015,-12.8329057265981));
#59666=CARTESIAN_POINT('Ctrl Pts',(-10.3703047272601,38.7337956967718,-12.8338140064349));
#59667=CARTESIAN_POINT('Ctrl Pts',(-10.3691828501228,38.7352838331315,-12.8347247235238));
#59668=CARTESIAN_POINT('Ctrl Pts',(-10.2297794583371,38.9205231532402,-12.9483917264144));
#59669=CARTESIAN_POINT('Ctrl Pts',(-10.1237094532379,39.1011906672438,-13.0964292382757));
#59670=CARTESIAN_POINT('Ctrl Pts',(-10.0208952490217,39.360673140197,-13.3756530051914));
#59671=CARTESIAN_POINT('Ctrl Pts',(-10.,39.4508344663996,-13.4925906505731));
#59672=CARTESIAN_POINT('Ctrl Pts',(-10.,39.5242048993244,-13.6106575888162));
#59673=CARTESIAN_POINT('Origin',(6.61363325216158E-15,38.7323075626015,
8.67361737988404E-16));
#59674=CARTESIAN_POINT('Origin',(-6.5,38.7323075626015,-16.2480768092719));
#59675=CARTESIAN_POINT('Origin',(-6.5,40.2323075626015,-31.8229001029736));
#59676=CARTESIAN_POINT('Ctrl Pts',(-6.,40.2323075626015,-16.7705098312484));
#59677=CARTESIAN_POINT('Ctrl Pts',(-6.,40.2152260685424,-16.7705098300399));
#59678=CARTESIAN_POINT('Ctrl Pts',(-6.00087270480098,40.1983584811302,-16.7697298783156));
#59679=CARTESIAN_POINT('Ctrl Pts',(-6.00256838001511,40.1816934989509,-16.7682104533614));
#59680=CARTESIAN_POINT('Ctrl Pts',(-6.00291333028549,40.178303350849,-16.7679013575838));
#59681=CARTESIAN_POINT('Ctrl Pts',(-6.00329235512771,40.1749215836645,-16.7675616445011));
#59682=CARTESIAN_POINT('Ctrl Pts',(-6.0037052686087,40.1715481408978,-16.7671913871201));
#59683=CARTESIAN_POINT('Ctrl Pts',(-6.005335465801,40.1582296681913,-16.765729597736));
#59684=CARTESIAN_POINT('Ctrl Pts',(-6.00749386985472,40.1450410361966,-16.7637923412657));
#59685=CARTESIAN_POINT('Ctrl Pts',(-6.01016893654584,40.1319804512336,-16.7613838478594));
#59686=CARTESIAN_POINT('Ctrl Pts',(-6.01150217107971,40.1254711470122,-16.7601834715868));
#59687=CARTESIAN_POINT('Ctrl Pts',(-6.01296373632936,40.1189936487289,-16.7588660602385));
#59688=CARTESIAN_POINT('Ctrl Pts',(-6.01455377974561,40.1125480291574,-16.7574302675289));
#59689=CARTESIAN_POINT('Ctrl Pts',(-6.0169439717228,40.1028588168814,-16.7552719489697));
#59690=CARTESIAN_POINT('Ctrl Pts',(-6.01963110947182,40.0932249571053,-16.7528410281537));
#59691=CARTESIAN_POINT('Ctrl Pts',(-6.02257533346268,40.0837623210638,-16.7501687385702));
#59692=CARTESIAN_POINT('Ctrl Pts',(-6.02389791871011,40.0795115769393,-16.7489683099374));
#59693=CARTESIAN_POINT('Ctrl Pts',(-6.02527425556365,40.0752883249674,-16.7477175528816));
#59694=CARTESIAN_POINT('Ctrl Pts',(-6.02670067639266,40.0711003969021,-16.7464194186541));
#59695=CARTESIAN_POINT('Ctrl Pts',(-6.02807072595986,40.0670779731429,-16.745172585882));
#59696=CARTESIAN_POINT('Ctrl Pts',(-6.02948329310936,40.063098660006,-16.7438852854621));
#59697=CARTESIAN_POINT('Ctrl Pts',(-6.03093707782595,40.0591602985701,-16.7425585794677));
#59698=CARTESIAN_POINT('Ctrl Pts',(-6.03387632863431,40.0511977495752,-16.7398762554468));
#59699=CARTESIAN_POINT('Ctrl Pts',(-6.03698370699615,40.0434031654531,-16.7370331048754));
#59700=CARTESIAN_POINT('Ctrl Pts',(-6.04024790247354,40.0357674679134,-16.7340364148325));
#59701=CARTESIAN_POINT('Ctrl Pts',(-6.0449141209408,40.024852118904,-16.7297525995659));
#59702=CARTESIAN_POINT('Ctrl Pts',(-6.0499000474802,40.0142610236446,-16.7251561505607));
#59703=CARTESIAN_POINT('Ctrl Pts',(-6.05518149077389,40.0039727938111,-16.7202613803198));
#59704=CARTESIAN_POINT('Ctrl Pts',(-6.05744858312296,39.9995565072311,-16.7181602697812));
#59705=CARTESIAN_POINT('Ctrl Pts',(-6.0597701483618,39.9951960798736,-16.7160040490599));
#59706=CARTESIAN_POINT('Ctrl Pts',(-6.06214427791603,39.9908901509711,-16.7137939059645));
#59707=CARTESIAN_POINT('Ctrl Pts',(-6.06864070612356,39.9791076608659,-16.7077462006395));
#59708=CARTESIAN_POINT('Ctrl Pts',(-6.07553063592893,39.9677331969345,-16.7012947219666));
#59709=CARTESIAN_POINT('Ctrl Pts',(-6.08278766669716,39.9567462769058,-16.6944505893577));
#59710=CARTESIAN_POINT('Ctrl Pts',(-6.08461402447538,39.9539812277425,-16.6927281445694));
#59711=CARTESIAN_POINT('Ctrl Pts',(-6.08646377242624,39.9512405363443,-16.6909806468571));
#59712=CARTESIAN_POINT('Ctrl Pts',(-6.08833629232153,39.9485242090016,-16.6892084804434));
#59713=CARTESIAN_POINT('Ctrl Pts',(-6.09070655159091,39.9450858476368,-16.686965249875));
#59714=CARTESIAN_POINT('Ctrl Pts',(-6.0931134023071,39.9416865866905,-16.6846823645151));
#59715=CARTESIAN_POINT('Ctrl Pts',(-6.09555574756902,39.9383265314523,-16.6823604186901));
#59716=CARTESIAN_POINT('Ctrl Pts',(-6.09801610063588,39.9349417019858,-16.6800213527845));
#59717=CARTESIAN_POINT('Ctrl Pts',(-6.10051625664023,39.9315916991154,-16.6776390419408));
#59718=CARTESIAN_POINT('Ctrl Pts',(-6.10304466826099,39.928290351569,-16.6752240173384));
#59719=CARTESIAN_POINT('Ctrl Pts',(-6.10678165416141,39.92341096835,-16.6716546171608));
#59720=CARTESIAN_POINT('Ctrl Pts',(-6.11056908515597,39.9186518404417,-16.668024432723));
#59721=CARTESIAN_POINT('Ctrl Pts',(-6.11440532151745,39.9140046239577,-16.6643343458043));
#59722=CARTESIAN_POINT('Ctrl Pts',(-6.12544919130915,39.9006260807951,-16.6537112153166));
#59723=CARTESIAN_POINT('Ctrl Pts',(-6.13689162615053,39.8881758726312,-16.6425950921152));
#59724=CARTESIAN_POINT('Ctrl Pts',(-6.14866874643051,39.8765458402052,-16.6310255748251));
#59725=CARTESIAN_POINT('Ctrl Pts',(-6.16044586671049,39.8649158077793,-16.619456057535));
#59726=CARTESIAN_POINT('Ctrl Pts',(-6.17255719994684,39.8541058231107,-16.6074330450772));
#59727=CARTESIAN_POINT('Ctrl Pts',(-6.18495795774414,39.8440440390462,-16.5949803772694));
#59728=CARTESIAN_POINT('Ctrl Pts',(-6.19115833664278,39.839013147014,-16.5887540433655));
#59729=CARTESIAN_POINT('Ctrl Pts',(-6.19743103892612,39.8341693874632,-16.5824202196346));
#59730=CARTESIAN_POINT('Ctrl Pts',(-6.2037717941715,39.8295062938081,-16.5759807931943));
#59731=CARTESIAN_POINT('Ctrl Pts',(-6.20694217179419,39.8271747469806,-16.5727610799741));
#59732=CARTESIAN_POINT('Ctrl Pts',(-6.21012955915248,39.824888363891,-16.5695149694884));
#59733=CARTESIAN_POINT('Ctrl Pts',(-6.21333344646887,39.8226463997159,-16.5662426651369));
#59734=CARTESIAN_POINT('Ctrl Pts',(-6.21653733378526,39.8204044355407,-16.5629703607854));
#59735=CARTESIAN_POINT('Ctrl Pts',(-6.21975872711503,39.8182063277282,-16.5596708190893));
#59736=CARTESIAN_POINT('Ctrl Pts',(-6.22298327133341,39.816060360099,-16.5563585361363));
#59737=CARTESIAN_POINT('Ctrl Pts',(-6.23588144820696,39.8074764895821,-16.5431094043243));
#59738=CARTESIAN_POINT('Ctrl Pts',(-6.24887960590686,39.7996874748855,-16.5296056075263));
#59739=CARTESIAN_POINT('Ctrl Pts',(-6.26195557855337,39.7926087889069,-16.515863299996));
#59740=CARTESIAN_POINT('Ctrl Pts',(-6.26491334532597,39.7910076000127,-16.5127548092022));
#59741=CARTESIAN_POINT('Ctrl Pts',(-6.2678751485978,39.7894428128996,-16.5096340420518));
#59742=CARTESIAN_POINT('Ctrl Pts',(-6.27084071420014,39.7879135687944,-16.506501210133));
#59743=CARTESIAN_POINT('Ctrl Pts',(-6.28528892650271,39.780463103535,-16.4912380776512));
#59744=CARTESIAN_POINT('Ctrl Pts',(-6.2998262820572,39.7738559475515,-16.4756886097743));
#59745=CARTESIAN_POINT('Ctrl Pts',(-6.31443187001688,39.768018354096,-16.4598673206089));
#59746=CARTESIAN_POINT('Ctrl Pts',(-6.32333492367592,39.7644599620671,-16.4502232181747));
#59747=CARTESIAN_POINT('Ctrl Pts',(-6.33226341030448,39.7611876883161,-16.440478106521));
#59748=CARTESIAN_POINT('Ctrl Pts',(-6.34121473427545,39.7581899257814,-16.4306331935693));
#59749=CARTESIAN_POINT('Ctrl Pts',(-6.34735648803554,39.7561330770538,-16.4238783234143));
#59750=CARTESIAN_POINT('Ctrl Pts',(-6.35350901798207,39.7542054768412,-16.4170764545765));
#59751=CARTESIAN_POINT('Ctrl Pts',(-6.3596706706762,39.7524037396,-16.4102288970642));
#59752=CARTESIAN_POINT('Ctrl Pts',(-6.3635201769234,39.7512781002448,-16.4059508702538));
#59753=CARTESIAN_POINT('Ctrl Pts',(-6.36737627692165,39.7502009295338,-16.4016516058271));
#59754=CARTESIAN_POINT('Ctrl Pts',(-6.37122409342676,39.7491753178836,-16.3973476877078));
#59755=CARTESIAN_POINT('Ctrl Pts',(-6.37457974424939,39.7482808899468,-16.3935942742178));
#59756=CARTESIAN_POINT('Ctrl Pts',(-6.3779317495519,39.7474248597862,-16.389834380521));
#59757=CARTESIAN_POINT('Ctrl Pts',(-6.38128159473997,39.7466060693528,-16.3860663752365));
#59758=CARTESIAN_POINT('Ctrl Pts',(-6.38955863476667,39.7445829426677,-16.3767561149677));
#59759=CARTESIAN_POINT('Ctrl Pts',(-6.39781703593733,39.7427883967616,-16.3674024363885));
#59760=CARTESIAN_POINT('Ctrl Pts',(-6.40605643102158,39.7412122502155,-16.3580063013025));
#59761=CARTESIAN_POINT('Ctrl Pts',(-6.41109566421616,39.7402482753225,-16.3522596032327));
#59762=CARTESIAN_POINT('Ctrl Pts',(-6.4161277746267,39.7393658825604,-16.3464970397648));
#59763=CARTESIAN_POINT('Ctrl Pts',(-6.42115275150614,39.7385633481733,-16.3407187505363));
#59764=CARTESIAN_POINT('Ctrl Pts',(-6.43174690801946,39.7368713652831,-16.3285363859334));
#59765=CARTESIAN_POINT('Ctrl Pts',(-6.4423094285119,39.7355342933199,-16.3162840767447));
#59766=CARTESIAN_POINT('Ctrl Pts',(-6.45283975421962,39.7345366200808,-16.3039636584199));
#59767=CARTESIAN_POINT('Ctrl Pts',(-6.4686319955505,39.7330404178742,-16.2854868301735));
#59768=CARTESIAN_POINT('Ctrl Pts',(-6.48435190789287,39.7323075626015,-16.266856742178));
#59769=CARTESIAN_POINT('Ctrl Pts',(-6.5,39.7323075626015,-16.2480768092719));
#59770=CARTESIAN_POINT('Origin',(-5.,52.,-16.7705098312484));
#59771=CARTESIAN_POINT('Origin',(-5.,40.2323075626015,-16.7705098312484));
#59772=CARTESIAN_POINT('Ctrl Pts',(-14.1696709084508,34.2228423347593,-8.45401835497186));
#59773=CARTESIAN_POINT('Ctrl Pts',(-14.4598881528388,34.2800112558736,-7.96758898230353));
#59774=CARTESIAN_POINT('Ctrl Pts',(-15.0284388422964,34.3091931864527,-7.97011831445158));
#59775=CARTESIAN_POINT('Ctrl Pts',(-14.1687509928547,34.2417094783908,-8.45556021361394));
#59776=CARTESIAN_POINT('Ctrl Pts',(-14.4590195349379,34.2974823791094,-7.96916514970434));
#59777=CARTESIAN_POINT('Ctrl Pts',(-15.027463174257,34.3259639809838,-7.97157191635228));
#59778=CARTESIAN_POINT('Ctrl Pts',(-14.1678668544491,34.2605265108349,-8.45704153677041));
#59779=CARTESIAN_POINT('Ctrl Pts',(-14.4581845937863,34.3149090256939,-7.97067959720386));
#59780=CARTESIAN_POINT('Ctrl Pts',(-15.0265254516828,34.3426902318517,-7.97296845218914));
#59781=CARTESIAN_POINT('Ctrl Pts',(-14.1661635328208,34.2981938523499,-8.45989441550156));
#59782=CARTESIAN_POINT('Ctrl Pts',(-14.4565759909218,34.3497943960948,-7.97359633424001));
#59783=CARTESIAN_POINT('Ctrl Pts',(-15.024718898452,34.3761723132014,-7.97565803480127));
#59784=CARTESIAN_POINT('Ctrl Pts',(-14.1653454356421,34.3170219168472,-8.46126415076535));
#59785=CARTESIAN_POINT('Ctrl Pts',(-14.4558033400937,34.3672326811367,-7.97499678944735));
#59786=CARTESIAN_POINT('Ctrl Pts',(-15.0238512196152,34.3929083705295,-7.97694936773952));
#59787=CARTESIAN_POINT('Ctrl Pts',(-14.1629917065432,34.373489337447,-8.46520379440197));
#59788=CARTESIAN_POINT('Ctrl Pts',(-14.4535804037852,34.41953098386,-7.97902465759217));
#59789=CARTESIAN_POINT('Ctrl Pts',(-15.0213548402835,34.4431016332889,-7.98066350984471));
#59790=CARTESIAN_POINT('Ctrl Pts',(-14.1615566384215,34.4111119211253,-8.4676041477937));
#59791=CARTESIAN_POINT('Ctrl Pts',(-14.4522248265318,34.454380888302,-7.98147914140516));
#59792=CARTESIAN_POINT('Ctrl Pts',(-15.0198327983173,34.4765439298872,-7.98292646932796));
#59793=CARTESIAN_POINT('Ctrl Pts',(-14.1576526183944,34.5239129308506,-8.47413110853782));
#59794=CARTESIAN_POINT('Ctrl Pts',(-14.4485372614658,34.5588642949711,-7.98815276719896));
#59795=CARTESIAN_POINT('Ctrl Pts',(-15.0156921710414,34.5768114940933,-7.98907983290995));
#59796=CARTESIAN_POINT('Ctrl Pts',(-14.1555848703909,34.5990246231075,-8.47758373051289));
#59797=CARTESIAN_POINT('Ctrl Pts',(-14.446583355318,34.6284571865908,-7.99168420593832));
#59798=CARTESIAN_POINT('Ctrl Pts',(-15.0134991049499,34.6435774427604,-7.99233483016131));
#59799=CARTESIAN_POINT('Ctrl Pts',(-14.1509771790097,34.8240952679178,-8.4852743386372));
#59800=CARTESIAN_POINT('Ctrl Pts',(-14.4422301623517,34.8369697425827,-7.99954874151129));
#59801=CARTESIAN_POINT('Ctrl Pts',(-15.008612159576,34.8436402381527,-7.99958523498254));
#59802=CARTESIAN_POINT('Ctrl Pts',(-14.1500330992177,34.9737899010413,-8.48684678418226));
#59803=CARTESIAN_POINT('Ctrl Pts',(-14.4413373565372,34.9757252603891,-8.00115815623579));
#59804=CARTESIAN_POINT('Ctrl Pts',(-15.0076108628144,34.9767021342601,-8.00106767539272));
#59805=CARTESIAN_POINT('Ctrl Pts',(-14.1534989333457,35.4218322689878,-8.48106645017854));
#59806=CARTESIAN_POINT('Ctrl Pts',(-14.4446127086534,35.3909181528281,-7.99524560707017));
#59807=CARTESIAN_POINT('Ctrl Pts',(-15.0112867474724,35.3749620168757,-7.99561820204977));
#59808=CARTESIAN_POINT('Ctrl Pts',(-14.1642118082204,35.7191401530233,-8.46324178895702));
#59809=CARTESIAN_POINT('Ctrl Pts',(-14.454761563286,35.6666794668494,-7.97697017454646));
#59810=CARTESIAN_POINT('Ctrl Pts',(-15.0226488876287,35.6392356915726,-7.97881380780291));
#59811=CARTESIAN_POINT('Ctrl Pts',(-14.2018700963651,36.3110245203784,-8.3998954453284));
#59812=CARTESIAN_POINT('Ctrl Pts',(-14.4903036805241,36.2145680745722,-7.91223236340415));
#59813=CARTESIAN_POINT('Ctrl Pts',(-15.0625894960227,36.1653551292289,-7.91909334909917));
#59814=CARTESIAN_POINT('Ctrl Pts',(-14.2288151924285,36.6056011119585,-8.35437505244428));
#59815=CARTESIAN_POINT('Ctrl Pts',(-14.5157733460828,36.4872920363756,-7.86562765440656));
#59816=CARTESIAN_POINT('Ctrl Pts',(-15.0911676285592,36.4272009883655,-7.87617850054425));
#59817=CARTESIAN_POINT('Ctrl Pts',(-14.2678515285549,36.9354562627635,-8.28724846986359));
#59818=CARTESIAN_POINT('Ctrl Pts',(-14.5524221273012,36.7911880341194,-7.7973135407053));
#59819=CARTESIAN_POINT('Ctrl Pts',(-15.1325698029845,36.7204055669061,-7.81289418035236));
#59820=CARTESIAN_POINT('Ctrl Pts',(-14.272310834891,36.9720923458365,-8.27956682548256));
#59821=CARTESIAN_POINT('Ctrl Pts',(-14.5566164314028,36.8250040101967,-7.78948085637131));
#59822=CARTESIAN_POINT('Ctrl Pts',(-15.1372993703662,36.7529709740877,-7.80565222610578));
#59823=CARTESIAN_POINT('Ctrl Pts',(-14.2814663750741,37.0452925529125,-8.26376437000761));
#59824=CARTESIAN_POINT('Ctrl Pts',(-14.5652251137911,36.8925526698609,-7.77337133120969));
#59825=CARTESIAN_POINT('Ctrl Pts',(-15.1470097917179,36.8180378248002,-7.79075428816105));
#59826=CARTESIAN_POINT('Ctrl Pts',(-14.2861536017617,37.081785083136,-8.25565910563603));
#59827=CARTESIAN_POINT('Ctrl Pts',(-14.5696312954759,36.9262202981498,-7.76510980926654));
#59828=CARTESIAN_POINT('Ctrl Pts',(-15.1519810928061,36.850475629465,-7.78311296160134));
#59829=CARTESIAN_POINT('Ctrl Pts',(-14.3005366026303,37.1909436147287,-8.23073635121615));
#59830=CARTESIAN_POINT('Ctrl Pts',(-14.5831518360579,37.0269359064794,-7.7397041366779));
#59831=CARTESIAN_POINT('Ctrl Pts',(-15.1672357906114,36.9475054352928,-7.7596167619714));
#59832=CARTESIAN_POINT('Ctrl Pts',(-14.3105536680637,37.263290615546,-8.21331202705747));
#59833=CARTESIAN_POINT('Ctrl Pts',(-14.5925608990619,37.0936355928615,-7.7219524972774));
#59834=CARTESIAN_POINT('Ctrl Pts',(-15.1778599510383,37.0118138805059,-7.74318978992613));
#59835=CARTESIAN_POINT('Ctrl Pts',(-14.3418348010998,37.4790826477386,-8.15864801908498));
#59836=CARTESIAN_POINT('Ctrl Pts',(-14.6219410641221,37.2926085843646,-7.66625367882849));
#59837=CARTESIAN_POINT('Ctrl Pts',(-15.211036910134,37.2036290201708,-7.69165469791198));
#59838=CARTESIAN_POINT('Ctrl Pts',(-14.3643283878283,37.6212795682079,-8.11901917638115));
#59839=CARTESIAN_POINT('Ctrl Pts',(-14.6430362895773,37.4235089284438,-7.62591654935295));
#59840=CARTESIAN_POINT('Ctrl Pts',(-15.2348937448071,37.3300262828855,-7.65429417319524));
#59841=CARTESIAN_POINT('Ctrl Pts',(-14.4363019502445,38.0430610597211,-7.9907944336361));
#59842=CARTESIAN_POINT('Ctrl Pts',(-14.7105067497658,37.8118623201918,-7.49538846499181));
#59843=CARTESIAN_POINT('Ctrl Pts',(-15.3112293408869,37.7049431641283,-7.53340889331172));
#59844=CARTESIAN_POINT('Ctrl Pts',(-14.49026980554,38.3178484315225,-7.8928871878268));
#59845=CARTESIAN_POINT('Ctrl Pts',(-14.7609541970719,38.0639420611781,-7.39588717756517));
#59846=CARTESIAN_POINT('Ctrl Pts',(-15.3684679759171,37.9491986058153,-7.44110576650622));
#59847=CARTESIAN_POINT('Ctrl Pts',(-14.6080482783172,38.8552917835711,-7.67271221247472));
#59848=CARTESIAN_POINT('Ctrl Pts',(-14.8703740139742,38.5549584396854,-7.17322618837634));
#59849=CARTESIAN_POINT('Ctrl Pts',(-15.4933845372648,38.4269260298234,-7.2335333987612));
#59850=CARTESIAN_POINT('Ctrl Pts',(-14.6718611162741,39.1179471327802,-7.55044413842592));
#59851=CARTESIAN_POINT('Ctrl Pts',(-14.9295100780991,38.794189655202,-7.04967693049274));
#59852=CARTESIAN_POINT('Ctrl Pts',(-15.5610648206959,38.6603974512983,-7.11826383427611));
#59853=CARTESIAN_POINT('Ctrl Pts',(-14.7480666188548,39.4067715675604,-7.3989787087425));
#59854=CARTESIAN_POINT('Ctrl Pts',(-14.999316825149,39.0547855952716,-6.89817098281311));
#59855=CARTESIAN_POINT('Ctrl Pts',(-15.6418888381287,38.9171302822837,-6.97546814291349));
#59856=CARTESIAN_POINT('Ctrl Pts',(-14.7565941785648,39.4387656880567,-7.38195749962283));
#59857=CARTESIAN_POINT('Ctrl Pts',(-15.0071581686653,39.0837656036217,-6.88107637534832));
#59858=CARTESIAN_POINT('Ctrl Pts',(-15.6509332197322,38.9455695005142,-6.95942121181813));
#59859=CARTESIAN_POINT('Ctrl Pts',(-14.7737256022962,39.502412269052,-7.34761186407861));
#59860=CARTESIAN_POINT('Ctrl Pts',(-15.0228997481459,39.1413825527381,-6.84659981861948));
#59861=CARTESIAN_POINT('Ctrl Pts',(-15.6691029114839,39.002144239138,-6.92704148796774));
#59862=CARTESIAN_POINT('Ctrl Pts',(-14.7823346424693,39.5340844533758,-7.33027717344031));
#59863=CARTESIAN_POINT('Ctrl Pts',(-15.0308049908594,39.1700375342947,-6.82920681792526));
#59864=CARTESIAN_POINT('Ctrl Pts',(-15.6782337117527,39.0302972919077,-6.91069901878126));
#59865=CARTESIAN_POINT('Ctrl Pts',(-14.808284656594,39.6286524867301,-7.27779013265149));
#59866=CARTESIAN_POINT('Ctrl Pts',(-15.0546319241823,39.2556023565078,-6.77653515305077));
#59867=CARTESIAN_POINT('Ctrl Pts',(-15.7057564538778,39.1143577659461,-6.8612162865755));
#59868=CARTESIAN_POINT('Ctrl Pts',(-14.8257484822497,39.6910999140348,-7.24215491242092));
#59869=CARTESIAN_POINT('Ctrl Pts',(-15.0706345822693,39.31199951062,-6.74082930478049));
#59870=CARTESIAN_POINT('Ctrl Pts',(-15.7242786933826,39.1698665902847,-6.8276207929431));
#59871=CARTESIAN_POINT('Ctrl Pts',(-14.8785762907581,39.876683136037,-7.1333351875412));
#59872=CARTESIAN_POINT('Ctrl Pts',(-15.1190327204018,39.4796219387076,-6.63176677641015));
#59873=CARTESIAN_POINT('Ctrl Pts',(-15.7803081869927,39.3348294541919,-6.72502980625943));
#59874=CARTESIAN_POINT('Ctrl Pts',(-14.9143760584171,39.9980613049761,-7.05823809590922));
#59875=CARTESIAN_POINT('Ctrl Pts',(-15.1516954791241,39.5888243403568,-6.5567294842393));
#59876=CARTESIAN_POINT('Ctrl Pts',(-15.8182776378986,39.4427211600206,-6.65423120166715));
#59877=CARTESIAN_POINT('Ctrl Pts',(-15.0231004266237,40.3553871225062,-6.82537958602282));
#59878=CARTESIAN_POINT('Ctrl Pts',(-15.2508296348633,39.9103610239103,-6.3239951350709));
#59879=CARTESIAN_POINT('Ctrl Pts',(-15.9335913612037,39.7603441088107,-6.43470129294701));
#59880=CARTESIAN_POINT('Ctrl Pts',(-15.0973449297501,40.5845463158894,-6.66007288714214));
#59881=CARTESIAN_POINT('Ctrl Pts',(-15.31792988494,40.114768031037,-6.15976330372408));
#59882=CARTESIAN_POINT('Ctrl Pts',(-16.0123355319573,39.9640411696614,-6.2788565940716));
#59883=CARTESIAN_POINT('Ctrl Pts',(-15.2472968949109,41.0254173108877,-6.30922595793956));
#59884=CARTESIAN_POINT('Ctrl Pts',(-15.4523126364001,40.5055857309467,-5.81354666702777));
#59885=CARTESIAN_POINT('Ctrl Pts',(-16.1713754941982,40.3559264985848,-5.94809181206602));
#59886=CARTESIAN_POINT('Ctrl Pts',(-15.3230087426575,41.2371284648137,-6.12368686448347));
#59887=CARTESIAN_POINT('Ctrl Pts',(-15.5196455447178,40.6918988399555,-5.63122192702778));
#59888=CARTESIAN_POINT('Ctrl Pts',(-16.2516759396333,40.5441141908017,-5.77317280154761));
#59889=CARTESIAN_POINT('Ctrl Pts',(-15.4173521697931,41.4908768942127,-5.87860618526534));
#59890=CARTESIAN_POINT('Ctrl Pts',(-15.6023498902727,40.9125245108878,-5.39340306565551));
#59891=CARTESIAN_POINT('Ctrl Pts',(-16.3517371496677,40.7696683504473,-5.54212030933746));
#59892=CARTESIAN_POINT('Ctrl Pts',(-15.4362061333438,41.541080480963,-5.82893036895881));
#59893=CARTESIAN_POINT('Ctrl Pts',(-15.6189216498825,40.9563040712589,-5.34503370394812));
#59894=CARTESIAN_POINT('Ctrl Pts',(-16.3717337779055,40.814293760811,-5.49528788992432));
#59895=CARTESIAN_POINT('Ctrl Pts',(-15.4644422759024,41.6155621820111,-5.75341180123559));
#59896=CARTESIAN_POINT('Ctrl Pts',(-15.6436600403385,41.0210733659742,-5.27169025022555));
#59897=CARTESIAN_POINT('Ctrl Pts',(-16.4016812016563,40.8804997173657,-5.42409193382638));
#59898=CARTESIAN_POINT('Ctrl Pts',(-15.4738394697509,41.6402325166288,-5.72809098740203));
#59899=CARTESIAN_POINT('Ctrl Pts',(-15.6518901269291,41.042522534143,-5.24709833812979));
#59900=CARTESIAN_POINT('Ctrl Pts',(-16.4116479225022,40.9024289036886,-5.40022045953334));
#59901=CARTESIAN_POINT('Ctrl Pts',(-15.4925703942472,41.689181898316,-5.67723496738244));
#59902=CARTESIAN_POINT('Ctrl Pts',(-15.6682749940766,41.0850380021743,-5.1977485436834));
#59903=CARTESIAN_POINT('Ctrl Pts',(-16.4315140544655,40.9459394651512,-5.35227539009512));
#59904=CARTESIAN_POINT('Ctrl Pts',(-15.5019086640392,41.7134729307954,-5.65168764188966));
#59905=CARTESIAN_POINT('Ctrl Pts',(-15.6764336314637,41.1061140969787,-5.17297859437461));
#59906=CARTESIAN_POINT('Ctrl Pts',(-16.4414182800811,40.967531494057,-5.32819036948575));
#59907=CARTESIAN_POINT('Ctrl Pts',(-15.5484555651202,41.8340156143712,-5.52335553940722));
#59908=CARTESIAN_POINT('Ctrl Pts',(-15.7171539857794,41.2108612547213,-5.04834447526745));
#59909=CARTESIAN_POINT('Ctrl Pts',(-16.4907862052723,41.074680546041,-5.20720387542547));
#59910=CARTESIAN_POINT('Ctrl Pts',(-15.5852305114518,41.9275319640208,-5.41878553611691));
#59911=CARTESIAN_POINT('Ctrl Pts',(-15.7490791740827,41.2915492195499,-4.94737813664718));
#59912=CARTESIAN_POINT('Ctrl Pts',(-16.5297899365528,41.1578061902771,-5.10861936072794));
#59913=CARTESIAN_POINT('Ctrl Pts',(-15.6938508583456,42.199498468939,-5.0993756835597));
#59914=CARTESIAN_POINT('Ctrl Pts',(-15.8432282443095,41.526068650345,-4.63908945210971));
#59915=CARTESIAN_POINT('Ctrl Pts',(-16.64499333428,41.3995541945398,-4.80749222676696));
#59916=CARTESIAN_POINT('Ctrl Pts',(-15.7639910093299,42.369390564411,-4.87885064391805));
#59917=CARTESIAN_POINT('Ctrl Pts',(-15.9031097774975,41.6705184443034,-4.42842552480797));
#59918=CARTESIAN_POINT('Ctrl Pts',(-16.7193844041967,41.5505693905269,-4.59958983270443));
#59919=CARTESIAN_POINT('Ctrl Pts',(-15.8980969848804,42.6866289429011,-4.42234195955402));
#59920=CARTESIAN_POINT('Ctrl Pts',(-16.0164770439618,41.938203868012,-3.99591210397994));
#59921=CARTESIAN_POINT('Ctrl Pts',(-16.8616180139052,41.8325590604172,-4.16921127494601));
#59922=CARTESIAN_POINT('Ctrl Pts',(-15.9620670091645,42.8339757168234,-4.18635981457349));
#59923=CARTESIAN_POINT('Ctrl Pts',(-16.069837618137,42.061051465547,-3.77409145591909));
#59924=CARTESIAN_POINT('Ctrl Pts',(-16.9294650101271,41.9635339702937,-3.94673652549938));
#59925=CARTESIAN_POINT('Ctrl Pts',(-16.0521582726785,43.037709823846,-3.82021108244197));
#59926=CARTESIAN_POINT('Ctrl Pts',(-16.1440256404094,42.2291011383052,-3.43385778245536));
#59927=CARTESIAN_POINT('Ctrl Pts',(-17.0250163496069,42.1446309546378,-3.60154580164102));
#59928=CARTESIAN_POINT('Ctrl Pts',(-16.0812108244472,43.102733976819,-3.69612831892062));
#59929=CARTESIAN_POINT('Ctrl Pts',(-16.1678670548505,42.2825951618778,-3.31868636626619));
#59930=CARTESIAN_POINT('Ctrl Pts',(-17.0558296625103,42.2024302014641,-3.48456541848317));
#59931=CARTESIAN_POINT('Ctrl Pts',(-16.1231583043917,43.1958323041313,-3.50684228674254));
#59932=CARTESIAN_POINT('Ctrl Pts',(-16.2020593980967,42.358743766398,-3.14397959827399));
#59933=CARTESIAN_POINT('Ctrl Pts',(-17.1003194136399,42.2851842704153,-3.30611394037726));
#59934=CARTESIAN_POINT('Ctrl Pts',(-16.1368688153599,43.2261249913638,-3.44321966940264));
#59935=CARTESIAN_POINT('Ctrl Pts',(-16.2132166154573,42.3834909358494,-3.0852944650872));
#59936=CARTESIAN_POINT('Ctrl Pts',(-17.1148608648885,42.3121111033463,-3.24613302164169));
#59937=CARTESIAN_POINT('Ctrl Pts',(-16.1570050576291,43.2704363362883,-3.3469780073553));
#59938=CARTESIAN_POINT('Ctrl Pts',(-16.2295461487012,42.4195814461551,-2.99676810231204));
#59939=CARTESIAN_POINT('Ctrl Pts',(-17.1362174853078,42.3514989656337,-3.15540014162311));
#59940=CARTESIAN_POINT('Ctrl Pts',(-16.1636460804533,43.2850199841448,-3.31476016326283));
#59941=CARTESIAN_POINT('Ctrl Pts',(-16.234927397343,42.4314525764685,-2.96714277235139));
#59942=CARTESIAN_POINT('Ctrl Pts',(-17.1432609944394,42.3644622081519,-3.12502641655731));
#59943=CARTESIAN_POINT('Ctrl Pts',(-16.176779066406,43.3138032530051,-3.25006285951472));
#59944=CARTESIAN_POINT('Ctrl Pts',(-16.2455540938229,42.4548543838694,-2.90771276300664));
#59945=CARTESIAN_POINT('Ctrl Pts',(-17.1571899188963,42.3900473359813,-3.0640323254552));
#59946=CARTESIAN_POINT('Ctrl Pts',(-16.1832563592051,43.3279707317643,-3.21765573302902));
#59947=CARTESIAN_POINT('Ctrl Pts',(-16.2507873073283,42.4663580683418,-2.87797525515983));
#59948=CARTESIAN_POINT('Ctrl Pts',(-17.164059774934,42.4026406504781,-3.03348015236247));
#59949=CARTESIAN_POINT('Ctrl Pts',(-16.2407423662139,43.4534701977211,-2.92546660438112));
#59950=CARTESIAN_POINT('Ctrl Pts',(-16.2973926330638,42.5686355463496,-2.60882804918763));
#59951=CARTESIAN_POINT('Ctrl Pts',(-17.2250297821921,42.5141957311396,-2.75801565386698));
#59952=CARTESIAN_POINT('Ctrl Pts',(-16.2860851710674,43.5507845829967,-2.66201787685001));
#59953=CARTESIAN_POINT('Ctrl Pts',(-16.3334056853608,42.6464652770683,-2.36955567429105));
#59954=CARTESIAN_POINT('Ctrl Pts',(-17.27312063616,42.6006974071258,-2.50964648325415));
#59955=CARTESIAN_POINT('Ctrl Pts',(-16.3644674413509,43.7174968151427,-2.12770174998652));
#59956=CARTESIAN_POINT('Ctrl Pts',(-16.395286619085,42.7792030237934,-1.88723589636282));
#59957=CARTESIAN_POINT('Ctrl Pts',(-17.3562533467079,42.7488860578871,-2.00591410770285));
#59958=CARTESIAN_POINT('Ctrl Pts',(-16.3975090775376,43.7868935216046,-1.85683435243505));
#59959=CARTESIAN_POINT('Ctrl Pts',(-16.4209906605381,42.8337387768024,-1.64478289056291));
#59960=CARTESIAN_POINT('Ctrl Pts',(-17.3912975066884,42.810572019061,-1.75055090464328));
#59961=CARTESIAN_POINT('Ctrl Pts',(-16.4371973244655,43.8698191922474,-1.44484551307843));
#59962=CARTESIAN_POINT('Ctrl Pts',(-16.4517290374466,42.8986843931254,-1.27807359738039));
#59963=CARTESIAN_POINT('Ctrl Pts',(-17.4333911016012,42.8842837265137,-1.36214391805839));
#59964=CARTESIAN_POINT('Ctrl Pts',(-16.4487802554229,43.8939261909356,-1.30656641831514));
#59965=CARTESIAN_POINT('Ctrl Pts',(-16.4606689802262,42.9175109064172,-1.15517368833686));
#59966=CARTESIAN_POINT('Ctrl Pts',(-17.4456760285918,42.9057121696064,-1.23177978830181));
#59967=CARTESIAN_POINT('Ctrl Pts',(-16.4685324538335,43.9349488754536,-1.02806931366241));
#59968=CARTESIAN_POINT('Ctrl Pts',(-16.4758894976883,42.9495081386978,-0.908068000066032));
#59969=CARTESIAN_POINT('Ctrl Pts',(-17.4666253297105,42.9421767782951,-0.969223595380726));
#59970=CARTESIAN_POINT('Ctrl Pts',(-16.4767018066094,43.9518647448791,-0.887851353093695));
#59971=CARTESIAN_POINT('Ctrl Pts',(-16.4821582142198,42.9626536650404,-0.783956213361243));
#59972=CARTESIAN_POINT('Ctrl Pts',(-17.4752897950108,42.9572131064008,-0.837031578665104));
#59973=CARTESIAN_POINT('Ctrl Pts',(-16.4862967209135,43.9717089312722,-0.676029616417883));
#59974=CARTESIAN_POINT('Ctrl Pts',(-16.4895137451409,42.9780633749711,-0.596718279805704));
#59975=CARTESIAN_POINT('Ctrl Pts',(-17.4854662190897,42.9748523834323,-0.637334318512984));
#59976=CARTESIAN_POINT('Ctrl Pts',(-16.4890517437789,43.977401569991,-0.605173122314613));
#59977=CARTESIAN_POINT('Ctrl Pts',(-16.4916238230334,42.9824805634447,-0.534110465633991));
#59978=CARTESIAN_POINT('Ctrl Pts',(-17.4883882131625,42.9799125065679,-0.57053358332299));
#59979=CARTESIAN_POINT('Ctrl Pts',(-16.492506023628,43.9845357058383,-0.498508314718125));
#59980=CARTESIAN_POINT('Ctrl Pts',(-16.4942681869357,42.9880140786458,-0.439912398698345));
#59981=CARTESIAN_POINT('Ctrl Pts',(-17.49205184321,42.9862539607906,-0.469974168759785));
#59982=CARTESIAN_POINT('Ctrl Pts',(-16.4935448911152,43.9866805929804,-0.462870708599939));
#59983=CARTESIAN_POINT('Ctrl Pts',(-16.4950632373273,42.9896773373646,-0.408444310922235));
#59984=CARTESIAN_POINT('Ctrl Pts',(-17.4931536723775,42.9881605271315,-0.436376425617608));
#59985=CARTESIAN_POINT('Ctrl Pts',(-16.495392016117,43.9904934577505,-0.391554086603203));
#59986=CARTESIAN_POINT('Ctrl Pts',(-16.4964765826267,42.9926335814917,-0.345482344139571));
#59987=CARTESIAN_POINT('Ctrl Pts',(-17.4951127443838,42.9915497401849,-0.36914189982643));
#59988=CARTESIAN_POINT('Ctrl Pts',(-16.4961991039929,43.9921590221803,-0.355925418204801));
#59989=CARTESIAN_POINT('Ctrl Pts',(-16.4970939068081,42.9939245371181,-0.314034598998794));
#59990=CARTESIAN_POINT('Ctrl Pts',(-17.4959687466422,42.9930302419732,-0.335552582820379));
#59991=CARTESIAN_POINT('Ctrl Pts',(-16.4996553193878,43.9992904788907,-0.177929344977772));
#59992=CARTESIAN_POINT('Ctrl Pts',(-16.499737824245,42.9994528692837,-0.156906377895304));
#59993=CARTESIAN_POINT('Ctrl Pts',(-17.4996344297213,42.9993693144289,-0.167744837011927));
#59994=CARTESIAN_POINT('Ctrl Pts',(-16.5005671676994,44.0011697501096,-0.0360034841747721));
#59995=CARTESIAN_POINT('Ctrl Pts',(-16.5004336035839,43.0009063138008,-0.0317784680747621));
#59996=CARTESIAN_POINT('Ctrl Pts',(-17.5006015414388,43.0010397779723,-0.0339426786824198));
#59997=CARTESIAN_POINT('Ctrl Pts',(-16.4978545553025,43.9955752404001,0.388390909530019));
#59998=CARTESIAN_POINT('Ctrl Pts',(-16.4983604076717,42.9965730007167,0.34258128637437));
#59999=CARTESIAN_POINT('Ctrl Pts',(-17.4977245284721,42.9960668801614,0.366159780026568));
#60000=CARTESIAN_POINT('Ctrl Pts',(-16.488785846129,43.9768969118701,0.669479171266392));
#60001=CARTESIAN_POINT('Ctrl Pts',(-16.4914621272788,42.9821709666193,0.590248849637306));
#60002=CARTESIAN_POINT('Ctrl Pts',(-17.488106200346,42.9794639216913,0.631158814660471));
#60003=CARTESIAN_POINT('Ctrl Pts',(-16.4566137829713,43.9102406346531,1.22805693613211));
#60004=CARTESIAN_POINT('Ctrl Pts',(-16.4667388442969,42.9303002753056,1.08490481084554));
#60005=CARTESIAN_POINT('Ctrl Pts',(-17.4539843153664,42.9202138974404,1.15776411487348));
#60006=CARTESIAN_POINT('Ctrl Pts',(-16.4335093295897,43.8622622073091,1.50554633472257));
#60007=CARTESIAN_POINT('Ctrl Pts',(-16.4489907660971,42.8929980278654,1.33109833842561));
#60008=CARTESIAN_POINT('Ctrl Pts',(-17.4294795919199,42.8775664063642,1.41937028185803));
#60009=CARTESIAN_POINT('Ctrl Pts',(-16.3960891495453,43.783793740335,1.85015317363005));
#60010=CARTESIAN_POINT('Ctrl Pts',(-16.4197798825902,42.8310926576272,1.63991769895437));
#60011=CARTESIAN_POINT('Ctrl Pts',(-17.3897915222624,42.8078166581088,1.74425215023244));
#60012=CARTESIAN_POINT('Ctrl Pts',(-16.3881779026531,43.767173088473,1.91896157031875));
#60013=CARTESIAN_POINT('Ctrl Pts',(-16.4136093423201,42.817995097094,1.70150596722071));
#60014=CARTESIAN_POINT('Ctrl Pts',(-17.3814008058283,42.7930427452666,1.80912201914365));
#60015=CARTESIAN_POINT('Ctrl Pts',(-16.375673948842,43.740841555206,2.0220039170481));
#60016=CARTESIAN_POINT('Ctrl Pts',(-16.4038270264028,42.7971893690875,1.79393530076847));
#60017=CARTESIAN_POINT('Ctrl Pts',(-17.3681390366586,42.7696369379822,1.90626631910862));
#60018=CARTESIAN_POINT('Ctrl Pts',(-16.3713997812811,43.7318309227685,2.05632298830878));
#60019=CARTESIAN_POINT('Ctrl Pts',(-16.4004812785263,42.7900667948439,1.82472882562818));
#60020=CARTESIAN_POINT('Ctrl Pts',(-17.3636058286238,42.7616274868815,1.93862099907206));
#60021=CARTESIAN_POINT('Ctrl Pts',(-16.3626396751579,43.7133407089755,2.12490420765856));
#60022=CARTESIAN_POINT('Ctrl Pts',(-16.3936154941633,42.7754354074154,1.88631707234903));
#60023=CARTESIAN_POINT('Ctrl Pts',(-17.3543148069932,42.7451917413354,2.0032766940958));
#60024=CARTESIAN_POINT('Ctrl Pts',(-16.3581504674953,43.7038542075336,2.15919050412873));
#60025=CARTESIAN_POINT('Ctrl Pts',(-16.3900932136698,42.7679218136654,1.9171321516777));
#60026=CARTESIAN_POINT('Ctrl Pts',(-17.3495535260841,42.7367592956301,2.03560047527918));
#60027=CARTESIAN_POINT('Ctrl Pts',(-16.335218649852,43.6553329579177,2.33016678950607));
#60028=CARTESIAN_POINT('Ctrl Pts',(-16.3721055730023,42.7295090646878,2.07069458061821));
#60029=CARTESIAN_POINT('Ctrl Pts',(-17.3252319015473,42.6936292957481,2.19679023923976));
#60030=CARTESIAN_POINT('Ctrl Pts',(-16.315354751774,43.6131097667714,2.46525055695651));
#60031=CARTESIAN_POINT('Ctrl Pts',(-16.3564409704719,42.6959272836267,2.19259820200646));
#60032=CARTESIAN_POINT('Ctrl Pts',(-17.3041641304931,42.6560975705951,2.32414193923568));
#60033=CARTESIAN_POINT('Ctrl Pts',(-16.2515056057596,43.4765147512805,2.8655905997197));
#60034=CARTESIAN_POINT('Ctrl Pts',(-16.3058885440615,42.5869423044208,2.55446830067613));
#60035=CARTESIAN_POINT('Ctrl Pts',(-17.2364453397946,42.5346797786526,2.7015668953238));
#60036=CARTESIAN_POINT('Ctrl Pts',(-16.2032672081898,43.3722448995847,3.12594764367366));
#60037=CARTESIAN_POINT('Ctrl Pts',(-16.2673330709852,42.5030995032564,2.7919929023725));
#60038=CARTESIAN_POINT('Ctrl Pts',(-17.1852834023163,42.441995466392,2.94702134755456));
#60039=CARTESIAN_POINT('Ctrl Pts',(-16.0968875664402,43.1381380127393,3.63422998231717));
#60040=CARTESIAN_POINT('Ctrl Pts',(-16.1809970935074,42.3122776252218,3.25988799511517));
#60041=CARTESIAN_POINT('Ctrl Pts',(-17.07245651017,42.2339004556738,3.42621008435598));
#60042=CARTESIAN_POINT('Ctrl Pts',(-16.0387426559475,43.0082992884229,3.88215383492437));
#60043=CARTESIAN_POINT('Ctrl Pts',(-16.1333904856796,42.2057238967836,3.48991370242924));
#60044=CARTESIAN_POINT('Ctrl Pts',(-17.0107876651219,42.118488256322,3.65994300926234));
#60045=CARTESIAN_POINT('Ctrl Pts',(-15.9607089630699,42.8300074294681,4.18445557032663));
#60046=CARTESIAN_POINT('Ctrl Pts',(-16.0682434684036,42.0567601433772,3.77421115204722));
#60047=CARTESIAN_POINT('Ctrl Pts',(-16.9280246578707,41.9600066039851,3.94494127844591));
#60048=CARTESIAN_POINT('Ctrl Pts',(-15.9448345125254,42.7935473084438,4.2445349020985));
#60049=CARTESIAN_POINT('Ctrl Pts',(-16.0550169591108,42.026372413421,3.83055888715714));
#60050=CARTESIAN_POINT('Ctrl Pts',(-16.9111881192775,41.9275976074833,4.00158172585483));
#60051=CARTESIAN_POINT('Ctrl Pts',(-15.9125710995365,42.7190148602521,4.3639323057479));
#60052=CARTESIAN_POINT('Ctrl Pts',(-16.0280522148975,41.964087720814,3.94277369967183));
#60053=CARTESIAN_POINT('Ctrl Pts',(-16.8769693480609,41.8613465424687,4.1141449347411));
#60054=CARTESIAN_POINT('Ctrl Pts',(-15.8961777996028,42.6809324048149,4.42326572017825));
#60055=CARTESIAN_POINT('Ctrl Pts',(-16.0143130159987,41.9321895117794,3.99865250806258));
#60056=CARTESIAN_POINT('Ctrl Pts',(-16.8595825146128,41.8274954710167,4.17008216045151));
#60057=CARTESIAN_POINT('Ctrl Pts',(-15.8462844618934,42.5643109368609,4.60002845907672));
#60058=CARTESIAN_POINT('Ctrl Pts',(-15.9724388258778,41.8344100525786,4.16519179553658));
#60059=CARTESIAN_POINT('Ctrl Pts',(-16.8066653386068,41.723831943736,4.33672716677812));
#60060=CARTESIAN_POINT('Ctrl Pts',(-15.8122905956358,42.4839122053499,4.71544824060082));
#60061=CARTESIAN_POINT('Ctrl Pts',(-15.9437057928047,41.7665897154923,4.27457431431909));
#60062=CARTESIAN_POINT('Ctrl Pts',(-16.7706112375754,41.652366404853,4.44554042885686));
#60063=CARTESIAN_POINT('Ctrl Pts',(-15.708466257085,42.2349319229732,5.05470392926197));
#60064=CARTESIAN_POINT('Ctrl Pts',(-15.8557182823553,41.5561640523473,4.59624091151791));
#60065=CARTESIAN_POINT('Ctrl Pts',(-16.6604945155305,41.4310505980033,4.76537744171326));
#60066=CARTESIAN_POINT('Ctrl Pts',(-15.6367937805477,42.0585895493903,5.27155542705688));
#60067=CARTESIAN_POINT('Ctrl Pts',(-15.7941524221352,41.4054489545328,4.80429063353521));
#60068=CARTESIAN_POINT('Ctrl Pts',(-16.5844782517039,41.274301821729,4.96981656414753));
#60069=CARTESIAN_POINT('Ctrl Pts',(-15.490346672854,41.6855007303992,5.68751055477781));
#60070=CARTESIAN_POINT('Ctrl Pts',(-15.6669541386688,41.0833353282907,5.20593767654318));
#60071=CARTESIAN_POINT('Ctrl Pts',(-16.42915556251,40.9426673158617,5.36196281266631));
#60072=CARTESIAN_POINT('Ctrl Pts',(-15.4155675047962,41.4887542028889,5.88661251495239));
#60073=CARTESIAN_POINT('Ctrl Pts',(-15.6013785695094,40.9122288799408,5.39970005563699));
#60074=CARTESIAN_POINT('Ctrl Pts',(-16.3498443229104,40.7677815136044,5.54966836406231));
#60075=CARTESIAN_POINT('Ctrl Pts',(-15.3024448812762,41.1779991716065,6.17216839972268));
#60076=CARTESIAN_POINT('Ctrl Pts',(-15.5009241601739,40.6387285873814,5.6799934650858));
#60077=CARTESIAN_POINT('Ctrl Pts',(-16.2298657833509,40.4915548192431,5.81887929950314));
#60078=CARTESIAN_POINT('Ctrl Pts',(-15.2645790020526,41.0718024829547,6.26516634094168));
#60079=CARTESIAN_POINT('Ctrl Pts',(-15.4672614165944,40.5452444380058,5.77127906622756));
#60080=CARTESIAN_POINT('Ctrl Pts',(-16.1897050020046,40.3971577625623,5.90655412600363));
#60081=CARTESIAN_POINT('Ctrl Pts',(-15.2077254227751,40.9084929741541,6.4013676517502));
#60082=CARTESIAN_POINT('Ctrl Pts',(-15.4164278105277,40.4007199180155,5.90553521152224));
#60083=CARTESIAN_POINT('Ctrl Pts',(-16.1294057515143,40.2519937548357,6.03495940239176));
#60084=CARTESIAN_POINT('Ctrl Pts',(-15.1887651989012,40.853386989109,6.44621852703614));
#60085=CARTESIAN_POINT('Ctrl Pts',(-15.3994674120309,40.3519488749432,5.94974031533987));
#60086=CARTESIAN_POINT('Ctrl Pts',(-16.1092964229923,40.2030106569473,6.07724305571356));
#60087=CARTESIAN_POINT('Ctrl Pts',(-15.1508585131677,40.7418148130405,6.53481506085914));
#60088=CARTESIAN_POINT('Ctrl Pts',(-15.365491794666,40.2530328359572,6.03717495128596));
#60089=CARTESIAN_POINT('Ctrl Pts',(-16.0690923625353,40.1038353894078,6.16076840762205));
#60090=CARTESIAN_POINT('Ctrl Pts',(-15.1319787469483,40.685544542223,6.57840481672826));
#60091=CARTESIAN_POINT('Ctrl Pts',(-15.348535637605,40.2030632212813,6.08025593853515));
#60092=CARTESIAN_POINT('Ctrl Pts',(-16.0490683678638,40.0538173708934,6.20186312687394));
#60093=CARTESIAN_POINT('Ctrl Pts',(-15.0380664911524,40.4019030685421,6.79276143414887));
#60094=CARTESIAN_POINT('Ctrl Pts',(-15.2644245680603,39.9519367964584,6.29138993605124));
#60095=CARTESIAN_POINT('Ctrl Pts',(-15.9494644607597,39.8016916163679,6.40395017364007));
#60096=CARTESIAN_POINT('Ctrl Pts',(-14.9644461532019,40.1675514041411,6.95288768593992));
#60097=CARTESIAN_POINT('Ctrl Pts',(-15.1976171693671,39.7421821058477,6.45092268656129));
#60098=CARTESIAN_POINT('Ctrl Pts',(-15.8713822833035,39.5933790259089,6.55491094954876));
#60099=CARTESIAN_POINT('Ctrl Pts',(-14.8222211698946,39.6838140960417,7.25114166432459));
#60100=CARTESIAN_POINT('Ctrl Pts',(-15.06786594057,39.3068953284827,6.74885869506734));
#60101=CARTESIAN_POINT('Ctrl Pts',(-15.7205376048291,39.1633903075869,6.83609315171071));
#60102=CARTESIAN_POINT('Ctrl Pts',(-14.7536128479239,39.4344290298586,7.38926853498414));
#60103=CARTESIAN_POINT('Ctrl Pts',(-15.0048054725226,39.0812939904251,6.88766092280371));
#60104=CARTESIAN_POINT('Ctrl Pts',(-15.6477712019922,38.9417146931311,6.96631377005003));
#60105=CARTESIAN_POINT('Ctrl Pts',(-14.6235443336384,38.9199395169773,7.64345031191053));
#60106=CARTESIAN_POINT('Ctrl Pts',(-14.8848011659622,38.6139543580119,7.14351801279062));
#60107=CARTESIAN_POINT('Ctrl Pts',(-15.5098197481496,38.4843906818341,7.20594642230858));
#60108=CARTESIAN_POINT('Ctrl Pts',(-14.5620800221653,38.6548384656211,7.7595087284317));
#60109=CARTESIAN_POINT('Ctrl Pts',(-14.827716689627,38.3720620877045,7.26095612384862));
#60110=CARTESIAN_POINT('Ctrl Pts',(-15.4446303262328,38.2487453026412,7.31536176370244));
#60111=CARTESIAN_POINT('Ctrl Pts',(-14.4912109590877,38.3128451067789,7.89022745753408));
#60112=CARTESIAN_POINT('Ctrl Pts',(-14.7615399553527,38.0581196581985,7.39373762359809));
#60113=CARTESIAN_POINT('Ctrl Pts',(-15.369466168806,37.944751206059,7.43859827658201));
#60114=CARTESIAN_POINT('Ctrl Pts',(-14.4773360216078,38.2439139811986,7.91565127929397));
#60115=CARTESIAN_POINT('Ctrl Pts',(-14.7486090785329,37.9949822886081,7.41950389459761));
#60116=CARTESIAN_POINT('Ctrl Pts',(-15.3547503258741,37.883479094363,7.46256686250324));
#60117=CARTESIAN_POINT('Ctrl Pts',(-14.4570026893877,38.1396985883734,7.95268958299778));
#60118=CARTESIAN_POINT('Ctrl Pts',(-14.7296347176249,37.8994093453111,7.45707777466083));
#60119=CARTESIAN_POINT('Ctrl Pts',(-15.3331846705994,37.7908431896831,7.49748512881753));
#60120=CARTESIAN_POINT('Ctrl Pts',(-14.4502995623675,38.1047958815478,7.9648621653037));
#60121=CARTESIAN_POINT('Ctrl Pts',(-14.7233795289916,37.8674039475413,7.46942463090051));
#60122=CARTESIAN_POINT('Ctrl Pts',(-15.326075293378,37.7598185613842,7.50896096392519));
#60123=CARTESIAN_POINT('Ctrl Pts',(-14.4370862536553,38.0348626145466,7.98878759631039));
#60124=CARTESIAN_POINT('Ctrl Pts',(-14.711044089513,37.8032526976823,7.49369902639856));
#60125=CARTESIAN_POINT('Ctrl Pts',(-15.3120611781612,37.6976556573663,7.531516925812));
#60126=CARTESIAN_POINT('Ctrl Pts',(-14.430578191227,37.9998443555349,8.00053668324475));
#60127=CARTESIAN_POINT('Ctrl Pts',(-14.7049654891278,37.7711173950731,7.50562346769514));
#60128=CARTESIAN_POINT('Ctrl Pts',(-15.3051586876244,37.6665283160382,7.54259350608998));
#60129=CARTESIAN_POINT('Ctrl Pts',(-14.3985378950991,37.8244951111472,8.05821896776018));
#60130=CARTESIAN_POINT('Ctrl Pts',(-14.6750683621745,37.6103672676509,7.56410181532715));
#60131=CARTESIAN_POINT('Ctrl Pts',(-15.2711765555705,37.5106623209909,7.59697411101706));
#60132=CARTESIAN_POINT('Ctrl Pts',(-14.3745058364078,37.6833906877742,8.10096493484399));
#60133=CARTESIAN_POINT('Ctrl Pts',(-14.652561930448,37.4806229720141,7.60757184213281));
#60134=CARTESIAN_POINT('Ctrl Pts',(-15.2456880081703,37.3852361669233,7.63727333921995));
#60135=CARTESIAN_POINT('Ctrl Pts',(-14.3074780704631,37.2575991659697,8.21914076587046));
#60136=CARTESIAN_POINT('Ctrl Pts',(-14.5898331467566,37.0893377713944,7.72760627073598));
#60137=CARTESIAN_POINT('Ctrl Pts',(-15.1745979538034,37.0067548141695,7.74868489717074));
#60138=CARTESIAN_POINT('Ctrl Pts',(-14.2695523034726,36.9704386282229,8.28453464061196));
#60139=CARTESIAN_POINT('Ctrl Pts',(-14.5540974775854,36.8241663199945,7.79441727640368));
#60140=CARTESIAN_POINT('Ctrl Pts',(-15.1343736550051,36.7515010028509,7.81033568794618));
#60141=CARTESIAN_POINT('Ctrl Pts',(-14.2086105787285,36.3893814021093,8.38862459376293));
#60142=CARTESIAN_POINT('Ctrl Pts',(-14.4967075641971,36.2872858361014,7.90063819784113));
#60143=CARTESIAN_POINT('Ctrl Pts',(-15.069738492784,36.2350056907777,7.90846763065641));
#60144=CARTESIAN_POINT('Ctrl Pts',(-14.1855946049829,36.0954849072401,8.42732167623407));
#60145=CARTESIAN_POINT('Ctrl Pts',(-14.474938277723,36.0150460990806,7.94027178393654));
#60146=CARTESIAN_POINT('Ctrl Pts',(-15.04532761125,35.9737643619689,7.94494972814297));
#60147=CARTESIAN_POINT('Ctrl Pts',(-14.1632592796937,35.6493675288365,8.46476803043535));
#60148=CARTESIAN_POINT('Ctrl Pts',(-14.4538374531707,35.601719694416,7.97857185535198));
#60149=CARTESIAN_POINT('Ctrl Pts',(-15.0216386300259,35.5772155811991,7.98025268877251));
#60150=CARTESIAN_POINT('Ctrl Pts',(-14.1578452220156,35.4997817266829,8.47381023741147));
#60151=CARTESIAN_POINT('Ctrl Pts',(-14.4487195544893,35.4631107873063,7.98782407910831));
#60152=CARTESIAN_POINT('Ctrl Pts',(-15.0158964475708,35.4442504237115,7.98877732802181));
#60153=CARTESIAN_POINT('Ctrl Pts',(-14.1528931524912,35.2740434072532,8.48207673460457));
#60154=CARTESIAN_POINT('Ctrl Pts',(-14.4440400975708,35.2539384493497,7.99627922136717));
#60155=CARTESIAN_POINT('Ctrl Pts',(-15.0106442526529,35.2435941397839,7.99657065897525));
#60156=CARTESIAN_POINT('Ctrl Pts',(-14.1517706094402,35.1985706100121,8.48394895723216));
#60157=CARTESIAN_POINT('Ctrl Pts',(-14.442979184077,35.184001549869,7.9981943881281));
#60158=CARTESIAN_POINT('Ctrl Pts',(-15.0094536766753,35.1765072088985,7.99833571715932));
#60159=CARTESIAN_POINT('Ctrl Pts',(-14.1508941306251,35.0850155880073,8.4854107517919));
#60160=CARTESIAN_POINT('Ctrl Pts',(-14.4421509241428,35.078778187705,7.99968953263258));
#60161=CARTESIAN_POINT('Ctrl Pts',(-15.0085240779375,35.0755694115626,7.99971384012147));
#60162=CARTESIAN_POINT('Ctrl Pts',(-14.150736560916,35.0470814239072,8.48567350216556));
#60163=CARTESIAN_POINT('Ctrl Pts',(-14.4420020169164,35.0436268600821,7.99995828626213));
#60164=CARTESIAN_POINT('Ctrl Pts',(-15.0083569585472,35.0418501545842,7.99996155087807));
#60165=CARTESIAN_POINT('Ctrl Pts',(-14.150692918513,34.9712377388823,8.48574627995365));
#60166=CARTESIAN_POINT('Ctrl Pts',(-14.4419607755292,34.9733482312172,8.0000327238654));
#60167=CARTESIAN_POINT('Ctrl Pts',(-15.0083106711502,34.9744335456731,8.00003016290435));
#60168=CARTESIAN_POINT('Ctrl Pts',(-14.1508066226917,34.9333329107061,8.48555667952094));
#60169=CARTESIAN_POINT('Ctrl Pts',(-14.4420682290436,34.9382240120611,7.99983879114063));
#60170=CARTESIAN_POINT('Ctrl Pts',(-15.0084312664928,34.940740365072,7.99985141504979));
#60171=CARTESIAN_POINT('Ctrl Pts',(-14.1520509011363,34.7438936238919,8.48348153993902));
#60172=CARTESIAN_POINT('Ctrl Pts',(-14.4432440959225,34.7626780463408,7.99771623713472));
#60173=CARTESIAN_POINT('Ctrl Pts',(-15.0097509557443,34.7723498879043,7.9978950544351));
#60174=CARTESIAN_POINT('Ctrl Pts',(-14.1552091806869,34.5926136214512,8.4782167591127));
#60175=CARTESIAN_POINT('Ctrl Pts',(-14.4462304856527,34.6224662811345,7.99232810421143));
#60176=CARTESIAN_POINT('Ctrl Pts',(-15.0131006462177,34.6378787746227,7.99293162477818));
#60177=CARTESIAN_POINT('Ctrl Pts',(-14.1631498026642,34.366097861864,8.46494029855902));
#60178=CARTESIAN_POINT('Ctrl Pts',(-14.4537301008296,34.4126736274608,7.97875461899514));
#60179=CARTESIAN_POINT('Ctrl Pts',(-15.0215225179599,34.4365314327682,7.98041509627186));
#60180=CARTESIAN_POINT('Ctrl Pts',(-14.1663304572642,34.2906600038508,8.45961782992988));
#60181=CARTESIAN_POINT('Ctrl Pts',(-14.4567347009781,34.34279668575,7.97331176954809));
#60182=CARTESIAN_POINT('Ctrl Pts',(-15.0248959395469,34.3694755589792,7.975397280748));
#60183=CARTESIAN_POINT('Ctrl Pts',(-14.1718962020967,34.1776041375939,8.45028822882502));
#60184=CARTESIAN_POINT('Ctrl Pts',(-14.4619896761171,34.2381138641883,7.96377525778024));
#60185=CARTESIAN_POINT('Ctrl Pts',(-15.0307990022117,34.2689814556387,7.96660169720576));
#60186=CARTESIAN_POINT('Ctrl Pts',(-14.1738839055404,34.1399356702887,8.44695401845093));
#60187=CARTESIAN_POINT('Ctrl Pts',(-14.4638665061005,34.2032333257984,7.96036678089891));
#60188=CARTESIAN_POINT('Ctrl Pts',(-15.0329071725568,34.2354983735906,7.96345833389448));
#60189=CARTESIAN_POINT('Ctrl Pts',(-14.1781231744824,34.0646323657967,8.43983651540518));
#60190=CARTESIAN_POINT('Ctrl Pts',(-14.4678686428001,34.1335117477056,7.95309163191476));
#60191=CARTESIAN_POINT('Ctrl Pts',(-15.0374033668614,34.1685621029298,7.95674823001028));
#60192=CARTESIAN_POINT('Ctrl Pts',(-14.1803761277451,34.026976116557,8.43605088762219));
#60193=CARTESIAN_POINT('Ctrl Pts',(-14.4699954006696,34.0986496666099,7.9492223146372));
#60194=CARTESIAN_POINT('Ctrl Pts',(-15.039792862775,34.1350898813783,7.953179288052));
#60195=CARTESIAN_POINT('Ctrl Pts',(-14.2018025764259,33.6887269670264,8.40001146214908));
#60196=CARTESIAN_POINT('Ctrl Pts',(-14.4902406725494,33.7851897713294,7.91234974711415));
#60197=CARTESIAN_POINT('Ctrl Pts',(-15.062517883968,33.8344239707358,7.91920272479425));
#60198=CARTESIAN_POINT('Ctrl Pts',(-14.2289622534947,33.3934618841932,8.35411823426493));
#60199=CARTESIAN_POINT('Ctrl Pts',(-14.5159096719755,33.5118586162235,7.86536934014895));
#60200=CARTESIAN_POINT('Ctrl Pts',(-15.091323602403,33.5719661192377,7.87593638279283));
#60201=CARTESIAN_POINT('Ctrl Pts',(-14.297587136116,32.8129757621643,8.2361192541527));
#60202=CARTESIAN_POINT('Ctrl Pts',(-14.5804718486074,32.975939942154,7.74503244923851));
#60203=CARTESIAN_POINT('Ctrl Pts',(-15.1641075683963,33.0559784553022,7.76469155241571));
#60204=CARTESIAN_POINT('Ctrl Pts',(-14.3390533631708,32.5277562904371,8.16400873147055));
#60205=CARTESIAN_POINT('Ctrl Pts',(-14.6194905451471,32.7128565901746,7.67142630106037));
#60206=CARTESIAN_POINT('Ctrl Pts',(-15.2080869006233,32.8024500359307,7.6967085685757));
#60207=CARTESIAN_POINT('Ctrl Pts',(-14.4344512245411,31.9668958072417,7.99412958149491));
#60208=CARTESIAN_POINT('Ctrl Pts',(-14.7087759143519,32.1972833069676,7.49877760542043));
#60209=CARTESIAN_POINT('Ctrl Pts',(-15.3092664499803,32.3039073842282,7.53655314061732));
#60210=CARTESIAN_POINT('Ctrl Pts',(-14.4883838105694,31.691255013237,7.89636074701349));
#60211=CARTESIAN_POINT('Ctrl Pts',(-14.7592010426945,31.9443746233512,7.39939956315832));
#60212=CARTESIAN_POINT('Ctrl Pts',(-15.3664676782412,32.0588933451493,7.44438050229219));
#60213=CARTESIAN_POINT('Ctrl Pts',(-14.5550635668316,31.3864313723232,7.77176756628671));
#60214=CARTESIAN_POINT('Ctrl Pts',(-14.8209199446041,31.6669143175934,7.27386759669347));
#60215=CARTESIAN_POINT('Ctrl Pts',(-15.4371886314425,31.7879389976144,7.32691891770422));
#60216=CARTESIAN_POINT('Ctrl Pts',(-14.5625558613898,31.352635473547,7.75772049298618));
#60217=CARTESIAN_POINT('Ctrl Pts',(-14.827877420134,31.6360499048315,7.25966604997201));
#60218=CARTESIAN_POINT('Ctrl Pts',(-15.4451350045509,31.7578981987159,7.31367588564878));
#60219=CARTESIAN_POINT('Ctrl Pts',(-14.5777038502899,31.2851903557158,7.72921800162461));
#60220=CARTESIAN_POINT('Ctrl Pts',(-14.8419359589025,31.5744837961381,7.2308617271771));
#60221=CARTESIAN_POINT('Ctrl Pts',(-15.4612010532912,31.697946982851,7.28680485001122));
#60222=CARTESIAN_POINT('Ctrl Pts',(-14.5853648004003,31.2515184553974,7.71475260653216));
#60223=CARTESIAN_POINT('Ctrl Pts',(-14.849042235293,31.543760796002,7.21624805914054));
#60224=CARTESIAN_POINT('Ctrl Pts',(-15.469326303495,31.6680164047788,7.2731674405612));
#60225=CARTESIAN_POINT('Ctrl Pts',(-14.6085452032034,31.1509057610832,7.67082157327148));
#60226=CARTESIAN_POINT('Ctrl Pts',(-14.8705436711721,31.4519516854403,7.171859977806));
#60227=CARTESIAN_POINT('Ctrl Pts',(-15.4939115790748,31.5785828987784,7.2317509780494));
#60228=CARTESIAN_POINT('Ctrl Pts',(-14.6242529880176,31.0844047949656,7.64083891095088));
#60229=CARTESIAN_POINT('Ctrl Pts',(-14.8850903709531,31.3913603681064,7.14160216923058));
#60230=CARTESIAN_POINT('Ctrl Pts',(-15.5105713510105,31.5194709288242,7.20348449527989));
#60231=CARTESIAN_POINT('Ctrl Pts',(-14.6720790763943,30.8865851637151,7.54883265535859));
#60232=CARTESIAN_POINT('Ctrl Pts',(-14.929376159556,31.2110903439192,7.04872760978158));
#60233=CARTESIAN_POINT('Ctrl Pts',(-15.5612959899498,31.3436312567038,7.11674459069576));
#60234=CARTESIAN_POINT('Ctrl Pts',(-14.7048994575313,30.7569483641181,7.48475247389081));
#60235=CARTESIAN_POINT('Ctrl Pts',(-14.95966877612,31.0933259986506,6.98419535501427));
#60236=CARTESIAN_POINT('Ctrl Pts',(-15.5961054854356,31.2283985458312,7.05633229878906));
#60237=CARTESIAN_POINT('Ctrl Pts',(-14.8057173802565,30.3745068040017,7.28444119078806));
#60238=CARTESIAN_POINT('Ctrl Pts',(-15.052677543726,30.7458140689667,6.78241054451384));
#60239=CARTESIAN_POINT('Ctrl Pts',(-15.7030335847703,30.888450492549,6.86748664417107));
#60240=CARTESIAN_POINT('Ctrl Pts',(-14.8760647694745,30.1281517423914,7.14016324914458));
#60241=CARTESIAN_POINT('Ctrl Pts',(-15.1171363078512,30.5235314070459,6.63773030177344));
#60242=CARTESIAN_POINT('Ctrl Pts',(-15.7776444528623,30.6694682154397,6.73146703642075));
#60243=CARTESIAN_POINT('Ctrl Pts',(-15.0208334639485,29.6517703450343,6.83035843117765));
#60244=CARTESIAN_POINT('Ctrl Pts',(-15.2487759421767,30.0960400709944,6.32894683063836));
#60245=CARTESIAN_POINT('Ctrl Pts',(-15.9311870068286,30.2460180844943,6.43939515378203));
#60246=CARTESIAN_POINT('Ctrl Pts',(-15.0952589444123,29.4217455787918,6.66483128140236));
#60247=CARTESIAN_POINT('Ctrl Pts',(-15.3160581108554,29.8908120505933,6.16445964685839));
#60248=CARTESIAN_POINT('Ctrl Pts',(-16.0101231232976,30.0415516256819,6.28334262225704));
#60249=CARTESIAN_POINT('Ctrl Pts',(-15.1895776666482,29.1442442832826,6.4443022486447));
#60250=CARTESIAN_POINT('Ctrl Pts',(-15.4001942830716,29.6459545222953,5.94785171931794));
#60251=CARTESIAN_POINT('Ctrl Pts',(-16.1101581311846,29.79488380734,6.07543646335386));
#60252=CARTESIAN_POINT('Ctrl Pts',(-15.2085060076969,29.0892469278519,6.39951354132192));
#60253=CARTESIAN_POINT('Ctrl Pts',(-15.4171256703624,29.5972806483711,5.90370851153158));
#60254=CARTESIAN_POINT('Ctrl Pts',(-16.1302336446393,29.745997269232,6.03321141943556));
#60255=CARTESIAN_POINT('Ctrl Pts',(-15.2369722744217,29.0075062116329,6.33129394724583));
#60256=CARTESIAN_POINT('Ctrl Pts',(-15.4425151412656,29.5251196490867,5.83662745356123));
#60257=CARTESIAN_POINT('Ctrl Pts',(-16.160425139482,29.6733388547696,5.96889665059839));
#60258=CARTESIAN_POINT('Ctrl Pts',(-15.246473323653,28.980385210548,6.30838130181911));
#60259=CARTESIAN_POINT('Ctrl Pts',(-15.4509873595446,29.5011789547939,5.81409473052649));
#60260=CARTESIAN_POINT('Ctrl Pts',(-16.170502009992,29.6492312982821,5.94729550340031));
#60261=CARTESIAN_POINT('Ctrl Pts',(-15.2654961612181,28.926395398229,6.26220810975159));
#60262=CARTESIAN_POINT('Ctrl Pts',(-15.4679323239667,29.4535620737581,5.76872117594484));
#60263=CARTESIAN_POINT('Ctrl Pts',(-16.1906777466895,29.601240353964,5.90376522131281));
#60264=CARTESIAN_POINT('Ctrl Pts',(-15.2750230398706,28.8995124220965,6.23893492398287));
#60265=CARTESIAN_POINT('Ctrl Pts',(-15.4764096537653,29.4298736780045,5.74586728371073));
#60266=CARTESIAN_POINT('Ctrl Pts',(-16.2007820120252,29.5773443751773,5.88182417079429));
#60267=CARTESIAN_POINT('Ctrl Pts',(-15.3225922161938,28.7660296571919,6.12195830143935));
#60268=CARTESIAN_POINT('Ctrl Pts',(-15.5187963268113,29.3120701815224,5.63080434349472));
#60269=CARTESIAN_POINT('Ctrl Pts',(-16.2512341685254,29.4586930286934,5.77154317966401));
#60270=CARTESIAN_POINT('Ctrl Pts',(-15.3604967735573,28.6620554042277,6.02628494806573));
#60271=CARTESIAN_POINT('Ctrl Pts',(-15.552341978002,29.22088933467,5.5371846231952));
#60272=CARTESIAN_POINT('Ctrl Pts',(-16.2914359721255,29.3662714703737,5.68134607909259));
#60273=CARTESIAN_POINT('Ctrl Pts',(-15.4734024711476,28.3583437765312,5.73303598356708));
#60274=CARTESIAN_POINT('Ctrl Pts',(-15.6521452749257,28.9546179419119,5.25025045759224));
#60275=CARTESIAN_POINT('Ctrl Pts',(-16.4111844387542,29.0963055792408,5.40488240853399));
#60276=CARTESIAN_POINT('Ctrl Pts',(-15.5475928105337,28.166793334864,5.52924812560617));
#60277=CARTESIAN_POINT('Ctrl Pts',(-15.716867186315,28.7887594038429,5.0526403038573));
#60278=CARTESIAN_POINT('Ctrl Pts',(-16.4898711630596,28.9260385198999,5.21275917575155));
#60279=CARTESIAN_POINT('Ctrl Pts',(-15.6920332500668,27.804967416518,5.10493090212559));
#60280=CARTESIAN_POINT('Ctrl Pts',(-15.8416653101424,28.4777545766966,4.64442044202835));
#60281=CARTESIAN_POINT('Ctrl Pts',(-16.6430655678803,28.6044154813285,4.8127294699215));
#60282=CARTESIAN_POINT('Ctrl Pts',(-15.7622877731009,27.6346927109898,4.88440241921411));
#60283=CARTESIAN_POINT('Ctrl Pts',(-15.9016653391294,28.3329345034696,4.43369484971485));
#60284=CARTESIAN_POINT('Ctrl Pts',(-16.7175779415832,28.4530601877117,4.6048238295626));
#60285=CARTESIAN_POINT('Ctrl Pts',(-15.8634153592665,27.3953869383753,4.54052076838177));
#60286=CARTESIAN_POINT('Ctrl Pts',(-15.9868838517309,28.1316515312056,4.10893296665195));
#60287=CARTESIAN_POINT('Ctrl Pts',(-16.8248344717416,28.2403439451399,4.280625640225));
#60288=CARTESIAN_POINT('Ctrl Pts',(-15.8964154242514,27.3183086387693,4.42370773816891));
#60289=CARTESIAN_POINT('Ctrl Pts',(-16.0146143413019,28.0669533026489,3.99868427600105));
#60290=CARTESIAN_POINT('Ctrl Pts',(-16.8598345410939,28.1718299012522,4.17049887771516));
#60291=CARTESIAN_POINT('Ctrl Pts',(-15.9446833059184,27.2068010501802,4.24510042840518));
#60292=CARTESIAN_POINT('Ctrl Pts',(-16.0548906467027,27.9739186191265,3.83109036355919));
#60293=CARTESIAN_POINT('Ctrl Pts',(-16.9110277485907,28.0727120445427,4.00211488200807));
#60294=CARTESIAN_POINT('Ctrl Pts',(-15.9605671695884,27.1703172329925,4.18499971903105));
#60295=CARTESIAN_POINT('Ctrl Pts',(-16.0681256678962,27.9435097431242,3.7747202284785));
#60296=CARTESIAN_POINT('Ctrl Pts',(-16.9278742708902,28.0402819849552,3.94545428055366));
#60297=CARTESIAN_POINT('Ctrl Pts',(-15.9840630498228,27.1166326670936,4.09398463298263));
#60298=CARTESIAN_POINT('Ctrl Pts',(-16.0876324266849,27.8989052244231,3.68960145288528));
#60299=CARTESIAN_POINT('Ctrl Pts',(-16.9527941436941,27.9925623707134,3.85964881224669));
#60300=CARTESIAN_POINT('Ctrl Pts',(-15.9918400182461,27.098911365518,4.06350224576308));
#60301=CARTESIAN_POINT('Ctrl Pts',(-16.0940844067552,27.8841885644318,3.66110082717283));
#60302=CARTESIAN_POINT('Ctrl Pts',(-16.9610424436527,27.9768101027221,3.83091120811858));
#60303=CARTESIAN_POINT('Ctrl Pts',(-16.0072802673827,27.0638183876329,4.00224638321511));
#60304=CARTESIAN_POINT('Ctrl Pts',(-16.1068754781049,27.8550811453129,3.60388755733143));
#60305=CARTESIAN_POINT('Ctrl Pts',(-16.9774184653475,27.9456163445231,3.77316157340969));
#60306=CARTESIAN_POINT('Ctrl Pts',(-16.0149484597681,27.0464356133835,3.97145286285566));
#60307=CARTESIAN_POINT('Ctrl Pts',(-16.11321832627,27.8406819961272,3.57515643717542));
#60308=CARTESIAN_POINT('Ctrl Pts',(-16.9855513967497,27.9301649896533,3.74413064513307));
#60309=CARTESIAN_POINT('Ctrl Pts',(-16.0833253347986,26.8918211440726,3.69342860679508));
#60310=CARTESIAN_POINT('Ctrl Pts',(-16.1700064472163,27.7120571742295,3.3145971632474));
#60311=CARTESIAN_POINT('Ctrl Pts',(-17.0580723245784,27.7927299060094,3.48202023522934));
#60312=CARTESIAN_POINT('Ctrl Pts',(-16.1392489563977,26.7681000791065,3.44139585389464));
#60313=CARTESIAN_POINT('Ctrl Pts',(-16.2154998129262,27.611079704592,3.08181765987248));
#60314=CARTESIAN_POINT('Ctrl Pts',(-17.1173852570175,27.6827556258494,3.24441359968121));
#60315=CARTESIAN_POINT('Ctrl Pts',(-16.2403199527415,26.5474550953827,2.92755360879577));
#60316=CARTESIAN_POINT('Ctrl Pts',(-16.2970459414564,27.4321275309776,2.61077340535992));
#60317=CARTESIAN_POINT('Ctrl Pts',(-17.2245817678271,27.4866267514743,2.7599832001616));
#60318=CARTESIAN_POINT('Ctrl Pts',(-16.2854701813921,26.4505327273823,2.66574409615585));
#60319=CARTESIAN_POINT('Ctrl Pts',(-16.3329171219314,27.3545890540287,2.37293766614214));
#60320=CARTESIAN_POINT('Ctrl Pts',(-17.272468374468,27.4004735355853,2.51315941724635));
#60321=CARTESIAN_POINT('Ctrl Pts',(-16.3638891417636,26.2837240365077,2.13210289884751));
#60322=CARTESIAN_POINT('Ctrl Pts',(-16.3948333150909,27.2217630392128,1.89119238259305));
#60323=CARTESIAN_POINT('Ctrl Pts',(-17.3556399985759,27.252199143428,2.01006333898577));
#60324=CARTESIAN_POINT('Ctrl Pts',(-16.3971609665106,26.2138347665803,1.86027258862789));
#60325=CARTESIAN_POINT('Ctrl Pts',(-16.4207214647061,27.1668306081169,1.64783726428005));
#60326=CARTESIAN_POINT('Ctrl Pts',(-17.3909282981186,27.1900753483798,1.75379233941467));
#60327=CARTESIAN_POINT('Ctrl Pts',(-16.4372282316227,26.1301157641184,1.44461189527185));
#60328=CARTESIAN_POINT('Ctrl Pts',(-16.4517534962573,27.1012636221844,1.27786031263812));
#60329=CARTESIAN_POINT('Ctrl Pts',(-17.4334238818719,27.1156584568399,1.36192367232642));
#60330=CARTESIAN_POINT('Ctrl Pts',(-16.4489425836071,26.1057357203802,1.30473676381471));
#60331=CARTESIAN_POINT('Ctrl Pts',(-16.4607946572,27.0822242725002,1.15354204459136));
#60332=CARTESIAN_POINT('Ctrl Pts',(-17.4458481948988,27.0939873072066,1.23005486149115));
#60333=CARTESIAN_POINT('Ctrl Pts',(-16.4614235356195,26.0798156556365,1.12817920332052));
#60334=CARTESIAN_POINT('Ctrl Pts',(-16.4704032550175,27.0620254439469,0.997028004066201));
#60335=CARTESIAN_POINT('Ctrl Pts',(-17.4590855680403,27.0709472494042,1.06360328933017));
#60336=CARTESIAN_POINT('Ctrl Pts',(-16.4638105601819,26.074861696503,1.09279299652423));
#60337=CARTESIAN_POINT('Ctrl Pts',(-16.4722410434965,27.0581642796167,0.965648605363661));
#60338=CARTESIAN_POINT('Ctrl Pts',(-17.4616172607913,27.0665437301925,1.03024255564937));
#60339=CARTESIAN_POINT('Ctrl Pts',(-16.4683507346043,26.0654443842168,1.02209528756755));
#60340=CARTESIAN_POINT('Ctrl Pts',(-16.4757345383337,27.0508278725685,0.902983985062077));
#60341=CARTESIAN_POINT('Ctrl Pts',(-17.4664325973152,27.0581727860028,0.963591516895074));
#60342=CARTESIAN_POINT('Ctrl Pts',(-16.470506063436,26.0609765048028,0.986753620408229));
#60343=CARTESIAN_POINT('Ctrl Pts',(-16.4773917386444,27.047349490258,0.871673646590079));
#60344=CARTESIAN_POINT('Ctrl Pts',(-17.4687185521219,27.0542013375728,0.930272773451819));
#60345=CARTESIAN_POINT('Ctrl Pts',(-16.4766286018102,26.0482910800257,0.880750072548012));
#60346=CARTESIAN_POINT('Ctrl Pts',(-16.4820979767805,27.0374753525219,0.777776718980477));
#60347=CARTESIAN_POINT('Ctrl Pts',(-17.4752121534494,27.0429254045267,0.830336768726166));
#60348=CARTESIAN_POINT('Ctrl Pts',(-16.4802523787863,26.0407916272951,0.810109642405695));
#60349=CARTESIAN_POINT('Ctrl Pts',(-16.4848785011,27.0316471633613,0.715279089642234));
#60350=CARTESIAN_POINT('Ctrl Pts',(-17.4790555532451,27.0362592242133,0.763739730217897));
#60351=CARTESIAN_POINT('Ctrl Pts',(-16.4897560121036,26.0211373031105,0.598273404163521));
#60352=CARTESIAN_POINT('Ctrl Pts',(-16.4921690314085,27.0163743171162,0.527896985305773));
#60353=CARTESIAN_POINT('Ctrl Pts',(-17.4891351643784,27.0187887139739,0.564028798530454));
#60354=CARTESIAN_POINT('Ctrl Pts',(-16.4942684087839,26.0118246449525,0.457162601989202));
#60355=CARTESIAN_POINT('Ctrl Pts',(-16.4956179815424,27.0091615199262,0.403342719886046));
#60356=CARTESIAN_POINT('Ctrl Pts',(-17.4939210395996,27.0105107954566,0.430995045648165));
#60357=CARTESIAN_POINT('Ctrl Pts',(-16.4996728834952,26.0006733566253,0.175164846125518));
#60358=CARTESIAN_POINT('Ctrl Pts',(-16.4997511923146,27.0005192273558,0.154469345431858));
#60359=CARTESIAN_POINT('Ctrl Pts',(-17.4996530582721,27.0005985392793,0.165138575470091));
#60360=CARTESIAN_POINT('Ctrl Pts',(-16.5005649496479,25.9988348222276,0.0342778948658427));
#60361=CARTESIAN_POINT('Ctrl Pts',(-16.5004319098763,26.9990972249887,0.0302562756544078));
#60362=CARTESIAN_POINT('Ctrl Pts',(-17.5005991890068,26.9989642864088,0.0323158604794608));
#60363=CARTESIAN_POINT('Ctrl Pts',(-16.4978390182597,26.0044568076987,-0.388049293380772));
#60364=CARTESIAN_POINT('Ctrl Pts',(-16.4983485327184,27.0034518225239,-0.342280149680354));
#60365=CARTESIAN_POINT('Ctrl Pts',(-17.4977080496968,27.0039616068747,-0.365837717665129));
#60366=CARTESIAN_POINT('Ctrl Pts',(-16.4888223219516,26.0230271690527,-0.669156567504712));
#60367=CARTESIAN_POINT('Ctrl Pts',(-16.4914905865413,27.0177691015244,-0.589955966903106));
#60368=CARTESIAN_POINT('Ctrl Pts',(-17.4881448869157,27.020468594845,-0.630854676420441));
#60369=CARTESIAN_POINT('Ctrl Pts',(-16.4645479010849,26.0733210916423,-1.09014697727432));
#60370=CARTESIAN_POINT('Ctrl Pts',(-16.4728185592198,27.0569442887207,-0.963125072170838));
#60371=CARTESIAN_POINT('Ctrl Pts',(-17.4623992890308,27.0651743036164,-1.02774799205062));
#60372=CARTESIAN_POINT('Ctrl Pts',(-16.4546639962014,26.0938323280556,-1.23036518951515));
#60373=CARTESIAN_POINT('Ctrl Pts',(-16.4652151995949,27.0729175749462,-1.08745697835527));
#60374=CARTESIAN_POINT('Ctrl Pts',(-17.4519163596122,27.0834065139337,-1.15994024599047));
#60375=CARTESIAN_POINT('Ctrl Pts',(-16.4400673858426,26.1242298032478,-1.40549624934421));
#60376=CARTESIAN_POINT('Ctrl Pts',(-16.4539221087833,27.0967120128198,-1.2433380557798));
#60377=CARTESIAN_POINT('Ctrl Pts',(-17.4364351061955,27.1104264917492,-1.32504696908299));
#60378=CARTESIAN_POINT('Ctrl Pts',(-16.4370359610415,26.130547367242,-1.44051537232677));
#60379=CARTESIAN_POINT('Ctrl Pts',(-16.4515773822401,27.1016553378582,-1.27449396665141));
#60380=CARTESIAN_POINT('Ctrl Pts',(-17.433219958682,27.1160421042443,-1.35806163047139));
#60381=CARTESIAN_POINT('Ctrl Pts',(-16.4307488113996,26.1436611143959,-1.51053938021269));
#60382=CARTESIAN_POINT('Ctrl Pts',(-16.4467096966894,27.1119250811992,-1.33683413188026));
#60383=CARTESIAN_POINT('Ctrl Pts',(-17.4265517696646,27.1276987683228,-1.42407753017187));
#60384=CARTESIAN_POINT('Ctrl Pts',(-16.4274906111759,26.1504624708553,-1.54556967700777));
#60385=CARTESIAN_POINT('Ctrl Pts',(-16.4441850672634,27.1172550250431,-1.36803947412004));
#60386=CARTESIAN_POINT('Ctrl Pts',(-17.4230961027206,27.1337444184933,-1.45710272580348));
#60387=CARTESIAN_POINT('Ctrl Pts',(-16.4173982522689,26.1715491252668,-1.65044486531198));
#60388=CARTESIAN_POINT('Ctrl Pts',(-16.43635996178,27.1337879226008,-1.46149208806462));
#60389=CARTESIAN_POINT('Ctrl Pts',(-17.4123920858232,27.1524881114378,-1.55597495718666));
#60390=CARTESIAN_POINT('Ctrl Pts',(-16.4102542800575,26.186500310749,-1.72000002026246));
#60391=CARTESIAN_POINT('Ctrl Pts',(-16.4308099461936,27.1455302764211,-1.52357398570511));
#60392=CARTESIAN_POINT('Ctrl Pts',(-17.4048151454351,27.1657780539216,-1.62154884066042));
#60393=CARTESIAN_POINT('Ctrl Pts',(-16.3725127956242,26.2656547133766,-2.06599962503883));
#60394=CARTESIAN_POINT('Ctrl Pts',(-16.4014953816007,27.2076634406906,-1.83207874075241));
#60395=CARTESIAN_POINT('Ctrl Pts',(-17.3647862987107,27.2361375233113,-1.94774375420961));
#60396=CARTESIAN_POINT('Ctrl Pts',(-16.3358579567688,26.3430155684638,-2.33712916293811));
#60397=CARTESIAN_POINT('Ctrl Pts',(-16.3728357498743,27.2687196259979,-2.07564354115728));
#60398=CARTESIAN_POINT('Ctrl Pts',(-17.3259099538696,27.3049027273893,-2.20335409300917));
#60399=CARTESIAN_POINT('Ctrl Pts',(-16.2509489421038,26.5246876648651,-2.86863842077008));
#60400=CARTESIAN_POINT('Ctrl Pts',(-16.3054421715168,27.4140279801895,-2.55725670467926));
#60401=CARTESIAN_POINT('Ctrl Pts',(-17.2358549388741,27.4663890355697,-2.70444026200191));
#60402=CARTESIAN_POINT('Ctrl Pts',(-16.2026914231958,26.6290018643058,-3.12901661081332));
#60403=CARTESIAN_POINT('Ctrl Pts',(-16.2668736654531,27.4979009908363,-2.79478543759917));
#60404=CARTESIAN_POINT('Ctrl Pts',(-17.1846727213246,27.5591127682956,-2.94991464986886));
#60405=CARTESIAN_POINT('Ctrl Pts',(-16.1224929527533,26.8055233058917,-3.511724585575));
#60406=CARTESIAN_POINT('Ctrl Pts',(-16.2015927972012,27.6422088112504,-3.14811650491222));
#60407=CARTESIAN_POINT('Ctrl Pts',(-17.099613737892,27.7160207163362,-3.31071678104154));
#60408=CARTESIAN_POINT('Ctrl Pts',(-16.0944573592689,26.8677122005455,-3.6379817080266));
#60409=CARTESIAN_POINT('Ctrl Pts',(-16.1787224577041,27.6931119961222,-3.2648130549793));
#60410=CARTESIAN_POINT('Ctrl Pts',(-17.0698790172897,27.7712997338665,-3.42974706475798));
#60411=CARTESIAN_POINT('Ctrl Pts',(-16.0578742587549,26.9496675749635,-3.79416704657873));
#60412=CARTESIAN_POINT('Ctrl Pts',(-16.1486081613594,27.7607465434304,-3.4101345555538));
#60413=CARTESIAN_POINT('Ctrl Pts',(-17.0310787593147,27.844148955511,-3.57699250183713));
#60414=CARTESIAN_POINT('Ctrl Pts',(-16.0504807062728,26.9662697489414,-3.82532226629593));
#60415=CARTESIAN_POINT('Ctrl Pts',(-16.1425271619055,27.7744328577361,-3.43908652601369));
#60416=CARTESIAN_POINT('Ctrl Pts',(-17.0232371126848,27.8589064435178,-3.60636442612413));
#60417=CARTESIAN_POINT('Ctrl Pts',(-16.0355419811776,26.999897690748,-3.88746893406826));
#60418=CARTESIAN_POINT('Ctrl Pts',(-16.1302215604399,27.8021911773562,-3.49689960574396));
#60419=CARTESIAN_POINT('Ctrl Pts',(-17.0073930103687,27.8887979473173,-3.66495387724952));
#60420=CARTESIAN_POINT('Ctrl Pts',(-16.0279925473271,27.0169331053863,-3.91847760489801));
#60421=CARTESIAN_POINT('Ctrl Pts',(-16.1239938076285,27.8162702352096,-3.52577621154247));
#60422=CARTESIAN_POINT('Ctrl Pts',(-16.9993860349865,27.9039405380826,-3.69418764098899));
#60423=CARTESIAN_POINT('Ctrl Pts',(-16.005151309949,27.0686067279126,-4.01113187201297));
#60424=CARTESIAN_POINT('Ctrl Pts',(-16.1051372201557,27.8589989859183,-3.61208369701427));
#60425=CARTESIAN_POINT('Ctrl Pts',(-16.9751604803637,27.9498726471105,-3.78153846518201));
#60426=CARTESIAN_POINT('Ctrl Pts',(-15.9896858552224,27.1037684311926,-4.07232971282369));
#60427=CARTESIAN_POINT('Ctrl Pts',(-16.0923233519077,27.8881659099294,-3.66925480659103));
#60428=CARTESIAN_POINT('Ctrl Pts',(-16.9587577251248,27.9811274943278,-3.8392333993061));
#60429=CARTESIAN_POINT('Ctrl Pts',(-15.9112419315778,27.2830923847797,-4.37551697666845));
#60430=CARTESIAN_POINT('Ctrl Pts',(-16.0274373719239,28.0366047023604,-3.95173322375266));
#60431=CARTESIAN_POINT('Ctrl Pts',(-16.875559624845,28.1405265645112,-4.1250665099463));
#60432=CARTESIAN_POINT('Ctrl Pts',(-15.844918315659,27.4377681716844,-4.60912492170408));
#60433=CARTESIAN_POINT('Ctrl Pts',(-15.9717543805869,28.166270657865,-4.1723242724571));
#60434=CARTESIAN_POINT('Ctrl Pts',(-16.8052163950039,28.2780161525077,-4.34530295645177));
#60435=CARTESIAN_POINT('Ctrl Pts',(-15.7069099448858,27.7688775711428,-5.05949097805553));
#60436=CARTESIAN_POINT('Ctrl Pts',(-15.8543812193166,28.447094636339,-4.60083479731583));
#60437=CARTESIAN_POINT('Ctrl Pts',(-16.6588438813315,28.5723356188943,-4.76989048439904));
#60438=CARTESIAN_POINT('Ctrl Pts',(-15.6352206245408,27.9453128342832,-5.27624649105232));
#60439=CARTESIAN_POINT('Ctrl Pts',(-15.7928000382307,28.5978883814961,-4.80878789175796));
#60440=CARTESIAN_POINT('Ctrl Pts',(-16.5828097529458,28.7291669638434,-4.97423911600232));
#60441=CARTESIAN_POINT('Ctrl Pts',(-15.5249581839362,28.2263776622186,-5.58908746041189));
#60442=CARTESIAN_POINT('Ctrl Pts',(-15.696693052097,28.8413995443161,-5.11191611245));
#60443=CARTESIAN_POINT('Ctrl Pts',(-16.4658647407159,28.9790023663985,-5.26917336342192));
#60444=CARTESIAN_POINT('Ctrl Pts',(-15.4877493740823,28.3228072898136,-5.69131489459601));
#60445=CARTESIAN_POINT('Ctrl Pts',(-15.6642132176884,28.9249883773396,-5.21099932125141));
#60446=CARTESIAN_POINT('Ctrl Pts',(-16.4264008511294,29.0647175909937,-5.36554939547687));
#60447=CARTESIAN_POINT('Ctrl Pts',(-15.431421554897,28.4716312472057,-5.84158285664235));
#60448=CARTESIAN_POINT('Ctrl Pts',(-15.6147184969787,29.0547764285091,-5.3573483822539));
#60449=CARTESIAN_POINT('Ctrl Pts',(-16.3666592249758,29.1970055530476,-5.50721616119523));
#60450=CARTESIAN_POINT('Ctrl Pts',(-15.4125599052749,28.5219362190851,-5.8911597188493));
#60451=CARTESIAN_POINT('Ctrl Pts',(-15.5981338876659,29.098657869549,-5.40563341726845));
#60452=CARTESIAN_POINT('Ctrl Pts',(-16.3466544449051,29.2417210836625,-5.55395529043817));
#60453=CARTESIAN_POINT('Ctrl Pts',(-15.3841604516061,28.5984513320056,-5.9647546987206));
#60454=CARTESIAN_POINT('Ctrl Pts',(-15.5730837024597,29.1655935118162,-5.47748185994016));
#60455=CARTESIAN_POINT('Ctrl Pts',(-16.3165338123512,29.3097345173226,-5.62333776313334));
#60456=CARTESIAN_POINT('Ctrl Pts',(-15.3746761425149,28.6241326720875,-5.98915795629746));
#60457=CARTESIAN_POINT('Ctrl Pts',(-15.5647153050045,29.1880623175047,-5.50130549482725));
#60458=CARTESIAN_POINT('Ctrl Pts',(-16.3064746965653,29.3325623752064,-5.64634420119125));
#60459=CARTESIAN_POINT('Ctrl Pts',(-15.3556755438085,28.6758503150148,-6.03770718948676));
#60460=CARTESIAN_POINT('Ctrl Pts',(-15.547931168814,29.2333546452359,-5.54873830674073));
#60461=CARTESIAN_POINT('Ctrl Pts',(-16.2863225465049,29.3785336133291,-5.69211452210701));
#60462=CARTESIAN_POINT('Ctrl Pts',(-15.3461631123057,28.7018763061624,-6.06184308744346));
#60463=CARTESIAN_POINT('Ctrl Pts',(-15.5395188506324,29.2561687234751,-5.57233816417615));
#60464=CARTESIAN_POINT('Ctrl Pts',(-16.2762336039025,29.4016678276794,-5.71486890398771));
#60465=CARTESIAN_POINT('Ctrl Pts',(-15.2606323097608,28.9371409426806,-6.27738721348527));
#60466=CARTESIAN_POINT('Ctrl Pts',(-15.4642290688267,29.4614132947124,-5.7820464495127));
#60467=CARTESIAN_POINT('Ctrl Pts',(-16.1855191168777,29.610791949213,-5.918075487456));
#60468=CARTESIAN_POINT('Ctrl Pts',(-15.1848342114096,29.1545099575102,-6.45796308382094));
#60469=CARTESIAN_POINT('Ctrl Pts',(-15.3964943458008,29.6534800554759,-5.96008229317087));
#60470=CARTESIAN_POINT('Ctrl Pts',(-16.1051271935059,29.8040088510832,-6.08831536510389));
#60471=CARTESIAN_POINT('Ctrl Pts',(-15.0356595911467,29.6056859311573,-6.79804515130241));
#60472=CARTESIAN_POINT('Ctrl Pts',(-15.2622391988625,30.0548640664217,-6.29665836970821));
#60473=CARTESIAN_POINT('Ctrl Pts',(-15.9469116879931,30.2050541610657,-6.40893145588782));
#60474=CARTESIAN_POINT('Ctrl Pts',(-14.9622788975724,29.8394929473934,-6.95754936214554));
#60475=CARTESIAN_POINT('Ctrl Pts',(-15.1956484255345,30.2641311892708,-6.45556673433959));
#60476=CARTESIAN_POINT('Ctrl Pts',(-15.8690836788716,30.4128826199675,-6.55930579570915));
#60477=CARTESIAN_POINT('Ctrl Pts',(-14.8199953655875,30.3240935251076,-7.25568882321979));
#60478=CARTESIAN_POINT('Ctrl Pts',(-15.0658271140403,30.7002416979089,-6.75341440551023));
#60479=CARTESIAN_POINT('Ctrl Pts',(-15.7181769032676,30.8436386889222,-6.8403800356117));
#60480=CARTESIAN_POINT('Ctrl Pts',(-14.7510880041712,30.5748839284072,-7.39432626488165));
#60481=CARTESIAN_POINT('Ctrl Pts',(-15.0024895581545,30.9271154442475,-6.89273010331883));
#60482=CARTESIAN_POINT('Ctrl Pts',(-15.645093337422,31.0665634920556,-6.9710820001448));
#60483=CARTESIAN_POINT('Ctrl Pts',(-14.6691811405517,30.8997312170887,-7.55423164883944));
#60484=CARTESIAN_POINT('Ctrl Pts',(-14.9266314159884,31.2233129771628,-7.0542966399533));
#60485=CARTESIAN_POINT('Ctrl Pts',(-15.5582224218811,31.3553166373777,-7.12183455119867));
#60486=CARTESIAN_POINT('Ctrl Pts',(-14.653011891398,30.9652703749227,-7.5855411589654));
#60487=CARTESIAN_POINT('Ctrl Pts',(-14.9116910431975,31.2829158941087,-7.08584557342882));
#60488=CARTESIAN_POINT('Ctrl Pts',(-15.5410732180678,31.4135736666364,-7.15135193426238));
#60489=CARTESIAN_POINT('Ctrl Pts',(-14.6291056146706,31.0644531496729,-7.63148523917637));
#60490=CARTESIAN_POINT('Ctrl Pts',(-14.8895640652671,31.3732579073334,-7.13220066227062));
#60491=CARTESIAN_POINT('Ctrl Pts',(-15.5157180762066,31.5017361330234,-7.19466621881002));
#60492=CARTESIAN_POINT('Ctrl Pts',(-14.6211948006132,31.0976597721854,-7.64662987407586));
#60493=CARTESIAN_POINT('Ctrl Pts',(-14.8822417942904,31.4035020137527,-7.14747837210504));
#60494=CARTESIAN_POINT('Ctrl Pts',(-15.507327818792,31.5312531308516,-7.20894398896686));
#60495=CARTESIAN_POINT('Ctrl Pts',(-14.6054941177937,31.1643679687753,-7.67657654190212));
#60496=CARTESIAN_POINT('Ctrl Pts',(-14.867701061467,31.4642882513809,-7.17769919573129));
#60497=CARTESIAN_POINT('Ctrl Pts',(-15.4906755795184,31.5905493055579,-7.23717653788107));
#60498=CARTESIAN_POINT('Ctrl Pts',(-14.5977025585871,31.1978776275757,-7.69138168422876));
#60499=CARTESIAN_POINT('Ctrl Pts',(-14.8604807256331,31.4948381920921,-7.19264621846369));
#60500=CARTESIAN_POINT('Ctrl Pts',(-15.4824118045141,31.6203356689469,-7.2511342477555));
#60501=CARTESIAN_POINT('Ctrl Pts',(-14.5591761411658,31.3656598443161,-7.76432516797013));
#60502=CARTESIAN_POINT('Ctrl Pts',(-14.8248199038901,31.6476138839898,-7.26619003874707));
#60503=CARTESIAN_POINT('Ctrl Pts',(-15.4415504529436,31.7694754172071,-7.31990251526702));
#60504=CARTESIAN_POINT('Ctrl Pts',(-14.5296413627691,31.5010285289678,-7.81939903927279));
#60505=CARTESIAN_POINT('Ctrl Pts',(-14.7973600530408,31.7713364293414,-7.32192638233487));
#60506=CARTESIAN_POINT('Ctrl Pts',(-15.4102256876126,31.8898031368429,-7.37182401004875));
#60507=CARTESIAN_POINT('Ctrl Pts',(-14.4452230147646,31.9105732769504,-7.97492632680715));
#60508=CARTESIAN_POINT('Ctrl Pts',(-14.7189160078809,32.1454427835541,-7.47912726165049));
#60509=CARTESIAN_POINT('Ctrl Pts',(-15.3206910766111,32.2538429128796,-7.51844906238992));
#60510=CARTESIAN_POINT('Ctrl Pts',(-14.394524204208,32.1881803100535,-8.06571177616595));
#60511=CARTESIAN_POINT('Ctrl Pts',(-14.6714240271853,32.4005576020766,-7.57152225977134));
#60512=CARTESIAN_POINT('Ctrl Pts',(-15.266919610253,32.5006047200686,-7.60403803792814));
#60513=CARTESIAN_POINT('Ctrl Pts',(-14.3060495457409,32.7527931145422,-8.22161662427291));
#60514=CARTESIAN_POINT('Ctrl Pts',(-14.5884881552083,32.9202575071458,-7.73013444004218));
#60515=CARTESIAN_POINT('Ctrl Pts',(-15.1730828518141,33.0024827684609,-7.75101903992668));
#60516=CARTESIAN_POINT('Ctrl Pts',(-14.2682728616157,33.0397984670644,-8.2867370209155));
#60517=CARTESIAN_POINT('Ctrl Pts',(-14.552893734404,33.1852802024212,-7.79666355226168));
#60518=CARTESIAN_POINT('Ctrl Pts',(-15.133016671222,33.2575986374368,-7.81241200590781));
#60519=CARTESIAN_POINT('Ctrl Pts',(-14.2226573712228,33.4777284594361,-8.36462327469889));
#60520=CARTESIAN_POINT('Ctrl Pts',(-14.5098903723144,33.5903491926421,-7.87622892641895));
#60521=CARTESIAN_POINT('Ctrl Pts',(-15.0846366059366,33.6468697416979,-7.8858401244665));
#60522=CARTESIAN_POINT('Ctrl Pts',(-14.2092942502116,33.6249441231039,-8.38727953342513));
#60523=CARTESIAN_POINT('Ctrl Pts',(-14.4972860759252,33.7265132279608,-7.8993776669338));
#60524=CARTESIAN_POINT('Ctrl Pts',(-15.0704635986376,33.7777281094489,-7.90719955992493));
#60525=CARTESIAN_POINT('Ctrl Pts',(-14.1921874059586,33.8476922922332,-8.41617145140093));
#60526=CARTESIAN_POINT('Ctrl Pts',(-14.4811437317631,33.9326839034157,-7.92890420892895));
#60527=CARTESIAN_POINT('Ctrl Pts',(-15.0523199760526,33.9757264819735,-7.93443773206372));
#60528=CARTESIAN_POINT('Ctrl Pts',(-14.1869748028688,33.9222626039221,-8.42495286656801));
#60529=CARTESIAN_POINT('Ctrl Pts',(-14.4762244556026,34.0017015413618,-7.93787844712968));
#60530=CARTESIAN_POINT('Ctrl Pts',(-15.0467914575584,34.0420112034973,-7.94271650708992));
#60531=CARTESIAN_POINT('Ctrl Pts',(-14.1799126492618,34.0346090885612,-8.43682988299433));
#60532=CARTESIAN_POINT('Ctrl Pts',(-14.4695579078732,34.105716008113,-7.95001849700854));
#60533=CARTESIAN_POINT('Ctrl Pts',(-15.0393012946864,34.1418747453823,-7.95391369446155));
#60534=CARTESIAN_POINT('Ctrl Pts',(-14.1776847259483,34.0721397627187,-8.44057300476486));
#60535=CARTESIAN_POINT('Ctrl Pts',(-14.4674547435269,34.1404623010022,-7.9538444086756));
#60536=CARTESIAN_POINT('Ctrl Pts',(-15.0369383456894,34.1752353446439,-7.95744256335628));
#60537=CARTESIAN_POINT('Ctrl Pts',(-14.1745348393834,34.1285598388531,-8.44586089729133));
#60538=CARTESIAN_POINT('Ctrl Pts',(-14.4644807945682,34.192704719503,-7.95924986164786));
#60539=CARTESIAN_POINT('Ctrl Pts',(-15.0335975569284,34.2253865234225,-7.96242778198736));
#60540=CARTESIAN_POINT('Ctrl Pts',(-14.173516877044,34.1473872089809,-8.4475690610768));
#60541=CARTESIAN_POINT('Ctrl Pts',(-14.4635196895548,34.2101377324663,-7.96099596612494));
#60542=CARTESIAN_POINT('Ctrl Pts',(-15.0325178998889,34.242121963541,-7.96403817202918));
#60543=CARTESIAN_POINT('Ctrl Pts',(-14.1720382860565,34.1756594493329,-8.45004921553296));
#60544=CARTESIAN_POINT('Ctrl Pts',(-14.4621235724204,34.2363181267017,-7.96353136267135));
#60545=CARTESIAN_POINT('Ctrl Pts',(-15.0309496973357,34.2672528438503,-7.96637636482709));
#60546=CARTESIAN_POINT('Ctrl Pts',(-14.171553481119,34.1850887269927,-8.45086225174429));
#60547=CARTESIAN_POINT('Ctrl Pts',(-14.4616658100524,34.2450496654721,-7.96436249848284));
#60548=CARTESIAN_POINT('Ctrl Pts',(-15.0304355102747,34.2756344239947,-7.96714286358229));
#60549=CARTESIAN_POINT('Ctrl Pts',(-14.1706000477243,34.2039577059635,-8.45246089334986));
#60550=CARTESIAN_POINT('Ctrl Pts',(-14.4607655369268,34.2625227778338,-7.96599675441144));
#60551=CARTESIAN_POINT('Ctrl Pts',(-15.029424293044,34.2924068497441,-7.96865000047954));
#60552=CARTESIAN_POINT('Ctrl Pts',(-14.1701308662489,34.2134087629436,-8.45324742565082));
#60553=CARTESIAN_POINT('Ctrl Pts',(-14.4603225019436,34.2712748866038,-7.96680082574036));
#60554=CARTESIAN_POINT('Ctrl Pts',(-15.028926676316,34.3008077891872,-7.96939151350123));
#60555=CARTESIAN_POINT('Ctrl Pts',(-14.1696709084508,34.2228423347593,-8.45401835497186));
#60556=CARTESIAN_POINT('Ctrl Pts',(-14.4598881528388,34.2800112558736,-7.96758898230353));
#60557=CARTESIAN_POINT('Ctrl Pts',(-15.0284388422964,34.3091931864527,-7.97011831445158));
#60558=CARTESIAN_POINT('Ctrl Pts',(-6.,40.2323075626015,-16.7705098312484));
#60559=CARTESIAN_POINT('Ctrl Pts',(-6.,40.2323075626015,-15.4288690447485));
#60560=CARTESIAN_POINT('Ctrl Pts',(-4.71428571428571,40.2323075626015,-15.8121949837485));
#60561=CARTESIAN_POINT('Ctrl Pts',(-6.,40.2152831433091,-16.7705098300439));
#60562=CARTESIAN_POINT('Ctrl Pts',(-5.99999999918455,40.2289031540789,-15.4288690446538));
#60563=CARTESIAN_POINT('Ctrl Pts',(-4.71428571810276,40.1812343046596,-15.8121949826105));
#60564=CARTESIAN_POINT('Ctrl Pts',(-6.00086709959613,40.1984135664914,-16.7697348999033));
#60565=CARTESIAN_POINT('Ctrl Pts',(-5.99947691569071,40.2255290821746,-15.4288072509424));
#60566=CARTESIAN_POINT('Ctrl Pts',(-4.71673836819782,40.1306255743571,-15.8114643341001));
#60567=CARTESIAN_POINT('Ctrl Pts',(-6.00426966178499,40.1649734181343,-16.7666864482411));
#60568=CARTESIAN_POINT('Ctrl Pts',(-5.99746228399819,40.218435826368,-15.4285622514261));
#60569=CARTESIAN_POINT('Ctrl Pts',(-4.72636275685162,40.0303051291139,-15.8085900798646));
#60570=CARTESIAN_POINT('Ctrl Pts',(-6.00680532946631,40.1484027206558,-16.7644127338286));
#60571=CARTESIAN_POINT('Ctrl Pts',(-5.99597239391959,40.2147209114066,-15.4283793290426));
#60572=CARTESIAN_POINT('Ctrl Pts',(-4.7335350744668,39.980593036709,-15.8064462917098));
#60573=CARTESIAN_POINT('Ctrl Pts',(-6.01353255271329,40.1155581374418,-16.7583557139617));
#60574=CARTESIAN_POINT('Ctrl Pts',(-5.99214798696173,40.2065622671074,-15.4278851619237));
#60575=CARTESIAN_POINT('Ctrl Pts',(-4.75256350655548,39.8820592871776,-15.8007353876353));
#60576=CARTESIAN_POINT('Ctrl Pts',(-6.01772404886921,40.0992842400478,-16.7545725300023));
#60577=CARTESIAN_POINT('Ctrl Pts',(-5.98981636127134,40.202124845771,-15.4275745721604));
#60578=CARTESIAN_POINT('Ctrl Pts',(-4.76441945116622,39.8332375945207,-15.7971683851509));
#60579=CARTESIAN_POINT('Ctrl Pts',(-6.0240219807572,40.0791319892091,-16.74885556262));
#60580=CARTESIAN_POINT('Ctrl Pts',(-5.98648250852101,40.1958724239871,-15.4270937726593));
#60581=CARTESIAN_POINT('Ctrl Pts',(-4.78223360305063,39.7727808425291,-15.7917781019688));
#60582=CARTESIAN_POINT('Ctrl Pts',(-6.02533572392216,40.0751078557388,-16.7476616129027));
#60583=CARTESIAN_POINT('Ctrl Pts',(-5.98579543217186,40.1945875299876,-15.4269930200015));
#60584=CARTESIAN_POINT('Ctrl Pts',(-4.78594961957438,39.7607084421942,-15.7906523778123));
#60585=CARTESIAN_POINT('Ctrl Pts',(-6.02806562891379,40.0670929379168,-16.7451772260115));
#60586=CARTESIAN_POINT('Ctrl Pts',(-5.98438622375446,40.191946424886,-15.4267821748928));
#60587=CARTESIAN_POINT('Ctrl Pts',(-4.79367134987588,39.7366636883665,-15.7883099560211));
#60588=CARTESIAN_POINT('Ctrl Pts',(-6.0294779907155,40.0631130239638,-16.7438902481684));
#60589=CARTESIAN_POINT('Ctrl Pts',(-5.98366611306037,40.1905939935738,-15.4266723903639));
#60590=CARTESIAN_POINT('Ctrl Pts',(-4.79766631700306,39.7247239468563,-15.78709651963));
#60591=CARTESIAN_POINT('Ctrl Pts',(-6.03385527087601,40.051254796774,-16.739895758248));
#60592=CARTESIAN_POINT('Ctrl Pts',(-5.98146696546189,40.1864358470219,-15.4263296304894));
#60593=CARTESIAN_POINT('Ctrl Pts',(-4.81004776537665,39.6891492647827,-15.7833302864913));
#60594=CARTESIAN_POINT('Ctrl Pts',(-6.03696028948911,40.0434579430007,-16.7370547926887));
#60595=CARTESIAN_POINT('Ctrl Pts',(-5.97994756331896,40.1835265738621,-15.426083083921));
#60596=CARTESIAN_POINT('Ctrl Pts',(-4.81883053366853,39.6657587040667,-15.7806516615182));
#60597=CARTESIAN_POINT('Ctrl Pts',(-6.04682316560899,40.0203864307978,-16.7280004451824));
#60598=CARTESIAN_POINT('Ctrl Pts',(-5.97529225782466,40.1743463310241,-15.4252854635617));
#60599=CARTESIAN_POINT('Ctrl Pts',(-4.84672838163821,39.5965441666547,-15.7721147057772));
#60600=CARTESIAN_POINT('Ctrl Pts',(-6.05412752167962,40.0054300386619,-16.7212571411063));
#60601=CARTESIAN_POINT('Ctrl Pts',(-5.97205156506919,40.1676130008118,-15.4246764580379));
#60602=CARTESIAN_POINT('Ctrl Pts',(-4.86738927571349,39.551674990914,-15.7657567326582));
#60603=CARTESIAN_POINT('Ctrl Pts',(-6.07016106549893,39.9763502064277,-16.7063311041315));
#60604=CARTESIAN_POINT('Ctrl Pts',(-5.9656350667376,40.1526685017272,-15.4232639946225));
#60605=CARTESIAN_POINT('Ctrl Pts',(-4.91274129944868,39.4644354939485,-15.7516836128517));
#60606=CARTESIAN_POINT('Ctrl Pts',(-6.07889031425637,39.9622267963988,-16.698148412995));
#60607=CARTESIAN_POINT('Ctrl Pts',(-5.96246129227807,40.1444721129303,-15.422462446856));
#60608=CARTESIAN_POINT('Ctrl Pts',(-4.93743260243233,39.4220652635496,-15.7439685032292));
#60609=CARTESIAN_POINT('Ctrl Pts',(-6.09069779316276,39.9450985529772,-16.6869735595439));
#60610=CARTESIAN_POINT('Ctrl Pts',(-5.95877416318781,40.1331449703773,-15.4212977072095));
#60611=CARTESIAN_POINT('Ctrl Pts',(-4.97083090084792,39.3706805338393,-15.7334322133972));
#60612=CARTESIAN_POINT('Ctrl Pts',(-6.09310418619124,39.9416992657338,-16.6846911400641));
#60613=CARTESIAN_POINT('Ctrl Pts',(-5.9580529547782,40.1308323519191,-15.4210572678978));
#60614=CARTESIAN_POINT('Ctrl Pts',(-4.97763755498991,39.3604826718443,-15.7312802176574));
#60615=CARTESIAN_POINT('Ctrl Pts',(-6.09800731088457,39.934953794505,-16.680029715004));
#60616=CARTESIAN_POINT('Ctrl Pts',(-5.95664664771447,40.1260992628088,-15.420559060673));
#60617=CARTESIAN_POINT('Ctrl Pts',(-4.99150639388168,39.3402462584659,-15.7268851599783));
#60618=CARTESIAN_POINT('Ctrl Pts',(-6.10050726882805,39.931603434497,-16.6776476264958));
#60619=CARTESIAN_POINT('Ctrl Pts',(-5.95596070720442,40.1236759648656,-15.4203009955482));
#60620=CARTESIAN_POINT('Ctrl Pts',(-4.99857770366056,39.3301951786403,-15.7246391906029));
#60621=CARTESIAN_POINT('Ctrl Pts',(-6.10811946799149,39.9216641845842,-16.670376806369));
#60622=CARTESIAN_POINT('Ctrl Pts',(-5.95397565819811,40.1162694017168,-15.419501917334));
#60623=CARTESIAN_POINT('Ctrl Pts',(-5.0201093515106,39.3003774278449,-15.7177838461912));
#60624=CARTESIAN_POINT('Ctrl Pts',(-6.11333262437216,39.915200818976,-16.6653744832296));
#60625=CARTESIAN_POINT('Ctrl Pts',(-5.95274853351578,40.1111506689315,-15.4189363070628));
#60626=CARTESIAN_POINT('Ctrl Pts',(-5.03485513807882,39.2809873322929,-15.7130673697086));
#60627=CARTESIAN_POINT('Ctrl Pts',(-6.1293748326009,39.8962861790546,-16.6499024080798));
#60628=CARTESIAN_POINT('Ctrl Pts',(-5.94943970565223,40.0952810454962,-15.4171310107049));
#60629=CARTESIAN_POINT('Ctrl Pts',(-5.08023166821929,39.2242434108254,-15.6984794137196));
#60630=CARTESIAN_POINT('Ctrl Pts',(-6.1406056663782,39.884309238974,-16.6389685998647));
#60631=CARTESIAN_POINT('Ctrl Pts',(-5.94771464892963,40.0839766925516,-15.4157800254322));
#60632=CARTESIAN_POINT('Ctrl Pts',(-5.11199888523177,39.1883125922345,-15.6881703937412));
#60633=CARTESIAN_POINT('Ctrl Pts',(-6.16409905708717,39.8615816843069,-16.6158372464421));
#60634=CARTESIAN_POINT('Ctrl Pts',(-5.94564861891527,40.0599452805169,-15.4126949205069));
#60635=CARTESIAN_POINT('Ctrl Pts',(-5.17845161828455,39.1201299272022,-15.6663608327766));
#60636=CARTESIAN_POINT('Ctrl Pts',(-6.17636172059827,39.8508311824304,-16.6036396930356));
#60637=CARTESIAN_POINT('Ctrl Pts',(-5.94529765421637,40.0472399899623,-15.4109653218148));
#60638=CARTESIAN_POINT('Ctrl Pts',(-5.21313743796322,39.0878784218881,-15.6548602815568));
#60639=CARTESIAN_POINT('Ctrl Pts',(-6.19552162464795,39.8356220321449,-16.5843510979584));
#60640=CARTESIAN_POINT('Ctrl Pts',(-5.94612875976558,40.0271363620363,-15.4079956032292));
#60641=CARTESIAN_POINT('Ctrl Pts',(-5.26733259558317,39.0422509713317,-15.6366738925849));
#60642=CARTESIAN_POINT('Ctrl Pts',(-6.20203613099305,39.8307053430792,-16.5777559291836));
#60643=CARTESIAN_POINT('Ctrl Pts',(-5.94662867798683,40.0202869469601,-15.4069471500247));
#60644=CARTESIAN_POINT('Ctrl Pts',(-5.28575934167097,39.0275009037357,-15.6304555901406));
#60645=CARTESIAN_POINT('Ctrl Pts',(-6.21200068125232,39.8235618043476,-16.567606697845));
#60646=CARTESIAN_POINT('Ctrl Pts',(-5.94775936498885,40.0097653187781,-15.4052685020573));
#60647=CARTESIAN_POINT('Ctrl Pts',(-5.31394478425411,39.0060702879891,-15.6208863152272));
#60648=CARTESIAN_POINT('Ctrl Pts',(-6.21535764108576,39.8212169930998,-16.5641774763452));
#60649=CARTESIAN_POINT('Ctrl Pts',(-5.9481991858846,40.0062198151304,-15.4046917890623));
#60650=CARTESIAN_POINT('Ctrl Pts',(-5.32344018506321,38.9990358545671,-15.6176530490547));
#60651=CARTESIAN_POINT('Ctrl Pts',(-6.22212086912811,39.8166154680804,-16.5572476494714));
#60652=CARTESIAN_POINT('Ctrl Pts',(-5.94920983527497,39.9990692704025,-15.4035042743602));
#60653=CARTESIAN_POINT('Ctrl Pts',(-5.34257045811315,38.9852312785673,-15.6111192124296));
#60654=CARTESIAN_POINT('Ctrl Pts',(-6.22552135620163,39.8143625551259,-16.5537529884858));
#60655=CARTESIAN_POINT('Ctrl Pts',(-5.94977935255954,39.9954706760488,-15.4028946209305));
#60656=CARTESIAN_POINT('Ctrl Pts',(-5.35218897920305,38.9784725405973,-15.6078242462156));
#60657=CARTESIAN_POINT('Ctrl Pts',(-6.24261647292014,39.8033336673682,-16.5361308383412));
#60658=CARTESIAN_POINT('Ctrl Pts',(-5.95294841354305,39.9774321071524,-15.3997736035282));
#60659=CARTESIAN_POINT('Ctrl Pts',(-5.4005437367575,38.9453858752107,-15.5912090764345));
#60660=CARTESIAN_POINT('Ctrl Pts',(-6.25658842504356,39.7952630018719,-16.5215575392438));
#60661=CARTESIAN_POINT('Ctrl Pts',(-5.95654259008027,39.9626139216758,-15.3970056111323));
#60662=CARTESIAN_POINT('Ctrl Pts',(-5.44006440260921,38.9211738813271,-15.5774685367124));
#60663=CARTESIAN_POINT('Ctrl Pts',(-6.28509305730017,39.7805641079001,-16.4914450749466));
#60664=CARTESIAN_POINT('Ctrl Pts',(-5.96611579674779,39.9325466076702,-15.3908337573467));
#60665=CARTESIAN_POINT('Ctrl Pts',(-5.52069179030617,38.8770771975832,-15.5490767852386));
#60666=CARTESIAN_POINT('Ctrl Pts',(-6.29962582233355,39.7739360664052,-16.4759058887031));
#60667=CARTESIAN_POINT('Ctrl Pts',(-5.97206780921745,39.917312384644,-15.3874384220071));
#60668=CARTESIAN_POINT('Ctrl Pts',(-5.56179875453699,38.8571930741266,-15.5344255519103));
#60669=CARTESIAN_POINT('Ctrl Pts',(-6.32923798954882,39.7621006130703,-16.4438289832851));
#60670=CARTESIAN_POINT('Ctrl Pts',(-5.98657812285022,39.8867276348292,-15.3799070345543));
#60671=CARTESIAN_POINT('Ctrl Pts',(-5.64555888478752,38.8216867138941,-15.5041816131072));
#60672=CARTESIAN_POINT('Ctrl Pts',(-6.34431740281587,39.7568932093963,-16.427291325653));
#60673=CARTESIAN_POINT('Ctrl Pts',(-5.99510387590282,39.8713890796003,-15.3757815092243));
#60674=CARTESIAN_POINT('Ctrl Pts',(-5.68821208193698,38.8060645022573,-15.4885889638827));
#60675=CARTESIAN_POINT('Ctrl Pts',(-6.36350899238667,39.7512813707633,-16.4059633038224));
#60676=CARTESIAN_POINT('Ctrl Pts',(-6.00757171375912,39.8522872563196,-15.3700673381977));
#60677=CARTESIAN_POINT('Ctrl Pts',(-5.74249686425784,38.7892289872689,-15.4684796865372));
#60678=CARTESIAN_POINT('Ctrl Pts',(-6.36736640469525,39.7502035609108,-16.4016626515698));
#60679=CARTESIAN_POINT('Ctrl Pts',(-6.01014306585411,39.8484887840959,-15.368902314736));
#60680=CARTESIAN_POINT('Ctrl Pts',(-5.75340783051444,38.7859955579257,-15.464424785742));
#60681=CARTESIAN_POINT('Ctrl Pts',(-6.37508178304079,39.7481470746211,-16.393032726381));
#60682=CARTESIAN_POINT('Ctrl Pts',(-6.01543918049613,39.8409465314235,-15.3665281828108));
#60683=CARTESIAN_POINT('Ctrl Pts',(-5.77523132908179,38.7798260982638,-15.456287999183));
#60684=CARTESIAN_POINT('Ctrl Pts',(-6.37894373953493,39.7471671729223,-16.3886990350584));
#60685=CARTESIAN_POINT('Ctrl Pts',(-6.01816590364594,39.8371987683928,-15.3653180873047));
#60686=CARTESIAN_POINT('Ctrl Pts',(-5.78615514903906,38.7768863939058,-15.4522019473171));
#60687=CARTESIAN_POINT('Ctrl Pts',(-6.39054216941777,39.7443708383147,-16.3756416702532));
#60688=CARTESIAN_POINT('Ctrl Pts',(-6.02657153999075,39.8260491189418,-15.3616221037249));
#60689=CARTESIAN_POINT('Ctrl Pts',(-5.81896213621546,38.7684973890572,-15.4398907177147));
#60690=CARTESIAN_POINT('Ctrl Pts',(-6.39829119296333,39.7426976933212,-16.3668617166323));
#60691=CARTESIAN_POINT('Ctrl Pts',(-6.0324962949229,39.8187094218724,-15.3590612008815));
#60692=CARTESIAN_POINT('Ctrl Pts',(-5.84088080302002,38.7634779552291,-15.4316124756347));
#60693=CARTESIAN_POINT('Ctrl Pts',(-6.42158691874072,39.7382413617845,-16.3402955022825));
#60694=CARTESIAN_POINT('Ctrl Pts',(-6.05116583633343,39.797127595989,-15.351106610322));
#60695=CARTESIAN_POINT('Ctrl Pts',(-5.90677442716201,38.750108959213,-15.4065643308179));
#60696=CARTESIAN_POINT('Ctrl Pts',(-6.43718213048319,39.7360200677615,-16.3222830574036));
#60697=CARTESIAN_POINT('Ctrl Pts',(-6.06488620812391,39.7831957544441,-15.3454045239078));
#60698=CARTESIAN_POINT('Ctrl Pts',(-5.95088659762375,38.743445078172,-15.3895811683148));
#60699=CARTESIAN_POINT('Ctrl Pts',(-6.46849740752571,39.7330531695987,-16.2856443359368));
#60700=CARTESIAN_POINT('Ctrl Pts',(-6.09483924332511,39.7566876277051,-15.333160094272));
#60701=CARTESIAN_POINT('Ctrl Pts',(-6.03946409560143,38.7345443835025,-15.3550360882633));
#60702=CARTESIAN_POINT('Ctrl Pts',(-6.484217551678,39.7323075626015,-16.2670179887174));
#60703=CARTESIAN_POINT('Ctrl Pts',(-6.11103676931995,39.7441010190891,-15.3266299702959));
#60704=CARTESIAN_POINT('Ctrl Pts',(-6.08392963895787,38.7323075641139,-15.3374741067549));
#60705=CARTESIAN_POINT('Ctrl Pts',(-6.5,39.7323075626015,-16.2480768092719));
#60706=CARTESIAN_POINT('Ctrl Pts',(-6.12857142857143,39.7323075626015,-15.3196152773135));
#60707=CARTESIAN_POINT('Ctrl Pts',(-6.12857142857143,38.7323075626015,-15.3196152773135));
#60708=CARTESIAN_POINT('Origin',(-37.,45.4641016151378,-17.5));
#60709=CARTESIAN_POINT('Origin',(-45.2221315177632,44.4440520797063,-25.3383443274765));
#60710=CARTESIAN_POINT('Origin',(-11.,51.,0.));
#60711=CARTESIAN_POINT('Origin',(-6.5,54.4282032302755,-24.));
#60712=CARTESIAN_POINT('',(-6.5,52.3811718911434,-24.5));
#60713=CARTESIAN_POINT('',(-6.5,54.4282032302755,-24.5));
#60714=CARTESIAN_POINT('Ctrl Pts',(-6.50000000000002,52.3811718911434,-24.5));
#60715=CARTESIAN_POINT('Ctrl Pts',(-6.45484712541262,52.3374123315343,-24.5));
#60716=CARTESIAN_POINT('Ctrl Pts',(-6.4063809595238,52.2931062029975,-24.4937365926974));
#60717=CARTESIAN_POINT('Ctrl Pts',(-6.29450947020769,52.1982971503326,-24.4606141098908));
#60718=CARTESIAN_POINT('Ctrl Pts',(-6.23114032575744,52.1503834195514,-24.4274665133501));
#60719=CARTESIAN_POINT('Ctrl Pts',(-6.13253307624096,52.0829899601412,-24.3440537454782));
#60720=CARTESIAN_POINT('Ctrl Pts',(-6.08952339015813,52.0568515986448,-24.2932685081818));
#60721=CARTESIAN_POINT('Ctrl Pts',(-6.0267513370081,52.0210538996719,-24.1747375197227));
#60722=CARTESIAN_POINT('Ctrl Pts',(-6.00719188754555,52.0110551102428,-24.1069871550009));
#60723=CARTESIAN_POINT('Ctrl Pts',(-6.00059405760162,52.0049022588122,-24.0279494392554));
#60724=CARTESIAN_POINT('Ctrl Pts',(-6.,52.0040117065365,-24.0140517567783));
#60725=CARTESIAN_POINT('Ctrl Pts',(-6.,52.0032753870454,-24.));
#60726=CARTESIAN_POINT('Origin',(-27.1034840901754,53.,1.07291666666666));
#60727=CARTESIAN_POINT('Origin',(-27.1034840901754,53.,1.07291666666666));
#60728=CARTESIAN_POINT('Origin',(-5.47112164030075,53.000000000001,-24.5000000000001));
#60729=CARTESIAN_POINT('Origin',(-3.43565291283912,53.,26.90625));
#60730=CARTESIAN_POINT('Origin',(-3.43565291283912,53.,26.90625));
#60731=CARTESIAN_POINT('Origin',(6.61363325216158E-15,53.,24.));
#60732=CARTESIAN_POINT('Origin',(3.43565291283914,53.,26.90625));
#60733=CARTESIAN_POINT('Origin',(3.43565291283914,53.,26.90625));
#60734=CARTESIAN_POINT('Origin',(15.2695685015073,53.,12.9166666666666));
#60735=CARTESIAN_POINT('Origin',(6.61287431064084E-15,53.,0.));
#60736=CARTESIAN_POINT('Origin',(15.2695685015073,53.,-12.9166666666667));
#60737=CARTESIAN_POINT('Origin',(27.1034840901754,53.,1.07291666666666));
#60738=CARTESIAN_POINT('Ctrl Pts',(15.8769086599362,26.2075694296671,4.49152217004988));
#60739=CARTESIAN_POINT('Ctrl Pts',(15.9873632533133,26.9858847285589,4.10107844589208));
#60740=CARTESIAN_POINT('Ctrl Pts',(16.8391456316905,27.0868129846264,4.28736180648697));
#60741=CARTESIAN_POINT('Ctrl Pts',(15.8582352049183,26.2455000465674,4.55753024670209));
#60742=CARTESIAN_POINT('Ctrl Pts',(15.9714605842203,27.0177778865802,4.16347898353059));
#60743=CARTESIAN_POINT('Ctrl Pts',(16.8193404549634,27.1209505355579,4.35036951074904));
#60744=CARTESIAN_POINT('Ctrl Pts',(15.8392331472462,26.2842765272885,4.62312840029494));
#60745=CARTESIAN_POINT('Ctrl Pts',(15.9552081857089,27.0505108449272,4.2257203082126));
#60746=CARTESIAN_POINT('Ctrl Pts',(16.7991867589916,27.155849366436,4.41298592969122));
#60747=CARTESIAN_POINT('Ctrl Pts',(15.810254271091,26.3437152476807,4.72091258212513));
#60748=CARTESIAN_POINT('Ctrl Pts',(15.9303287054477,27.1008592013043,4.31876680254219));
#60749=CARTESIAN_POINT('Ctrl Pts',(16.7684515907413,27.2093442101895,4.50632537208709));
#60750=CARTESIAN_POINT('Ctrl Pts',(15.8005153477853,26.3637405141118,4.75340512204032));
#60751=CARTESIAN_POINT('Ctrl Pts',(15.9219634459718,27.1178269445236,4.34968902000699));
#60752=CARTESIAN_POINT('Ctrl Pts',(16.7581224307191,27.2273669484456,4.53734097703345));
#60753=CARTESIAN_POINT('Ctrl Pts',(15.7808817629062,26.4042169640041,4.81818599630767));
#60754=CARTESIAN_POINT('Ctrl Pts',(15.9050753095569,27.1521659834681,4.4114003037423));
#60755=CARTESIAN_POINT('Ctrl Pts',(16.7372989339143,27.263795750215,4.59917726355392));
#60756=CARTESIAN_POINT('Ctrl Pts',(15.7709841530912,26.4246742589405,4.85048383592628));
#60757=CARTESIAN_POINT('Ctrl Pts',(15.8965503240519,27.1695414485629,4.44219808335061));
#60758=CARTESIAN_POINT('Ctrl Pts',(16.72680147,27.2822073140643,4.63000701827412));
#60759=CARTESIAN_POINT('Ctrl Pts',(15.7211457888462,26.527963020949,5.01135996312586));
#60760=CARTESIAN_POINT('Ctrl Pts',(15.8536759108252,27.2571485161243,4.59535151664664));
#60761=CARTESIAN_POINT('Ctrl Pts',(16.6739426048502,27.3751671919753,4.78357058767493));
#60762=CARTESIAN_POINT('Ctrl Pts',(15.6803478341989,26.6133981550309,5.13748080940201));
#60763=CARTESIAN_POINT('Ctrl Pts',(15.8183072530954,27.3301139516917,4.71622063716264));
#60764=CARTESIAN_POINT('Ctrl Pts',(16.6306720509859,27.452058805977,4.90395866359305));
#60765=CARTESIAN_POINT('Ctrl Pts',(15.5555633441787,26.8779283667801,5.50840431704435));
#60766=CARTESIAN_POINT('Ctrl Pts',(15.7099001145759,27.5563845907162,5.07174318477029));
#60767=CARTESIAN_POINT('Ctrl Pts',(16.4983248790498,27.6901359766523,5.25802199793798));
#60768=CARTESIAN_POINT('Ctrl Pts',(15.4691874138206,27.065223688674,5.74578785429625));
#60769=CARTESIAN_POINT('Ctrl Pts',(15.633882786453,27.7183716325533,5.30193650363448));
#60770=CARTESIAN_POINT('Ctrl Pts',(16.4067140519913,27.8587017525446,5.48461536708638));
#60771=CARTESIAN_POINT('Ctrl Pts',(15.2920609491932,27.4613270309352,6.20183111975059));
#60772=CARTESIAN_POINT('Ctrl Pts',(15.4763461124972,28.0643447982136,5.74688779723174));
#60773=CARTESIAN_POINT('Ctrl Pts',(16.2188526682064,28.2151947332129,5.91992938097804));
#60774=CARTESIAN_POINT('Ctrl Pts',(15.201305139851,27.6701352530085,6.42048862811649));
#60775=CARTESIAN_POINT('Ctrl Pts',(15.394911415866,28.2479943353604,5.96182339691564));
#60776=CARTESIAN_POINT('Ctrl Pts',(16.1225965145591,28.4031221189222,6.12864790645227));
#60777=CARTESIAN_POINT('Ctrl Pts',(15.063397310651,27.9997968012076,6.73477167440303));
#60778=CARTESIAN_POINT('Ctrl Pts',(15.2696355732375,28.541402061921,6.27340007303451));
#60779=CARTESIAN_POINT('Ctrl Pts',(15.9763306474089,28.6998174915388,6.42864535457189));
#60780=CARTESIAN_POINT('Ctrl Pts',(15.0171329992815,28.112431629095,6.83724424346893));
#60781=CARTESIAN_POINT('Ctrl Pts',(15.2275847859334,28.6416330504077,6.37495337745684));
#60782=CARTESIAN_POINT('Ctrl Pts',(15.9272624420383,28.8011888294802,6.52646007755072));
#60783=CARTESIAN_POINT('Ctrl Pts',(14.9474944335502,28.2856028304495,6.98752160996693));
#60784=CARTESIAN_POINT('Ctrl Pts',(15.1639331114985,28.7965496531306,6.52450489168869));
#60785=CARTESIAN_POINT('Ctrl Pts',(15.8534033631529,28.957042899895,6.66990665258495));
#60786=CARTESIAN_POINT('Ctrl Pts',(14.9242413338947,28.3440301462527,7.03704185847933));
#60787=CARTESIAN_POINT('Ctrl Pts',(15.1426746889094,28.8488125585796,6.57377108052547));
#60788=CARTESIAN_POINT('Ctrl Pts',(15.8287409864956,29.0096274805124,6.71717597981947));
#60789=CARTESIAN_POINT('Ctrl Pts',(14.889327508177,28.4327426653544,7.11046135857809));
#60790=CARTESIAN_POINT('Ctrl Pts',(15.1106696590438,28.9283638930351,6.64696562658708));
#60791=CARTESIAN_POINT('Ctrl Pts',(15.7917111742834,29.0894687421935,6.78725822899178));
#60792=CARTESIAN_POINT('Ctrl Pts',(14.8776905601943,28.4624753483755,7.13477680771444));
#60793=CARTESIAN_POINT('Ctrl Pts',(15.1000012851191,28.9550247920885,6.67120233635647));
#60794=CARTESIAN_POINT('Ctrl Pts',(15.7793689575767,29.1162281550713,6.81046843005605));
#60795=CARTESIAN_POINT('Ctrl Pts',(14.8544631761811,28.522162195526,7.183010528203));
#60796=CARTESIAN_POINT('Ctrl Pts',(15.0786880317589,29.0085874834985,6.71930924825527));
#60797=CARTESIAN_POINT('Ctrl Pts',(15.7547338552975,29.1699463138537,6.85650970805247));
#60798=CARTESIAN_POINT('Ctrl Pts',(14.8428668837395,28.5521312162157,7.20694113675592));
#60799=CARTESIAN_POINT('Ctrl Pts',(15.0680376418045,29.0355024561561,6.74319259210144));
#60800=CARTESIAN_POINT('Ctrl Pts',(15.7424347580747,29.1969184306039,6.87935256133954));
#60801=CARTESIAN_POINT('Ctrl Pts',(14.7386765131152,28.8229821364781,7.42065217988111));
#60802=CARTESIAN_POINT('Ctrl Pts',(14.9728123593002,29.2775407023946,6.95538233905929));
#60803=CARTESIAN_POINT('Ctrl Pts',(15.6319298287787,29.4406842412807,7.08334946253237));
#60804=CARTESIAN_POINT('Ctrl Pts',(14.6473111890801,29.071748056285,7.59881636225689));
#60805=CARTESIAN_POINT('Ctrl Pts',(14.8881630949714,29.5024636848611,7.13446033202847));
#60806=CARTESIAN_POINT('Ctrl Pts',(15.535027218385,29.6645735542109,7.25341527124138));
#60807=CARTESIAN_POINT('Ctrl Pts',(14.4693728540855,29.5855591847265,7.93240092198966));
#60808=CARTESIAN_POINT('Ctrl Pts',(14.7224664869594,29.9694548692142,7.47059284153777));
#60809=CARTESIAN_POINT('Ctrl Pts',(15.3463047553347,30.1270035400911,7.57183689452032));
#60810=CARTESIAN_POINT('Ctrl Pts',(14.3827951407555,29.8506033440453,8.08782034517746));
#60811=CARTESIAN_POINT('Ctrl Pts',(14.6412849462596,30.2115686379399,7.62808869657179));
#60812=CARTESIAN_POINT('Ctrl Pts',(15.254479912919,30.3655432686509,7.72019179758978));
#60813=CARTESIAN_POINT('Ctrl Pts',(14.2583927643846,30.261019135023,8.30392342666024));
#60814=CARTESIAN_POINT('Ctrl Pts',(14.5238989245498,30.5889923546909,7.84801190409701));
#60815=CARTESIAN_POINT('Ctrl Pts',(15.1225380068262,30.7349174586429,7.92647201231362));
#60816=CARTESIAN_POINT('Ctrl Pts',(14.2178380489227,30.3999707062553,8.37311388575839));
#60817=CARTESIAN_POINT('Ctrl Pts',(14.4856296693811,30.7167001609698,7.9183828465517));
#60818=CARTESIAN_POINT('Ctrl Pts',(15.0795254320222,30.8599738652951,7.99251745021501));
#60819=CARTESIAN_POINT('Ctrl Pts',(14.1388980403649,30.6823345265142,8.50573436767722));
#60820=CARTESIAN_POINT('Ctrl Pts',(14.4110045335691,30.9766778340591,8.0534028711467));
#60821=CARTESIAN_POINT('Ctrl Pts',(14.9958011856818,31.1141012882541,8.1191097289101));
#60822=CARTESIAN_POINT('Ctrl Pts',(14.1005125570259,30.825746585496,8.56916458200204));
#60823=CARTESIAN_POINT('Ctrl Pts',(14.3746261627414,31.1089703880548,8.11810372149017));
#60824=CARTESIAN_POINT('Ctrl Pts',(14.9550893113803,31.2431721338399,8.17965675141353));
#60825=CARTESIAN_POINT('Ctrl Pts',(14.0448396969175,31.0443707833594,8.65989242941114));
#60826=CARTESIAN_POINT('Ctrl Pts',(14.3217244652542,31.3111850624393,8.21083048026107));
#60827=CARTESIAN_POINT('Ctrl Pts',(14.896042341965,31.4399339005038,8.26626060646187));
#60828=CARTESIAN_POINT('Ctrl Pts',(14.0265998696782,31.1178302470309,8.68939833580717));
#60829=CARTESIAN_POINT('Ctrl Pts',(14.3043940626367,31.3791100903781,8.24097506569154));
#60830=CARTESIAN_POINT('Ctrl Pts',(14.8766970715514,31.5060474140306,8.29442533516559));
#60831=CARTESIAN_POINT('Ctrl Pts',(13.9997539373385,31.2289203061233,8.73253551550609));
#60832=CARTESIAN_POINT('Ctrl Pts',(14.2788527797159,31.4819620626231,8.28509109464653));
#60833=CARTESIAN_POINT('Ctrl Pts',(14.8482241146408,31.6060284614212,8.3356017343517));
#60834=CARTESIAN_POINT('Ctrl Pts',(13.9908909448787,31.266100496257,8.7467275967966));
#60835=CARTESIAN_POINT('Ctrl Pts',(14.2704211048916,31.5163797260547,8.29960214590518));
#60836=CARTESIAN_POINT('Ctrl Pts',(14.838823971551,31.6394906306444,8.34914872097351));
#60837=CARTESIAN_POINT('Ctrl Pts',(13.9733426643655,31.34076551118,8.77473463235667));
#60838=CARTESIAN_POINT('Ctrl Pts',(14.253720076538,31.5855220469117,8.32824609388835));
#60839=CARTESIAN_POINT('Ctrl Pts',(14.8202121599515,31.7066891401708,8.3758827097203));
#60840=CARTESIAN_POINT('Ctrl Pts',(13.9646513850397,31.3782767417852,8.78855907279825));
#60841=CARTESIAN_POINT('Ctrl Pts',(14.2454446251434,31.6202717609735,8.342389472868));
#60842=CARTESIAN_POINT('Ctrl Pts',(14.8109941368322,31.7404492457889,8.38907876649581));
#60843=CARTESIAN_POINT('Ctrl Pts',(13.9217346730834,31.566257920696,8.85660464288024));
#60844=CARTESIAN_POINT('Ctrl Pts',(14.2046283298307,31.794206482269,8.41191502944778));
#60845=CARTESIAN_POINT('Ctrl Pts',(14.7654764146937,31.9096322969191,8.45403135644424));
#60846=CARTESIAN_POINT('Ctrl Pts',(13.8891759531169,31.7177786407323,8.90752381063715));
#60847=CARTESIAN_POINT('Ctrl Pts',(14.1735469248987,31.9348489839235,8.46411039451801));
#60848=CARTESIAN_POINT('Ctrl Pts',(14.7309444404168,32.0460009372101,8.50263601677879));
#60849=CARTESIAN_POINT('Ctrl Pts',(13.797229628424,32.1757915805991,9.04981828300803));
#60850=CARTESIAN_POINT('Ctrl Pts',(14.0858535568985,32.3596444525066,8.60976381822387));
#60851=CARTESIAN_POINT('Ctrl Pts',(14.6334256167163,32.458212559268,8.63846255958131));
#60852=CARTESIAN_POINT('Ctrl Pts',(13.7435707260252,32.4857275239348,9.13075893855157));
#60853=CARTESIAN_POINT('Ctrl Pts',(14.0343219801121,32.6485678536188,8.69311636580977));
#60854=CARTESIAN_POINT('Ctrl Pts',(14.5765146617579,32.7371548930406,8.71572409483911));
#60855=CARTESIAN_POINT('Ctrl Pts',(13.6537210422616,33.1151908161921,9.26457752924306));
#60856=CARTESIAN_POINT('Ctrl Pts',(13.9480657183463,33.2358005618801,8.83077671102261));
#60857=CARTESIAN_POINT('Ctrl Pts',(14.481219547549,33.3036718249763,8.84346002411218));
#60858=CARTESIAN_POINT('Ctrl Pts',(13.6175303913262,33.434717557105,9.31745805895241));
#60859=CARTESIAN_POINT('Ctrl Pts',(13.9131698025808,33.5346731534088,8.88537710590861));
#60860=CARTESIAN_POINT('Ctrl Pts',(14.4428355251485,33.5912458765277,8.89393689342034));
#60861=CARTESIAN_POINT('Ctrl Pts',(13.5846002426724,33.8405183507168,9.36529610646282));
#60862=CARTESIAN_POINT('Ctrl Pts',(13.88142692472,33.9146324799541,8.93474090246188));
#60863=CARTESIAN_POINT('Ctrl Pts',(14.4079096116133,33.956466571422,8.93960048526914));
#60864=CARTESIAN_POINT('Ctrl Pts',(13.5786296974971,33.9219987331534,9.37394813624565));
#60865=CARTESIAN_POINT('Ctrl Pts',(13.875675508425,33.9908623767473,8.94366201738552));
#60866=CARTESIAN_POINT('Ctrl Pts',(14.4015772154364,34.029798911697,8.94785924088037));
#60867=CARTESIAN_POINT('Ctrl Pts',(13.5706234030671,34.0447089994668,9.38553155036112));
#60868=CARTESIAN_POINT('Ctrl Pts',(13.8679615185176,34.1056958349204,8.9556072796306));
#60869=CARTESIAN_POINT('Ctrl Pts',(14.3930856914591,34.1402381454566,8.95891613645648));
#60870=CARTESIAN_POINT('Ctrl Pts',(13.568112892907,34.0856940452786,9.38916021637687));
#60871=CARTESIAN_POINT('Ctrl Pts',(13.8655426622907,34.144048511225,8.95934916121749));
#60872=CARTESIAN_POINT('Ctrl Pts',(14.3904230292606,34.1771246847184,8.96237986304967));
#60873=CARTESIAN_POINT('Ctrl Pts',(13.5634127761087,34.1678290467875,9.39594864334385));
#60874=CARTESIAN_POINT('Ctrl Pts',(13.8610138988738,34.2209130571112,8.9663495479683));
#60875=CARTESIAN_POINT('Ctrl Pts',(14.3854380571442,34.2510461821083,8.96885972533652));
#60876=CARTESIAN_POINT('Ctrl Pts',(13.561221484919,34.2090153261087,9.39911083275795));
#60877=CARTESIAN_POINT('Ctrl Pts',(13.8589022053104,34.2594602815295,8.9696108109939));
#60878=CARTESIAN_POINT('Ctrl Pts',(14.3831139605077,34.2881138315147,8.97187817888002));
#60879=CARTESIAN_POINT('Ctrl Pts',(13.5511043760099,34.4148121032376,9.41370128814102));
#60880=CARTESIAN_POINT('Ctrl Pts',(13.849155508049,34.45201534129,8.98465351724142));
#60881=CARTESIAN_POINT('Ctrl Pts',(14.3723836940155,34.4733309209789,8.98580543178569));
#60882=CARTESIAN_POINT('Ctrl Pts',(13.5456900690161,34.5790374616588,9.42148098687002));
#60883=CARTESIAN_POINT('Ctrl Pts',(13.8439323192676,34.6058139523128,8.99268414889771));
#60884=CARTESIAN_POINT('Ctrl Pts',(14.3666412473947,34.6211337356892,8.9932315081297));
#60885=CARTESIAN_POINT('Ctrl Pts',(13.537394573329,35.0705004043849,9.43340033567814));
#60886=CARTESIAN_POINT('Ctrl Pts',(13.8359355950147,35.065908922897,9.00497875543769));
#60887=CARTESIAN_POINT('Ctrl Pts',(14.3578429948253,35.0634503604854,9.00460906824679));
#60888=CARTESIAN_POINT('Ctrl Pts',(13.5424689320019,35.3965264297717,9.4261476475004));
#60889=CARTESIAN_POINT('Ctrl Pts',(13.840841926183,35.3715820736891,8.99747657812311));
#60890=CARTESIAN_POINT('Ctrl Pts',(14.3632248902148,35.356873767978,8.99768604786805));
#60891=CARTESIAN_POINT('Ctrl Pts',(13.5731452714314,36.04542889236,9.38192153491666));
#60892=CARTESIAN_POINT('Ctrl Pts',(13.8704062236138,35.9789562622814,8.95186307707126));
#60893=CARTESIAN_POINT('Ctrl Pts',(14.3957604001304,35.9408859530551,8.95547021242402));
#60894=CARTESIAN_POINT('Ctrl Pts',(13.5987464460997,36.3683053308453,9.34494758660724));
#60895=CARTESIAN_POINT('Ctrl Pts',(13.8951293553185,36.2813491153718,8.91364706576509));
#60896=CARTESIAN_POINT('Ctrl Pts',(14.4229131602539,36.231474732343,8.92017689772887));
#60897=CARTESIAN_POINT('Ctrl Pts',(13.6429948627497,36.7699519970002,9.28002899073296));
#60898=CARTESIAN_POINT('Ctrl Pts',(13.9376215104944,36.6560661788744,8.84688422821406));
#60899=CARTESIAN_POINT('Ctrl Pts',(14.4698432966875,36.5929567118635,8.85820914649669));
#60900=CARTESIAN_POINT('Ctrl Pts',(13.6524563224124,36.850183759103,9.26610806147943));
#60901=CARTESIAN_POINT('Ctrl Pts',(13.9467191680184,36.7310121656428,8.83254762593825));
#60902=CARTESIAN_POINT('Ctrl Pts',(14.4798781777861,36.6651652938272,8.84492098660861));
#60903=CARTESIAN_POINT('Ctrl Pts',(13.6675536049653,36.9703850215887,9.24381193101625));
#60904=CARTESIAN_POINT('Ctrl Pts',(13.9612232706366,36.8432141958407,8.80960244735883));
#60905=CARTESIAN_POINT('Ctrl Pts',(14.4958904463355,36.7733464241577,8.82363831640363));
#60906=CARTESIAN_POINT('Ctrl Pts',(13.6727368747274,37.0104277105771,9.23614406980858));
#60907=CARTESIAN_POINT('Ctrl Pts',(13.9662034537542,36.8805966404157,8.80170992007976));
#60908=CARTESIAN_POINT('Ctrl Pts',(14.5013878534575,36.8093848422754,8.81631899426101));
#60909=CARTESIAN_POINT('Ctrl Pts',(13.6834029259183,37.0904642664689,9.22033487953449));
#60910=CARTESIAN_POINT('Ctrl Pts',(13.9764488572415,36.9553002795284,8.7854406320722));
#60911=CARTESIAN_POINT('Ctrl Pts',(14.5127003314097,36.8814177386533,8.8012284033937));
#60912=CARTESIAN_POINT('Ctrl Pts',(13.6888901621671,37.1304892288409,9.21218691413121));
#60913=CARTESIAN_POINT('Ctrl Pts',(13.981718702735,36.9926517283056,8.77705647210948));
#60914=CARTESIAN_POINT('Ctrl Pts',(14.5185201272134,36.9174402028251,8.79345080003374));
#60915=CARTESIAN_POINT('Ctrl Pts',(13.7170045302029,37.3300355326774,9.17035509250042));
#60916=CARTESIAN_POINT('Ctrl Pts',(14.0087376674906,37.1790072230197,8.73397918025916));
#60917=CARTESIAN_POINT('Ctrl Pts',(14.54833839483,37.0970318665379,8.75352042409837));
#60918=CARTESIAN_POINT('Ctrl Pts',(13.7416559284244,37.4877914628441,9.13341262033751));
#60919=CARTESIAN_POINT('Ctrl Pts',(14.0323966113954,37.3261029988049,8.69597582707544));
#60920=CARTESIAN_POINT('Ctrl Pts',(14.5744838161833,37.2390121959723,8.71825715532235));
#60921=CARTESIAN_POINT('Ctrl Pts',(13.8215245864057,37.955680800248,9.01247985304086));
#60922=CARTESIAN_POINT('Ctrl Pts',(14.1090338931848,37.7625210439417,8.57154787918128));
#60923=CARTESIAN_POINT('Ctrl Pts',(14.6591929945098,37.6601125767095,8.60282133020325));
#60924=CARTESIAN_POINT('Ctrl Pts',(13.8826479129921,38.2604495486085,8.91841437366726));
#60925=CARTESIAN_POINT('Ctrl Pts',(14.1675770164119,38.045983743127,8.47485390450271));
#60926=CARTESIAN_POINT('Ctrl Pts',(14.7240207625428,37.9344044350983,8.51303155432319));
#60927=CARTESIAN_POINT('Ctrl Pts',(14.017864413363,38.8567193826118,8.7043383036793));
#60928=CARTESIAN_POINT('Ctrl Pts',(14.2964001885856,38.5986463447174,8.2557534008036));
#60929=CARTESIAN_POINT('Ctrl Pts',(14.867432194178,38.4710472548887,8.30868621311197));
#60930=CARTESIAN_POINT('Ctrl Pts',(14.0919600671857,39.1482188475984,8.58432510753208));
#60931=CARTESIAN_POINT('Ctrl Pts',(14.3668901384109,38.868224427513,8.13293860738287));
#60932=CARTESIAN_POINT('Ctrl Pts',(14.9460184901712,38.7333967582374,8.19412816209205));
#60933=CARTESIAN_POINT('Ctrl Pts',(14.1910981741539,39.5046875011412,8.41808951704303));
#60934=CARTESIAN_POINT('Ctrl Pts',(14.4602864178378,39.1952890069765,7.96429217292035));
#60935=CARTESIAN_POINT('Ctrl Pts',(15.0511649604324,39.0542185263549,8.03544873490342));
#60936=CARTESIAN_POINT('Ctrl Pts',(14.2112522061825,39.5755849617352,8.38402921489386));
#60937=CARTESIAN_POINT('Ctrl Pts',(14.4793252621244,39.2605217727158,7.92963051378782));
#60938=CARTESIAN_POINT('Ctrl Pts',(15.0725404478885,39.1180262370522,8.00293662835892));
#60939=CARTESIAN_POINT('Ctrl Pts',(14.2419443789457,39.6813410899015,8.33171225457276));
#60940=CARTESIAN_POINT('Ctrl Pts',(14.5082645353832,39.3576677969082,7.8764721428416));
#60941=CARTESIAN_POINT('Ctrl Pts',(15.1050927502537,39.2132067466253,7.9529977116705));
#60942=CARTESIAN_POINT('Ctrl Pts',(14.2522556469912,39.7165068507578,8.31406240552784));
#60943=CARTESIAN_POINT('Ctrl Pts',(14.5179878775877,39.3899757919214,7.8585332814314));
#60944=CARTESIAN_POINT('Ctrl Pts',(15.1160289430727,39.244855929495,7.93615012856782));
#60945=CARTESIAN_POINT('Ctrl Pts',(14.2729796736805,39.7864832103593,8.27843438972032));
#60946=CARTESIAN_POINT('Ctrl Pts',(14.5375184271283,39.454233053145,7.82233732493678));
#60947=CARTESIAN_POINT('Ctrl Pts',(15.1380089699858,39.3078346492803,7.90214156794191));
#60948=CARTESIAN_POINT('Ctrl Pts',(14.2833976444658,39.821312032634,8.26044739242331));
#60949=CARTESIAN_POINT('Ctrl Pts',(14.5473308926922,39.4861993542643,7.80407040917203));
#60950=CARTESIAN_POINT('Ctrl Pts',(15.1490583323553,39.3391805874545,7.88497216155336));
#60951=CARTESIAN_POINT('Ctrl Pts',(14.3357529130929,39.9946689703288,8.1696522999116));
#60952=CARTESIAN_POINT('Ctrl Pts',(14.5967120092205,39.6455467928789,7.71171681169117));
#60953=CARTESIAN_POINT('Ctrl Pts',(15.2045866440913,39.4952018220261,7.79830411842659));
#60954=CARTESIAN_POINT('Ctrl Pts',(14.3784853171976,40.1308377145353,8.09426602317428));
#60955=CARTESIAN_POINT('Ctrl Pts',(14.6368508121003,39.7702029993696,7.63528497359585));
#60956=CARTESIAN_POINT('Ctrl Pts',(15.2499088883933,39.6177536843613,7.72634449117004));
#60957=CARTESIAN_POINT('Ctrl Pts',(14.5087039436106,40.5321094868054,7.85998980656673));
#60958=CARTESIAN_POINT('Ctrl Pts',(14.7591580200955,40.1377641963223,7.39760736865633));
#60959=CARTESIAN_POINT('Ctrl Pts',(15.3880195437736,39.9788982574772,7.50271719341424));
#60960=CARTESIAN_POINT('Ctrl Pts',(14.5982023821632,40.7900005483541,7.69300623367248));
#60961=CARTESIAN_POINT('Ctrl Pts',(14.8426060415872,40.3722055486072,7.22904427170515));
#60962=CARTESIAN_POINT('Ctrl Pts',(15.4829421245151,40.2110001980916,7.34332378435791));
#60963=CARTESIAN_POINT('Ctrl Pts',(14.7800664680989,41.2876229200236,7.33753997602127));
#60964=CARTESIAN_POINT('Ctrl Pts',(15.0109560529092,40.8221747459924,6.87233168107768));
#60965=CARTESIAN_POINT('Ctrl Pts',(15.675828261863,40.6588603029792,7.00401508691933));
#60966=CARTESIAN_POINT('Ctrl Pts',(14.8724375414028,41.52735181651,7.14905700140747));
#60967=CARTESIAN_POINT('Ctrl Pts',(15.095954979395,41.0376573972687,6.68377387394993));
#60968=CARTESIAN_POINT('Ctrl Pts',(15.7737975755315,40.8746162950652,6.82409952271975));
#60969=CARTESIAN_POINT('Ctrl Pts',(15.0114481107896,41.8736142592902,6.84971015627378));
#60970=CARTESIAN_POINT('Ctrl Pts',(15.2224090930038,41.3459299263025,6.38732005887134));
#60971=CARTESIAN_POINT('Ctrl Pts',(15.9212330152907,41.1862524710463,6.53835935782291));
#60972=CARTESIAN_POINT('Ctrl Pts',(15.0578619379628,41.9868080692592,6.74715158759131));
#60973=CARTESIAN_POINT('Ctrl Pts',(15.2646135022824,41.4466957957362,6.2856493085689));
#60974=CARTESIAN_POINT('Ctrl Pts',(15.9704597981201,41.2881268926528,6.44046254412343));
#60975=CARTESIAN_POINT('Ctrl Pts',(15.1158035851444,42.1255077461633,6.61538440065119));
#60976=CARTESIAN_POINT('Ctrl Pts',(15.3169420693408,41.5694200795832,6.15578753526126));
#60977=CARTESIAN_POINT('Ctrl Pts',(16.0319130547786,41.4129565926847,6.31468477759303));
#60978=CARTESIAN_POINT('Ctrl Pts',(15.1273876432894,42.1531065685038,6.5888532043739));
#60979=CARTESIAN_POINT('Ctrl Pts',(15.3274204676051,41.5938817796405,6.12959010828534));
#60980=CARTESIAN_POINT('Ctrl Pts',(16.0441991761153,41.4377955309865,6.28935954534903));
#60981=CARTESIAN_POINT('Ctrl Pts',(15.1504884935602,42.2078934932818,6.53555979741833));
#60982=CARTESIAN_POINT('Ctrl Pts',(15.3482944605132,41.6423974913488,6.07700707977798));
#60983=CARTESIAN_POINT('Ctrl Pts',(16.0687000757785,41.4871037596636,6.23848856701855));
#60984=CARTESIAN_POINT('Ctrl Pts',(15.16201224007,42.2350982910057,6.50878184192637));
#60985=CARTESIAN_POINT('Ctrl Pts',(15.358696260029,41.6664657192515,6.05060545885006));
#60986=CARTESIAN_POINT('Ctrl Pts',(16.0809222302044,41.511588075854,6.21292779194116));
#60987=CARTESIAN_POINT('Ctrl Pts',(15.1964975395775,42.3161505365769,6.4280547185655));
#60988=CARTESIAN_POINT('Ctrl Pts',(15.3898184625834,41.7381711202028,5.97100372060078));
#60989=CARTESIAN_POINT('Ctrl Pts',(16.1174975446523,41.5845350915181,6.13587008487654));
#60990=CARTESIAN_POINT('Ctrl Pts',(15.2193731284631,42.369435949201,6.37371235824478));
#60991=CARTESIAN_POINT('Ctrl Pts',(15.4103998557409,41.785178466038,5.91754508925415));
#60992=CARTESIAN_POINT('Ctrl Pts',(16.1417595309143,41.6324919593784,6.08399783316048));
#60993=CARTESIAN_POINT('Ctrl Pts',(15.3331009005101,42.6321602692512,6.09938186690947));
#60994=CARTESIAN_POINT('Ctrl Pts',(15.5130467364772,42.0177626523262,5.64666607840681));
#60995=CARTESIAN_POINT('Ctrl Pts',(16.2623798847315,41.8689438306172,5.82213691472101));
#60996=CARTESIAN_POINT('Ctrl Pts',(15.4219981693841,42.8305241152713,5.87155766518555));
#60997=CARTESIAN_POINT('Ctrl Pts',(15.5920752292007,42.1908243853748,5.42418175931921));
#60998=CARTESIAN_POINT('Ctrl Pts',(16.3566648587587,42.0474712782004,5.60466836487157));
#60999=CARTESIAN_POINT('Ctrl Pts',(15.5937398520647,43.2042079887926,5.39893455941937));
#61000=CARTESIAN_POINT('Ctrl Pts',(15.7433940983337,42.5145580603963,4.96612969069518));
#61001=CARTESIAN_POINT('Ctrl Pts',(16.5388151099388,42.3837867376654,5.15352814195569));
#61002=CARTESIAN_POINT('Ctrl Pts',(15.6765892287066,43.3795270223867,5.1541366866717));
#61003=CARTESIAN_POINT('Ctrl Pts',(15.8155572122032,42.6648295333535,4.73048547856337));
#61004=CARTESIAN_POINT('Ctrl Pts',(16.6266856526138,42.5415738546014,4.91985745378921));
#61005=CARTESIAN_POINT('Ctrl Pts',(15.8343896714213,43.7068883556104,4.64679228744702));
#61006=CARTESIAN_POINT('Ctrl Pts',(15.9517394444224,42.9433539713678,4.24602967800665));
#61007=CARTESIAN_POINT('Ctrl Pts',(16.7940497399473,42.8361990298401,4.43557418320846));
#61008=CARTESIAN_POINT('Ctrl Pts',(15.9093461307783,43.8589341148382,4.38424982322478));
#61009=CARTESIAN_POINT('Ctrl Pts',(16.0155885969954,43.0711748346473,3.99726291403837));
#61010=CARTESIAN_POINT('Ctrl Pts',(16.8735490068819,42.9730402005446,4.18496547848737));
#61011=CARTESIAN_POINT('Ctrl Pts',(15.9968739190125,44.0337693958938,4.04412643478191));
#61012=CARTESIAN_POINT('Ctrl Pts',(16.0891131415095,43.2163723621957,3.67917462890213));
#61013=CARTESIAN_POINT('Ctrl Pts',(16.9663814979273,43.130391939171,3.86030226102062));
#61014=CARTESIAN_POINT('Ctrl Pts',(16.0140705480854,44.0679730886499,3.97550284079341));
#61015=CARTESIAN_POINT('Ctrl Pts',(16.1035854874514,43.24484060037,3.6148164769343));
#61016=CARTESIAN_POINT('Ctrl Pts',(16.9846203450266,43.1611752596937,3.79479792452804));
#61017=CARTESIAN_POINT('Ctrl Pts',(16.0393769684763,44.11811371591,3.87164771798298));
#61018=CARTESIAN_POINT('Ctrl Pts',(16.1248097475127,43.2864454847151,3.5176909846929));
#61019=CARTESIAN_POINT('Ctrl Pts',(17.0114604845068,43.2063018202117,3.6956634942118));
#61020=CARTESIAN_POINT('Ctrl Pts',(16.0477158723614,44.1346030656301,3.83693785631023));
#61021=CARTESIAN_POINT('Ctrl Pts',(16.1317988050306,43.300120944147,3.48523803964491));
#61022=CARTESIAN_POINT('Ctrl Pts',(17.0203047755308,43.2211422335718,3.66253135522116));
#61023=CARTESIAN_POINT('Ctrl Pts',(16.0641840025573,44.1671063213702,3.76739554137956));
#61024=CARTESIAN_POINT('Ctrl Pts',(16.1455826144819,43.3270461204439,3.42028257915105));
#61025=CARTESIAN_POINT('Ctrl Pts',(17.0377709720975,43.2503951610147,3.59615005800666));
#61026=CARTESIAN_POINT('Ctrl Pts',(16.0723155893667,44.1831249045866,3.73255341105548));
#61027=CARTESIAN_POINT('Ctrl Pts',(16.1523788294993,43.3402986366979,3.38777194787044));
#61028=CARTESIAN_POINT('Ctrl Pts',(17.0463953813549,43.2648118846088,3.56289166263266));
#61029=CARTESIAN_POINT('Ctrl Pts',(16.112456458332,44.2620570473186,3.55798830906263));
#61030=CARTESIAN_POINT('Ctrl Pts',(16.1859599003788,43.4056750884538,3.22467629046144));
#61031=CARTESIAN_POINT('Ctrl Pts',(17.0889690250921,43.3358508065297,3.39626134644081));
#61032=CARTESIAN_POINT('Ctrl Pts',(16.1429146628079,44.321490558741,3.41720255158772));
#61033=CARTESIAN_POINT('Ctrl Pts',(16.2112170112945,43.4545025083997,3.09399963066693));
#61034=CARTESIAN_POINT('Ctrl Pts',(17.1212731775395,43.389340961842,3.26187494898354));
#61035=CARTESIAN_POINT('Ctrl Pts',(16.229144054607,44.4887700038955,2.99144640783051));
#61036=CARTESIAN_POINT('Ctrl Pts',(16.282607511081,43.591807170456,2.6991480196057));
#61037=CARTESIAN_POINT('Ctrl Pts',(17.2127285815789,43.5398924483796,2.85547137921157));
#61038=CARTESIAN_POINT('Ctrl Pts',(16.2797738357512,44.5856221569172,2.70308430094746));
#61039=CARTESIAN_POINT('Ctrl Pts',(16.3237841620316,43.6700048185059,2.43483412170548));
#61040=CARTESIAN_POINT('Ctrl Pts',(17.2664268276358,43.6270593773696,2.58021665754872));
#61041=CARTESIAN_POINT('Ctrl Pts',(16.3662877960953,44.7499338788673,2.11715012589449));
#61042=CARTESIAN_POINT('Ctrl Pts',(16.3937978726645,43.8021685587023,1.90074237494269));
#61043=CARTESIAN_POINT('Ctrl Pts',(17.3581840457416,43.7749399125848,2.02091588916502));
#61044=CARTESIAN_POINT('Ctrl Pts',(16.402174958515,44.8173953240164,1.8195789350148));
#61045=CARTESIAN_POINT('Ctrl Pts',(16.4224358551378,43.8557423131687,1.6316735546018));
#61046=CARTESIAN_POINT('Ctrl Pts',(17.3962461828893,43.8356552065899,1.73687068039507));
#61047=CARTESIAN_POINT('Ctrl Pts',(16.4440583713838,44.8958262298579,1.36601500577945));
#61048=CARTESIAN_POINT('Ctrl Pts',(16.4557537708206,43.9178757918761,1.22353172397691));
#61049=CARTESIAN_POINT('Ctrl Pts',(17.4406679778708,43.9062430148725,1.30392332311912));
#61050=CARTESIAN_POINT('Ctrl Pts',(16.4560267904858,44.9181691585247,1.21362389233826));
#61051=CARTESIAN_POINT('Ctrl Pts',(16.465245045828,43.9355291501292,1.08657788633077));
#61052=CARTESIAN_POINT('Ctrl Pts',(17.4533617541891,43.9263516483037,1.15845908846732));
#61053=CARTESIAN_POINT('Ctrl Pts',(16.4708618799835,44.9458224158849,0.98317551882238));
#61054=CARTESIAN_POINT('Ctrl Pts',(16.476991410704,43.9573497406529,0.879856072656254));
#61055=CARTESIAN_POINT('Ctrl Pts',(17.4690959376098,43.9512395775681,0.938485656355758));
#61056=CARTESIAN_POINT('Ctrl Pts',(16.4752871841395,44.9540627945076,0.906048965804147));
#61057=CARTESIAN_POINT('Ctrl Pts',(16.4804918339109,43.9638465742228,0.810700730796114));
#61058=CARTESIAN_POINT('Ctrl Pts',(17.4737894414959,43.9586559173861,0.864864860870638));
#61059=CARTESIAN_POINT('Ctrl Pts',(16.4811281425855,44.9649323439329,0.789884978814111));
#61060=CARTESIAN_POINT('Ctrl Pts',(16.4851083683136,43.9724103538098,0.706624078649839));
#61061=CARTESIAN_POINT('Ctrl Pts',(17.4799843964452,43.9684385109803,0.753981062883885));
#61062=CARTESIAN_POINT('Ctrl Pts',(16.4829427373917,44.9683078282227,0.751074106761979));
#61063=CARTESIAN_POINT('Ctrl Pts',(16.4865420704517,43.9750690241147,0.671857267230879));
#61064=CARTESIAN_POINT('Ctrl Pts',(17.4819089664434,43.9714764465119,0.716934323975719));
#61065=CARTESIAN_POINT('Ctrl Pts',(16.4863013241423,44.9745536029427,0.673336652475124));
#61066=CARTESIAN_POINT('Ctrl Pts',(16.4891948319328,43.9799871259377,0.602238655241295));
#61067=CARTESIAN_POINT('Ctrl Pts',(17.4854711034336,43.9770976431059,0.642730395542892));
#61068=CARTESIAN_POINT('Ctrl Pts',(16.4878418236565,44.9774174003737,0.634492642641704));
#61069=CARTESIAN_POINT('Ctrl Pts',(16.4904109816433,43.9822411637506,0.567462772022506));
#61070=CARTESIAN_POINT('Ctrl Pts',(17.4871049662947,43.9796750605875,0.605652025131273));
#61071=CARTESIAN_POINT('Ctrl Pts',(16.4948535761857,44.9904491876333,0.44039544480284));
#61072=CARTESIAN_POINT('Ctrl Pts',(16.4959475121185,43.9925006421478,0.393653808714096));
#61073=CARTESIAN_POINT('Ctrl Pts',(17.4945416725464,43.9914036677432,0.420377440177512));
#61074=CARTESIAN_POINT('Ctrl Pts',(16.4982530996368,44.9967581364226,0.285510603939235));
#61075=CARTESIAN_POINT('Ctrl Pts',(16.4986230123992,43.9974523683355,0.255222110228282));
#61076=CARTESIAN_POINT('Ctrl Pts',(17.4981472271006,43.9970817212605,0.272532829876073));
#61077=CARTESIAN_POINT('Ctrl Pts',(16.5007066493061,45.0013123694504,-0.0234886818206301));
#61078=CARTESIAN_POINT('Ctrl Pts',(16.5005562753881,44.001030959175,-0.0210215393702913));
#61079=CARTESIAN_POINT('Ctrl Pts',(17.5007494764801,44.0011805303849,-0.0224210128910837));
#61080=CARTESIAN_POINT('Ctrl Pts',(16.4997606328126,44.999557489536,-0.177603113095881));
#61081=CARTESIAN_POINT('Ctrl Pts',(16.4998121438015,43.9996542479657,-0.158706164302627));
#61082=CARTESIAN_POINT('Ctrl Pts',(17.4997461257051,43.9996011387621,-0.16953023225577));
#61083=CARTESIAN_POINT('Ctrl Pts',(16.4935850865834,44.9880905305289,-0.485071950900073));
#61084=CARTESIAN_POINT('Ctrl Pts',(16.4949439253717,43.9906402228509,-0.433673029434492));
#61085=CARTESIAN_POINT('Ctrl Pts',(17.4931963049589,43.989280876643,-0.46302319302334));
#61086=CARTESIAN_POINT('Ctrl Pts',(16.4883555209821,44.9783783650866,-0.638426349728915));
#61087=CARTESIAN_POINT('Ctrl Pts',(16.4908241367169,43.983010890298,-0.570831093510023));
#61088=CARTESIAN_POINT('Ctrl Pts',(17.4876497967006,43.9805399287279,-0.609406926989948));
#61089=CARTESIAN_POINT('Ctrl Pts',(16.4736638585154,44.951044676118,-0.944380784970185));
#61090=CARTESIAN_POINT('Ctrl Pts',(16.4792132612985,43.9614766171799,-0.844947715891262));
#61091=CARTESIAN_POINT('Ctrl Pts',(17.47206773271,43.9559396112014,-0.901454321999671));
#61092=CARTESIAN_POINT('Ctrl Pts',(16.4642017308171,44.9334231368575,-1.09698081900314));
#61093=CARTESIAN_POINT('Ctrl Pts',(16.4717324138027,43.9475908096718,-0.981785275421627));
#61094=CARTESIAN_POINT('Ctrl Pts',(17.4620321440808,43.940080227518,-1.04711798067983));
#61095=CARTESIAN_POINT('Ctrl Pts',(16.441085917582,44.8902614198252,-1.40142762961972));
#61096=CARTESIAN_POINT('Ctrl Pts',(16.4533815640137,43.9134527552254,-1.25544439804365));
#61097=CARTESIAN_POINT('Ctrl Pts',(17.4375153759351,43.9012346862572,-1.33772627995896));
#61098=CARTESIAN_POINT('Ctrl Pts',(16.4274322046631,44.8647212958546,-1.55327440899518));
#61099=CARTESIAN_POINT('Ctrl Pts',(16.4425275239753,43.8932305455644,-1.39214821663313));
#61100=CARTESIAN_POINT('Ctrl Pts',(17.4230341672312,43.8782485769846,-1.48267092310701));
#61101=CARTESIAN_POINT('Ctrl Pts',(16.4038318406658,44.8204219027532,-1.78047704290001));
#61102=CARTESIAN_POINT('Ctrl Pts',(16.4236582623586,43.8579704062684,-1.59747887342057));
#61103=CARTESIAN_POINT('Ctrl Pts',(17.3980034815883,43.8383791273345,-1.69954615022252));
#61104=CARTESIAN_POINT('Ctrl Pts',(16.3954450179849,44.8046567812815,-1.85611662919189));
#61105=CARTESIAN_POINT('Ctrl Pts',(16.4169484530449,43.8454168392665,-1.66586277048818));
#61106=CARTESIAN_POINT('Ctrl Pts',(17.3891083678211,43.8241905193902,-1.77174756870095));
#61107=CARTESIAN_POINT('Ctrl Pts',(16.3820871255076,44.7795006112695,-1.96943341649774));
#61108=CARTESIAN_POINT('Ctrl Pts',(16.4062319638247,43.8253349631854,-1.768514534337));
#61109=CARTESIAN_POINT('Ctrl Pts',(17.3749409080326,43.8015499687257,-1.879913585899));
#61110=CARTESIAN_POINT('Ctrl Pts',(16.377504880929,44.770863776863,-2.00718191127611));
#61111=CARTESIAN_POINT('Ctrl Pts',(16.4025541708227,43.8184380318085,-1.80271826733453));
#61112=CARTESIAN_POINT('Ctrl Pts',(17.3700809523118,43.7937768185068,-1.91594623764296));
#61113=CARTESIAN_POINT('Ctrl Pts',(16.3680815161057,44.7530851039602,-2.08263122802109));
#61114=CARTESIAN_POINT('Ctrl Pts',(16.3949823625954,43.8042269216823,-1.87113562920749));
#61115=CARTESIAN_POINT('Ctrl Pts',(17.3600864758251,43.7777760145525,-1.98796603532164));
#61116=CARTESIAN_POINT('Ctrl Pts',(16.3632376023291,44.7439379841849,-2.12035312043325));
#61117=CARTESIAN_POINT('Ctrl Pts',(16.3910864954017,43.7969092708944,-1.90536667503487));
#61118=CARTESIAN_POINT('Ctrl Pts',(17.3549489921576,43.7695436076108,-2.02397329393255));
#61119=CARTESIAN_POINT('Ctrl Pts',(16.3384034872043,44.6969941607675,-2.30860270705501));
#61120=CARTESIAN_POINT('Ctrl Pts',(16.3711201266365,43.7593731860622,-2.0760735616022));
#61121=CARTESIAN_POINT('Ctrl Pts',(17.328609782944,43.727294170591,-2.20366606939342));
#61122=CARTESIAN_POINT('Ctrl Pts',(16.316666398052,44.6557569516807,-2.45734547442349));
#61123=CARTESIAN_POINT('Ctrl Pts',(16.3535610329279,43.7262614947939,-2.21154871046545));
#61124=CARTESIAN_POINT('Ctrl Pts',(17.3055552971597,43.6901806864659,-2.34564779295502));
#61125=CARTESIAN_POINT('Ctrl Pts',(16.2696860394868,44.566166141375,-2.75126612719684));
#61126=CARTESIAN_POINT('Ctrl Pts',(16.315383867761,43.6539391818024,-2.48026578450734));
#61127=CARTESIAN_POINT('Ctrl Pts',(17.2557276510028,43.609548964849,-2.62620839879226));
#61128=CARTESIAN_POINT('Ctrl Pts',(16.2444425920206,44.5178122627343,-2.89644386444925));
#61129=CARTESIAN_POINT('Ctrl Pts',(16.2947921426187,43.6147800923035,-2.61343081272645));
#61130=CARTESIAN_POINT('Ctrl Pts',(17.2289543007661,43.5660304785905,-2.76478713969546));
#61131=CARTESIAN_POINT('Ctrl Pts',(16.1637732673119,44.3623460870145,-3.32680665282513));
#61132=CARTESIAN_POINT('Ctrl Pts',(16.228751596228,43.4885065479902,-3.00872279958398));
#61133=CARTESIAN_POINT('Ctrl Pts',(17.1433959375855,43.4261109338679,-3.17558795847649));
#61134=CARTESIAN_POINT('Ctrl Pts',(16.1034130962697,44.2448568131152,-3.60683310989697));
#61135=CARTESIAN_POINT('Ctrl Pts',(16.1788594609402,43.3922946051711,-3.26840131996947));
#61136=CARTESIAN_POINT('Ctrl Pts',(17.0793775817667,43.3203705977857,-3.44288592546756));
#61137=CARTESIAN_POINT('Ctrl Pts',(15.971082818307,43.9829218056908,-4.15375397007533));
#61138=CARTESIAN_POINT('Ctrl Pts',(16.0678613880117,43.1749038617298,-3.78004646974489));
#61139=CARTESIAN_POINT('Ctrl Pts',(16.9390273041549,43.0846291125409,-3.96494672006258));
#61140=CARTESIAN_POINT('Ctrl Pts',(15.8991086468391,43.8384751876644,-4.42064712392545));
#61141=CARTESIAN_POINT('Ctrl Pts',(16.0069841963327,43.0542208336615,-4.03164651818705));
#61142=CARTESIAN_POINT('Ctrl Pts',(16.8626910699957,42.9546271680979,-4.2197083547663));
#61143=CARTESIAN_POINT('Ctrl Pts',(15.8027846939592,43.6409776592958,-4.74622028184776));
#61144=CARTESIAN_POINT('Ctrl Pts',(15.9239456942855,42.8862343965702,-4.3427395313841));
#61145=CARTESIAN_POINT('Ctrl Pts',(16.7605293128805,42.7768794073196,-4.53048272074057));
#61146=CARTESIAN_POINT('Ctrl Pts',(15.7832020058401,43.6006290479835,-4.81093189184897));
#61147=CARTESIAN_POINT('Ctrl Pts',(15.9071072368669,42.8520156916865,-4.40437522421748));
#61148=CARTESIAN_POINT('Ctrl Pts',(16.7397597973034,42.740565660211,-4.59225289128511));
#61149=CARTESIAN_POINT('Ctrl Pts',(15.7533680246834,43.5388242348736,-4.90739530557529));
#61150=CARTESIAN_POINT('Ctrl Pts',(15.8813574947029,42.7994203500316,-4.49651575444794));
#61151=CARTESIAN_POINT('Ctrl Pts',(16.7081176995267,42.684941333135,-4.68433160073687));
#61152=CARTESIAN_POINT('Ctrl Pts',(15.7433467070133,43.5180089530702,-4.93944909919554));
#61153=CARTESIAN_POINT('Ctrl Pts',(15.8727041546145,42.7817018827648,-4.52713625468849));
#61154=CARTESIAN_POINT('Ctrl Pts',(16.6974890303406,42.6662075810719,-4.71492840247447));
#61155=CARTESIAN_POINT('Ctrl Pts',(15.7231535893805,43.4759493179362,-5.00335528875631));
#61156=CARTESIAN_POINT('Ctrl Pts',(15.8552432110586,42.7458557749306,-4.58824457822864));
#61157=CARTESIAN_POINT('Ctrl Pts',(16.6760720897177,42.628353912667,-4.77592976284654));
#61158=CARTESIAN_POINT('Ctrl Pts',(15.7129877823714,43.4547173657021,-5.03518828987221));
#61159=CARTESIAN_POINT('Ctrl Pts',(15.8464411539109,42.7277396174676,-4.61871374081455));
#61160=CARTESIAN_POINT('Ctrl Pts',(16.6652901742407,42.6092451572783,-4.80631580816218));
#61161=CARTESIAN_POINT('Ctrl Pts',(15.6619216546864,43.3477580321763,-5.19344863237848));
#61162=CARTESIAN_POINT('Ctrl Pts',(15.8022819829115,42.6366080996778,-4.76993809467135));
#61163=CARTESIAN_POINT('Ctrl Pts',(16.6111291357615,42.512981765177,-4.95738249258125));
#61164=CARTESIAN_POINT('Ctrl Pts',(15.6202189508121,43.2594435926603,-5.31745448945332));
#61165=CARTESIAN_POINT('Ctrl Pts',(15.7659413926522,42.5608428041457,-4.88922064491253));
#61166=CARTESIAN_POINT('Ctrl Pts',(16.566898999381,42.4334987763842,-5.07575171548048));
#61167=CARTESIAN_POINT('Ctrl Pts',(15.4929526417546,42.9864272209814,-5.68195984817183));
#61168=CARTESIAN_POINT('Ctrl Pts',(15.6548243306024,42.3262950844098,-5.23984103420753));
#61169=CARTESIAN_POINT('Ctrl Pts',(16.431919595095,42.1877840621362,-5.42368863587617));
#61170=CARTESIAN_POINT('Ctrl Pts',(15.4052313951022,42.7936764333705,-5.91496728026137));
#61171=CARTESIAN_POINT('Ctrl Pts',(15.5772391839006,42.1588707010981,-5.46658244560214));
#61172=CARTESIAN_POINT('Ctrl Pts',(16.3388819173383,42.0143083672418,-5.64610481430131));
#61173=CARTESIAN_POINT('Ctrl Pts',(15.2260498958022,42.3869745661045,-6.36202772981797));
#61174=CARTESIAN_POINT('Ctrl Pts',(15.4171543510239,41.8022449748656,-5.90416869454143));
#61175=CARTESIAN_POINT('Ctrl Pts',(16.1488409510981,41.6482767143899,-6.07284432319289));
#61176=CARTESIAN_POINT('Ctrl Pts',(15.134584339902,42.1730236614296,-6.57607876549311));
#61177=CARTESIAN_POINT('Ctrl Pts',(15.3347222581386,41.6133575955481,-6.11522249445178));
#61178=CARTESIAN_POINT('Ctrl Pts',(16.051832035793,41.4557209144361,-6.27716576157246));
#61179=CARTESIAN_POINT('Ctrl Pts',(14.9961179851292,41.8358199562313,-6.88324481216384));
#61180=CARTESIAN_POINT('Ctrl Pts',(15.2084472214612,41.3122217578598,-6.42057772001959));
#61181=CARTESIAN_POINT('Ctrl Pts',(15.9049737927767,41.1522376006794,-6.57036971072575));
#61182=CARTESIAN_POINT('Ctrl Pts',(14.9497520217687,41.7206997451385,-6.98331039827688));
#61183=CARTESIAN_POINT('Ctrl Pts',(15.16614239646,41.2094392579748,-6.52001184677474));
#61184=CARTESIAN_POINT('Ctrl Pts',(15.8557977745928,41.0486294178944,-6.66588685926462));
#61185=CARTESIAN_POINT('Ctrl Pts',(14.8800931267622,41.5438354639073,-7.12991977140524));
#61186=CARTESIAN_POINT('Ctrl Pts',(15.1022410222233,41.0507224912159,-6.666282802179));
#61187=CARTESIAN_POINT('Ctrl Pts',(15.7819171342091,40.8894515756627,-6.80583216820748));
#61188=CARTESIAN_POINT('Ctrl Pts',(14.8568552878022,41.484182951149,-7.1782077589911));
#61189=CARTESIAN_POINT('Ctrl Pts',(15.0809202996962,40.9971980762009,-6.71444353496276));
#61190=CARTESIAN_POINT('Ctrl Pts',(15.7572709430864,40.8357643178049,-6.85192524646453));
#61191=CARTESIAN_POINT('Ctrl Pts',(14.8219981963677,41.3936403419064,-7.24976367789764));
#61192=CARTESIAN_POINT('Ctrl Pts',(15.0488556165099,40.9157605080403,-6.78595401277065));
#61193=CARTESIAN_POINT('Ctrl Pts',(15.720301303522,40.7542759750313,-6.92022862282764));
#61194=CARTESIAN_POINT('Ctrl Pts',(14.8103768169327,41.3632758321973,-7.27347409955783));
#61195=CARTESIAN_POINT('Ctrl Pts',(15.0381645224724,40.8884513593707,-6.80964490693201));
#61196=CARTESIAN_POINT('Ctrl Pts',(15.7079755988858,40.7269479181449,-6.94286129770825));
#61197=CARTESIAN_POINT('Ctrl Pts',(14.7871949947469,41.3023381908314,-7.32048844844451));
#61198=CARTESIAN_POINT('Ctrl Pts',(15.0168199878777,40.8336038430639,-6.85664802598089));
#61199=CARTESIAN_POINT('Ctrl Pts',(15.6833888197048,40.6721040445935,-6.98773863017686));
#61200=CARTESIAN_POINT('Ctrl Pts',(14.7756276476925,41.2717472261591,-7.34380663171041));
#61201=CARTESIAN_POINT('Ctrl Pts',(15.0061600357127,40.8060495548255,-6.8799753372946));
#61202=CARTESIAN_POINT('Ctrl Pts',(15.6711204221094,40.6445721782689,-7.00999689573379));
#61203=CARTESIAN_POINT('Ctrl Pts',(14.6717534680737,40.9953295236136,-7.551980979435));
#61204=CARTESIAN_POINT('Ctrl Pts',(14.910895023212,40.5582946685239,-7.08717243073097));
#61205=CARTESIAN_POINT('Ctrl Pts',(15.5609508466639,40.3957962636541,-7.20870876993529));
#61206=CARTESIAN_POINT('Ctrl Pts',(14.5810647211324,40.741832913012,-7.72504743234233));
#61207=CARTESIAN_POINT('Ctrl Pts',(14.8266034407128,40.3284650320611,-7.26150923309475));
#61208=CARTESIAN_POINT('Ctrl Pts',(15.4647658178036,40.1676493290605,-7.37390856444987));
#61209=CARTESIAN_POINT('Ctrl Pts',(14.4053000909514,40.2189658652342,-8.04805166012557));
#61210=CARTESIAN_POINT('Ctrl Pts',(14.6624713147881,39.8520942263093,-7.58761069327075));
#61211=CARTESIAN_POINT('Ctrl Pts',(15.2783487987737,39.6970690159146,-7.68223078049221));
#61212=CARTESIAN_POINT('Ctrl Pts',(14.3202196741063,39.9495964563036,-8.19798859025269));
#61213=CARTESIAN_POINT('Ctrl Pts',(14.5824821731141,39.6054725337204,-7.73982483051287));
#61214=CARTESIAN_POINT('Ctrl Pts',(15.1881119978371,39.4546365627441,-7.82535239493351));
#61215=CARTESIAN_POINT('Ctrl Pts',(14.1987070119549,39.5329899966079,-8.40554259396074));
#61216=CARTESIAN_POINT('Ctrl Pts',(14.4675712776125,39.2216395207323,-7.95135792883057));
#61217=CARTESIAN_POINT('Ctrl Pts',(15.0592349397921,39.0796907709945,-8.02347212656833));
#61218=CARTESIAN_POINT('Ctrl Pts',(14.1592228767318,39.3920245639935,-8.47182899757806));
#61219=CARTESIAN_POINT('Ctrl Pts',(14.4302307228589,39.0918382370354,-8.01887552296388));
#61220=CARTESIAN_POINT('Ctrl Pts',(15.0173578287548,38.9528218891227,-8.08674551157961));
#61221=CARTESIAN_POINT('Ctrl Pts',(14.0826436992676,39.1057333760433,-8.59852461046018));
#61222=CARTESIAN_POINT('Ctrl Pts',(14.3576897375667,38.8277840539175,-8.14804214154577));
#61223=CARTESIAN_POINT('Ctrl Pts',(14.9361374939208,38.6951598352862,-8.20768223360701));
#61224=CARTESIAN_POINT('Ctrl Pts',(14.0455484751751,38.9604078024459,-8.65893401842002));
#61225=CARTESIAN_POINT('Ctrl Pts',(14.3224658365587,38.6935038701764,-8.20974266782632));
#61226=CARTESIAN_POINT('Ctrl Pts',(14.8967940762729,38.564366826571,-8.26534575917441));
#61227=CARTESIAN_POINT('Ctrl Pts',(13.9741231020615,38.6651847931096,-8.77373659465044));
#61228=CARTESIAN_POINT('Ctrl Pts',(14.2545506255991,38.4203292745446,-8.32708424104715));
#61229=CARTESIAN_POINT('Ctrl Pts',(14.8210398970475,38.2986661336681,-8.37493003741839));
#61230=CARTESIAN_POINT('Ctrl Pts',(13.9397927396565,38.5152876114838,-8.82813006373624));
#61231=CARTESIAN_POINT('Ctrl Pts',(14.2218349017627,38.2814009529421,-8.38277478959687));
#61232=CARTESIAN_POINT('Ctrl Pts',(14.7846289082318,38.1637586777924,-8.42685107588136));
#61233=CARTESIAN_POINT('Ctrl Pts',(13.8906779238092,38.2868159369556,-8.90505431363061));
#61234=CARTESIAN_POINT('Ctrl Pts',(14.1749330362927,38.0691860959213,-8.46165291031302));
#61235=CARTESIAN_POINT('Ctrl Pts',(14.7325374397322,37.9581341823412,-8.50027876989112));
#61236=CARTESIAN_POINT('Ctrl Pts',(13.8747711745264,38.2103676139026,-8.92981141108521));
#61237=CARTESIAN_POINT('Ctrl Pts',(14.1597438957798,37.9981958667913,-8.48703108097704));
#61238=CARTESIAN_POINT('Ctrl Pts',(14.7156666457513,37.8893306954536,-8.5239105447298));
#61239=CARTESIAN_POINT('Ctrl Pts',(13.8439407534612,38.0569848263093,-8.977533703511));
#61240=CARTESIAN_POINT('Ctrl Pts',(14.1302874730393,37.855684813066,-8.53596677843347));
#61241=CARTESIAN_POINT('Ctrl Pts',(14.6829677161225,37.7512861943861,-8.569463642424));
#61242=CARTESIAN_POINT('Ctrl Pts',(13.8290135932356,37.9800341471073,-9.00050435994528));
#61243=CARTESIAN_POINT('Ctrl Pts',(14.1160133673981,37.7841410413401,-8.5595362357428));
#61244=CARTESIAN_POINT('Ctrl Pts',(14.6671358801619,37.6820305869951,-8.59139017821769));
#61245=CARTESIAN_POINT('Ctrl Pts',(13.7568984117905,37.5939762225734,-9.11092076643811));
#61246=CARTESIAN_POINT('Ctrl Pts',(14.0471914590982,37.4259317837796,-8.67257888611769));
#61247=CARTESIAN_POINT('Ctrl Pts',(14.5906500859663,37.3345784750488,-8.6967876579279));
#61248=CARTESIAN_POINT('Ctrl Pts',(13.7072727192612,37.2809629485317,-9.185091616072));
#61249=CARTESIAN_POINT('Ctrl Pts',(13.9994761483249,37.1338465170385,-8.74902077756027));
#61250=CARTESIAN_POINT('Ctrl Pts',(14.5380167776266,37.0528665436847,-8.76758710574609));
#61251=CARTESIAN_POINT('Ctrl Pts',(13.6262054933649,36.6462732759949,-9.30493187769102));
#61252=CARTESIAN_POINT('Ctrl Pts',(13.921580734334,36.5412824787765,-8.8723756821566));
#61253=CARTESIAN_POINT('Ctrl Pts',(14.4520363909247,36.481645869576,-8.881980084429));
#61254=CARTESIAN_POINT('Ctrl Pts',(13.5947644787342,36.3245972840291,-9.35060353862456));
#61255=CARTESIAN_POINT('Ctrl Pts',(13.8912417590967,36.2402098290348,-8.91955632269035));
#61256=CARTESIAN_POINT('Ctrl Pts',(14.4186898613794,36.192137492116,-8.92557576079275));
#61257=CARTESIAN_POINT('Ctrl Pts',(13.5680981899448,35.9167592473805,-9.38918524120016));
#61258=CARTESIAN_POINT('Ctrl Pts',(13.8655300244092,35.8582683652265,-8.95937275428701));
#61259=CARTESIAN_POINT('Ctrl Pts',(14.3904074352514,35.8250832785829,-8.96240375051597));
#61260=CARTESIAN_POINT('Ctrl Pts',(13.563396609019,35.8349039817843,-9.39597376806161));
#61261=CARTESIAN_POINT('Ctrl Pts',(13.8609990456103,35.781659697871,-8.96637441288284));
#61262=CARTESIAN_POINT('Ctrl Pts',(14.3854209101992,35.7514135434756,-8.96888370787827));
#61263=CARTESIAN_POINT('Ctrl Pts',(13.5573153151024,35.7116818529589,-9.40474423377933));
#61264=CARTESIAN_POINT('Ctrl Pts',(13.8551377884079,35.6663146218422,-8.97542077741386));
#61265=CARTESIAN_POINT('Ctrl Pts',(14.3789710533313,35.6405136334663,-8.97725551630533));
#61266=CARTESIAN_POINT('Ctrl Pts',(13.5554500621166,35.670534598073,-9.40743230188023));
#61267=CARTESIAN_POINT('Ctrl Pts',(13.8533400041568,35.6277987228642,-8.97819335621356));
#61268=CARTESIAN_POINT('Ctrl Pts',(14.376992754778,35.6034811060435,-8.97982139943131));
#61269=CARTESIAN_POINT('Ctrl Pts',(13.5520471598156,35.5880922883365,-9.41233375306736));
#61270=CARTESIAN_POINT('Ctrl Pts',(13.8500601058613,35.5506254644722,-8.98324892780074));
#61271=CARTESIAN_POINT('Ctrl Pts',(14.3733836161508,35.5292830312532,-8.98450005753594));
#61272=CARTESIAN_POINT('Ctrl Pts',(13.5505083952296,35.546760927592,-9.41454874069695));
#61273=CARTESIAN_POINT('Ctrl Pts',(13.8485767969778,35.5119327236365,-8.98553376080348));
#61274=CARTESIAN_POINT('Ctrl Pts',(14.3717515931607,35.4920848085696,-8.98661436391861));
#61275=CARTESIAN_POINT('Ctrl Pts',(13.5436599334148,35.3402581736772,-9.4244027805627));
#61276=CARTESIAN_POINT('Ctrl Pts',(13.8419765765307,35.3186517971435,-8.99569616213354));
#61277=CARTESIAN_POINT('Ctrl Pts',(14.3644880734125,35.3062323400024,-8.99602049284851));
#61278=CARTESIAN_POINT('Ctrl Pts',(13.5408828403502,35.1756098619451,-9.42838755837681));
#61279=CARTESIAN_POINT('Ctrl Pts',(13.8392970574126,35.1644357229371,-8.99980993277378));
#61280=CARTESIAN_POINT('Ctrl Pts',(14.3615426717746,35.1580488673189,-8.99982414466763));
#61281=CARTESIAN_POINT('Ctrl Pts',(13.5405110292838,34.6832904888057,-9.4289215318621));
#61282=CARTESIAN_POINT('Ctrl Pts',(13.8389385644398,34.7034489893202,-9.0003608189815));
#61283=CARTESIAN_POINT('Ctrl Pts',(14.3611483267235,34.7149614551366,-9.00033384633901));
#61284=CARTESIAN_POINT('Ctrl Pts',(13.5508830762733,34.3572427818775,-9.41407821971699));
#61285=CARTESIAN_POINT('Ctrl Pts',(13.8489658444416,34.3977979636559,-8.98500808730318));
#61286=CARTESIAN_POINT('Ctrl Pts',(14.3721489822692,34.4215185342681,-8.98616523030746));
#61287=CARTESIAN_POINT('Ctrl Pts',(13.5919101658448,33.7093421596287,-9.3547463310013));
#61288=CARTESIAN_POINT('Ctrl Pts',(13.8884912540378,33.7915493337399,-8.92382970966888));
#61289=CARTESIAN_POINT('Ctrl Pts',(14.4156625599663,33.8384080055227,-8.92953024469643));
#61290=CARTESIAN_POINT('Ctrl Pts',(13.6225642332904,33.3874892491063,-9.31025704675605));
#61291=CARTESIAN_POINT('Ctrl Pts',(13.918075940792,33.4902694887766,-8.87786426091058));
#61292=CARTESIAN_POINT('Ctrl Pts',(14.4481744486006,33.5487404014116,-8.88706320021167));
#61293=CARTESIAN_POINT('Ctrl Pts',(13.6728215061252,32.9877546659562,-9.23603126196882));
#61294=CARTESIAN_POINT('Ctrl Pts',(13.9662896916563,33.1176686895628,-8.80158654504113));
#61295=CARTESIAN_POINT('Ctrl Pts',(14.5014776139512,33.1889792966578,-8.81621131403715));
#61296=CARTESIAN_POINT('Ctrl Pts',(13.6834694495751,32.9079370045103,-9.22025322157322));
#61297=CARTESIAN_POINT('Ctrl Pts',(13.9765194353422,33.04316387348,-8.78534664166924));
#61298=CARTESIAN_POINT('Ctrl Pts',(14.512770886892,33.1171434052856,-8.8011504571503));
#61299=CARTESIAN_POINT('Ctrl Pts',(13.7003208658972,32.7884041875066,-9.19517860529697));
#61300=CARTESIAN_POINT('Ctrl Pts',(13.9926934407437,32.9316762091749,-8.75955865151019));
#61301=CARTESIAN_POINT('Ctrl Pts',(14.5306436002406,33.0095638758911,-8.77721559591971));
#61302=CARTESIAN_POINT('Ctrl Pts',(13.7060845825789,32.7485921967665,-9.18658577875371));
#61303=CARTESIAN_POINT('Ctrl Pts',(13.9982261245286,32.8945388634974,-8.75071959428219));
#61304=CARTESIAN_POINT('Ctrl Pts',(14.5367566328563,32.9737330861968,-8.76901335232183));
#61305=CARTESIAN_POINT('Ctrl Pts',(13.7179025671362,32.6690327731066,-9.1689291639627));
#61306=CARTESIAN_POINT('Ctrl Pts',(14.0095670511447,32.8203417227802,-8.73256083164095));
#61307=CARTESIAN_POINT('Ctrl Pts',(14.5492908582467,32.9021296088266,-8.75215931076496));
#61308=CARTESIAN_POINT('Ctrl Pts',(13.7239585686921,32.6292758377139,-9.15986274004417));
#61309=CARTESIAN_POINT('Ctrl Pts',(14.0153773261073,32.7832719182194,-8.7232377974293));
#61310=CARTESIAN_POINT('Ctrl Pts',(14.5557138899543,32.866348368934,-8.74350499700366));
#61311=CARTESIAN_POINT('Ctrl Pts',(13.7548626759315,32.431249484037,-9.11349220398879));
#61312=CARTESIAN_POINT('Ctrl Pts',(14.0450499694982,32.5984782080405,-8.67551437811789));
#61313=CARTESIAN_POINT('Ctrl Pts',(14.5884909717086,32.68812466034,-8.69924221182081));
#61314=CARTESIAN_POINT('Ctrl Pts',(13.7816505762543,32.2747815938857,-9.07297363099581));
#61315=CARTESIAN_POINT('Ctrl Pts',(14.0707296805897,32.4527267404774,-8.63386437079738));
#61316=CARTESIAN_POINT('Ctrl Pts',(14.6169023800244,32.5473035669041,-8.66056539224569));
#61317=CARTESIAN_POINT('Ctrl Pts',(13.8676321749174,31.81095992879,-8.94146242624562));
#61318=CARTESIAN_POINT('Ctrl Pts',(14.1531401560041,32.0205075798369,-8.49864781023208));
#61319=CARTESIAN_POINT('Ctrl Pts',(14.7080949798849,32.1298640911792,-8.53503196772206));
#61320=CARTESIAN_POINT('Ctrl Pts',(13.9324346139195,31.5091733617932,-8.84054425749788));
#61321=CARTESIAN_POINT('Ctrl Pts',(14.2151101095553,31.7401896155852,-8.39501754289617));
#61322=CARTESIAN_POINT('Ctrl Pts',(14.7768248366031,31.858256196006,-8.43870098837303));
#61323=CARTESIAN_POINT('Ctrl Pts',(14.0741833838855,30.9193680769779,-8.61308998655124));
#61324=CARTESIAN_POINT('Ctrl Pts',(14.3499236459374,31.1943251121412,-8.16249577569527));
#61325=CARTESIAN_POINT('Ctrl Pts',(14.927164432396,31.3274314704435,-8.22158554640244));
#61326=CARTESIAN_POINT('Ctrl Pts',(14.1511326299876,30.6313511296127,-8.48655143147596));
#61327=CARTESIAN_POINT('Ctrl Pts',(14.4229773435497,30.9284342184197,-8.03318226008555));
#61328=CARTESIAN_POINT('Ctrl Pts',(15.0087772653985,31.0682162329507,-8.10079874377953));
#61329=CARTESIAN_POINT('Ctrl Pts',(14.2533131033264,30.2795421476305,-8.31232202503868));
#61330=CARTESIAN_POINT('Ctrl Pts',(14.5190087190408,30.6063167166278,-7.85672407191655));
#61331=CARTESIAN_POINT('Ctrl Pts',(15.1171504874915,30.7515881692275,-7.93448885616022));
#61332=CARTESIAN_POINT('Ctrl Pts',(14.2740494070183,30.2095920172121,-8.27667110983962));
#61333=CARTESIAN_POINT('Ctrl Pts',(14.5385522750191,30.5420833308275,-7.82050094551189));
#61334=CARTESIAN_POINT('Ctrl Pts',(15.1391435357377,30.6886330556848,-7.9004584371993));
#61335=CARTESIAN_POINT('Ctrl Pts',(14.3055755882552,30.1052800677474,-8.2219796808514));
#61336=CARTESIAN_POINT('Ctrl Pts',(14.5682064898189,30.4464618904594,-7.76502157216377));
#61337=CARTESIAN_POINT('Ctrl Pts',(15.1725803924368,30.5947523069326,-7.84825298230988));
#61338=CARTESIAN_POINT('Ctrl Pts',(14.3161507193771,30.0706249144069,-8.20355330284792));
#61339=CARTESIAN_POINT('Ctrl Pts',(14.5781545712646,30.4146890015269,-7.74632436847072));
#61340=CARTESIAN_POINT('Ctrl Pts',(15.1837964400011,30.5635626708233,-7.83066416704026));
#61341=CARTESIAN_POINT('Ctrl Pts',(14.3373878813408,30.0016749048532,-8.16638028459182));
#61342=CARTESIAN_POINT('Ctrl Pts',(14.5981197517123,30.3515071790422,-7.70862194354184));
#61343=CARTESIAN_POINT('Ctrl Pts',(15.2063207012272,30.5015076660714,-7.79518083140264));
#61344=CARTESIAN_POINT('Ctrl Pts',(14.3480555521587,29.9673613219152,-8.14762387652105));
#61345=CARTESIAN_POINT('Ctrl Pts',(14.6081424657647,30.3200808943631,-7.68960598698859));
#61346=CARTESIAN_POINT('Ctrl Pts',(15.2176348969313,30.4706254432956,-7.77727698747795));
#61347=CARTESIAN_POINT('Ctrl Pts',(14.4016253212505,29.796591116269,-8.05299667723724));
#61348=CARTESIAN_POINT('Ctrl Pts',(14.6585457278825,30.1634387265338,-7.59351316959592));
#61349=CARTESIAN_POINT('Ctrl Pts',(15.2744513150548,30.3169322675397,-7.68695102437855));
#61350=CARTESIAN_POINT('Ctrl Pts',(14.4452205721895,29.6625254514556,-7.97459247489173));
#61351=CARTESIAN_POINT('Ctrl Pts',(14.6993851879577,30.0409902873586,-7.51416748480995));
#61352=CARTESIAN_POINT('Ctrl Pts',(15.3206886998058,30.1962731766416,-7.61211065004841));
#61353=CARTESIAN_POINT('Ctrl Pts',(14.5777133703464,29.2676726547534,-7.73138816583178));
#61354=CARTESIAN_POINT('Ctrl Pts',(14.8234915893807,29.6801465523773,-7.26788478492355));
#61355=CARTESIAN_POINT('Ctrl Pts',(15.4612113551328,29.8409056814626,-7.37996108259175));
#61356=CARTESIAN_POINT('Ctrl Pts',(14.668309347519,29.0142068836985,-7.55861955891375));
#61357=CARTESIAN_POINT('Ctrl Pts',(14.907692286347,29.4503611487385,-7.09386429377839));
#61358=CARTESIAN_POINT('Ctrl Pts',(15.5572979917242,29.6127865022682,-7.21504559587684));
#61359=CARTESIAN_POINT('Ctrl Pts',(14.8515808217713,28.5257802291976,-7.19184092179889));
#61360=CARTESIAN_POINT('Ctrl Pts',(15.0767699379545,29.009999766832,-6.72666722324951));
#61361=CARTESIAN_POINT('Ctrl Pts',(15.7516768131561,29.1732025427066,-6.86493871876546));
#61362=CARTESIAN_POINT('Ctrl Pts',(14.9442617876913,28.2908215774306,-6.99783092564266));
#61363=CARTESIAN_POINT('Ctrl Pts',(15.1617270035886,28.7995023384666,-6.53309448498094));
#61364=CARTESIAN_POINT('Ctrl Pts',(15.8499748005742,28.9617397708295,-6.67974736165878));
#61365=CARTESIAN_POINT('Ctrl Pts',(15.0831691896633,27.9520228746188,-6.6903405523582));
#61366=CARTESIAN_POINT('Ctrl Pts',(15.2875727332987,28.4989406174798,-6.2294513637031));
#61367=CARTESIAN_POINT('Ctrl Pts',(15.997300820026,28.656820960667,-6.38623382970425));
#61368=CARTESIAN_POINT('Ctrl Pts',(15.1294538068838,27.8413684918233,-6.58509205486735));
#61369=CARTESIAN_POINT('Ctrl Pts',(15.3294819925269,28.4007955047577,-6.12542316901587));
#61370=CARTESIAN_POINT('Ctrl Pts',(16.0463905618979,28.5572320234826,-6.28576935691975));
#61371=CARTESIAN_POINT('Ctrl Pts',(15.1871165528599,27.7059137885866,-6.44998867645945));
#61372=CARTESIAN_POINT('Ctrl Pts',(15.3813309114973,28.2813976823567,-5.99268560044396));
#61373=CARTESIAN_POINT('Ctrl Pts',(16.1075480141302,28.4353227996728,-6.15680704431937));
#61374=CARTESIAN_POINT('Ctrl Pts',(15.1986427411563,27.6789586010782,-6.4227826599171));
#61375=CARTESIAN_POINT('Ctrl Pts',(15.3917112172421,28.2575974144608,-5.96590506721411));
#61376=CARTESIAN_POINT('Ctrl Pts',(16.1197727583312,28.4110631327084,-6.13083766552066));
#61377=CARTESIAN_POINT('Ctrl Pts',(15.22161650098,27.6254631882903,-6.36814489211147));
#61378=CARTESIAN_POINT('Ctrl Pts',(15.4123784799737,28.2104073796915,-5.91216422792328));
#61379=CARTESIAN_POINT('Ctrl Pts',(16.1441388650521,28.3629172647956,-6.07868343378511));
#61380=CARTESIAN_POINT('Ctrl Pts',(15.2330706037456,27.5989075417468,-6.34069797064005));
#61381=CARTESIAN_POINT('Ctrl Pts',(15.4226712022193,28.1870046176015,-5.88518855411238));
#61382=CARTESIAN_POINT('Ctrl Pts',(16.1562871548775,28.3390171846542,-6.05248410033579));
#61383=CARTESIAN_POINT('Ctrl Pts',(15.2673288583536,27.5198130564946,-6.25797352384566));
#61384=CARTESIAN_POINT('Ctrl Pts',(15.4534493940906,28.1173044903271,-5.80387679627119));
#61385=CARTESIAN_POINT('Ctrl Pts',(16.1926216640663,28.2678321532352,-5.97351985746979));
#61386=CARTESIAN_POINT('Ctrl Pts',(15.290028934829,27.4678465591937,-6.20231237797931));
#61387=CARTESIAN_POINT('Ctrl Pts',(15.4737789443219,28.0716437659571,-5.7492990645817));
#61388=CARTESIAN_POINT('Ctrl Pts',(16.2166975007587,28.2210623091367,-5.92038876513649));
#61389=CARTESIAN_POINT('Ctrl Pts',(15.4027606748132,27.2117871716814,-5.92145102020388));
#61390=CARTESIAN_POINT('Ctrl Pts',(15.5750557618011,27.8458706821111,-5.47287876127004));
#61391=CARTESIAN_POINT('Ctrl Pts',(16.336261456746,27.9906088770429,-5.65229383850497));
#61392=CARTESIAN_POINT('Ctrl Pts',(15.4904827104974,27.0189801350607,-5.68860317193879));
#61393=CARTESIAN_POINT('Ctrl Pts',(15.6526357170028,27.6784129519233,-5.24631783516924));
#61394=CARTESIAN_POINT('Ctrl Pts',(16.429299971196,27.8170825577775,-5.43002999028148));
#61395=CARTESIAN_POINT('Ctrl Pts',(15.6591637426249,26.656905604576,-5.20632802772958));
#61396=CARTESIAN_POINT('Ctrl Pts',(15.8004769809526,27.3661724733035,-4.7806667702281));
#61397=CARTESIAN_POINT('Ctrl Pts',(16.6082040777263,27.4912155066444,-4.96967645923575));
#61398=CARTESIAN_POINT('Ctrl Pts',(15.740127626065,26.4876389347608,-4.95690180582163));
#61399=CARTESIAN_POINT('Ctrl Pts',(15.8705932694381,27.2218129160782,-4.54154452839877));
#61400=CARTESIAN_POINT('Ctrl Pts',(16.6940748548538,27.3388755168911,-4.73158780209777));
#61401=CARTESIAN_POINT('Ctrl Pts',(15.8934770180544,26.1729335212289,-4.44070731669338));
#61402=CARTESIAN_POINT('Ctrl Pts',(16.0021812140351,26.9553860849679,-4.05065590845588));
#61403=CARTESIAN_POINT('Ctrl Pts',(16.8567181309159,27.0556406687916,-4.2388567198354));
#61404=CARTESIAN_POINT('Ctrl Pts',(15.9658678958422,26.0274910774788,-4.17394304589581));
#61405=CARTESIAN_POINT('Ctrl Pts',(16.063469476959,26.8337655896831,-3.79898706599225));
#61406=CARTESIAN_POINT('Ctrl Pts',(16.9334963265846,26.9247424816998,-3.9842181095779));
#61407=CARTESIAN_POINT('Ctrl Pts',(16.0497732597612,25.8612989242681,-3.82881501888285));
#61408=CARTESIAN_POINT('Ctrl Pts',(16.1335491117151,26.6964316563818,-3.4775371624284));
#61409=CARTESIAN_POINT('Ctrl Pts',(17.022486852709,26.7751695575831,-3.65477773800455));
#61410=CARTESIAN_POINT('Ctrl Pts',(16.0662245959121,25.8288433557414,-3.75920417681785));
#61411=CARTESIAN_POINT('Ctrl Pts',(16.1473132271782,26.6695565389256,-3.41252921961847));
#61412=CARTESIAN_POINT('Ctrl Pts',(17.0399352376671,26.745959548768,-3.58833102853059));
#61413=CARTESIAN_POINT('Ctrl Pts',(16.0903819375245,25.7813551666353,-3.65388920287835));
#61414=CARTESIAN_POINT('Ctrl Pts',(16.1674564707937,26.6303518394139,-3.314450412959));
#61415=CARTESIAN_POINT('Ctrl Pts',(17.0655566573174,26.7032201824222,-3.48780310422709));
#61416=CARTESIAN_POINT('Ctrl Pts',(16.098345616361,25.7657292707521,-3.61864269610625));
#61417=CARTESIAN_POINT('Ctrl Pts',(16.1740922821313,26.6174582718761,-3.28163420148606));
#61418=CARTESIAN_POINT('Ctrl Pts',(17.0740029824056,26.6891568774627,-3.45415871318928));
#61419=CARTESIAN_POINT('Ctrl Pts',(16.1140455830658,25.7349771707284,-3.54807574507184));
#61420=CARTESIAN_POINT('Ctrl Pts',(16.187157008452,26.5921127531103,-3.21599816456815));
#61421=CARTESIAN_POINT('Ctrl Pts',(17.0906544601812,26.6614799900588,-3.38679935442564));
#61422=CARTESIAN_POINT('Ctrl Pts',(16.1217882988379,25.7198383195558,-3.51272748888179));
#61423=CARTESIAN_POINT('Ctrl Pts',(16.1935907787688,26.5796514011833,-3.183153417088));
#61424=CARTESIAN_POINT('Ctrl Pts',(17.0988664304859,26.6478550252466,-3.35305783899775));
#61425=CARTESIAN_POINT('Ctrl Pts',(16.1599613732448,25.6453253627483,-3.33566278782528));
#61426=CARTESIAN_POINT('Ctrl Pts',(16.2253388524004,26.518251457348,-3.01842711386761));
#61427=CARTESIAN_POINT('Ctrl Pts',(17.1393530195516,26.5807933703941,-3.18404154235054));
#61428=CARTESIAN_POINT('Ctrl Pts',(16.1887703626542,25.5894928519857,-3.19297659606595));
#61429=CARTESIAN_POINT('Ctrl Pts',(16.2490907879542,26.4726133412268,-2.88653753270067));
#61430=CARTESIAN_POINT('Ctrl Pts',(17.1699080046339,26.5305441154266,-3.04784109434391));
#61431=CARTESIAN_POINT('Ctrl Pts',(16.2698459579849,25.4332047189377,-2.76182079317166));
#61432=CARTESIAN_POINT('Ctrl Pts',(16.3158320106216,26.3449718406617,-2.48834572470189));
#61433=CARTESIAN_POINT('Ctrl Pts',(17.255897261409,26.3898848090645,-2.63628330557435));
#61434=CARTESIAN_POINT('Ctrl Pts',(16.316765145617,25.3439309463016,-2.47026039537153));
#61435=CARTESIAN_POINT('Ctrl Pts',(16.3537805742651,26.2732399080745,-2.22215610964296));
#61436=CARTESIAN_POINT('Ctrl Pts',(17.3056600298758,26.3095384218259,-2.35797567052832));
#61437=CARTESIAN_POINT('Ctrl Pts',(16.3954028639435,25.1952391193477,-1.87876985450263));
#61438=CARTESIAN_POINT('Ctrl Pts',(16.417121596869,26.154131014951,-1.68483850356858));
#61439=CARTESIAN_POINT('Ctrl Pts',(17.3890636589622,26.1757157908581,-1.79337109958107));
#61440=CARTESIAN_POINT('Ctrl Pts',(16.4271241236573,25.1358193426336,-1.57884042903499));
#61441=CARTESIAN_POINT('Ctrl Pts',(16.4423268469724,26.1071199172671,-1.41447090107595));
#61442=CARTESIAN_POINT('Ctrl Pts',(17.4227074149731,26.1222379977279,-1.50707484923427));
#61443=CARTESIAN_POINT('Ctrl Pts',(16.4624867292185,25.0697740909849,-1.12241556867003));
#61444=CARTESIAN_POINT('Ctrl Pts',(16.4703739907714,26.0549329007231,-1.00461697464686));
#61445=CARTESIAN_POINT('Ctrl Pts',(17.4602132031594,26.0627972771039,-1.07139660369267));
#61446=CARTESIAN_POINT('Ctrl Pts',(16.472236231715,25.0516136052353,-0.96918375449722));
#61447=CARTESIAN_POINT('Ctrl Pts',(16.4780841724723,26.0406189166,-0.867184356346633));
#61448=CARTESIAN_POINT('Ctrl Pts',(17.4705535833765,26.0464528419075,-0.925129882160084));
#61449=CARTESIAN_POINT('Ctrl Pts',(16.483684081477,25.0303119318585,-0.737651684679333));
#61450=CARTESIAN_POINT('Ctrl Pts',(16.4871294638992,26.0238409108057,-0.65980157630425));
#61451=CARTESIAN_POINT('Ctrl Pts',(17.4826952403163,26.0272813376459,-0.704122012867659));
#61452=CARTESIAN_POINT('Ctrl Pts',(16.4869704992073,25.0242017345862,-0.660193474939691));
#61453=CARTESIAN_POINT('Ctrl Pts',(16.4897239001879,26.0190318513568,-0.590448368527771));
#61454=CARTESIAN_POINT('Ctrl Pts',(17.4861808345135,26.0217821608405,-0.630184636034853));
#61455=CARTESIAN_POINT('Ctrl Pts',(16.4904030883612,25.0178224283329,-0.563013510054482));
#61456=CARTESIAN_POINT('Ctrl Pts',(16.49243229442,26.0140133058613,-0.50348874580496));
#61457=CARTESIAN_POINT('Ctrl Pts',(17.4898214587776,26.0160407857062,-0.537421948832318));
#61458=CARTESIAN_POINT('Ctrl Pts',(16.4910558314609,25.0166095003478,-0.543559654133235));
#61459=CARTESIAN_POINT('Ctrl Pts',(16.4929473390123,26.0130590575589,-0.486079274150305));
#61460=CARTESIAN_POINT('Ctrl Pts',(17.4905137619999,26.0149491506782,-0.518852360396683));
#61461=CARTESIAN_POINT('Ctrl Pts',(16.4922934176736,25.0143100694522,-0.504616051390933));
#61462=CARTESIAN_POINT('Ctrl Pts',(16.4939237271056,26.0112502223663,-0.451231779951065));
#61463=CARTESIAN_POINT('Ctrl Pts',(17.4918263532193,26.0128796630442,-0.481678924038814));
#61464=CARTESIAN_POINT('Ctrl Pts',(16.492878650155,25.0132228433094,-0.485110633925368));
#61465=CARTESIAN_POINT('Ctrl Pts',(16.4943853634874,26.0103950931405,-0.433779992803541));
#61466=CARTESIAN_POINT('Ctrl Pts',(17.4924470542556,26.0119011596235,-0.463060117772013));
#61467=CARTESIAN_POINT('Ctrl Pts',(16.4945258261512,25.0101630686332,-0.4267689702364));
#61468=CARTESIAN_POINT('Ctrl Pts',(16.495684601932,26.00798859576,-0.381582487394922));
#61469=CARTESIAN_POINT('Ctrl Pts',(17.4941940588796,26.0091473627552,-0.407370351815588));
#61470=CARTESIAN_POINT('Ctrl Pts',(16.4954853336232,25.0083811132544,-0.387907202711105));
#61471=CARTESIAN_POINT('Ctrl Pts',(16.4964411138925,26.0065876292943,-0.346823188777901));
#61472=CARTESIAN_POINT('Ctrl Pts',(17.4952117181403,26.0075436030163,-0.370275030893979));
#61473=CARTESIAN_POINT('Ctrl Pts',(16.4995936624279,25.0007522824497,-0.193760702128921));
#61474=CARTESIAN_POINT('Ctrl Pts',(16.4996807717234,26.0005888276808,-0.173146702174422));
#61475=CARTESIAN_POINT('Ctrl Pts',(17.4995690360396,26.0006776561714,-0.184953384322929));
#61476=CARTESIAN_POINT('Ctrl Pts',(16.5006753927425,24.9987456794828,-0.0389627034907101));
#61477=CARTESIAN_POINT('Ctrl Pts',(16.5005316011594,25.9990147346703,-0.0348510197095155));
#61478=CARTESIAN_POINT('Ctrl Pts',(17.5007163254734,25.9988717134746,-0.037191668888471));
#61479=CARTESIAN_POINT('Ctrl Pts',(16.4985185160909,25.0027491746321,0.269616919228709));
#61480=CARTESIAN_POINT('Ctrl Pts',(16.4988321329034,26.0021605183102,0.241013621938643));
#61481=CARTESIAN_POINT('Ctrl Pts',(17.498428729471,26.0024748589104,0.257361586454653));
#61482=CARTESIAN_POINT('Ctrl Pts',(16.4952798552968,25.0087594435861,0.42339852392335));
#61483=CARTESIAN_POINT('Ctrl Pts',(16.4962832364797,26.0068778358239,0.378456519338701));
#61484=CARTESIAN_POINT('Ctrl Pts',(17.4949937865805,26.0078841002541,0.404153107768947));
#61485=CARTESIAN_POINT('Ctrl Pts',(16.4845588751127,25.0286833763451,0.729960620582834));
#61486=CARTESIAN_POINT('Ctrl Pts',(16.4878225611123,26.0225547920612,0.65283101053216));
#61487=CARTESIAN_POINT('Ctrl Pts',(17.4836230517336,26.0258156379645,0.696780543053585));
#61488=CARTESIAN_POINT('Ctrl Pts',(16.4770765097712,25.042597132783,0.882741101116753));
#61489=CARTESIAN_POINT('Ctrl Pts',(16.4819182165634,26.0335005894375,0.789640705789399));
#61490=CARTESIAN_POINT('Ctrl Pts',(17.4756872107313,26.0383380173717,0.842616446032084));
#61491=CARTESIAN_POINT('Ctrl Pts',(16.457933564706,25.0782732358425,1.18730995963222));
#61492=CARTESIAN_POINT('Ctrl Pts',(16.4667568417188,26.0616602772347,1.06294377615386));
#61493=CARTESIAN_POINT('Ctrl Pts',(17.4553840901105,26.0704465068189,1.1333412453569));
#61494=CARTESIAN_POINT('Ctrl Pts',(16.4462729445412,25.1000356045573,1.33909833326507));
#61495=CARTESIAN_POINT('Ctrl Pts',(16.457512962125,26.0788495239333,1.19931940286108));
#61496=CARTESIAN_POINT('Ctrl Pts',(17.4430167673428,26.0900326366225,1.27823013746166));
#61497=CARTESIAN_POINT('Ctrl Pts',(16.4188289862862,25.1514109395644,1.64168597230913));
#61498=CARTESIAN_POINT('Ctrl Pts',(16.4356580866948,26.1195950064352,1.4719247367756));
#61499=CARTESIAN_POINT('Ctrl Pts',(17.4139095429865,26.1362704333346,1.56706377336382));
#61500=CARTESIAN_POINT('Ctrl Pts',(16.4030456111901,25.1810238589603,1.7924852401837));
#61501=CARTESIAN_POINT('Ctrl Pts',(16.4230656732971,26.1431161224906,1.60804089841558));
#61502=CARTESIAN_POINT('Ctrl Pts',(17.3971696019414,26.1629220581204,1.7110085193938));
#61503=CARTESIAN_POINT('Ctrl Pts',(16.3763135366034,25.231375580585,2.01794006740895));
#61504=CARTESIAN_POINT('Ctrl Pts',(16.4016055889564,26.1833366410978,1.81239942992283));
#61505=CARTESIAN_POINT('Ctrl Pts',(17.3688174054951,26.2082386029367,1.92621538597846));
#61506=CARTESIAN_POINT('Ctrl Pts',(16.3668932777758,25.2491486628916,2.09296761713974));
#61507=CARTESIAN_POINT('Ctrl Pts',(16.3940375747528,26.1975406923544,1.88043508573692));
#61508=CARTESIAN_POINT('Ctrl Pts',(17.3588262232113,26.2242343754568,1.99783258786826));
#61509=CARTESIAN_POINT('Ctrl Pts',(16.3520023700009,25.2773017719863,2.20532214078148));
#61510=CARTESIAN_POINT('Ctrl Pts',(16.3820388971085,26.2201011771275,1.98254008226397));
#61511=CARTESIAN_POINT('Ctrl Pts',(17.3430328383105,26.2495721710511,2.10508008086908));
#61512=CARTESIAN_POINT('Ctrl Pts',(16.3469119771516,25.2869350853555,2.24274251216562));
#61513=CARTESIAN_POINT('Ctrl Pts',(16.3779351975318,26.2278235718406,2.01655526539809));
#61514=CARTESIAN_POINT('Ctrl Pts',(17.3376339375129,26.2582421522511,2.1407995239869));
#61515=CARTESIAN_POINT('Ctrl Pts',(16.3364782736115,25.3067015799831,2.31752082632262));
#61516=CARTESIAN_POINT('Ctrl Pts',(16.369513853826,26.2436857621179,2.0845855843958));
#61517=CARTESIAN_POINT('Ctrl Pts',(17.3265678897919,26.2760319955966,2.21217881933827));
#61518=CARTESIAN_POINT('Ctrl Pts',(16.3311312276683,25.3168418552601,2.35490405296875));
#61519=CARTESIAN_POINT('Ctrl Pts',(16.3651936132304,26.2518304450527,2.11862215055674));
#61520=CARTESIAN_POINT('Ctrl Pts',(17.3208967811602,26.285158242412,2.24786280615268));
#61521=CARTESIAN_POINT('Ctrl Pts',(16.2819566384181,25.4102034773501,2.69049912871399));
#61522=CARTESIAN_POINT('Ctrl Pts',(16.3255665769557,26.3266105865415,2.42325772140721));
#61523=CARTESIAN_POINT('Ctrl Pts',(17.2687419212362,26.3691836940896,2.56820353924912));
#61524=CARTESIAN_POINT('Ctrl Pts',(16.2309920113021,25.5076777154244,2.9814187974019));
#61525=CARTESIAN_POINT('Ctrl Pts',(16.2841214219777,26.4053051020533,2.6899166416278));
#61526=CARTESIAN_POINT('Ctrl Pts',(17.2146886258162,26.4569103521462,2.84589917037985));
#61527=CARTESIAN_POINT('Ctrl Pts',(16.1736472161052,25.6188908313694,3.26544571674037));
#61528=CARTESIAN_POINT('Ctrl Pts',(16.2365230528882,26.4968270314871,2.95402066052848));
#61529=CARTESIAN_POINT('Ctrl Pts',(17.1538683056082,26.5570022944821,3.11701616046811));
#61530=CARTESIAN_POINT('Ctrl Pts',(16.4590359785375,20.1091944935103,0.023011592823693));
#61531=CARTESIAN_POINT('Ctrl Pts',(16.4271965341628,20.1902603108686,1.05278036905647));
#61532=CARTESIAN_POINT('Ctrl Pts',(17.3953642409772,20.5502649459156,1.02026723798077));
#61533=CARTESIAN_POINT('Ctrl Pts',(16.5316577284859,19.9154749454276,0.0395707565384078));
#61534=CARTESIAN_POINT('Ctrl Pts',(16.4879246572657,20.0254557281703,1.07950524961033));
#61535=CARTESIAN_POINT('Ctrl Pts',(17.4679845765535,20.3888322238513,1.03484672596902));
#61536=CARTESIAN_POINT('Ctrl Pts',(16.6034030152266,19.724010227151,0.0649122476643638));
#61537=CARTESIAN_POINT('Ctrl Pts',(16.5465862722544,19.8645616579358,1.1140637205542));
#61538=CARTESIAN_POINT('Ctrl Pts',(17.5397268922733,20.2292780573011,1.05715075962855));
#61539=CARTESIAN_POINT('Ctrl Pts',(16.744970961061,19.3454312478812,0.132696775849498));
#61540=CARTESIAN_POINT('Ctrl Pts',(16.6602111583784,19.5489225084427,1.19790262588923));
#61541=CARTESIAN_POINT('Ctrl Pts',(17.6812725629732,19.9137955745397,1.11677044650688));
#61542=CARTESIAN_POINT('Ctrl Pts',(16.8147959023614,19.15831105953,0.175140612617222));
#61543=CARTESIAN_POINT('Ctrl Pts',(16.7151746590028,19.3941162803857,1.24743104684572));
#61544=CARTESIAN_POINT('Ctrl Pts',(17.7510782956021,19.757862084349,1.15408688832136));
#61545=CARTESIAN_POINT('Ctrl Pts',(16.9521986924116,18.78829106961,0.277198432090005));
#61546=CARTESIAN_POINT('Ctrl Pts',(16.8209509865544,19.0909503211262,1.36068099990159));
#61547=CARTESIAN_POINT('Ctrl Pts',(17.8884066526975,19.4495120925816,1.24376538253356));
#61548=CARTESIAN_POINT('Ctrl Pts',(17.0197775730774,18.6053910460792,0.33681026323465));
#61549=CARTESIAN_POINT('Ctrl Pts',(16.871742873146,18.9425660229543,1.42466616590782));
#61550=CARTESIAN_POINT('Ctrl Pts',(17.9559303491669,19.2970954065821,1.29612559894816));
#61551=CARTESIAN_POINT('Ctrl Pts',(17.1190709679907,18.3341847189676,0.439566509587872));
#61552=CARTESIAN_POINT('Ctrl Pts',(16.9440617016846,18.7260133044026,1.53064143694302));
#61553=CARTESIAN_POINT('Ctrl Pts',(18.0550933334177,19.0710901337005,1.38633699361548));
#61554=CARTESIAN_POINT('Ctrl Pts',(17.1518213623139,18.2443072781152,0.476046143457168));
#61555=CARTESIAN_POINT('Ctrl Pts',(16.9676606711903,18.6543970536208,1.5678998215709));
#61556=CARTESIAN_POINT('Ctrl Pts',(18.0877922559576,18.9961922665532,1.41835657614485));
#61557=CARTESIAN_POINT('Ctrl Pts',(17.2003606779556,18.1102824927287,0.53420980976954));
#61558=CARTESIAN_POINT('Ctrl Pts',(17.002019006833,18.5485258471271,1.62629031883017));
#61559=CARTESIAN_POINT('Ctrl Pts',(18.1362391230538,18.8845049451975,1.46939781628312));
#61560=CARTESIAN_POINT('Ctrl Pts',(17.2164426130913,18.0657395120991,0.554172071041801));
#61561=CARTESIAN_POINT('Ctrl Pts',(17.0133328640638,18.5133846587384,1.64623854105085));
#61562=CARTESIAN_POINT('Ctrl Pts',(18.1522876971816,18.8473857948172,1.48691383709229));
#61563=CARTESIAN_POINT('Ctrl Pts',(17.2483983308808,17.9769188381794,0.595266832712274));
#61564=CARTESIAN_POINT('Ctrl Pts',(17.0356241199857,18.4435548304955,1.6870145481646));
#61565=CARTESIAN_POINT('Ctrl Pts',(18.1841709974958,18.7733685663955,1.5229689425839));
#61566=CARTESIAN_POINT('Ctrl Pts',(17.2642156130721,17.9327979927603,0.616327327634305));
#61567=CARTESIAN_POINT('Ctrl Pts',(17.0465605940939,18.408991549976,1.70777441346281));
#61568=CARTESIAN_POINT('Ctrl Pts',(18.199949347906,18.7366011952906,1.54144485057487));
#61569=CARTESIAN_POINT('Ctrl Pts',(17.3423810485448,17.7139016011755,0.724053234204549));
#61570=CARTESIAN_POINT('Ctrl Pts',(17.1004716187916,18.2370235580736,1.81391718075492));
#61571=CARTESIAN_POINT('Ctrl Pts',(18.2779055045962,18.5541875356366,1.63594086850669));
#61572=CARTESIAN_POINT('Ctrl Pts',(17.4020798909505,17.543948296683,0.818101992014677));
#61573=CARTESIAN_POINT('Ctrl Pts',(17.1397482995283,18.1064705157127,1.90384392042449));
#61574=CARTESIAN_POINT('Ctrl Pts',(18.3373901375251,18.4125597820159,1.71840946033613));
#61575=CARTESIAN_POINT('Ctrl Pts',(17.5151946090821,17.2141267403257,1.02191071411103));
#61576=CARTESIAN_POINT('Ctrl Pts',(17.2111122741965,17.8569602745908,2.09328504050278));
#61577=CARTESIAN_POINT('Ctrl Pts',(18.4499480234508,18.1377084848054,1.89705572630751));
#61578=CARTESIAN_POINT('Ctrl Pts',(17.5686124281954,17.0542582812458,1.13166952369181));
#61579=CARTESIAN_POINT('Ctrl Pts',(17.2430573179698,17.7382644719926,2.19292283456572));
#61580=CARTESIAN_POINT('Ctrl Pts',(18.5030233178418,18.0044847693226,1.99323241936555));
#61581=CARTESIAN_POINT('Ctrl Pts',(17.6682752987396,16.7446855460758,1.36740039352683));
#61582=CARTESIAN_POINT('Ctrl Pts',(17.2994473380135,17.5122427624059,2.4008695734411));
#61583=CARTESIAN_POINT('Ctrl Pts',(18.6018307891431,17.7465074894261,2.19972574330706));
#61584=CARTESIAN_POINT('Ctrl Pts',(17.7145243522751,16.594979202804,1.49336803899043));
#61585=CARTESIAN_POINT('Ctrl Pts',(17.3237386272113,17.4052155445271,2.50922972451975));
#61586=CARTESIAN_POINT('Ctrl Pts',(18.6475671361265,17.6217522041873,2.31003851895677));
#61587=CARTESIAN_POINT('Ctrl Pts',(17.7670709494956,16.4144680486652,1.66165226591233));
#61588=CARTESIAN_POINT('Ctrl Pts',(17.3490690346078,17.2791176138107,2.64887744438743));
#61589=CARTESIAN_POINT('Ctrl Pts',(18.6993332924172,17.4713262417462,2.45736893303087));
#61590=CARTESIAN_POINT('Ctrl Pts',(17.7773159546806,16.3786978765719,1.69585204953799));
#61591=CARTESIAN_POINT('Ctrl Pts',(17.3539160552592,17.2541015552392,2.6772316437113));
#61592=CARTESIAN_POINT('Ctrl Pts',(18.7094151971177,17.4415177652829,2.48730848910089));
#61593=CARTESIAN_POINT('Ctrl Pts',(17.7922687108733,16.325548896176,1.74798467850413));
#61594=CARTESIAN_POINT('Ctrl Pts',(17.3608049212334,17.2171380154186,2.72009853858696));
#61595=CARTESIAN_POINT('Ctrl Pts',(18.7241120427853,17.3972269480623,2.53294423139505));
#61596=CARTESIAN_POINT('Ctrl Pts',(17.7971838211124,16.3079169628778,1.76550107196727));
#61597=CARTESIAN_POINT('Ctrl Pts',(17.36304058461,17.2048927323774,2.73446477736455));
#61598=CARTESIAN_POINT('Ctrl Pts',(18.7289399725856,17.3825336704678,2.54827723569099));
#61599=CARTESIAN_POINT('Ctrl Pts',(17.8068724998976,16.2728234255862,1.80081496910026));
#61600=CARTESIAN_POINT('Ctrl Pts',(17.3673860983665,17.1805763928498,2.76332308063254));
#61601=CARTESIAN_POINT('Ctrl Pts',(18.7384504053793,17.3532890558995,2.57918840373732));
#61602=CARTESIAN_POINT('Ctrl Pts',(17.8116492768538,16.2553497222102,1.81862527130614));
#61603=CARTESIAN_POINT('Ctrl Pts',(17.369496984659,17.1684977611069,2.77782524857301));
#61604=CARTESIAN_POINT('Ctrl Pts',(18.7431360490359,17.338727636486,2.59477776943123));
#61605=CARTESIAN_POINT('Ctrl Pts',(17.835091711741,16.1687058794947,1.90808130716663));
#61606=CARTESIAN_POINT('Ctrl Pts',(17.3797315284296,17.1085643067264,2.85061578024528));
#61607=CARTESIAN_POINT('Ctrl Pts',(18.7661143769998,17.2665244342873,2.67307644354688));
#61608=CARTESIAN_POINT('Ctrl Pts',(17.8524871153197,16.1015191310896,1.9811249412165));
#61609=CARTESIAN_POINT('Ctrl Pts',(17.3867870687763,17.0626954637632,2.90902060208184));
#61610=CARTESIAN_POINT('Ctrl Pts',(18.7831105947819,17.2105354772255,2.73700263540102));
#61611=CARTESIAN_POINT('Ctrl Pts',(17.9004839498672,15.9062454260188,2.20464101652785));
#61612=CARTESIAN_POINT('Ctrl Pts',(17.4049013625984,16.9298674264324,3.08585335220375));
#61613=CARTESIAN_POINT('Ctrl Pts',(18.8298189469103,17.047807389685,2.93259943046952));
#61614=CARTESIAN_POINT('Ctrl Pts',(17.9269071636239,15.7844281968184,2.35948710426806));
#61615=CARTESIAN_POINT('Ctrl Pts',(17.4126737657556,16.8489775129713,3.2043514593929));
#61616=CARTESIAN_POINT('Ctrl Pts',(18.8552622062664,16.9462930322008,3.06807804330981));
#61617=CARTESIAN_POINT('Ctrl Pts',(17.9575346714358,15.614170143894,2.60051765040973));
#61618=CARTESIAN_POINT('Ctrl Pts',(17.4186455070294,16.7368756953305,3.38350954430276));
#61619=CARTESIAN_POINT('Ctrl Pts',(18.8842055180459,16.8044113211377,3.27893177721889));
#61620=CARTESIAN_POINT('Ctrl Pts',(17.9662399299004,15.5594996501156,2.68232428765808));
#61621=CARTESIAN_POINT('Ctrl Pts',(17.4196743615776,16.7009605910879,3.44366696183719));
#61622=CARTESIAN_POINT('Ctrl Pts',(18.8923136078949,16.7588525765766,3.35049154672856));
#61623=CARTESIAN_POINT('Ctrl Pts',(17.9804993640783,15.4543610677294,2.8489005711619));
#61624=CARTESIAN_POINT('Ctrl Pts',(17.4198882444818,16.6319204969828,3.5646923241279));
#61625=CARTESIAN_POINT('Ctrl Pts',(18.9053007953748,16.6712370909416,3.49619525754758));
#61626=CARTESIAN_POINT('Ctrl Pts',(17.986053674335,15.4038928976034,2.93367015391985));
#61627=CARTESIAN_POINT('Ctrl Pts',(17.4190642517473,16.5988418210516,3.625506476283));
#61628=CARTESIAN_POINT('Ctrl Pts',(18.9101800346347,16.629180282881,3.57033914248333));
#61629=CARTESIAN_POINT('Ctrl Pts',(17.993840269328,15.3072328393525,3.10623404351813));
#61630=CARTESIAN_POINT('Ctrl Pts',(17.4156152191415,16.5352552788028,3.74801297800127));
#61631=CARTESIAN_POINT('Ctrl Pts',(18.9165314277074,16.5486302338962,3.7212669995102));
#61632=CARTESIAN_POINT('Ctrl Pts',(17.9960727385546,15.2610408122494,3.19402824639033));
#61633=CARTESIAN_POINT('Ctrl Pts',(17.4129850963717,16.5047904497612,3.80964503225668));
#61634=CARTESIAN_POINT('Ctrl Pts',(18.9180037747939,16.5101368784898,3.79805087941676));
#61635=CARTESIAN_POINT('Ctrl Pts',(17.9967772718942,15.1950447530921,3.32805498011324));
#61636=CARTESIAN_POINT('Ctrl Pts',(17.4076993677159,16.4609072677679,3.90287558319925));
#61637=CARTESIAN_POINT('Ctrl Pts',(18.9174982244806,16.4551401620879,3.91526698385196));
#61638=CARTESIAN_POINT('Ctrl Pts',(17.996571056543,15.1735921344216,3.37312636457799));
#61639=CARTESIAN_POINT('Ctrl Pts',(17.4057109865791,16.4465714494365,3.93411056442095));
#61640=CARTESIAN_POINT('Ctrl Pts',(18.916876930227,16.4372629798948,3.95468481362002));
#61641=CARTESIAN_POINT('Ctrl Pts',(17.9952480179863,15.131814858786,3.46403649967884));
#61642=CARTESIAN_POINT('Ctrl Pts',(17.4012829714188,16.4184858944737,3.99688191374779));
#61643=CARTESIAN_POINT('Ctrl Pts',(18.9146995251255,16.4024485837588,4.03419118394147));
#61644=CARTESIAN_POINT('Ctrl Pts',(17.9941350799946,15.1116102126343,3.50961367764491));
#61645=CARTESIAN_POINT('Ctrl Pts',(17.3988562915068,16.4048217541979,4.02822857708018));
#61646=CARTESIAN_POINT('Ctrl Pts',(18.9131497582954,16.3856113784195,4.07405096435664));
#61647=CARTESIAN_POINT('Ctrl Pts',(17.9894447446815,15.0530145947759,3.64670240077642));
#61648=CARTESIAN_POINT('Ctrl Pts',(17.3909482301197,16.3648708917027,4.12228170075606));
#61649=CARTESIAN_POINT('Ctrl Pts',(18.907119450644,16.3367816971689,4.19394263224871));
#61650=CARTESIAN_POINT('Ctrl Pts',(17.98451648757,15.0166405335387,3.73857085294315));
#61651=CARTESIAN_POINT('Ctrl Pts',(17.3848513030829,16.3396865216089,4.18485667628148));
#61652=CARTESIAN_POINT('Ctrl Pts',(18.9012585754435,16.3064699791306,4.27428659583135));
#61653=CARTESIAN_POINT('Ctrl Pts',(17.9710553602389,14.9491283812115,3.92321824386789));
#61654=CARTESIAN_POINT('Ctrl Pts',(17.3710242878969,16.2918598145745,4.31030626208985));
#61655=CARTESIAN_POINT('Ctrl Pts',(18.8858504484229,16.2502098524752,4.4357735571199));
#61656=CARTESIAN_POINT('Ctrl Pts',(17.9625224589627,14.9179904470399,4.01599722125423));
#61657=CARTESIAN_POINT('Ctrl Pts',(17.3633020844883,16.2692492133529,4.37310190417037));
#61658=CARTESIAN_POINT('Ctrl Pts',(18.8763031679861,16.2242615737717,4.51691658730071));
#61659=CARTESIAN_POINT('Ctrl Pts',(17.9418292246949,14.860850901726,4.20243289837371));
#61660=CARTESIAN_POINT('Ctrl Pts',(17.3461928936806,16.2263988612261,4.49936190571207));
#61661=CARTESIAN_POINT('Ctrl Pts',(18.8534959064239,16.1766452861806,4.67997604966665));
#61662=CARTESIAN_POINT('Ctrl Pts',(17.9296688867409,14.8348493881004,4.29608962464074));
#61663=CARTESIAN_POINT('Ctrl Pts',(17.3368180429497,16.2061847160273,4.56274563312786));
#61664=CARTESIAN_POINT('Ctrl Pts',(18.8402359231131,16.1549773580455,4.76189250375669));
#61665=CARTESIAN_POINT('Ctrl Pts',(17.9016776590665,14.7879225853875,4.48425565734379));
#61666=CARTESIAN_POINT('Ctrl Pts',(17.3163113352066,16.1680417453508,4.69056595942866));
#61667=CARTESIAN_POINT('Ctrl Pts',(18.8099562188662,16.1158716891751,4.92647998774823));
#61668=CARTESIAN_POINT('Ctrl Pts',(17.8858467886268,14.7669973432221,4.57876498035805));
#61669=CARTESIAN_POINT('Ctrl Pts',(17.3051961155725,16.1501327045764,4.75491912530884));
#61670=CARTESIAN_POINT('Ctrl Pts',(18.7929365204291,16.0984339873699,5.00915103077204));
#61671=CARTESIAN_POINT('Ctrl Pts',(17.8504508492249,14.7302004084719,4.76861805064328));
#61672=CARTESIAN_POINT('Ctrl Pts',(17.2810567878328,16.1165998124299,4.88506415276689));
#61673=CARTESIAN_POINT('Ctrl Pts',(18.7550693416422,16.0677698750224,5.17523515457135));
#61674=CARTESIAN_POINT('Ctrl Pts',(17.8308858240908,14.7143287162555,4.86396180571914));
#61675=CARTESIAN_POINT('Ctrl Pts',(17.2680543324973,16.1009898507806,4.95076863804019));
#61676=CARTESIAN_POINT('Ctrl Pts',(18.7342219089113,16.0545434649538,5.25864824062171));
#61677=CARTESIAN_POINT('Ctrl Pts',(17.8040424705567,14.697656351034,4.98365580793276));
#61678=CARTESIAN_POINT('Ctrl Pts',(17.2504475689671,16.0829273849491,5.03417381304885));
#61679=CARTESIAN_POINT('Ctrl Pts',(18.7057139554211,16.0406498271644,5.3633742964716));
#61680=CARTESIAN_POINT('Ctrl Pts',(17.7985497183264,14.6944778990153,5.00764015025094));
#61681=CARTESIAN_POINT('Ctrl Pts',(17.2468638075045,16.0793928106346,5.05089349630703));
#61682=CARTESIAN_POINT('Ctrl Pts',(18.6998849211899,16.0380011170706,5.38435984131314));
#61683=CARTESIAN_POINT('Ctrl Pts',(17.7873487605497,14.6884515573287,5.05555431987132));
#61684=CARTESIAN_POINT('Ctrl Pts',(17.2395772081921,16.0724898364934,5.08437341715332));
#61685=CARTESIAN_POINT('Ctrl Pts',(18.6880066539913,16.0329791658634,5.42628425816146));
#61686=CARTESIAN_POINT('Ctrl Pts',(17.7816428554264,14.6856044510824,5.07947529630174));
#61687=CARTESIAN_POINT('Ctrl Pts',(17.2358762620874,16.0691226166571,5.10112607282942));
#61688=CARTESIAN_POINT('Ctrl Pts',(18.6819598521156,16.0306065771309,5.44721538470061));
#61689=CARTESIAN_POINT('Ctrl Pts',(17.7642114493362,14.677554866839,5.15113069843371));
#61690=CARTESIAN_POINT('Ctrl Pts',(17.2246034389948,16.0592795749159,5.15140072438751));
#61691=CARTESIAN_POINT('Ctrl Pts',(18.6634990155104,16.0238985905457,5.50991628113862));
#61692=CARTESIAN_POINT('Ctrl Pts',(17.7521723027935,14.6728440185356,5.19875761220163));
#61693=CARTESIAN_POINT('Ctrl Pts',(17.2168497938318,16.0530497158324,5.18499631250327));
#61694=CARTESIAN_POINT('Ctrl Pts',(18.650764595348,16.0199728832643,5.55159358109326));
#61695=CARTESIAN_POINT('Ctrl Pts',(17.7148192143042,14.6606304582502,5.34121409400244));
#61696=CARTESIAN_POINT('Ctrl Pts',(17.1928855233917,16.0353963778912,5.28589380831356));
#61697=CARTESIAN_POINT('Ctrl Pts',(18.6112985955892,16.009794916877,5.67626117295854));
#61698=CARTESIAN_POINT('Ctrl Pts',(17.6882702666085,14.6550452532322,5.43561962007091));
#61699=CARTESIAN_POINT('Ctrl Pts',(17.1759265998257,16.0249547390621,5.35353548466019));
#61700=CARTESIAN_POINT('Ctrl Pts',(18.5833049272282,16.0051405787367,5.75888734807405));
#61701=CARTESIAN_POINT('Ctrl Pts',(17.6319631314318,14.6487737552932,5.62332507276344));
#61702=CARTESIAN_POINT('Ctrl Pts',(17.1398746928238,16.0068264974026,5.48975029904835));
#61703=CARTESIAN_POINT('Ctrl Pts',(18.5240352467465,15.9999143310151,5.92319341230171));
#61704=CARTESIAN_POINT('Ctrl Pts',(17.6022048520147,14.6480876974245,5.71662496962117));
#61705=CARTESIAN_POINT('Ctrl Pts',(17.1208140006137,15.9991314162458,5.55824749460516));
#61706=CARTESIAN_POINT('Ctrl Pts',(18.4927591427342,15.9993426156233,6.0048732741055));
#61707=CARTESIAN_POINT('Ctrl Pts',(17.5082133108841,14.6531225803452,5.99489420103241));
#61708=CARTESIAN_POINT('Ctrl Pts',(17.0604058020015,15.9804134812741,5.76457570444654));
#61709=CARTESIAN_POINT('Ctrl Pts',(18.3941027932187,16.0035383520529,6.24852182898731));
#61710=CARTESIAN_POINT('Ctrl Pts',(17.4392709397385,14.6659198618794,6.17823569450356));
#61711=CARTESIAN_POINT('Ctrl Pts',(17.0156031963545,15.9734934665474,5.90440046372606));
#61712=CARTESIAN_POINT('Ctrl Pts',(18.3219022319539,16.0142027526621,6.40910175786889));
#61713=CARTESIAN_POINT('Ctrl Pts',(17.345440413842,14.6931450787676,6.40474884759392));
#61714=CARTESIAN_POINT('Ctrl Pts',(16.9524570790435,15.9727945398665,6.08359523647655));
#61715=CARTESIAN_POINT('Ctrl Pts',(18.2238061082988,16.0368904336869,6.60756858482206));
#61716=CARTESIAN_POINT('Ctrl Pts',(17.3262910773468,14.6991528841241,6.44991808472345));
#61717=CARTESIAN_POINT('Ctrl Pts',(16.9395918709281,15.9730468738618,6.11932400679305));
#61718=CARTESIAN_POINT('Ctrl Pts',(18.2037939992296,16.0418969380489,6.64714886601801));
#61719=CARTESIAN_POINT('Ctrl Pts',(17.2969942022215,14.7090018589149,6.51747218845496));
#61720=CARTESIAN_POINT('Ctrl Pts',(16.91976284683,15.9740345866775,6.17319709455581));
#61721=CARTESIAN_POINT('Ctrl Pts',(18.1731883149322,16.0501044171085,6.70635021441229));
#61722=CARTESIAN_POINT('Ctrl Pts',(17.2871349117687,14.7124239673732,6.53995233222814));
#61723=CARTESIAN_POINT('Ctrl Pts',(16.9130785924152,15.9744641578401,6.19116453544277));
#61724=CARTESIAN_POINT('Ctrl Pts',(18.1628903970445,16.0529561740322,6.72605178979342));
#61725=CARTESIAN_POINT('Ctrl Pts',(17.2672775991108,14.7195269072644,6.58473078371382));
#61726=CARTESIAN_POINT('Ctrl Pts',(16.8995745934923,15.9755246869321,6.22707698730837));
#61727=CARTESIAN_POINT('Ctrl Pts',(18.142153205609,16.0588752908132,6.76529760601478));
#61728=CARTESIAN_POINT('Ctrl Pts',(17.2572733605126,14.7232097949335,6.6070435056052));
#61729=CARTESIAN_POINT('Ctrl Pts',(16.8927512736487,15.9761553190149,6.24503272312702));
#61730=CARTESIAN_POINT('Ctrl Pts',(18.1317074372765,16.0619443636701,6.78485447850158));
#61731=CARTESIAN_POINT('Ctrl Pts',(17.2068788594663,14.7422717582395,6.7182295014901));
#61732=CARTESIAN_POINT('Ctrl Pts',(16.8583978923929,15.9798004972284,6.33448629417914));
#61733=CARTESIAN_POINT('Ctrl Pts',(18.0790973420651,16.0778293335824,6.88231301093151));
#61734=CARTESIAN_POINT('Ctrl Pts',(17.1653693899747,14.7595916588526,6.80597077954413));
#61735=CARTESIAN_POINT('Ctrl Pts',(16.8296806545478,15.9843227083645,6.40628853128631));
#61736=CARTESIAN_POINT('Ctrl Pts',(18.0357899748907,16.0922625833738,6.95923792167927));
#61737=CARTESIAN_POINT('Ctrl Pts',(17.0374181157849,14.8174391690287,7.06573918620837));
#61738=CARTESIAN_POINT('Ctrl Pts',(16.7403906073823,16.0027254972849,6.62060912535184));
#61739=CARTESIAN_POINT('Ctrl Pts',(17.9023688442237,16.1404688428348,7.18703525486854));
#61740=CARTESIAN_POINT('Ctrl Pts',(16.9475600453929,14.8638381887821,7.2343187616815));
#61741=CARTESIAN_POINT('Ctrl Pts',(16.676004214839,16.0214069152903,6.76401708988705));
#61742=CARTESIAN_POINT('Ctrl Pts',(17.8087626986413,16.1791346915417,7.33493716527047));
#61743=CARTESIAN_POINT('Ctrl Pts',(16.7593871717187,14.9710453070472,7.56294675844479));
#61744=CARTESIAN_POINT('Ctrl Pts',(16.5372832254195,16.072302724032,7.05030038222382));
#61745=CARTESIAN_POINT('Ctrl Pts',(17.6128899340039,16.2684739576301,7.62341025865086));
#61746=CARTESIAN_POINT('Ctrl Pts',(16.66107044624,15.0318575828356,7.72299307498027));
#61747=CARTESIAN_POINT('Ctrl Pts',(16.4632621472069,16.1041974200547,7.19296322794295));
#61748=CARTESIAN_POINT('Ctrl Pts',(17.5106213830702,16.3191508534299,7.76397957999253));
#61749=CARTESIAN_POINT('Ctrl Pts',(16.5331785751374,15.1163977359375,7.91798996938649));
#61750=CARTESIAN_POINT('Ctrl Pts',(16.363683758477,16.1530692164372,7.37184321612237));
#61751=CARTESIAN_POINT('Ctrl Pts',(17.3776610168937,16.3896009813358,7.93535376144086));
#61752=CARTESIAN_POINT('Ctrl Pts',(16.5073425396225,15.1337381226983,7.95674682628607));
#61753=CARTESIAN_POINT('Ctrl Pts',(16.3436274615726,16.1631828364744,7.40728149352596));
#61754=CARTESIAN_POINT('Ctrl Pts',(17.350804549412,16.404051303446,7.9694209838363));
#61755=CARTESIAN_POINT('Ctrl Pts',(16.4552077605916,15.1692434747578,8.03371146916027));
#61756=CARTESIAN_POINT('Ctrl Pts',(16.3029316796438,16.1842453845366,7.47800110793882));
#61757=CARTESIAN_POINT('Ctrl Pts',(17.2966172371086,16.4336390970814,8.0370840771131));
#61758=CARTESIAN_POINT('Ctrl Pts',(16.4289470322599,15.1873823884683,8.07186353228385));
#61759=CARTESIAN_POINT('Ctrl Pts',(16.2823261097163,16.1951736804993,7.51323025737201));
#61760=CARTESIAN_POINT('Ctrl Pts',(17.2693259015807,16.4487548582664,8.07063095624813));
#61761=CARTESIAN_POINT('Ctrl Pts',(16.3495983042681,15.2429346767302,8.18534944533382));
#61762=CARTESIAN_POINT('Ctrl Pts',(16.2199066334893,16.2290620068468,7.61822283696024));
#61763=CARTESIAN_POINT('Ctrl Pts',(17.1868723597951,16.4950484321605,8.17043566131922));
#61764=CARTESIAN_POINT('Ctrl Pts',(16.2959440226898,15.2814828159527,8.25971358276904));
#61765=CARTESIAN_POINT('Ctrl Pts',(16.1771667951557,16.2532836890568,7.68787236799991));
#61766=CARTESIAN_POINT('Ctrl Pts',(17.1311308780761,16.5271718810999,8.23585804734006));
#61767=CARTESIAN_POINT('Ctrl Pts',(16.187190221159,15.3615021794163,8.4059503498022));
#61768=CARTESIAN_POINT('Ctrl Pts',(16.0896613076013,16.3048931839763,7.82601148582257));
#61769=CARTESIAN_POINT('Ctrl Pts',(17.0181681919347,16.5938546843548,8.36455831953807));
#61770=CARTESIAN_POINT('Ctrl Pts',(16.132090655261,15.402973497386,8.47782290206415));
#61771=CARTESIAN_POINT('Ctrl Pts',(16.0449229247606,16.3322434767155,7.89450537829078));
#61772=CARTESIAN_POINT('Ctrl Pts',(16.9609469407587,16.6284141156668,8.42783613794276));
#61773=CARTESIAN_POINT('Ctrl Pts',(16.0623486088442,15.4565900493871,8.56615478270282));
#61774=CARTESIAN_POINT('Ctrl Pts',(15.9875357110085,16.3685339437292,7.97969610658542));
#61775=CARTESIAN_POINT('Ctrl Pts',(16.8885313500831,16.6730945758492,8.5056359305583));
#61776=CARTESIAN_POINT('Ctrl Pts',(16.0483568027876,15.467402285272,8.58374567928398));
#61777=CARTESIAN_POINT('Ctrl Pts',(15.9760448258777,16.3758585928759,7.99662595730545));
#61778=CARTESIAN_POINT('Ctrl Pts',(16.8740037632898,16.6821047723497,8.52113098104961));
#61779=CARTESIAN_POINT('Ctrl Pts',(16.0202872238867,15.489203582786,8.61877757332335));
#61780=CARTESIAN_POINT('Ctrl Pts',(15.9529421275418,16.3907011442425,8.0304074025005));
#61781=CARTESIAN_POINT('Ctrl Pts',(16.8448604825399,16.700272520346,8.55199220635214));
#61782=CARTESIAN_POINT('Ctrl Pts',(16.0062070274775,15.5001945865296,8.63622145671916));
#61783=CARTESIAN_POINT('Ctrl Pts',(15.9413286401597,16.3982198710585,8.04726199906429));
#61784=CARTESIAN_POINT('Ctrl Pts',(16.8302422728064,16.7094316900326,8.56736092530544));
#61785=CARTESIAN_POINT('Ctrl Pts',(15.9639006261601,15.5333825933383,8.68825415449347));
#61786=CARTESIAN_POINT('Ctrl Pts',(15.9064068601577,16.4210005179534,8.09756496571628));
#61787=CARTESIAN_POINT('Ctrl Pts',(16.7863209876344,16.7370883625705,8.61320847706342));
#61788=CARTESIAN_POINT('Ctrl Pts',(15.9355891535234,15.5558095777463,8.72256856997844));
#61789=CARTESIAN_POINT('Ctrl Pts',(15.8829080015083,16.4365560576359,8.13091450103497));
#61790=CARTESIAN_POINT('Ctrl Pts',(16.7569310542553,16.7557775159922,8.64345033245158));
#61791=CARTESIAN_POINT('Ctrl Pts',(15.7935142727831,15.6694196676398,8.89231733959516));
#61792=CARTESIAN_POINT('Ctrl Pts',(15.7654460880884,16.5154266792196,8.29516673757843));
#61793=CARTESIAN_POINT('Ctrl Pts',(16.6094545692347,16.8504525915035,8.79308481198999));
#61794=CARTESIAN_POINT('Ctrl Pts',(15.6782012682718,15.7650152188631,9.02229598142049));
#61795=CARTESIAN_POINT('Ctrl Pts',(15.6678545169391,16.584423347777,8.42399806744112));
#61796=CARTESIAN_POINT('Ctrl Pts',(16.4897904267136,16.9301155500535,8.90776544283607));
#61797=CARTESIAN_POINT('Ctrl Pts',(15.4446903454091,15.9649971701379,9.27157003213102));
#61798=CARTESIAN_POINT('Ctrl Pts',(15.4674094595755,16.7329835035073,8.67390873536768));
#61799=CARTESIAN_POINT('Ctrl Pts',(16.2475203695942,17.0967671767613,9.12791189678674));
#61800=CARTESIAN_POINT('Ctrl Pts',(15.3264914165494,16.0693856149141,9.39086266707201));
#61801=CARTESIAN_POINT('Ctrl Pts',(15.3646387505612,16.8123502221316,8.79517433817847));
#61802=CARTESIAN_POINT('Ctrl Pts',(16.1249134348094,17.1837575468854,9.23337528956514));
#61803=CARTESIAN_POINT('Ctrl Pts',(15.0875705659347,16.2866280399274,9.6194053126835));
#61804=CARTESIAN_POINT('Ctrl Pts',(15.1544604762242,16.9811904583532,9.02980769972348));
#61805=CARTESIAN_POINT('Ctrl Pts',(15.8771249439364,17.3647929014631,9.43565009494142));
#61806=CARTESIAN_POINT('Ctrl Pts',(14.9668478732092,16.3994827876149,9.72865388709201));
#61807=CARTESIAN_POINT('Ctrl Pts',(15.0471084939148,17.0704945862062,9.14336691901707));
#61808=CARTESIAN_POINT('Ctrl Pts',(15.7519425954886,17.4588385242348,9.53246024421486));
#61809=CARTESIAN_POINT('Ctrl Pts',(14.7232109117986,16.6335833330052,9.93750238929769));
#61810=CARTESIAN_POINT('Ctrl Pts',(14.8283473457646,17.258954975949,9.36240017693102));
#61811=CARTESIAN_POINT('Ctrl Pts',(15.4993427309287,17.6539223122627,9.71777676602946));
#61812=CARTESIAN_POINT('Ctrl Pts',(14.6002959559604,16.7548288643997,10.0371018524143));
#61813=CARTESIAN_POINT('Ctrl Pts',(14.7169704858705,17.357964069225,9.46806699747123));
#61814=CARTESIAN_POINT('Ctrl Pts',(15.3719244916505,17.7549602549693,9.80628272069675));
#61815=CARTESIAN_POINT('Ctrl Pts',(14.4145215062612,16.9431175621098,10.1793956077188));
#61816=CARTESIAN_POINT('Ctrl Pts',(14.5465177883743,17.5145354439133,9.62099020379824));
#61817=CARTESIAN_POINT('Ctrl Pts',(15.1793711691479,17.9118675030923,9.93293217024121));
#61818=CARTESIAN_POINT('Ctrl Pts',(14.3523630102681,17.006952463114,10.2256409441351));
#61819=CARTESIAN_POINT('Ctrl Pts',(14.4895201839198,17.5676954028143,9.6707281909746));
#61820=CARTESIAN_POINT('Ctrl Pts',(15.114949088864,17.9650632539259,9.97412895232606));
#61821=CARTESIAN_POINT('Ctrl Pts',(14.2588056678938,17.1043472732383,10.2932311994171));
#61822=CARTESIAN_POINT('Ctrl Pts',(14.4032304693875,17.6494581641149,9.74391620886052));
#61823=CARTESIAN_POINT('Ctrl Pts',(15.0179918642274,18.0462255956853,10.0343961461429));
#61824=CARTESIAN_POINT('Ctrl Pts',(14.2275428962468,17.1371113569171,10.3154811859238));
#61825=CARTESIAN_POINT('Ctrl Pts',(14.3744069573424,17.6769793096807,9.76801833846068));
#61826=CARTESIAN_POINT('Ctrl Pts',(14.9855941905893,18.0735289987137,10.0542450128963));
#61827=CARTESIAN_POINT('Ctrl Pts',(14.1651063844055,17.2029930321826,10.3592551672391));
#61828=CARTESIAN_POINT('Ctrl Pts',(14.3167427850065,17.7324684434336,9.81554948650699));
#61829=CARTESIAN_POINT('Ctrl Pts',(14.9208935457682,18.12843039485,10.0933144453783));
#61830=CARTESIAN_POINT('Ctrl Pts',(14.1339177282514,17.2361258045806,10.380790467117));
#61831=CARTESIAN_POINT('Ctrl Pts',(14.2878875452418,17.7604480955151,9.8389943174788));
#61832=CARTESIAN_POINT('Ctrl Pts',(14.8885751144014,18.1560410384386,10.1125450762014));
#61833=CARTESIAN_POINT('Ctrl Pts',(13.9781364881385,17.4027525271718,10.4867280999607));
#61834=CARTESIAN_POINT('Ctrl Pts',(14.144431831079,17.9006324325898,9.95387647546919));
#61835=CARTESIAN_POINT('Ctrl Pts',(14.7271571232573,18.2948966407755,10.2071949179051));
#61836=CARTESIAN_POINT('Ctrl Pts',(13.8540272655431,17.5391270979538,10.5659251844625));
#61837=CARTESIAN_POINT('Ctrl Pts',(14.028608363573,18.0172146350274,10.0413506176408));
#61838=CARTESIAN_POINT('Ctrl Pts',(14.5985769926317,18.4085421162159,10.2781140808652));
#61839=CARTESIAN_POINT('Ctrl Pts',(13.6072409325253,17.8182304543897,10.713529670147));
#61840=CARTESIAN_POINT('Ctrl Pts',(13.7971283710368,18.2578118922052,10.2058308444696));
#61841=CARTESIAN_POINT('Ctrl Pts',(14.3429475819855,18.6411282467177,10.4106278582409));
#61842=CARTESIAN_POINT('Ctrl Pts',(13.4845627999781,17.9609582798185,10.781937133576));
#61843=CARTESIAN_POINT('Ctrl Pts',(13.68137490276,18.3818077707664,10.2830660507971));
#61844=CARTESIAN_POINT('Ctrl Pts',(14.2158972008177,18.7600681011593,10.4722225230956));
#61845=CARTESIAN_POINT('Ctrl Pts',(13.2411241058063,18.253191261943,10.9079911532372));
#61846=CARTESIAN_POINT('Ctrl Pts',(13.4507300765943,18.6373898413164,10.4269274198646));
#61847=CARTESIAN_POINT('Ctrl Pts',(13.9638433346872,19.0035955862893,10.5861136733016));
#61848=CARTESIAN_POINT('Ctrl Pts',(13.1203620303411,18.4026943555333,10.9656391301105));
#61849=CARTESIAN_POINT('Ctrl Pts',(13.3357311395337,18.7689688605621,10.4937660511775));
#61850=CARTESIAN_POINT('Ctrl Pts',(13.8388382058427,19.1281814976295,10.6384113937824));
#61851=CARTESIAN_POINT('Ctrl Pts',(12.8813643765524,18.709160598925,11.0698962741953));
#61852=CARTESIAN_POINT('Ctrl Pts',(13.1073841447931,19.0401383352438,10.6164410863953));
#61853=CARTESIAN_POINT('Ctrl Pts',(13.5915263050113,19.3835700337331,10.7334679599571));
#61854=CARTESIAN_POINT('Ctrl Pts',(12.7631264212453,18.8661199837945,11.1165087586551));
#61855=CARTESIAN_POINT('Ctrl Pts',(12.9939167896628,19.1797318608651,10.6724778564328));
#61856=CARTESIAN_POINT('Ctrl Pts',(13.4692169404985,19.514369521206,10.7762296953549));
#61857=CARTESIAN_POINT('Ctrl Pts',(12.588256130994,19.107924240872,11.1776586988793));
#61858=CARTESIAN_POINT('Ctrl Pts',(12.8251498460236,19.396355589634,10.7479663558257));
#61859=CARTESIAN_POINT('Ctrl Pts',(13.288413035126,19.7158730686902,10.8327926739995));
#61860=CARTESIAN_POINT('Ctrl Pts',(12.5303820948896,19.1895895478315,11.1965773236667));
#61861=CARTESIAN_POINT('Ctrl Pts',(12.7693698581218,19.4694425906221,10.7716181429504));
#61862=CARTESIAN_POINT('Ctrl Pts',(13.228590194886,19.7839274912126,10.8503809199751));
#61863=CARTESIAN_POINT('Ctrl Pts',(12.4442875600793,19.3138133318091,11.2226618407279));
#61864=CARTESIAN_POINT('Ctrl Pts',(12.6861620401978,19.5809868737173,10.8048576816646));
#61865=CARTESIAN_POINT('Ctrl Pts',(13.1396233538652,19.8874473111499,10.8747803405286));
#61866=CARTESIAN_POINT('Ctrl Pts',(12.4156897929966,19.3555382597294,11.2309788997662));
#61867=CARTESIAN_POINT('Ctrl Pts',(12.6585422539374,19.6184329070213,10.8155506477599));
#61868=CARTESIAN_POINT('Ctrl Pts',(13.110076023704,19.9222180844219,10.8825872590395));
#61869=CARTESIAN_POINT('Ctrl Pts',(12.3589724361245,19.4392584338625,11.2467690565977));
#61870=CARTESIAN_POINT('Ctrl Pts',(12.6037297739884,19.6936318051644,10.8360783405224));
#61871=CARTESIAN_POINT('Ctrl Pts',(13.0514852202568,19.9919848962186,10.8974664623896));
#61872=CARTESIAN_POINT('Ctrl Pts',(12.3308287601266,19.4812877976075,11.254249927555));
#61873=CARTESIAN_POINT('Ctrl Pts',(12.5765109676552,19.7314166631751,10.8459258664003));
#61874=CARTESIAN_POINT('Ctrl Pts',(13.022416850563,20.0270093659881,10.9045459804305));
#61875=CARTESIAN_POINT('Ctrl Pts',(12.1912269576885,19.6923091894597,11.289563129842));
#61876=CARTESIAN_POINT('Ctrl Pts',(12.4419749171144,19.9204932765277,10.892849759858));
#61877=CARTESIAN_POINT('Ctrl Pts',(12.8782548607845,20.2028605259071,10.9381252948214));
#61878=CARTESIAN_POINT('Ctrl Pts',(12.0831043807717,19.8639143262306,11.3111434004142));
#61879=CARTESIAN_POINT('Ctrl Pts',(12.3369629663802,20.0754427469213,10.9238985178924));
#61880=CARTESIAN_POINT('Ctrl Pts',(12.7666864057961,20.3458635515731,10.9591889337323));
#61881=CARTESIAN_POINT('Ctrl Pts',(11.9791786279775,20.0387490638529,11.3256333545128));
#61882=CARTESIAN_POINT('Ctrl Pts',(12.235442756324,20.2343859095505,10.9477939369723));
#61883=CARTESIAN_POINT('Ctrl Pts',(12.659562935147,20.491560421201,10.974081743871));
#61884=CARTESIAN_POINT('Ctrl Pts',(16.5375680855082,20.0478523191736,0.351922770622401));
#61885=CARTESIAN_POINT('Ctrl Pts',(16.5498686081438,19.9784919885108,0.320595854365059));
#61886=CARTESIAN_POINT('Ctrl Pts',(16.5645008101836,19.909569989448,0.289650387375635));
#61887=CARTESIAN_POINT('Ctrl Pts',(16.5814951892386,19.8410460986085,0.259194053810624));
#61888=CARTESIAN_POINT('Ctrl Pts',(16.5876276939095,19.8163189179756,0.248203737115972));
#61889=CARTESIAN_POINT('Ctrl Pts',(16.5940682683641,19.7916436939745,0.237277153603447));
#61890=CARTESIAN_POINT('Ctrl Pts',(16.6008199371749,19.7670190220225,0.226419498601689));
#61891=CARTESIAN_POINT('Ctrl Pts',(16.6135508792567,19.7205867574685,0.205946311772581));
#61892=CARTESIAN_POINT('Ctrl Pts',(16.6273872562386,19.6743339367231,0.185717894040129));
#61893=CARTESIAN_POINT('Ctrl Pts',(16.6423581815811,19.6282521577127,0.165770386909323));
#61894=CARTESIAN_POINT('Ctrl Pts',(16.6498436442524,19.6052112682075,0.15579663334392));
#61895=CARTESIAN_POINT('Ctrl Pts',(16.6576148736858,19.5822076576934,0.145890788161576));
#61896=CARTESIAN_POINT('Ctrl Pts',(16.6656701975499,19.5592586752321,0.136065467307112));
#61897=CARTESIAN_POINT('Ctrl Pts',(16.6696978594819,19.5477841840015,0.131152806879879));
#61898=CARTESIAN_POINT('Ctrl Pts',(16.6737956214272,19.5363259044026,0.126261367078692));
#61899=CARTESIAN_POINT('Ctrl Pts',(16.6779639213557,19.5248837445505,0.121391733564308));
#61900=CARTESIAN_POINT('Ctrl Pts',(16.68004807132,19.5191626646244,0.118956916807116));
#61901=CARTESIAN_POINT('Ctrl Pts',(16.6821498564429,19.5134456148765,0.116527551626322));
#61902=CARTESIAN_POINT('Ctrl Pts',(16.6842693357308,19.5077325845678,0.114103713065847));
#61903=CARTESIAN_POINT('Ctrl Pts',(16.6853290753747,19.5048760694135,0.112891793785614));
#61904=CARTESIAN_POINT('Ctrl Pts',(16.6863950302563,19.5020157956128,0.111678464240845));
#61905=CARTESIAN_POINT('Ctrl Pts',(16.6874607163255,19.4991690245389,0.110473990584703));
#61906=CARTESIAN_POINT('Ctrl Pts',(16.6885264023947,19.496322253465,0.109269516928562));
#61907=CARTESIAN_POINT('Ctrl Pts',(16.68959629266,19.4934770520699,0.108065067624267));
#61908=CARTESIAN_POINT('Ctrl Pts',(16.6906703875662,19.4906334205523,0.106860642655115));
#61909=CARTESIAN_POINT('Origin',(0.,0.,0.));
#61910=CARTESIAN_POINT('Origin',(6.61325378140121E-15,20.5440037453176,
8.67361737988404E-16));
#61911=CARTESIAN_POINT('Ctrl Pts',(-13.7129564349448,20.6615335048059,9.85952349485951));
#61912=CARTESIAN_POINT('Ctrl Pts',(-13.2371163881454,20.6161954472713,9.8616439740488));
#61913=CARTESIAN_POINT('Ctrl Pts',(-12.9440892692056,20.5440037453176,10.2323288156136));
#61914=CARTESIAN_POINT('Ctrl Pts',(-13.7008624134648,20.7562745931684,9.87092777877101));
#61915=CARTESIAN_POINT('Ctrl Pts',(-13.2264454758027,20.7233778620598,9.87599115017895));
#61916=CARTESIAN_POINT('Ctrl Pts',(-12.9326863129145,20.6716508716995,10.2467537707557));
#61917=CARTESIAN_POINT('Ctrl Pts',(-13.6938907193449,20.8508740411617,9.87747041407926));
#61918=CARTESIAN_POINT('Ctrl Pts',(-13.2202702521004,20.8307764858601,9.88425338309928));
#61919=CARTESIAN_POINT('Ctrl Pts',(-12.9261130230882,20.7990969574018,10.2550285610119));
#61920=CARTESIAN_POINT('Ctrl Pts',(-13.6900072944242,21.0397796008549,9.88111811705835));
#61921=CARTESIAN_POINT('Ctrl Pts',(-13.2168370418637,21.0451161585058,9.88885105592462));
#61922=CARTESIAN_POINT('Ctrl Pts',(-12.9224515081237,21.0535913718615,10.2596420840599));
#61923=CARTESIAN_POINT('Ctrl Pts',(-13.6930958642434,21.1340866197803,9.87822261515375));
#61924=CARTESIAN_POINT('Ctrl Pts',(-13.2195733682617,21.1522378018448,9.88519381277553));
#61925=CARTESIAN_POINT('Ctrl Pts',(-12.9253635881698,21.1806406639321,10.2559800621746));
#61926=CARTESIAN_POINT('Ctrl Pts',(-13.7052327444816,21.2753200907549,9.86680289931835));
#61927=CARTESIAN_POINT('Ctrl Pts',(-13.2302950439844,21.3122978585196,9.87081048784163));
#61928=CARTESIAN_POINT('Ctrl Pts',(-12.9368069325275,21.3709184052818,10.2415362188021));
#61929=CARTESIAN_POINT('Ctrl Pts',(-13.7105300124574,21.3223600206349,9.86181478306048));
#61930=CARTESIAN_POINT('Ctrl Pts',(-13.2349772513254,21.3656075188109,9.86452423850202));
#61931=CARTESIAN_POINT('Ctrl Pts',(-12.9418014993605,21.4342948826322,10.2352270743557));
#61932=CARTESIAN_POINT('Ctrl Pts',(-13.720357190954,21.3928615448091,9.85254095225805));
#61933=CARTESIAN_POINT('Ctrl Pts',(-13.2436527129957,21.4453947467137,9.85285084207422));
#61934=CARTESIAN_POINT('Ctrl Pts',(-12.9510671249071,21.5292848798817,10.2234967185532));
#61935=CARTESIAN_POINT('Ctrl Pts',(-13.7239465270711,21.4163523209677,9.8491509266678));
#61936=CARTESIAN_POINT('Ctrl Pts',(-13.2468219311174,21.4719759498813,9.84858285770261));
#61937=CARTESIAN_POINT('Ctrl Pts',(-12.9544513560252,21.5609357545812,10.2192086490361));
#61938=CARTESIAN_POINT('Ctrl Pts',(-13.7298020217399,21.4515736639483,9.84361405487951));
#61939=CARTESIAN_POINT('Ctrl Pts',(-13.25198915428,21.511800561518,9.84161579593135));
#61940=CARTESIAN_POINT('Ctrl Pts',(-12.9599722510621,21.6083932667593,10.212204859321));
#61941=CARTESIAN_POINT('Ctrl Pts',(-13.7318308096277,21.4633010512971,9.84169465498939));
#61942=CARTESIAN_POINT('Ctrl Pts',(-13.2537795725195,21.5250593212155,9.83920044919479));
#61943=CARTESIAN_POINT('Ctrl Pts',(-12.9618851081689,21.6241950353554,10.2097769165122));
#61944=CARTESIAN_POINT('Ctrl Pts',(-13.7360304150215,21.4866713806995,9.83771906460812));
#61945=CARTESIAN_POINT('Ctrl Pts',(-13.2574850933722,21.5514732332995,9.83419845061536));
#61946=CARTESIAN_POINT('Ctrl Pts',(-12.9658447361586,21.6556852063039,10.2047479400592));
#61947=CARTESIAN_POINT('Ctrl Pts',(-13.7382026582792,21.4983229897648,9.83566152684288));
#61948=CARTESIAN_POINT('Ctrl Pts',(-13.2594015448338,21.5646384856195,9.83160997938521));
#61949=CARTESIAN_POINT('Ctrl Pts',(-12.9678928511819,21.6713852864878,10.2021452014677));
#61950=CARTESIAN_POINT('Ctrl Pts',(-13.7583954816181,21.6028889555656,9.81652257225709));
#61951=CARTESIAN_POINT('Ctrl Pts',(-13.2772366388668,21.6829047947831,9.80750493402147));
#61952=CARTESIAN_POINT('Ctrl Pts',(-12.9869317991238,21.8122857656886,10.177934563794));
#61953=CARTESIAN_POINT('Ctrl Pts',(-13.7809040295564,21.693719602389,9.79510721646933));
#61954=CARTESIAN_POINT('Ctrl Pts',(-13.2971007311209,21.7852988934574,9.78055185957662));
#61955=CARTESIAN_POINT('Ctrl Pts',(-13.0081541438556,21.9346925203426,10.1508423296431));
#61956=CARTESIAN_POINT('Ctrl Pts',(-13.8341301723179,21.8714587721286,9.7440196442469));
#61957=CARTESIAN_POINT('Ctrl Pts',(-13.3439003310147,21.9847542762144,9.71648353832225));
#61958=CARTESIAN_POINT('Ctrl Pts',(-13.0583387932841,22.1742604353913,10.0862015740016));
#61959=CARTESIAN_POINT('Ctrl Pts',(-13.8648496341611,21.9583663972777,9.7143454568808));
#61960=CARTESIAN_POINT('Ctrl Pts',(-13.3709025718912,22.0819353397743,9.67927384763397));
#61961=CARTESIAN_POINT('Ctrl Pts',(-13.0873028567095,22.2914203627217,10.0486505478074));
#61962=CARTESIAN_POINT('Ctrl Pts',(-13.9165696229565,22.0859247227897,9.66382831234646));
#61963=CARTESIAN_POINT('Ctrl Pts',(-13.4161030564968,22.2235043007119,9.6162866335379));
#61964=CARTESIAN_POINT('Ctrl Pts',(-13.1360674180666,22.4634190171285,9.98471087522344));
#61965=CARTESIAN_POINT('Ctrl Pts',(-13.9347512757793,22.1279760891408,9.64598616900946));
#61966=CARTESIAN_POINT('Ctrl Pts',(-13.4320016960487,22.2701169401881,9.59402578243727));
#61967=CARTESIAN_POINT('Ctrl Pts',(-13.1532101189578,22.520127147885,9.96212609982419));
#61968=CARTESIAN_POINT('Ctrl Pts',(-13.9586119850529,22.1799633981706,9.62243408712692));
#61969=CARTESIAN_POINT('Ctrl Pts',(-13.4528007586469,22.327479415284,9.56473185020972));
#61970=CARTESIAN_POINT('Ctrl Pts',(-13.1757073593519,22.5902429783183,9.93231047564518));
#61971=CARTESIAN_POINT('Ctrl Pts',(-13.9634401862198,22.1903303348201,9.61766179084814));
#61972=CARTESIAN_POINT('Ctrl Pts',(-13.4570131842341,22.3389231592103,9.5587907059358));
#61973=CARTESIAN_POINT('Ctrl Pts',(-13.1802596632253,22.6042254120874,9.92626886445875));
#61974=CARTESIAN_POINT('Ctrl Pts',(-13.9731827903011,22.2109522681602,9.60801815535573));
#61975=CARTESIAN_POINT('Ctrl Pts',(-13.4655097721022,22.361667873411,9.5467898447481));
#61976=CARTESIAN_POINT('Ctrl Pts',(-13.1894455471525,22.6320401834821,9.91405994122819));
#61977=CARTESIAN_POINT('Ctrl Pts',(-13.9781003259087,22.2212141419427,9.60314372718884));
#61978=CARTESIAN_POINT('Ctrl Pts',(-13.4697968130973,22.3729765457423,9.5407260615401));
#61979=CARTESIAN_POINT('Ctrl Pts',(-13.194082080646,22.645881795839,9.90788871798151));
#61980=CARTESIAN_POINT('Ctrl Pts',(-13.9929886664845,22.2518545078711,9.58836426018849));
#61981=CARTESIAN_POINT('Ctrl Pts',(-13.4827764946496,22.4067278212097,9.52233984264939));
#61982=CARTESIAN_POINT('Ctrl Pts',(-13.2081196590227,22.6872120460856,9.8891768245822));
#61983=CARTESIAN_POINT('Ctrl Pts',(-14.0030951729371,22.2720877777252,9.57830307479199));
#61984=CARTESIAN_POINT('Ctrl Pts',(-13.4915772298429,22.4289668826426,9.50983726183198));
#61985=CARTESIAN_POINT('Ctrl Pts',(-13.2176486506602,22.7145061408827,9.87643797357817));
#61986=CARTESIAN_POINT('Ctrl Pts',(-14.0544950872555,22.3723107632432,9.52697587647896));
#61987=CARTESIAN_POINT('Ctrl Pts',(-13.5364171985493,22.5392216393244,9.4459384887215));
#61988=CARTESIAN_POINT('Ctrl Pts',(-13.2661114274225,22.8497131272088,9.81144708832414));
#61989=CARTESIAN_POINT('Ctrl Pts',(-14.0983814638585,22.4494795558663,9.48265575102692));
#61990=CARTESIAN_POINT('Ctrl Pts',(-13.5745151620739,22.623246501772,9.39101851350584));
#61991=CARTESIAN_POINT('Ctrl Pts',(-13.307490010411,22.9538479586332,9.7553174356521));
#61992=CARTESIAN_POINT('Ctrl Pts',(-14.1908900778254,22.5982767086274,9.38783947033386));
#61993=CARTESIAN_POINT('Ctrl Pts',(-13.6544084086815,22.7837809574408,9.2741414794923));
#61994=CARTESIAN_POINT('Ctrl Pts',(-13.3947124185492,23.1547019112495,9.63520564761807));
#61995=CARTESIAN_POINT('Ctrl Pts',(-14.2395143208195,22.6699034777907,9.33734184539398));
#61996=CARTESIAN_POINT('Ctrl Pts',(-13.6962759549276,22.8603048839474,9.2120652177674));
#61997=CARTESIAN_POINT('Ctrl Pts',(-13.4405581326707,23.2514188762212,9.57122165649343));
#61998=CARTESIAN_POINT('Ctrl Pts',(-14.3028824235611,22.7561439383135,9.27043394448135));
#61999=CARTESIAN_POINT('Ctrl Pts',(-13.7503320008934,22.9510684986001,9.1305999395379));
#62000=CARTESIAN_POINT('Ctrl Pts',(-13.5003052014195,23.3679086709528,9.48642134320106));
#62001=CARTESIAN_POINT('Ctrl Pts',(-14.3156858423305,22.7732269395806,9.25686258744708));
#62002=CARTESIAN_POINT('Ctrl Pts',(-13.7612800093358,22.9690563554823,9.1140363510689));
#62003=CARTESIAN_POINT('Ctrl Pts',(-13.5123769960781,23.3909857126619,9.46921965085858));
#62004=CARTESIAN_POINT('Ctrl Pts',(-14.3415444610434,22.8070653424621,9.22934032392019));
#62005=CARTESIAN_POINT('Ctrl Pts',(-13.7833625282499,23.0045755462846,9.08049093073045));
#62006=CARTESIAN_POINT('Ctrl Pts',(-13.5367579796183,23.4367014225698,9.434332847721));
#62007=CARTESIAN_POINT('Ctrl Pts',(-14.3546119847482,22.8238361574984,9.21537617557595));
#62008=CARTESIAN_POINT('Ctrl Pts',(-13.7945085636611,23.0221227644561,9.06349111287955));
#62009=CARTESIAN_POINT('Ctrl Pts',(-13.5490787875207,23.4593609186655,9.41663094852836));
#62010=CARTESIAN_POINT('Ctrl Pts',(-14.3940884280465,22.8735437111473,9.17301313642827));
#62011=CARTESIAN_POINT('Ctrl Pts',(-13.8281767258758,23.0740233932832,9.01192667725968));
#62012=CARTESIAN_POINT('Ctrl Pts',(-13.5862994342721,23.5265284425343,9.36292504120361));
#62013=CARTESIAN_POINT('Ctrl Pts',(-14.4207294531298,22.9058268139983,9.14418892615148));
#62014=CARTESIAN_POINT('Ctrl Pts',(-13.8508147344641,23.1074533359785,8.97697022835382));
#62015=CARTESIAN_POINT('Ctrl Pts',(-13.6114181147807,23.5701596174622,9.32637822598396));
#62016=CARTESIAN_POINT('Ctrl Pts',(-14.5015145230641,23.0002161807818,9.0560103250754));
#62017=CARTESIAN_POINT('Ctrl Pts',(-13.9194392503705,23.2047432403349,8.87008512211998));
#62018=CARTESIAN_POINT('Ctrl Pts',(-13.687586895431,23.6977533801126,9.21455916568862));
#62019=CARTESIAN_POINT('Ctrl Pts',(-14.5565167428664,23.0598693881876,8.9949541376985));
#62020=CARTESIAN_POINT('Ctrl Pts',(-13.9658098008849,23.2650693985997,8.7966275351461));
#62021=CARTESIAN_POINT('Ctrl Pts',(-13.7394461306717,23.7784254927315,9.13711358232858));
#62022=CARTESIAN_POINT('Ctrl Pts',(-14.668344609763,23.1730054700806,8.86840507942585));
#62023=CARTESIAN_POINT('Ctrl Pts',(-14.0594549219421,23.3775022338952,8.6455112590186));
#62024=CARTESIAN_POINT('Ctrl Pts',(-13.8448838343227,23.9314901957697,8.97654812319932));
#62025=CARTESIAN_POINT('Ctrl Pts',(-14.7251713842222,23.2264870910406,8.80291165328951));
#62026=CARTESIAN_POINT('Ctrl Pts',(-14.1067652302453,23.4295449273,8.56776497327688));
#62027=CARTESIAN_POINT('Ctrl Pts',(-13.8984633639411,24.0038810977667,8.89342755183832));
#62028=CARTESIAN_POINT('Ctrl Pts',(-14.8115128374888,23.3022059813901,8.70132522573414));
#62029=CARTESIAN_POINT('Ctrl Pts',(-14.177907529371,23.501375403437,8.44854965801709));
#62030=CARTESIAN_POINT('Ctrl Pts',(-13.9798710203244,24.106421055664,8.76446179920621));
#62031=CARTESIAN_POINT('Ctrl Pts',(-14.8404776247069,23.3266935233931,8.66690442430847));
#62032=CARTESIAN_POINT('Ctrl Pts',(-14.201761297046,23.5243702015138,8.40818786835522));
#62033=CARTESIAN_POINT('Ctrl Pts',(-14.0071806765434,24.1395912869237,8.72075786856021));
#62034=CARTESIAN_POINT('Ctrl Pts',(-14.8841738662445,23.3622994228145,8.61442455050914));
#62035=CARTESIAN_POINT('Ctrl Pts',(-14.2375569630117,23.5573031545392,8.34701137746259));
#62036=CARTESIAN_POINT('Ctrl Pts',(-14.0483799902215,24.1878351113527,8.65411472810432));
#62037=CARTESIAN_POINT('Ctrl Pts',(-14.898780829388,23.3739803985349,8.59678975566993));
#62038=CARTESIAN_POINT('Ctrl Pts',(-14.2495188731664,23.5680437684686,8.32646567239338));
#62039=CARTESIAN_POINT('Ctrl Pts',(-14.0621522696036,24.2036643463797,8.63171906640857));
#62040=CARTESIAN_POINT('Ctrl Pts',(-14.9280737343777,23.3969664267311,8.56123466719224));
#62041=CARTESIAN_POINT('Ctrl Pts',(-14.2734612706719,23.5890201048075,8.28513372834998));
#62042=CARTESIAN_POINT('Ctrl Pts',(-14.0897712944622,24.2348178206969,8.58656190594739));
#62043=CARTESIAN_POINT('Ctrl Pts',(-14.9427728434619,23.4082813558474,8.54329819094064));
#62044=CARTESIAN_POINT('Ctrl Pts',(-14.2854527847599,23.5992633548238,8.2643275981937));
#62045=CARTESIAN_POINT('Ctrl Pts',(-14.1036304543349,24.2501554507848,8.5637798506607));
#62046=CARTESIAN_POINT('Ctrl Pts',(-15.0162918057908,23.463789382512,8.45309665896628));
#62047=CARTESIAN_POINT('Ctrl Pts',(-14.345589788043,23.6493359864249,8.15945005612194));
#62048=CARTESIAN_POINT('Ctrl Pts',(-14.1729483333222,24.3254089672111,8.4492018977763));
#62049=CARTESIAN_POINT('Ctrl Pts',(-15.0749937583277,23.5046581308708,8.37950805432951));
#62050=CARTESIAN_POINT('Ctrl Pts',(-14.3930063388903,23.6846359402687,8.07502243760036));
#62051=CARTESIAN_POINT('Ctrl Pts',(-14.2282958882168,24.3808520221291,8.35570011884672));
#62052=CARTESIAN_POINT('Ctrl Pts',(-15.1919438181211,23.5795869273186,8.22948916349949));
#62053=CARTESIAN_POINT('Ctrl Pts',(-14.486695680729,23.7467356064268,7.90470339609567));
#62054=CARTESIAN_POINT('Ctrl Pts',(-14.3385630878073,24.482570276287,8.1650313493404));
#62055=CARTESIAN_POINT('Ctrl Pts',(-15.2501924267091,23.613646051469,8.15305871293753));
#62056=CARTESIAN_POINT('Ctrl Pts',(-14.5329550676768,23.7734255231783,7.81879172377405));
#62057=CARTESIAN_POINT('Ctrl Pts',(-14.3934832041134,24.5288442366298,8.06786415465658));
#62058=CARTESIAN_POINT('Ctrl Pts',(-15.3660549813521,23.6750199888892,7.99730768353786));
#62059=CARTESIAN_POINT('Ctrl Pts',(-14.6241723132235,23.8185526248242,7.64575731456955));
#62060=CARTESIAN_POINT('Ctrl Pts',(-14.5027250417167,24.6123032785761,7.86980032335321));
#62061=CARTESIAN_POINT('Ctrl Pts',(-15.4236692333466,23.7023347223222,7.91798719626487));
#62062=CARTESIAN_POINT('Ctrl Pts',(-14.669110374985,23.8368802777693,7.55862491601526));
#62063=CARTESIAN_POINT('Ctrl Pts',(-14.5570470503623,24.6494882615742,7.76890380790145));
#62064=CARTESIAN_POINT('Ctrl Pts',(-15.5381155519261,23.7501002878386,7.7563480148621));
#62065=CARTESIAN_POINT('Ctrl Pts',(-14.7575757640514,23.8653814929517,7.38336094784725));
#62066=CARTESIAN_POINT('Ctrl Pts',(-14.6649535796959,24.7146000317624,7.56324148155097));
#62067=CARTESIAN_POINT('Ctrl Pts',(-15.5949477885535,23.7705518456696,7.67402967710675));
#62068=CARTESIAN_POINT('Ctrl Pts',(-14.8010775596278,23.8754457720047,7.29523076675808));
#62069=CARTESIAN_POINT('Ctrl Pts',(-14.7185382595438,24.7425278102842,7.45847612910266));
#62070=CARTESIAN_POINT('Ctrl Pts',(-15.6583759290202,23.7895227363621,7.57963700695744));
#62071=CARTESIAN_POINT('Ctrl Pts',(-14.848915766986,23.8821191585875,7.19618114873475));
#62072=CARTESIAN_POINT('Ctrl Pts',(-14.778341935074,24.7684964697845,7.33831261712725));
#62073=CARTESIAN_POINT('Ctrl Pts',(-15.6654185515291,23.7915749374926,7.56912092241342));
#62074=CARTESIAN_POINT('Ctrl Pts',(-14.8542511805829,23.8827998732592,7.18510330732812));
#62075=CARTESIAN_POINT('Ctrl Pts',(-14.7849821219855,24.7713067262627,7.32492503082377));
#62076=CARTESIAN_POINT('Ctrl Pts',(-15.6794568481,23.7955570617443,7.54808774958257));
#62077=CARTESIAN_POINT('Ctrl Pts',(-14.8648739978814,23.8840287355543,7.16298628917305));
#62078=CARTESIAN_POINT('Ctrl Pts',(-14.7982182301801,24.7767619627578,7.29814772847103));
#62079=CARTESIAN_POINT('Ctrl Pts',(-15.6864563544083,23.7974881670599,7.53756498179427));
#62080=CARTESIAN_POINT('Ctrl Pts',(-14.8701642040516,23.8845771129149,7.15194123209345));
#62081=CARTESIAN_POINT('Ctrl Pts',(-14.8048177647002,24.7794085602713,7.2847507825764));
#62082=CARTESIAN_POINT('Ctrl Pts',(-15.7073959645382,23.8031021002813,7.50597813481449));
#62083=CARTESIAN_POINT('Ctrl Pts',(-14.885984729689,23.8860275669589,7.11881961059018));
#62084=CARTESIAN_POINT('Ctrl Pts',(-14.8245608256785,24.787105926226,7.24453506904895));
#62085=CARTESIAN_POINT('Ctrl Pts',(-15.7212771599653,23.8066055693578,7.48489551226781));
#62086=CARTESIAN_POINT('Ctrl Pts',(-14.8964386686442,23.8867313559105,7.09681104447996));
#62087=CARTESIAN_POINT('Ctrl Pts',(-14.8376488099401,24.7919142997836,7.2176914258036));
#62088=CARTESIAN_POINT('Ctrl Pts',(-15.7626852346004,23.8164015449187,7.42157346868287));
#62089=CARTESIAN_POINT('Ctrl Pts',(-14.9276026898393,23.8880752497196,7.0308431001553));
#62090=CARTESIAN_POINT('Ctrl Pts',(-14.8766907088792,24.8053737133838,7.13706105153195));
#62091=CARTESIAN_POINT('Ctrl Pts',(-15.7899766087168,23.8219799870563,7.37925987478814));
#62092=CARTESIAN_POINT('Ctrl Pts',(-14.9480092475861,23.8879340460042,6.98716073149568));
#62093=CARTESIAN_POINT('Ctrl Pts',(-14.9024225759064,24.8130595406911,7.08317487963834));
#62094=CARTESIAN_POINT('Ctrl Pts',(-15.8709094466626,23.835869380065,7.2520222729819));
#62095=CARTESIAN_POINT('Ctrl Pts',(-15.0084598442621,23.8845192115295,6.8563707129466));
#62096=CARTESIAN_POINT('Ctrl Pts',(-14.9787306802509,24.8322686771154,6.92111892934993));
#62097=CARTESIAN_POINT('Ctrl Pts',(-15.9236097319743,23.841340127962,7.16680149302588));
#62098=CARTESIAN_POINT('Ctrl Pts',(-15.0473075053422,23.8782090354518,6.77041081593507));
#62099=CARTESIAN_POINT('Ctrl Pts',(-15.0284195206932,24.8399513694313,6.81255177500307));
#62100=CARTESIAN_POINT('Ctrl Pts',(-16.0265018511833,23.8446215600908,6.99556668801121));
#62101=CARTESIAN_POINT('Ctrl Pts',(-15.1226269240625,23.8580414080585,6.6003226406466));
#62102=CARTESIAN_POINT('Ctrl Pts',(-15.1254320902278,24.8449513768056,6.59435812349903));
#62103=CARTESIAN_POINT('Ctrl Pts',(-16.0766936861889,23.8424326922463,6.9095526644017));
#62104=CARTESIAN_POINT('Ctrl Pts',(-15.1590388789855,23.8441003828677,6.51628678808945));
#62105=CARTESIAN_POINT('Ctrl Pts',(-15.1727558203807,24.8422693073838,6.48473162798369));
#62106=CARTESIAN_POINT('Ctrl Pts',(-16.1745669329239,23.8301237547381,6.73672799807676));
#62107=CARTESIAN_POINT('Ctrl Pts',(-15.2296669338826,23.8088460726592,6.35006678355624));
#62108=CARTESIAN_POINT('Ctrl Pts',(-15.2650363101553,24.8261665177154,6.26441776396718));
#62109=CARTESIAN_POINT('Ctrl Pts',(-16.2222483460131,23.8200050092142,6.64991735889322));
#62110=CARTESIAN_POINT('Ctrl Pts',(-15.2638253783645,23.7874652737709,6.26798066443082));
#62111=CARTESIAN_POINT('Ctrl Pts',(-15.3099930710717,24.8127475992357,6.1537303994777));
#62112=CARTESIAN_POINT('Ctrl Pts',(-16.2802777157372,23.802096340301,6.54090305034875));
#62113=CARTESIAN_POINT('Ctrl Pts',(-15.3051135819173,23.7562469286197,6.16689903262489));
#62114=CARTESIAN_POINT('Ctrl Pts',(-15.3647064768095,24.7888483010614,6.01470595587148));
#62115=CARTESIAN_POINT('Ctrl Pts',(-16.29180496139,23.7982510047644,6.51907513414521));
#62116=CARTESIAN_POINT('Ctrl Pts',(-15.3133397276194,23.7497446711847,6.14666201036101));
#62117=CARTESIAN_POINT('Ctrl Pts',(-15.3755750227115,24.7837113625475,5.9868678002244));
#62118=CARTESIAN_POINT('Ctrl Pts',(-16.3089777985448,23.7920800113923,6.48629560658751));
#62119=CARTESIAN_POINT('Ctrl Pts',(-15.3255783192788,23.7396466784538,6.11641210641516));
#62120=CARTESIAN_POINT('Ctrl Pts',(-15.3917665548854,24.7754600011086,5.9450606097844));
#62121=CARTESIAN_POINT('Ctrl Pts',(-16.3146864551117,23.7899542488098,6.47535501215315));
#62122=CARTESIAN_POINT('Ctrl Pts',(-15.3296477791819,23.7362172980268,6.10632970857785));
#62123=CARTESIAN_POINT('Ctrl Pts',(-15.3971490025393,24.772616414018,5.93110659229477));
#62124=CARTESIAN_POINT('Ctrl Pts',(-16.326041455245,23.7855759764293,6.45350549629898));
#62125=CARTESIAN_POINT('Ctrl Pts',(-15.3377398062802,23.7292551260036,6.08623411212909));
#62126=CARTESIAN_POINT('Ctrl Pts',(-15.4078551454552,24.766757373037,5.90323831741779));
#62127=CARTESIAN_POINT('Ctrl Pts',(-16.3316870562881,23.7833238896394,6.44259808404498));
#62128=CARTESIAN_POINT('Ctrl Pts',(-15.3417617125046,23.725722850175,6.07622253802155));
#62129=CARTESIAN_POINT('Ctrl Pts',(-15.4131781407913,24.7637424872307,5.88932598557243));
#62130=CARTESIAN_POINT('Ctrl Pts',(-16.3597569709651,23.7717494556004,6.38814778227077));
#62131=CARTESIAN_POINT('Ctrl Pts',(-15.3617917351086,23.7077741903901,6.02624731012122));
#62132=CARTESIAN_POINT('Ctrl Pts',(-15.4396440601767,24.7482422328457,5.81987342823877));
#62133=CARTESIAN_POINT('Ctrl Pts',(-16.3817071352546,23.7614855762067,6.34486501522732));
#62134=CARTESIAN_POINT('Ctrl Pts',(-15.3774035575898,23.6926313283501,5.98692345337671));
#62135=CARTESIAN_POINT('Ctrl Pts',(-15.4603399296305,24.7344800177032,5.76466031221647));
#62136=CARTESIAN_POINT('Ctrl Pts',(-16.4460911353826,23.7276985047866,6.21585408598055));
#62137=CARTESIAN_POINT('Ctrl Pts',(-15.4233108987322,23.6447437182896,5.87028450901762));
#62138=CARTESIAN_POINT('Ctrl Pts',(-15.5210448436385,24.6891304564638,5.60007535499672));
#62139=CARTESIAN_POINT('Ctrl Pts',(-16.4870597369203,23.7011856762767,6.1309612979369));
#62140=CARTESIAN_POINT('Ctrl Pts',(-15.4524120750771,23.6097680793461,5.79496554732097));
#62141=CARTESIAN_POINT('Ctrl Pts',(-15.5596723827607,24.6534880145847,5.49175537508767));
#62142=CARTESIAN_POINT('Ctrl Pts',(-16.5653255738427,23.6401365395015,5.96347878929924));
#62143=CARTESIAN_POINT('Ctrl Pts',(-15.5082624063114,23.5338042852298,5.64817282485189));
#62144=CARTESIAN_POINT('Ctrl Pts',(-15.6334658856169,24.5713175830139,5.27802294063828));
#62145=CARTESIAN_POINT('Ctrl Pts',(-16.6026225537566,23.6056007131115,5.88088881453209));
#62146=CARTESIAN_POINT('Ctrl Pts',(-15.5349528356564,23.4928190256182,5.57683272933565));
#62147=CARTESIAN_POINT('Ctrl Pts',(-15.6686316100636,24.5247902538067,5.17261015704771));
#62148=CARTESIAN_POINT('Ctrl Pts',(-16.6737438347713,23.528267073217,5.71815276175897));
#62149=CARTESIAN_POINT('Ctrl Pts',(-15.5862895968411,23.404767618473,5.43765450767667));
#62150=CARTESIAN_POINT('Ctrl Pts',(-15.7356888173493,24.42052518513,4.96487762308654));
#62151=CARTESIAN_POINT('Ctrl Pts',(-16.7075680164773,23.4854706778622,5.63800609123987));
#62152=CARTESIAN_POINT('Ctrl Pts',(-15.6108864909551,23.3577197606882,5.36993478547871));
#62153=CARTESIAN_POINT('Ctrl Pts',(-15.7675801892024,24.3627893738512,4.86255711166091));
#62154=CARTESIAN_POINT('Ctrl Pts',(-16.7477821629421,23.4265259278568,5.53948762297091));
#62155=CARTESIAN_POINT('Ctrl Pts',(-15.640442194244,23.2950078236853,5.28746967965312));
#62156=CARTESIAN_POINT('Ctrl Pts',(-15.805496384108,24.2832257277335,4.73676835721291));
#62157=CARTESIAN_POINT('Ctrl Pts',(-16.7557216137502,23.4144639098627,5.51986739539677));
#62158=CARTESIAN_POINT('Ctrl Pts',(-15.6463076234428,23.2822371150873,5.27104653838932));
#62159=CARTESIAN_POINT('Ctrl Pts',(-15.8129821521461,24.2669424871855,4.71171648335875));
#62160=CARTESIAN_POINT('Ctrl Pts',(-16.7674774596505,23.395953969424,5.49056555479367));
#62161=CARTESIAN_POINT('Ctrl Pts',(-15.6550187536544,23.2627774898914,5.24657215146652));
#62162=CARTESIAN_POINT('Ctrl Pts',(-15.8240662353233,24.2419519469095,4.67430176293868));
#62163=CARTESIAN_POINT('Ctrl Pts',(-16.7713692055763,23.3897163634963,5.4808228929721));
#62164=CARTESIAN_POINT('Ctrl Pts',(-15.6579083290139,23.2562391945131,5.238439653045));
#62165=CARTESIAN_POINT('Ctrl Pts',(-15.827735595861,24.2335299973296,4.66186145875231));
#62166=CARTESIAN_POINT('Ctrl Pts',(-16.7790786053942,23.3771398737448,5.46143989175872));
#62167=CARTESIAN_POINT('Ctrl Pts',(-15.6636423926354,23.2430985419099,5.2222741523105));
#62168=CARTESIAN_POINT('Ctrl Pts',(-15.8350044584265,24.2165484323211,4.63711118636381));
#62169=CARTESIAN_POINT('Ctrl Pts',(-16.7828991720825,23.370796439779,5.45179230525798));
#62170=CARTESIAN_POINT('Ctrl Pts',(-15.6664889482879,23.236491490482,5.21423532879162));
#62171=CARTESIAN_POINT('Ctrl Pts',(-15.8386067071377,24.2079826737511,4.62479196472651));
#62172=CARTESIAN_POINT('Ctrl Pts',(-16.8018339398215,23.3388043651893,5.40377346815184));
#62173=CARTESIAN_POINT('Ctrl Pts',(-15.6806350337464,23.2032407115738,5.17421892820013));
#62174=CARTESIAN_POINT('Ctrl Pts',(-15.8564594878516,24.1647804218777,4.5634748554483));
#62175=CARTESIAN_POINT('Ctrl Pts',(-16.8164442132578,23.3123314605357,5.36605914410303));
#62176=CARTESIAN_POINT('Ctrl Pts',(-15.6916183434728,23.176080065211,5.14293310352819));
#62177=CARTESIAN_POINT('Ctrl Pts',(-15.8702348889878,24.1290241585185,4.51531351117569));
#62178=CARTESIAN_POINT('Ctrl Pts',(-16.8587554207317,23.2303040332693,5.25500886580051));
#62179=CARTESIAN_POINT('Ctrl Pts',(-15.7237160931746,23.0927127886327,5.05092031300736));
#62180=CARTESIAN_POINT('Ctrl Pts',(-15.9101283124877,24.0182117167204,4.37349553830628));
#62181=CARTESIAN_POINT('Ctrl Pts',(-16.8849395653287,23.1721462959427,5.18376112194714));
#62182=CARTESIAN_POINT('Ctrl Pts',(-15.7438852600433,23.0348480228381,4.99230333775579));
#62183=CARTESIAN_POINT('Ctrl Pts',(-15.9348162211413,23.9396193270414,4.28249928149494));
#62184=CARTESIAN_POINT('Ctrl Pts',(-16.9336814227243,23.0489054189936,5.04689481422135));
#62185=CARTESIAN_POINT('Ctrl Pts',(-15.7821317178199,22.9140451735304,4.87983224864429));
#62186=CARTESIAN_POINT('Ctrl Pts',(-15.9807728286811,23.7730294410803,4.10768400630364));
#62187=CARTESIAN_POINT('Ctrl Pts',(-16.9562386866201,22.9838226934723,4.98127579196471));
#62188=CARTESIAN_POINT('Ctrl Pts',(-15.8001793820112,22.8511599414675,4.82605841813765));
#62189=CARTESIAN_POINT('Ctrl Pts',(-16.0020411069034,23.6850325081959,4.02386439271881));
#62190=CARTESIAN_POINT('Ctrl Pts',(-16.987604927613,22.8808838764127,4.88722396565768));
#62191=CARTESIAN_POINT('Ctrl Pts',(-15.8257672390934,22.7527257626976,4.74893958754407));
#62192=CARTESIAN_POINT('Ctrl Pts',(-16.0316149906622,23.5458217813753,3.90371897690907));
#62193=CARTESIAN_POINT('Ctrl Pts',(-16.9976481065494,22.8456837005479,4.85660401111989));
#62194=CARTESIAN_POINT('Ctrl Pts',(-15.8340508273298,22.7192129009951,4.72381778995871));
#62195=CARTESIAN_POINT('Ctrl Pts',(-16.0410842740568,23.4982136910247,3.86460270090459));
#62196=CARTESIAN_POINT('Ctrl Pts',(-17.0121203952898,22.7915232573147,4.81180137192049));
#62197=CARTESIAN_POINT('Ctrl Pts',(-15.8461085603811,22.6678599797178,4.68703657852857));
#62198=CARTESIAN_POINT('Ctrl Pts',(-16.0547295745761,23.4249553174748,3.80736693372734));
#62199=CARTESIAN_POINT('Ctrl Pts',(-17.0168457071942,22.7732429751389,4.79705512920603));
#62200=CARTESIAN_POINT('Ctrl Pts',(-15.8500672783871,22.6505576473008,4.6749240778692));
#62201=CARTESIAN_POINT('Ctrl Pts',(-16.0591848688511,23.4002280123538,3.7885282309321));
#62202=CARTESIAN_POINT('Ctrl Pts',(-17.0237883943477,22.7454776880105,4.77522247845058));
#62203=CARTESIAN_POINT('Ctrl Pts',(-15.8559136123358,22.6243253288571,4.65698351812611));
#62204=CARTESIAN_POINT('Ctrl Pts',(-16.0657308308803,23.3626690002606,3.76063612595374));
#62205=CARTESIAN_POINT('Ctrl Pts',(-17.0260800299871,22.7361583484969,4.76798756875114));
#62206=CARTESIAN_POINT('Ctrl Pts',(-15.8578486816174,22.6155273689921,4.65103648873815));
#62207=CARTESIAN_POINT('Ctrl Pts',(-16.0678915160203,23.3500621669768,3.7513931759135));
#62208=CARTESIAN_POINT('Ctrl Pts',(-17.0306066910047,22.7174397302962,4.75364159618235));
#62209=CARTESIAN_POINT('Ctrl Pts',(-15.8616810873489,22.5978702503389,4.63924108014801));
#62210=CARTESIAN_POINT('Ctrl Pts',(-16.0721595105729,23.3247398553012,3.73306538887138));
#62211=CARTESIAN_POINT('Ctrl Pts',(-17.0328409840293,22.7080437567381,4.7465329043636));
#62212=CARTESIAN_POINT('Ctrl Pts',(-15.8635777645221,22.5890142967341,4.63339474291903));
#62213=CARTESIAN_POINT('Ctrl Pts',(-16.0742661298305,23.3120288483462,3.72398358138302));
#62214=CARTESIAN_POINT('Ctrl Pts',(-17.0526933776313,22.6231517872467,4.68313072942519));
#62215=CARTESIAN_POINT('Ctrl Pts',(-15.8804833690792,22.5090194337291,4.58120893371147));
#62216=CARTESIAN_POINT('Ctrl Pts',(-16.0929841004056,23.1971835740226,3.64298279899934));
#62217=CARTESIAN_POINT('Ctrl Pts',(-17.0685242872246,22.5453639920906,4.63085999071918));
#62218=CARTESIAN_POINT('Ctrl Pts',(-15.894267957528,22.4362044579173,4.53811448983722));
#62219=CARTESIAN_POINT('Ctrl Pts',(-16.1079103874777,23.0919335002713,3.57619999707222));
#62220=CARTESIAN_POINT('Ctrl Pts',(-17.0970409468598,22.3852544776922,4.53433068617298));
#62221=CARTESIAN_POINT('Ctrl Pts',(-15.9195637292118,22.2867607205428,4.4582405737583));
#62222=CARTESIAN_POINT('Ctrl Pts',(-16.1347975228886,22.8752733800206,3.45286726728094));
#62223=CARTESIAN_POINT('Ctrl Pts',(-17.1097258727485,22.3029325841582,4.4900723356221));
#62224=CARTESIAN_POINT('Ctrl Pts',(-15.9310656586748,22.2101710019765,4.42148888099321));
#62225=CARTESIAN_POINT('Ctrl Pts',(-16.1467575966226,22.7638630897231,3.39631760321678));
#62226=CARTESIAN_POINT('Ctrl Pts',(-17.1322932109451,22.1337448915264,4.40963331225656));
#62227=CARTESIAN_POINT('Ctrl Pts',(-15.9518657706561,22.0529296192241,4.35443896699023));
#62228=CARTESIAN_POINT('Ctrl Pts',(-16.1680353719467,22.5348731855549,3.29353705876987));
#62229=CARTESIAN_POINT('Ctrl Pts',(-17.1421754383553,22.0468795660126,4.37345174155353));
#62230=CARTESIAN_POINT('Ctrl Pts',(-15.9611598177471,21.9723049166285,4.32415374113437));
#62231=CARTESIAN_POINT('Ctrl Pts',(-16.1773529012751,22.4172942062458,3.2473050216081));
#62232=CARTESIAN_POINT('Ctrl Pts',(-17.1518385746547,21.9465183910894,4.33745974767627));
#62233=CARTESIAN_POINT('Ctrl Pts',(-15.9703702643961,21.8791492254028,4.29392263795542));
#62234=CARTESIAN_POINT('Ctrl Pts',(-16.1864638580397,22.2814390641004,3.20131455964727));
#62235=CARTESIAN_POINT('Ctrl Pts',(-17.1528919760102,21.9353304202433,4.33352625030006));
#62236=CARTESIAN_POINT('Ctrl Pts',(-15.971376200346,21.8687654542568,4.29061743074886));
#62237=CARTESIAN_POINT('Ctrl Pts',(-16.1874570651016,22.266294214612,3.19628833747367));
#62238=CARTESIAN_POINT('Ctrl Pts',(-17.1549585027494,21.9128805671971,4.32579136175763));
#62239=CARTESIAN_POINT('Ctrl Pts',(-15.9733532131519,21.8479295159697,4.28411514135217));
#62240=CARTESIAN_POINT('Ctrl Pts',(-16.1894055045299,22.2359042417173,3.18640467936431));
#62241=CARTESIAN_POINT('Ctrl Pts',(-17.1559725748067,21.9016073705072,4.32198639190832));
#62242=CARTESIAN_POINT('Ctrl Pts',(-15.9743252013516,21.8374668715494,4.28091504945802));
#62243=CARTESIAN_POINT('Ctrl Pts',(-16.1903616296819,22.2206438017773,3.1815426702273));
#62244=CARTESIAN_POINT('Ctrl Pts',(-17.1589399035528,21.8678484081765,4.31082703161848));
#62245=CARTESIAN_POINT('Ctrl Pts',(-15.9771743658607,21.8061355673508,4.27152575218795));
#62246=CARTESIAN_POINT('Ctrl Pts',(-16.1931593966801,22.1749442360078,3.16728315802819));
#62247=CARTESIAN_POINT('Ctrl Pts',(-17.160830065973,21.8452936463181,4.30368403020251));
#62248=CARTESIAN_POINT('Ctrl Pts',(-15.9789960926506,21.7852025809683,4.26551018369033));
#62249=CARTESIAN_POINT('Ctrl Pts',(-16.1949415499539,22.1444113936572,3.15815574296063));
#62250=CARTESIAN_POINT('Ctrl Pts',(-17.1662452354044,21.7774846198971,4.28313524343019));
#62251=CARTESIAN_POINT('Ctrl Pts',(-15.9842317551839,21.7222686670546,4.24819136151219));
#62252=CARTESIAN_POINT('Ctrl Pts',(-16.2000472809384,22.0526157783281,3.13189816377041));
#62253=CARTESIAN_POINT('Ctrl Pts',(-17.1695152559525,21.7320857415583,4.27060912258618));
#62254=CARTESIAN_POINT('Ctrl Pts',(-15.9874166448608,21.6801299212902,4.23761463613163));
#62255=CARTESIAN_POINT('Ctrl Pts',(-16.2031304438779,21.9911560722748,3.11589195795755));
#62256=CARTESIAN_POINT('Ctrl Pts',(-17.1724645676383,21.6864970381169,4.25923772206483));
#62257=CARTESIAN_POINT('Ctrl Pts',(-15.9903039058086,21.6378054978787,4.22799974991249));
#62258=CARTESIAN_POINT('Ctrl Pts',(-16.2059112228881,21.9294381812241,3.10136122305517));
#62259=CARTESIAN_POINT('Origin',(-13.7285795279453,20.5440037453176,10.8524699559538));
#62260=CARTESIAN_POINT('Ctrl Pts',(-12.9440892692056,20.5440037453176,10.2323288156136));
#62261=CARTESIAN_POINT('Ctrl Pts',(-13.2371163881454,20.6161954472713,9.8616439740488));
#62262=CARTESIAN_POINT('Ctrl Pts',(-13.7129564349448,20.6615335048059,9.85952349485951));
#62263=CARTESIAN_POINT('Ctrl Pts',(-12.9499039917696,20.44636701263,10.2249730817137));
#62264=CARTESIAN_POINT('Ctrl Pts',(-13.241415803247,20.541538390444,9.85197635982406));
#62265=CARTESIAN_POINT('Ctrl Pts',(-13.71912369608,20.6132210786213,9.8537079753423));
#62266=CARTESIAN_POINT('Ctrl Pts',(-12.9620352057415,20.3514474462748,10.2172624474079));
#62267=CARTESIAN_POINT('Ctrl Pts',(-13.2507379167627,20.4690074406104,9.83990414196894));
#62268=CARTESIAN_POINT('Ctrl Pts',(-13.73052511494,20.5662589469414,9.84673198254351));
#62269=CARTESIAN_POINT('Ctrl Pts',(-12.9971745343112,20.1663051389932,10.2011795440461));
#62270=CARTESIAN_POINT('Ctrl Pts',(-13.2778281273366,20.3275502669037,9.81157043613493));
#62271=CARTESIAN_POINT('Ctrl Pts',(-13.7623139834302,20.4746690904462,9.83075639181578));
#62272=CARTESIAN_POINT('Ctrl Pts',(-13.0201906855957,20.0760819079927,10.1928069593359));
#62273=CARTESIAN_POINT('Ctrl Pts',(-13.2957015322063,20.2584188213895,9.79523255295137));
#62274=CARTESIAN_POINT('Ctrl Pts',(-13.7827076838172,20.4300420744267,9.82175563922042));
#62275=CARTESIAN_POINT('Ctrl Pts',(-13.0619887611901,19.943864781223,10.1797878662283));
#62276=CARTESIAN_POINT('Ctrl Pts',(-13.3279845155654,20.1571560277764,9.76790383700773));
#62277=CARTESIAN_POINT('Ctrl Pts',(-13.8192667855096,20.3646560151673,9.80690367763832));
#62278=CARTESIAN_POINT('Ctrl Pts',(-13.0771373948911,19.9003134539564,10.1753714795664));
#62279=CARTESIAN_POINT('Ctrl Pts',(-13.3397248017635,20.1236498181765,9.75827221102949));
#62280=CARTESIAN_POINT('Ctrl Pts',(-13.8324507812609,20.3431204394681,9.80172742386782));
#62281=CARTESIAN_POINT('Ctrl Pts',(-13.1097549160981,19.8142002694475,10.1663917888589));
#62282=CARTESIAN_POINT('Ctrl Pts',(-13.3649782408832,20.0572725875454,9.73806010509094));
#62283=CARTESIAN_POINT('Ctrl Pts',(-13.8607136480924,20.3005431616034,9.79094716660411));
#62284=CARTESIAN_POINT('Ctrl Pts',(-13.1271023780073,19.7719591983959,10.1618619296081));
#62285=CARTESIAN_POINT('Ctrl Pts',(-13.378414869638,20.0246324390144,9.72754343587429));
#62286=CARTESIAN_POINT('Ctrl Pts',(-13.8756872686222,20.2796600689745,9.7853833256429));
#62287=CARTESIAN_POINT('Ctrl Pts',(-13.1819446233167,19.6476137998266,10.1481790406719));
#62288=CARTESIAN_POINT('Ctrl Pts',(-13.4209825632648,19.9280025133646,9.69479688704902));
#62289=CARTESIAN_POINT('Ctrl Pts',(-13.9228611331578,20.2181935537061,9.76823863621524));
#62290=CARTESIAN_POINT('Ctrl Pts',(-13.2222530148998,19.5678087202178,10.1389253299632));
#62291=CARTESIAN_POINT('Ctrl Pts',(-13.4522143245307,19.8657922607512,9.67150098704121));
#62292=CARTESIAN_POINT('Ctrl Pts',(-13.9573288153533,20.1787520795032,9.75619699835315));
#62293=CARTESIAN_POINT('Ctrl Pts',(-13.2658111744658,19.4906334205523,10.1295681579593));
#62294=CARTESIAN_POINT('Ctrl Pts',(-13.4855881182943,19.805690718136,9.64706941350936));
#62295=CARTESIAN_POINT('Ctrl Pts',(-13.9943709817605,20.1406244663728,9.74364801533399));
#62296=CARTESIAN_POINT('Origin',(-14.0099940747611,19.8417568621407,10.6978147062773));
#62297=CARTESIAN_POINT('Ctrl Pts',(-13.2658111744658,19.4906334205524,10.1295681579593));
#62298=CARTESIAN_POINT('Ctrl Pts',(-13.4855881182943,19.805690718136,9.64706941350936));
#62299=CARTESIAN_POINT('Ctrl Pts',(-13.9943709817605,20.1406244663728,9.74364801533399));
#62300=CARTESIAN_POINT('Ctrl Pts',(-13.3330814724857,19.3942003585853,10.1010567716054));
#62301=CARTESIAN_POINT('Ctrl Pts',(-13.5481243107023,19.7256553494083,9.61136837775977));
#62302=CARTESIAN_POINT('Ctrl Pts',(-14.0638031593701,20.0691577022518,9.72012608131962));
#62303=CARTESIAN_POINT('Ctrl Pts',(-13.4011178460067,19.3003908944215,10.0693235708264));
#62304=CARTESIAN_POINT('Ctrl Pts',(-13.6107780087442,19.6487795554127,9.57278594043353));
#62305=CARTESIAN_POINT('Ctrl Pts',(-14.134073189902,19.9996605572184,9.69412178028956));
#62306=CARTESIAN_POINT('Ctrl Pts',(-13.5384187734267,19.1175030228593,9.99981903770995));
#62307=CARTESIAN_POINT('Ctrl Pts',(-13.7365209035852,19.5001155576116,9.49010774169617));
#62308=CARTESIAN_POINT('Ctrl Pts',(-14.2759620462211,19.864217269711,9.63746756082801));
#62309=CARTESIAN_POINT('Ctrl Pts',(-13.6076846066159,19.0284254449248,9.96204590686114));
#62310=CARTESIAN_POINT('Ctrl Pts',(-13.7996545986511,19.4283439661347,9.44591917852276));
#62311=CARTESIAN_POINT('Ctrl Pts',(-14.3475817493338,19.7982722534542,9.6068163939335));
#62312=CARTESIAN_POINT('Ctrl Pts',(-13.7472084791682,18.8546463637298,9.88068555234443));
#62313=CARTESIAN_POINT('Ctrl Pts',(-13.9260237622311,19.2896983531623,9.35234401028892));
#62314=CARTESIAN_POINT('Ctrl Pts',(-14.4919140997087,19.6696686338088,9.54104741527293));
#62315=CARTESIAN_POINT('Ctrl Pts',(-13.8174669907381,18.7699457923012,9.83709751132101));
#62316=CARTESIAN_POINT('Ctrl Pts',(-13.989298667415,19.2228465000766,9.3028621243836));
#62317=CARTESIAN_POINT('Ctrl Pts',(-14.5646272658253,19.6070107231862,9.50592896453078));
#62318=CARTESIAN_POINT('Ctrl Pts',(-13.9587830475483,18.6046925960041,9.74419189541089));
#62319=CARTESIAN_POINT('Ctrl Pts',(-14.1156416099841,19.0939700992305,9.19891658502328));
#62320=CARTESIAN_POINT('Ctrl Pts',(-14.7109393570737,19.4848097716012,9.43129554138823));
#62321=CARTESIAN_POINT('Ctrl Pts',(-14.0298409119678,18.5241404513239,9.69487401464713));
#62322=CARTESIAN_POINT('Ctrl Pts',(-14.1787445834152,19.0319737530083,9.14435360774552));
#62323=CARTESIAN_POINT('Ctrl Pts',(-14.7845386303077,19.4252670888976,9.39178032763476));
#62324=CARTESIAN_POINT('Ctrl Pts',(-14.172594896334,18.3670608910262,9.59046937668944));
#62325=CARTESIAN_POINT('Ctrl Pts',(-14.3044456978952,18.9128418187715,9.03038842549872));
#62326=CARTESIAN_POINT('Ctrl Pts',(-14.9324519926951,19.3092027818523,9.30832722037077));
#62327=CARTESIAN_POINT('Ctrl Pts',(-14.2442912388678,18.290533610001,9.53538273635831));
#62328=CARTESIAN_POINT('Ctrl Pts',(-14.3670741811423,18.8557416967525,8.97088159072191));
#62329=CARTESIAN_POINT('Ctrl Pts',(-15.0067663210554,19.2526812602515,9.26438941351549));
#62330=CARTESIAN_POINT('Ctrl Pts',(-14.3342253809499,18.1973729705646,9.4628184729282));
#62331=CARTESIAN_POINT('Ctrl Pts',(-14.4444128857855,18.7878761408221,8.89396908392269));
#62332=CARTESIAN_POINT('Ctrl Pts',(-15.1000164536366,19.183903311546,9.2066277940443));
#62333=CARTESIAN_POINT('Ctrl Pts',(-14.3522279465606,18.1788659986889,9.44812001590431));
#62334=CARTESIAN_POINT('Ctrl Pts',(-14.4599444650823,18.7743836756288,8.87834625763803));
#62335=CARTESIAN_POINT('Ctrl Pts',(-15.1186844003074,19.1702415919389,9.19493326466006));
#62336=CARTESIAN_POINT('Ctrl Pts',(-14.3882626111411,18.1421028768693,9.41834812676606));
#62337=CARTESIAN_POINT('Ctrl Pts',(-14.4909537332673,18.7477161457633,8.84679920366087));
#62338=CARTESIAN_POINT('Ctrl Pts',(-15.1560541122317,19.1431062284371,9.17125694190101));
#62339=CARTESIAN_POINT('Ctrl Pts',(-14.4062921839539,18.1238495975253,9.40327640825083));
#62340=CARTESIAN_POINT('Ctrl Pts',(-14.506429325642,18.734544214775,8.83087535507227));
#62341=CARTESIAN_POINT('Ctrl Pts',(-15.1747532613805,19.1296347066541,9.15927652287954));
#62342=CARTESIAN_POINT('Ctrl Pts',(-14.4602437915794,18.0696447756957,9.35764595009415));
#62343=CARTESIAN_POINT('Ctrl Pts',(-14.552706703401,18.6955593831637,8.78271897853221));
#62344=CARTESIAN_POINT('Ctrl Pts',(-15.2307132513,19.0896341081692,9.1230214409286));
#62345=CARTESIAN_POINT('Ctrl Pts',(-14.4960880148582,18.0341872413021,9.32662342484023));
#62346=CARTESIAN_POINT('Ctrl Pts',(-14.5832283257351,18.6703926017591,8.75023077828758));
#62347=CARTESIAN_POINT('Ctrl Pts',(-15.2678981242241,19.0634739638261,9.09839438287258));
#62348=CARTESIAN_POINT('Ctrl Pts',(-14.6032291315409,17.9298203314146,9.23175293631501));
#62349=CARTESIAN_POINT('Ctrl Pts',(-14.6743100165152,18.5968732851352,8.6511117608008));
#62350=CARTESIAN_POINT('Ctrl Pts',(-15.379065193414,18.9864901941371,9.02314519607624));
#62351=CARTESIAN_POINT('Ctrl Pts',(-14.6741346420556,17.8629129481122,9.16610483335341));
#62352=CARTESIAN_POINT('Ctrl Pts',(-14.7336451616916,18.551149480899,8.58356324766789));
#62353=CARTESIAN_POINT('Ctrl Pts',(-15.4526599555671,18.9371604904354,8.97115719890328));
#62354=CARTESIAN_POINT('Ctrl Pts',(-14.8147873839916,17.7343652083541,9.02995827635105));
#62355=CARTESIAN_POINT('Ctrl Pts',(-14.8498233491032,18.465729859472,8.44542324423527));
#62356=CARTESIAN_POINT('Ctrl Pts',(-15.5986969684513,18.8424271750069,8.8635008260648));
#62357=CARTESIAN_POINT('Ctrl Pts',(-14.8845347880239,17.6727249346549,8.95945991700377));
#62358=CARTESIAN_POINT('Ctrl Pts',(-14.9066386172608,18.4261260159142,8.37476291962935));
#62359=CARTESIAN_POINT('Ctrl Pts',(-15.6711394016455,18.7970236297136,8.80783252485449));
#62360=CARTESIAN_POINT('Ctrl Pts',(-15.0227496766711,17.554755527474,8.81347462073762));
#62361=CARTESIAN_POINT('Ctrl Pts',(-15.017521019286,18.3530371598327,8.23067374372871));
#62362=CARTESIAN_POINT('Ctrl Pts',(-15.8147470349955,18.710170616878,8.69270927527942));
#62363=CARTESIAN_POINT('Ctrl Pts',(-15.0912173674794,17.4984260829599,8.73798808677873));
#62364=CARTESIAN_POINT('Ctrl Pts',(-15.0715513182918,18.3196525669407,8.15718105412623));
#62365=CARTESIAN_POINT('Ctrl Pts',(-15.8859124457149,18.6687209251363,8.6332546393608));
#62366=CARTESIAN_POINT('Ctrl Pts',(-15.2267381193355,17.3912430464634,8.58179117703503));
#62367=CARTESIAN_POINT('Ctrl Pts',(-15.1765900387789,18.2591644871512,8.00772044998079));
#62368=CARTESIAN_POINT('Ctrl Pts',(-16.0268297452482,18.5898927447856,8.51037741448558));
#62369=CARTESIAN_POINT('Ctrl Pts',(-15.293791452939,17.3403886748865,8.501081594441));
#62370=CARTESIAN_POINT('Ctrl Pts',(-15.2275513509012,18.2321712357141,7.93169574084797));
#62371=CARTESIAN_POINT('Ctrl Pts',(-16.096581905656,18.5525136868114,8.44695543962988));
#62372=CARTESIAN_POINT('Ctrl Pts',(-15.3931943675008,17.2684399247589,8.37583698834224));
#62373=CARTESIAN_POINT('Ctrl Pts',(-15.3011653770819,18.1967256137164,7.81658549406654));
#62374=CARTESIAN_POINT('Ctrl Pts',(-16.2000338179115,18.4996619197496,8.34864407946271));
#62375=CARTESIAN_POINT('Ctrl Pts',(-15.4261323093676,17.2451802795294,8.3333911142032));
#62376=CARTESIAN_POINT('Ctrl Pts',(-15.3253918923598,18.1856916248434,7.77776130742633));
#62377=CARTESIAN_POINT('Ctrl Pts',(-16.2343215641098,18.4825816407125,8.3153431447716));
#62378=CARTESIAN_POINT('Ctrl Pts',(-15.4752281274295,17.2114155910319,8.2686329570956));
#62379=CARTESIAN_POINT('Ctrl Pts',(-15.3609931745526,18.1704326848487,7.71929023227925));
#62380=CARTESIAN_POINT('Ctrl Pts',(-16.2854423994633,18.4577956901338,8.26456294500476));
#62381=CARTESIAN_POINT('Ctrl Pts',(-15.4915424610904,17.2003476249094,8.24686402229588));
#62382=CARTESIAN_POINT('Ctrl Pts',(-15.3727782070634,18.1655464655944,7.69968995222783));
#62383=CARTESIAN_POINT('Ctrl Pts',(-16.3024318301415,18.4496723941997,8.24749704105937));
#62384=CARTESIAN_POINT('Ctrl Pts',(-15.5240607039472,17.1785970420959,8.20295981544979));
#62385=CARTESIAN_POINT('Ctrl Pts',(-15.3961216670957,18.1562002365569,7.66037502911479));
#62386=CARTESIAN_POINT('Ctrl Pts',(-16.3363002450403,18.4337115689635,8.21308653597584));
#62387=CARTESIAN_POINT('Ctrl Pts',(-15.540218113459,17.167945517914,8.1808873369451));
#62388=CARTESIAN_POINT('Ctrl Pts',(-15.4076453357983,18.1517557131201,7.64071660882628));
#62389=CARTESIAN_POINT('Ctrl Pts',(-16.3531307989921,18.4258968558046,8.19579114970188));
#62390=CARTESIAN_POINT('Ctrl Pts',(-15.6204924118291,17.1158115451059,8.06991972797963));
#62391=CARTESIAN_POINT('Ctrl Pts',(-15.4649374078242,18.130506147785,7.5417338527351));
#62392=CARTESIAN_POINT('Ctrl Pts',(-16.4367611376568,18.387655095655,8.10886079937315));
#62393=CARTESIAN_POINT('Ctrl Pts',(-15.6830729216002,17.0776936936504,7.97921160142153));
#62394=CARTESIAN_POINT('Ctrl Pts',(-15.5080251086504,18.117315035564,7.46318153823152));
#62395=CARTESIAN_POINT('Ctrl Pts',(-16.5019954870926,18.3597187740705,8.03786762531124));
#62396=CARTESIAN_POINT('Ctrl Pts',(-15.8048218294665,17.0088582451554,7.79379764598993));
#62397=CARTESIAN_POINT('Ctrl Pts',(-15.589527127849,18.0978396117853,7.30672177657495));
#62398=CARTESIAN_POINT('Ctrl Pts',(-16.6289910393939,18.3093178392552,7.89287905000511));
#62399=CARTESIAN_POINT('Ctrl Pts',(-15.8639905947732,16.9781397369617,7.6990922607597));
#62400=CARTESIAN_POINT('Ctrl Pts',(-15.6278243988214,18.0916954466089,7.22887816643367));
#62401=CARTESIAN_POINT('Ctrl Pts',(-16.6907526087972,18.2868525602906,7.81888399718693));
#62402=CARTESIAN_POINT('Ctrl Pts',(-15.9787302986795,16.9244976836848,7.50547883953967));
#62403=CARTESIAN_POINT('Ctrl Pts',(-15.6997459333507,18.0861054933015,7.07442364118823));
#62404=CARTESIAN_POINT('Ctrl Pts',(-16.8106182005044,18.2476791889588,7.66772898825296));
#62405=CARTESIAN_POINT('Ctrl Pts',(-16.0343018499712,16.9015724052595,7.40657160377054));
#62406=CARTESIAN_POINT('Ctrl Pts',(-15.7332497211822,18.0867900683191,6.99790376875797));
#62407=CARTESIAN_POINT('Ctrl Pts',(-16.8687228322341,18.2309698251075,7.59056965666333));
#62408=CARTESIAN_POINT('Ctrl Pts',(-16.1147718948553,16.8734859053583,7.25483467642257));
#62409=CARTESIAN_POINT('Ctrl Pts',(-15.7798484592268,18.092614771922,6.88499408884766));
#62410=CARTESIAN_POINT('Ctrl Pts',(-16.9529490202363,18.2105552719868,7.4722804229554));
#62411=CARTESIAN_POINT('Ctrl Pts',(-16.1411134573278,16.865175788199,7.20369221675809));
#62412=CARTESIAN_POINT('Ctrl Pts',(-15.7948569320189,18.0953910933679,6.84743092050601));
#62413=CARTESIAN_POINT('Ctrl Pts',(-16.9805353881954,18.2045266761679,7.43242501444395));
#62414=CARTESIAN_POINT('Ctrl Pts',(-16.179873357956,16.8543648698465,7.12609670173211));
#62415=CARTESIAN_POINT('Ctrl Pts',(-15.8164668360564,18.1007300607159,6.79160558134888));
#62416=CARTESIAN_POINT('Ctrl Pts',(-17.0211518386022,18.1967038372177,7.37197466884147));
#62417=CARTESIAN_POINT('Ctrl Pts',(-16.1926678712388,16.851037084605,7.1000844945737));
#62418=CARTESIAN_POINT('Ctrl Pts',(-15.8235412294377,18.1027139619363,6.77302390988603));
#62419=CARTESIAN_POINT('Ctrl Pts',(-17.0345634258717,18.1942996744008,7.35171329796697));
#62420=CARTESIAN_POINT('Ctrl Pts',(-16.2180004190603,16.8449478242919,7.04775905974781));
#62421=CARTESIAN_POINT('Ctrl Pts',(-15.8374071874885,18.1070733465416,6.73600069327743));
#62422=CARTESIAN_POINT('Ctrl Pts',(-17.0611266078686,18.1899089301747,7.31096259568511));
#62423=CARTESIAN_POINT('Ctrl Pts',(-16.2305410528683,16.8421866209048,7.021438990984));
#62424=CARTESIAN_POINT('Ctrl Pts',(-15.8441979516698,18.1094515393965,6.71755750861181));
#62425=CARTESIAN_POINT('Ctrl Pts',(-17.0742809443064,18.1879225621902,7.29046794760879));
#62426=CARTESIAN_POINT('Ctrl Pts',(-16.2922822294683,16.8298893484966,6.88973237378449));
#62427=CARTESIAN_POINT('Ctrl Pts',(-15.8775127685803,18.1223215324931,6.6255585108361));
#62428=CARTESIAN_POINT('Ctrl Pts',(-17.1390667357784,18.1791017859522,7.18792777564085));
#62429=CARTESIAN_POINT('Ctrl Pts',(-16.3388527132311,16.82480604532,6.78351336529713));
#62430=CARTESIAN_POINT('Ctrl Pts',(-15.9012994364871,18.1354945701909,6.55484584731165));
#62431=CARTESIAN_POINT('Ctrl Pts',(-17.1880086635335,18.1755473529931,7.105281360654));
#62432=CARTESIAN_POINT('Ctrl Pts',(-16.42625671668,16.8244865951818,6.56935996317588));
#62433=CARTESIAN_POINT('Ctrl Pts',(-15.9444744339779,18.166665793471,6.41786159094849));
#62434=CARTESIAN_POINT('Ctrl Pts',(-17.2800328788574,18.175687345345,6.93874263504849));
#62435=CARTESIAN_POINT('Ctrl Pts',(-16.4670907877957,16.8292488785245,6.46142568826117));
#62436=CARTESIAN_POINT('Ctrl Pts',(-15.9637438210817,18.1847031383132,6.35181980812632));
#62437=CARTESIAN_POINT('Ctrl Pts',(-17.3231157119331,18.1793806176926,6.85485042618645));
#62438=CARTESIAN_POINT('Ctrl Pts',(-16.5428322128861,16.8492020210022,6.24380857126078));
#62439=CARTESIAN_POINT('Ctrl Pts',(-15.998670856686,18.2247711780283,6.2238904177288));
#62440=CARTESIAN_POINT('Ctrl Pts',(-17.4032368975643,18.1944406370503,6.685783601792));
#62441=CARTESIAN_POINT('Ctrl Pts',(-16.5777406346628,16.8643899311763,6.13412597445859));
#62442=CARTESIAN_POINT('Ctrl Pts',(-16.0142343185671,18.2467999928255,6.16223101846773));
#62443=CARTESIAN_POINT('Ctrl Pts',(-17.4402763132042,18.2058052131984,6.60060918559835));
#62444=CARTESIAN_POINT('Ctrl Pts',(-16.6135037166622,16.887843870671,6.00971363205832));
#62445=CARTESIAN_POINT('Ctrl Pts',(-16.0301006340142,18.2733421491226,6.09509973493942));
#62446=CARTESIAN_POINT('Ctrl Pts',(-17.4783728672101,18.2232745427781,6.50403280278535));
#62447=CARTESIAN_POINT('Ctrl Pts',(-16.6174285656065,16.8905385400829,5.99587585692918));
#62448=CARTESIAN_POINT('Ctrl Pts',(-16.0318496897817,18.2763319679881,6.08763237324531));
#62449=CARTESIAN_POINT('Ctrl Pts',(-17.4825561029328,18.225280813882,6.49329158746432));
#62450=CARTESIAN_POINT('Ctrl Pts',(-16.6251798307496,16.8961074160593,5.96817177686506));
#62451=CARTESIAN_POINT('Ctrl Pts',(-16.0353047841429,18.2823634442865,6.07275077263818));
#62452=CARTESIAN_POINT('Ctrl Pts',(-17.4908223733553,18.2294254288441,6.47178799400402));
#62453=CARTESIAN_POINT('Ctrl Pts',(-16.6290088701947,16.8989837089351,5.95429578968276));
#62454=CARTESIAN_POINT('Ctrl Pts',(-16.0370118502271,18.2854071690753,6.06533182326545));
#62455=CARTESIAN_POINT('Ctrl Pts',(-17.4949082093827,18.2315653247675,6.46101810150374));
#62456=CARTESIAN_POINT('Ctrl Pts',(-16.640327690256,16.9078699152518,5.9126963948273));
#62457=CARTESIAN_POINT('Ctrl Pts',(-16.0420655799591,18.2946050780723,6.04317482379761));
#62458=CARTESIAN_POINT('Ctrl Pts',(-17.5069934597519,18.2381741848721,6.42873203287291));
#62459=CARTESIAN_POINT('Ctrl Pts',(-16.6476390588876,16.9141283412814,5.88504004653775));
#62460=CARTESIAN_POINT('Ctrl Pts',(-16.0453328192631,18.3008046027441,6.02858871996637));
#62461=CARTESIAN_POINT('Ctrl Pts',(-17.5148098007386,18.2428257703185,6.40726933694612));
#62462=CARTESIAN_POINT('Ctrl Pts',(-16.668876924417,16.9339042773692,5.8023015083001));
#62463=CARTESIAN_POINT('Ctrl Pts',(-16.0548762168224,18.3196280402113,5.9852540398304));
#62464=CARTESIAN_POINT('Ctrl Pts',(-17.53754506196,18.2575159307706,6.34306548117756));
#62465=CARTESIAN_POINT('Ctrl Pts',(-16.6821074672649,16.9484219473983,5.74744970190452));
#62466=CARTESIAN_POINT('Ctrl Pts',(-16.0608653387976,18.3324239286334,5.95705652973751));
#62467=CARTESIAN_POINT('Ctrl Pts',(-17.5517505124874,18.2682895399416,6.30050845290031));
#62468=CARTESIAN_POINT('Ctrl Pts',(-16.7190627591152,16.9959765026082,5.58382645621117));
#62469=CARTESIAN_POINT('Ctrl Pts',(-16.0779779753248,18.3716198957327,5.87385449259152));
#62470=CARTESIAN_POINT('Ctrl Pts',(-17.5915635598182,18.3035512121968,6.17357906259382));
#62471=CARTESIAN_POINT('Ctrl Pts',(-16.7400555978829,17.0330066603434,5.47598507636511));
#62472=CARTESIAN_POINT('Ctrl Pts',(-16.0881503846021,18.3985925034547,5.82073746488337));
#62473=CARTESIAN_POINT('Ctrl Pts',(-17.614372369325,18.3309739871534,6.08994669325491));
#62474=CARTESIAN_POINT('Ctrl Pts',(-16.7748996695109,17.1179178086824,5.26288874533716));
#62475=CARTESIAN_POINT('Ctrl Pts',(-16.1068711035242,18.4545293431909,5.71670683995154));
#62476=CARTESIAN_POINT('Ctrl Pts',(-17.6526840179692,18.3937954811266,5.92472292226959));
#62477=CARTESIAN_POINT('Ctrl Pts',(-16.7887511957117,17.165797405872,5.15763334311937));
#62478=CARTESIAN_POINT('Ctrl Pts',(-16.1153790545225,18.4834009489052,5.6659869756034));
#62479=CARTESIAN_POINT('Ctrl Pts',(-17.6681871322247,18.4291931720276,5.84313118244005));
#62480=CARTESIAN_POINT('Ctrl Pts',(-16.8041731774862,17.2461122278424,5.00182303805251));
#62481=CARTESIAN_POINT('Ctrl Pts',(-16.1271293851317,18.5287334432286,5.59018616575563));
#62482=CARTESIAN_POINT('Ctrl Pts',(-17.6859716250702,18.488536683831,5.72236773806957));
#62483=CARTESIAN_POINT('Ctrl Pts',(-16.80842012977,17.2743020559593,4.95023234528506));
#62484=CARTESIAN_POINT('Ctrl Pts',(-16.1308693537085,18.5441726270768,5.56499312469953));
#62485=CARTESIAN_POINT('Ctrl Pts',(-17.6909869150959,18.5093607347263,5.68238443728928));
#62486=CARTESIAN_POINT('Ctrl Pts',(-16.8134387928951,17.3187824429628,4.87338836572715));
#62487=CARTESIAN_POINT('Ctrl Pts',(-16.1362139667238,18.5679584891248,5.52711906840436));
#62488=CARTESIAN_POINT('Ctrl Pts',(-17.6971302169662,18.5422117789673,5.62283295445145));
#62489=CARTESIAN_POINT('Ctrl Pts',(-16.8148874382565,17.3339975860732,4.84782944445022));
#62490=CARTESIAN_POINT('Ctrl Pts',(-16.1379523469422,18.5759993141217,5.51446949942686));
#62491=CARTESIAN_POINT('Ctrl Pts',(-17.6989495862611,18.5534478320083,5.60302622434831));
#62492=CARTESIAN_POINT('Ctrl Pts',(-16.8173177844478,17.3649734626395,4.79721739740923));
#62493=CARTESIAN_POINT('Ctrl Pts',(-16.1413150962685,18.5922074383504,5.48928101372498));
#62494=CARTESIAN_POINT('Ctrl Pts',(-17.7021076435685,18.5763207522729,5.56380568192218));
#62495=CARTESIAN_POINT('Ctrl Pts',(-16.81830211771,17.3807509529757,4.77213331007082));
#62496=CARTESIAN_POINT('Ctrl Pts',(-16.1429414050274,18.6003821235283,5.47672970918627));
#62497=CARTESIAN_POINT('Ctrl Pts',(-17.703449425713,18.5879699978769,5.54436787357638));
#62498=CARTESIAN_POINT('Ctrl Pts',(-16.8220954270744,17.4610719963788,4.64781136383888));
#62499=CARTESIAN_POINT('Ctrl Pts',(-16.1507859818905,18.64162416143,5.41417782127868));
#62500=CARTESIAN_POINT('Ctrl Pts',(-17.7089990632976,18.6472699541193,5.44803201127134));
#62501=CARTESIAN_POINT('Ctrl Pts',(-16.8215276491358,17.5299062590181,4.55186134052271));
#62502=CARTESIAN_POINT('Ctrl Pts',(-16.1561810404284,18.6758805436289,5.36460911067975));
#62503=CARTESIAN_POINT('Ctrl Pts',(-17.709737672067,18.6980744122179,5.37368742584704));
#62504=CARTESIAN_POINT('Ctrl Pts',(-16.8137088203987,17.6765330986877,4.36681604087379));
#62505=CARTESIAN_POINT('Ctrl Pts',(-16.1648649353469,18.7484754011972,5.26511564077504));
#62506=CARTESIAN_POINT('Ctrl Pts',(-17.7043582887925,18.8062737645121,5.23031280416359));
#62507=CARTESIAN_POINT('Ctrl Pts',(-16.8064567973355,17.7543260220656,4.27772105086972));
#62508=CARTESIAN_POINT('Ctrl Pts',(-16.1681498046237,18.7866860991184,5.21534216184175));
#62509=CARTESIAN_POINT('Ctrl Pts',(-17.6982392734343,18.863668906634,5.16128300573129));
#62510=CARTESIAN_POINT('Ctrl Pts',(-16.7908108551635,17.8777735500095,4.14924084351727));
#62511=CARTESIAN_POINT('Ctrl Pts',(-16.1710402262194,18.8483363059671,5.13994566835684));
#62512=CARTESIAN_POINT('Ctrl Pts',(-17.6841764321443,18.9547385014575,5.06173621213073));
#62513=CARTESIAN_POINT('Ctrl Pts',(-16.7847994760353,17.9200509798971,4.10727592102829));
#62514=CARTESIAN_POINT('Ctrl Pts',(-16.1716622035887,18.869516190848,5.11480160040562));
#62515=CARTESIAN_POINT('Ctrl Pts',(-17.6786733100718,18.9859259149757,5.02922140144999));
#62516=CARTESIAN_POINT('Ctrl Pts',(-16.7763053981147,17.9743268356373,4.05591029156792));
#62517=CARTESIAN_POINT('Ctrl Pts',(-16.171956931833,18.8970271211957,5.08321199995914));
#62518=CARTESIAN_POINT('Ctrl Pts',(-17.6707913903831,19.0259631606368,4.98942219883545));
#62519=CARTESIAN_POINT('Ctrl Pts',(-16.7745575630922,17.9852534999052,4.04569172176441));
#62520=CARTESIAN_POINT('Ctrl Pts',(-16.1719917095952,18.9025678356017,5.07690116321743));
#62521=CARTESIAN_POINT('Ctrl Pts',(-17.6691648279995,19.0340232881386,4.98150459759356));
#62522=CARTESIAN_POINT('Ctrl Pts',(-16.7709641270619,18.0072504455116,4.02536414779665));
#62523=CARTESIAN_POINT('Ctrl Pts',(-16.1720115721074,18.9137499738595,5.06427051983082));
#62524=CARTESIAN_POINT('Ctrl Pts',(-17.6658116455112,19.050249378955,4.9657542197225));
#62525=CARTESIAN_POINT('Ctrl Pts',(-16.7691176506656,18.0183255954815,4.01525090736688));
#62526=CARTESIAN_POINT('Ctrl Pts',(-16.1719966680687,18.9193935894147,5.05794822246791));
#62527=CARTESIAN_POINT('Ctrl Pts',(-17.6640841987627,19.0584189335486,4.95791816069434));
#62528=CARTESIAN_POINT('Ctrl Pts',(-16.7634483218102,18.0516727098935,3.98516089302837));
#62529=CARTESIAN_POINT('Ctrl Pts',(-16.1718758121784,18.9364205373016,5.03903418912846));
#62530=CARTESIAN_POINT('Ctrl Pts',(-17.6587675705056,19.0830172109,4.93460335385762));
#62531=CARTESIAN_POINT('Ctrl Pts',(-16.7594911869187,18.0740941534329,3.965407621031));
#62532=CARTESIAN_POINT('Ctrl Pts',(-16.171694082726,18.9479341486161,5.02645603071105));
#62533=CARTESIAN_POINT('Ctrl Pts',(-17.6550400294926,19.09955606405,4.91929767070209));
#62534=CARTESIAN_POINT('Ctrl Pts',(-16.7388442855259,18.1871389326756,3.86814986546794));
#62535=CARTESIAN_POINT('Ctrl Pts',(-16.1702666252171,19.0060927232367,4.9640131612077));
#62536=CARTESIAN_POINT('Ctrl Pts',(-17.635514525068,19.182941342502,4.84393739128064));
#62537=CARTESIAN_POINT('Ctrl Pts',(-16.719579385685,18.2805678928541,3.79515926871854));
#62538=CARTESIAN_POINT('Ctrl Pts',(-16.1674668650467,19.0553583202436,4.91452255413311));
#62539=CARTESIAN_POINT('Ctrl Pts',(-17.6170620237919,19.251855614714,4.7873778337322));
#62540=CARTESIAN_POINT('Ctrl Pts',(-16.6760920287696,18.4732081087098,3.65836854066126));
#62541=CARTESIAN_POINT('Ctrl Pts',(-16.1580801288288,19.1600515548782,4.81721936383231));
#62542=CARTESIAN_POINT('Ctrl Pts',(-17.5750533192918,19.3939530516457,4.68137555884256));
#62543=CARTESIAN_POINT('Ctrl Pts',(-16.6518681727065,18.5724200982118,3.59456982019734));
#62544=CARTESIAN_POINT('Ctrl Pts',(-16.1515441951085,19.2153318690365,4.76945799524684));
#62545=CARTESIAN_POINT('Ctrl Pts',(-17.5514956562874,19.4671367442649,4.63193394000491));
#62546=CARTESIAN_POINT('Ctrl Pts',(-16.6120711601853,18.7255472795203,3.50564398372098));
#62547=CARTESIAN_POINT('Ctrl Pts',(-16.1385914317911,19.3035904494646,4.69942714954636));
#62548=CARTESIAN_POINT('Ctrl Pts',(-17.5126004219238,19.5800987486598,4.56301866603759));
#62549=CARTESIAN_POINT('Ctrl Pts',(-16.598227256611,18.7773090937269,3.47713276907664));
#62550=CARTESIAN_POINT('Ctrl Pts',(-16.1337817240602,19.3337268967015,4.6764723023167));
#62551=CARTESIAN_POINT('Ctrl Pts',(-17.4990408092191,19.6182847258373,4.54092302367441));
#62552=CARTESIAN_POINT('Ctrl Pts',(-16.5766147929995,18.8560382528438,3.43606457582562));
#62553=CARTESIAN_POINT('Ctrl Pts',(-16.125752890255,19.3803013963805,4.64253099430504));
#62554=CARTESIAN_POINT('Ctrl Pts',(-17.4778314381254,19.6763676751938,4.50909627003073));
#62555=CARTESIAN_POINT('Ctrl Pts',(-16.5692661085865,18.882474353998,3.42265254898412));
#62556=CARTESIAN_POINT('Ctrl Pts',(-16.1229478535309,19.3960191571751,4.63132270544163));
#62557=CARTESIAN_POINT('Ctrl Pts',(-17.4706132806969,19.6958714905778,4.49870236157246));
#62558=CARTESIAN_POINT('Ctrl Pts',(-16.5543030537792,18.9356607661424,3.39642157189387));
#62559=CARTESIAN_POINT('Ctrl Pts',(-16.1170726225119,19.4278597569896,4.60912436043551));
#62560=CARTESIAN_POINT('Ctrl Pts',(-17.455903407128,19.7351118543264,4.47837438560283));
#62561=CARTESIAN_POINT('Ctrl Pts',(-16.5467098413558,18.9623361970568,3.38363919167274));
#62562=CARTESIAN_POINT('Ctrl Pts',(-16.1140117884356,19.4439357929648,4.59816504831983));
#62563=CARTESIAN_POINT('Ctrl Pts',(-17.4484324969103,19.7547931562087,4.46846865770835));
#62564=CARTESIAN_POINT('Ctrl Pts',(-16.508202977113,19.0961201099036,3.3213639916356));
#62565=CARTESIAN_POINT('Ctrl Pts',(-16.098169889326,19.524689281414,4.54436605394745));
#62566=CARTESIAN_POINT('Ctrl Pts',(-17.4105164892993,19.8535022542627,4.42020926695778));
#62567=CARTESIAN_POINT('Ctrl Pts',(-16.4756732929089,19.2044463729661,3.27676843062349));
#62568=CARTESIAN_POINT('Ctrl Pts',(-16.0834884075578,19.5920801013394,4.50338912963289));
#62569=CARTESIAN_POINT('Ctrl Pts',(-17.3783936837892,19.9334359956607,4.38565331806935));
#62570=CARTESIAN_POINT('Ctrl Pts',(-16.4075080632038,19.4236276169736,3.19750638204053));
#62571=CARTESIAN_POINT('Ctrl Pts',(-16.0501955905981,19.7318341839477,4.42667684719545));
#62572=CARTESIAN_POINT('Ctrl Pts',(-17.3109257615026,20.0951899517967,4.32425010281472));
#62573=CARTESIAN_POINT('Ctrl Pts',(-16.3718715237024,19.5344829234921,3.16284173499306));
#62574=CARTESIAN_POINT('Ctrl Pts',(-16.0316406956358,19.8041162452577,4.39087890945558));
#62575=CARTESIAN_POINT('Ctrl Pts',(-17.2755796078532,20.1770103953973,4.29740425493055));
#62576=CARTESIAN_POINT('Ctrl Pts',(-16.297689249875,19.7587108437685,3.10321810060762));
#62577=CARTESIAN_POINT('Ctrl Pts',(-15.9906690323896,19.9534816196041,4.32512422071333));
#62578=CARTESIAN_POINT('Ctrl Pts',(-17.2018700972943,20.3425337283146,4.25125855596935));
#62579=CARTESIAN_POINT('Ctrl Pts',(-16.2591431712307,19.8720835434029,3.07825968438735));
#62580=CARTESIAN_POINT('Ctrl Pts',(-15.9683052469682,20.0304964466515,4.29509127689048));
#62581=CARTESIAN_POINT('Ctrl Pts',(-17.163506384661,20.4262366718118,4.23195913303276));
#62582=CARTESIAN_POINT('Ctrl Pts',(-16.2091884282023,20.0153974657703,3.05314750912563));
#62583=CARTESIAN_POINT('Ctrl Pts',(-15.9378084682126,20.13015180225,4.26142632520722));
#62584=CARTESIAN_POINT('Ctrl Pts',(-17.1137137415339,20.5320627708622,4.21257430606212));
#62585=CARTESIAN_POINT('Ctrl Pts',(-16.1991200546222,20.0441069891588,3.0484364867405));
#62586=CARTESIAN_POINT('Ctrl Pts',(-15.9316281716696,20.1501045344835,4.2549337075549));
#62587=CARTESIAN_POINT('Ctrl Pts',(-17.1036744360849,20.5532633748179,4.20893982211271));
#62588=CARTESIAN_POINT('Ctrl Pts',(-16.1788950376696,20.101436421715,3.03965994049603));
#62589=CARTESIAN_POINT('Ctrl Pts',(-15.9190872506462,20.1901176618968,4.24241030450447));
#62590=CARTESIAN_POINT('Ctrl Pts',(-17.0835007615317,20.5956001829815,4.20217346458416));
#62591=CARTESIAN_POINT('Ctrl Pts',(-16.1687290012613,20.1300833200632,3.03558960937044));
#62592=CARTESIAN_POINT('Ctrl Pts',(-15.9127214251302,20.2101966625484,4.23637156842712));
#62593=CARTESIAN_POINT('Ctrl Pts',(-17.0733570306589,20.6167563162349,4.19903787894888));
#62594=CARTESIAN_POINT('Ctrl Pts',(-16.1380734967344,20.2159716731412,3.02431921476223));
#62595=CARTESIAN_POINT('Ctrl Pts',(-15.8933731832392,20.270545713034,4.21895892653054));
#62596=CARTESIAN_POINT('Ctrl Pts',(-17.0427584915315,20.680188767493,4.1903639156326));
#62597=CARTESIAN_POINT('Ctrl Pts',(-16.1174268255799,20.27316083266,3.01805921896905));
#62598=CARTESIAN_POINT('Ctrl Pts',(-15.8800805679254,20.3111220050017,4.20822312872908));
#62599=CARTESIAN_POINT('Ctrl Pts',(-17.0221365311604,20.7224291906978,4.18555791480855));
#62600=CARTESIAN_POINT('Ctrl Pts',(-16.0965766384649,20.3302824207005,3.01302436959042));
#62601=CARTESIAN_POINT('Ctrl Pts',(-15.8663823430535,20.3520823377266,4.19836680673276));
#62602=CARTESIAN_POINT('Ctrl Pts',(-17.0012980588419,20.7646233900099,4.18170722839425));
#62603=CARTESIAN_POINT('Origin',(-31.4,21.,7.));
#62604=CARTESIAN_POINT('',(-31.7,19.3924770032404,8.64926829419482));
#62605=CARTESIAN_POINT('Ctrl Pts',(-31.4046869279001,19.0836514699531,8.7616715958928));
#62606=CARTESIAN_POINT('Ctrl Pts',(-31.4396270223971,19.0842071229975,8.76146935472406));
#62607=CARTESIAN_POINT('Ctrl Pts',(-31.4796949749373,19.0925507901701,8.75843250822859));
#62608=CARTESIAN_POINT('Ctrl Pts',(-31.5457246229044,19.1194392293618,8.74864591671695));
#62609=CARTESIAN_POINT('Ctrl Pts',(-31.5824397836614,19.143919114572,8.73973596716218));
#62610=CARTESIAN_POINT('Ctrl Pts',(-31.6356608467856,19.1964897272736,8.72060182894167));
#62611=CARTESIAN_POINT('Ctrl Pts',(-31.6609177668595,19.2344479852018,8.70678615291121));
#62612=CARTESIAN_POINT('Ctrl Pts',(-31.6908725620847,19.3060567911241,8.68072267904415));
#62613=CARTESIAN_POINT('Ctrl Pts',(-31.7,19.3528406701053,8.66369473965147));
#62614=CARTESIAN_POINT('Ctrl Pts',(-31.7,19.3924770032404,8.64926829419483));
#62615=CARTESIAN_POINT('',(-31.7,23.291563283411,7.23011694737699));
#62616=CARTESIAN_POINT('Ctrl Pts',(-31.7,23.291563283411,7.23011694737701));
#62617=CARTESIAN_POINT('Ctrl Pts',(-31.7,23.3311996165461,7.21569050192038));
#62618=CARTESIAN_POINT('Ctrl Pts',(-31.6908725620847,23.3779834955273,7.1986625625277));
#62619=CARTESIAN_POINT('Ctrl Pts',(-31.6609177668595,23.4495923014496,7.17259908866064));
#62620=CARTESIAN_POINT('Ctrl Pts',(-31.6356608467856,23.4875505593778,7.15878341263018));
#62621=CARTESIAN_POINT('Ctrl Pts',(-31.5824397836614,23.5401211720794,7.13964927440967));
#62622=CARTESIAN_POINT('Ctrl Pts',(-31.5457246229044,23.5646010572896,7.1307393248549));
#62623=CARTESIAN_POINT('Ctrl Pts',(-31.4796949749373,23.5914894964812,7.12095273334326));
#62624=CARTESIAN_POINT('Ctrl Pts',(-31.4396270223971,23.5998331636539,7.11791588684779));
#62625=CARTESIAN_POINT('Ctrl Pts',(-31.4046869279001,23.6003888166983,7.11771364567905));
#62626=CARTESIAN_POINT('Origin',(-31.7,21.,7.));
#62627=CARTESIAN_POINT('Origin',(-29.,20.5,7.));
#62628=CARTESIAN_POINT('Origin',(-29.,21.5,7.));
#62629=CARTESIAN_POINT('Origin',(-31.7,21.,7.));
#62630=CARTESIAN_POINT('',(-31.7,23.6912516952905,7.08464226247173));
#62631=CARTESIAN_POINT('Origin',(-31.7,23.6912516952905,7.08464226247173));
#62632=CARTESIAN_POINT('Origin',(-50.,41.5,-36.5));
#62633=CARTESIAN_POINT('',(-35.6221012801966,49.1231323076242,-24.5));
#62634=CARTESIAN_POINT('',(-50.,49.1231323076242,-24.5));
#62635=CARTESIAN_POINT('',(-27.3778987198034,49.1231323076242,-24.5));
#62636=CARTESIAN_POINT('Origin',(-31.5,50.9282032302755,-21.6585366490161));
#62637=CARTESIAN_POINT('',(-50.,49.1231323076242,-24.5));
#62638=CARTESIAN_POINT('Origin',(-31.5,50.9282032302755,-35.7491074993019));
#62639=CARTESIAN_POINT('Origin',(-31.5,50.9282032302755,-24.5));
#62640=CARTESIAN_POINT('Origin',(-37.,54.4282032302755,-24.5));
#62956=UNCERTAINTY_MEASURE_WITH_UNIT(LENGTH_MEASURE(0.01),#62975,
'DISTANCE_ACCURACY_VALUE',
'Maximum model space distance between geometric entities at asserted c
onnectivities');
#62960=UNCERTAINTY_MEASURE_WITH_UNIT(LENGTH_MEASURE(0.01),#62975,
'DISTANCE_ACCURACY_VALUE',
'Maximum model space distance between geometric entities at asserted c
onnectivities');
#62970=(
GEOMETRIC_REPRESENTATION_CONTEXT(3)
GLOBAL_UNCERTAINTY_ASSIGNED_CONTEXT((#62956))
GLOBAL_UNIT_ASSIGNED_CONTEXT((#62975,#62977,#62978))
REPRESENTATION_CONTEXT('','3D')
);
#62974=(
GEOMETRIC_REPRESENTATION_CONTEXT(3)
GLOBAL_UNCERTAINTY_ASSIGNED_CONTEXT((#62960))
GLOBAL_UNIT_ASSIGNED_CONTEXT((#62975,#62977,#62978))
REPRESENTATION_CONTEXT('','3D')
);
#62975=(
LENGTH_UNIT()
NAMED_UNIT(*)
SI_UNIT(.MILLI.,.METRE.)
);
#62977=(
NAMED_UNIT(*)
PLANE_ANGLE_UNIT()
SI_UNIT($,.RADIAN.)
);
#62978=(
NAMED_UNIT(*)
SI_UNIT($,.STERADIAN.)
SOLID_ANGLE_UNIT()
);
#62988=SHAPE_DEFINITION_REPRESENTATION(#63001,#63029);
#63001=PRODUCT_DEFINITION_SHAPE('',$,#63043);
#63029=SHAPE_REPRESENTATION('',(#16488),#62970);
#63033=PRODUCT_DEFINITION_CONTEXT('part definition',#63074,'design');
#63043=PRODUCT_DEFINITION('Throttle Body Housing',
'Throttle Body Housing',#63056,#63033);
#63056=PRODUCT_DEFINITION_FORMATION('',$,#63085);
#63074=APPLICATION_CONTEXT(
'Core Data for Automotive Mechanical Design Process');
#63075=PRODUCT_CONTEXT('part definition',#63074,'mechanical');
#63085=PRODUCT('Throttle Body Housing','Throttle Body Housing',$,(#63075));
#63090=PRESENTATION_STYLE_ASSIGNMENT((#63092));
#63092=SURFACE_STYLE_USAGE(.BOTH.,#63094);
#63094=SURFACE_SIDE_STYLE('',(#63096));
#63096=SURFACE_STYLE_FILL_AREA(#63098);
#63098=FILL_AREA_STYLE('Opaque(202,209,238)',(#63100));
#63100=FILL_AREA_STYLE_COLOUR('Opaque(202,209,238)',#63102);
#63102=COLOUR_RGB('Opaque(202,209,238)', 0.66274510, 0.83137255, 0.94901961);
ENDSEC;
END-ISO-10303-21;
